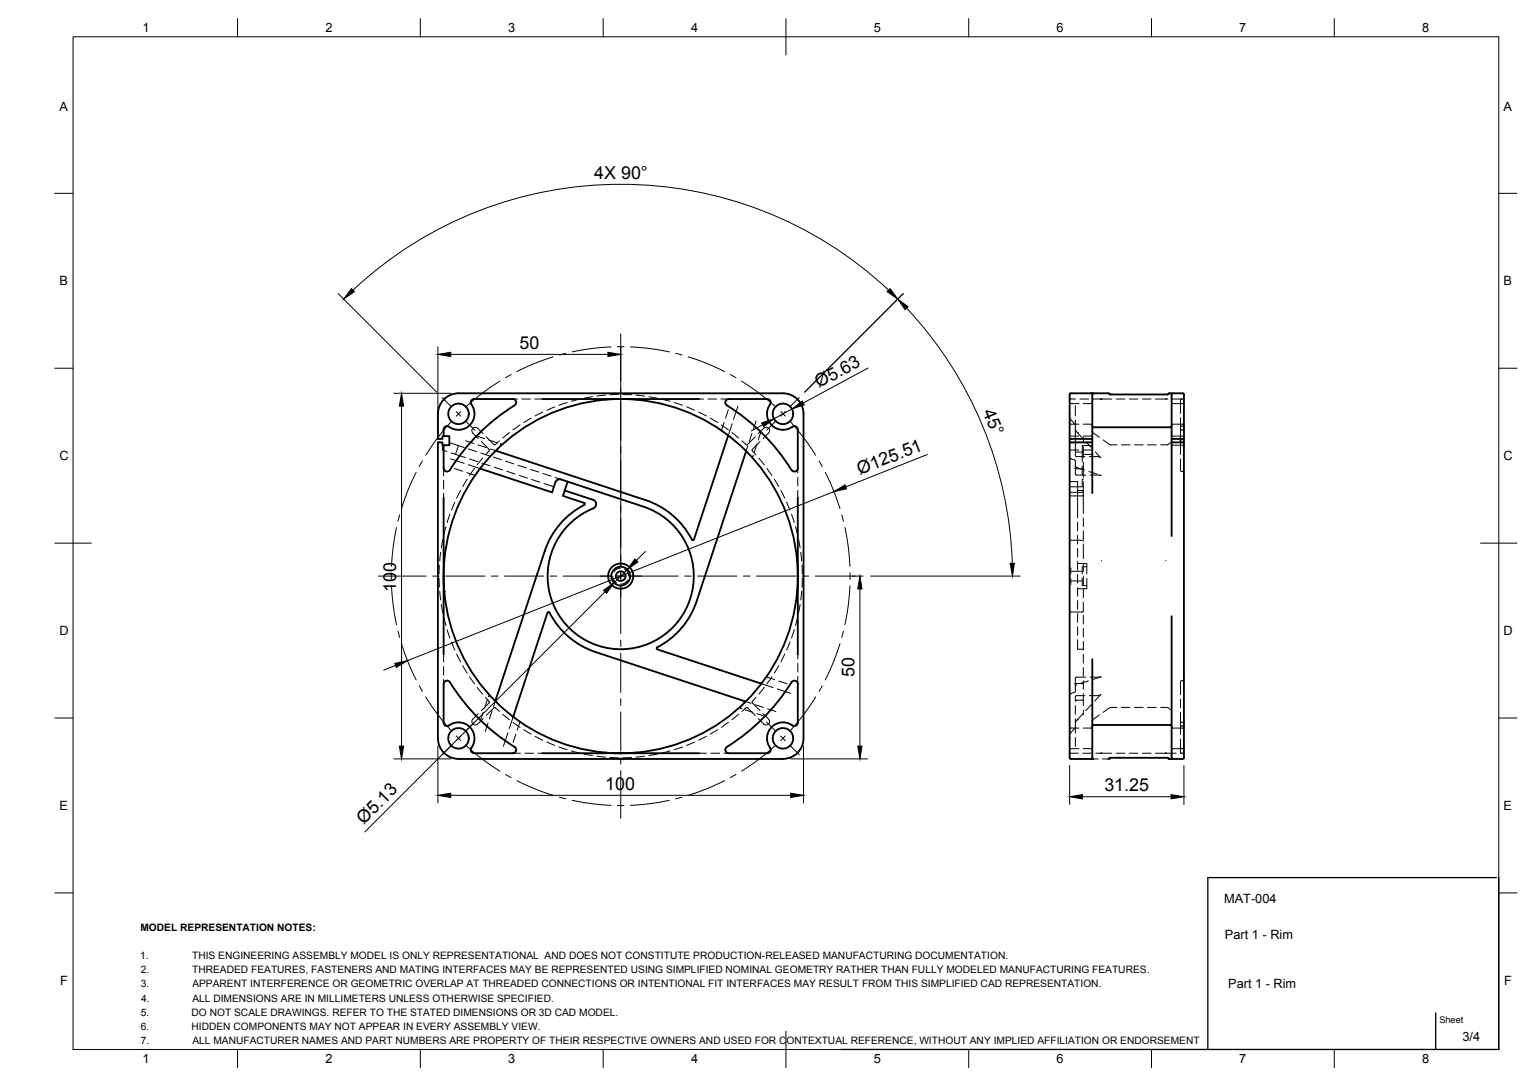
ISO-10303-21;
HEADER;
/* Generated by software containing ST-Developer
 * from STEP Tools, Inc. (www.steptools.com) 
 */

FILE_DESCRIPTION(
/* description */ ('STEP AP214'),
/* implementation_level */ '2;1');

FILE_NAME(
/* name */ 'Part 1 - Rim.step',
/* time_stamp */ '2026-11-14T05:34:33-08:00',
/* author */ (''),
/* organization */ (''),
/* preprocessor_version */ 'ST-DEVELOPER v20.2',
/* originating_system */ 'Autodesk Translation Framework v15.17.0.0',
/* authorisation */ '');

FILE_SCHEMA (('AUTOMOTIVE_DESIGN { 1 0 10303 214 3 1 1 }'));
ENDSEC;

DATA;
#10=MECHANICAL_DESIGN_GEOMETRIC_PRESENTATION_REPRESENTATION('',(#23),#37625);
#19=SHAPE_REPRESENTATION_RELATIONSHIP('SRR','None',#37639,#21);
#21=ADVANCED_BREP_SHAPE_REPRESENTATION('',(#25),#37623);
#23=STYLED_ITEM('',(#37658),#25);
#25=MANIFOLD_SOLID_BREP('Body1',#11497);
#27=SPHERICAL_SURFACE('',#12271,0.3125);
#28=SPHERICAL_SURFACE('',#12276,0.3125);
#29=SPHERICAL_SURFACE('',#12302,0.3125);
#30=SPHERICAL_SURFACE('',#12304,0.3125);
#31=SPHERICAL_SURFACE('',#12340,0.3125);
#32=SPHERICAL_SURFACE('',#12342,0.3125);
#33=SPHERICAL_SURFACE('',#12382,0.3125);
#34=SPHERICAL_SURFACE('',#12385,0.3125);
#35=SPHERICAL_SURFACE('',#12394,0.3125);
#36=SPHERICAL_SURFACE('',#12396,0.3125);
#37=SPHERICAL_SURFACE('',#12445,0.3125);
#38=SPHERICAL_SURFACE('',#12447,0.3125);
#39=SPHERICAL_SURFACE('',#12466,0.3125);
#40=SPHERICAL_SURFACE('',#12481,0.3125);
#41=SPHERICAL_SURFACE('',#12525,0.3125);
#42=SPHERICAL_SURFACE('',#12532,0.3125);
#43=SPHERICAL_SURFACE('',#12539,0.3125);
#44=SPHERICAL_SURFACE('',#12541,0.3125);
#45=SPHERICAL_SURFACE('',#12549,0.3125);
#46=SPHERICAL_SURFACE('',#12552,0.3125);
#47=SPHERICAL_SURFACE('',#12570,0.3125);
#48=SPHERICAL_SURFACE('',#12573,0.3125);
#49=SPHERICAL_SURFACE('',#12575,0.3125);
#50=SPHERICAL_SURFACE('',#12580,0.3125);
#51=SPHERICAL_SURFACE('',#12597,0.3125);
#52=SPHERICAL_SURFACE('',#12605,0.3125);
#53=SPHERICAL_SURFACE('',#12628,0.3125);
#54=SPHERICAL_SURFACE('',#12633,0.3125);
#55=SPHERICAL_SURFACE('',#12637,0.3125);
#56=SPHERICAL_SURFACE('',#12640,0.3125);
#57=SPHERICAL_SURFACE('',#12665,0.3125);
#58=SPHERICAL_SURFACE('',#12668,0.3125);
#59=SPHERICAL_SURFACE('',#12674,0.3125);
#60=SPHERICAL_SURFACE('',#12676,0.3125);
#61=SPHERICAL_SURFACE('',#12702,0.3125);
#62=SPHERICAL_SURFACE('',#12704,0.3125);
#63=SPHERICAL_SURFACE('',#12706,0.3125);
#64=SPHERICAL_SURFACE('',#12711,0.3125);
#65=SPHERICAL_SURFACE('',#12733,0.3125);
#66=SPHERICAL_SURFACE('',#12735,0.3125);
#67=SPHERICAL_SURFACE('',#12759,0.3125);
#68=SPHERICAL_SURFACE('',#12761,0.3125);
#69=SPHERICAL_SURFACE('',#12763,0.3125);
#70=SPHERICAL_SURFACE('',#12765,0.3125);
#71=SPHERICAL_SURFACE('',#12779,0.3125);
#72=SPHERICAL_SURFACE('',#12781,0.3125);
#73=SPHERICAL_SURFACE('',#12788,0.3125);
#74=SPHERICAL_SURFACE('',#12790,0.3125);
#75=(
BOUNDED_SURFACE()
B_SPLINE_SURFACE(3,2,((#23896,#23897,#23898),(#23899,#23900,#23901),(#23902,
#23903,#23904),(#23905,#23906,#23907)),.UNSPECIFIED.,.F.,.F.,.F.)
B_SPLINE_SURFACE_WITH_KNOTS((4,4),(3,3),(0.0326127356995135,0.0421285143028756),
(0.,1.),.UNSPECIFIED.)
GEOMETRIC_REPRESENTATION_ITEM()
RATIONAL_B_SPLINE_SURFACE(((1.,0.77336849210705,1.),(1.,0.770480922349025,
1.),(1.,0.767957745429666,1.),(1.,0.765689104422505,1.)))
REPRESENTATION_ITEM('')
SURFACE()
);
#76=(
BOUNDED_SURFACE()
B_SPLINE_SURFACE(3,2,((#23985,#23986,#23987),(#23988,#23989,#23990),(#23991,
#23992,#23993),(#23994,#23995,#23996),(#23997,#23998,#23999),(#24000,#24001,
#24002),(#24003,#24004,#24005),(#24006,#24007,#24008)),.UNSPECIFIED.,.F.,
 .F.,.F.)
B_SPLINE_SURFACE_WITH_KNOTS((4,2,2,4),(3,3),(0.000802853902805026,0.00108948501086238,
0.00137611611891974,0.00194937833503446),(0.,1.),.UNSPECIFIED.)
GEOMETRIC_REPRESENTATION_ITEM()
RATIONAL_B_SPLINE_SURFACE(((1.,0.923879532511285,1.),(1.,0.93126028758527,
1.),(1.,0.931596165488004,1.),(1.,0.918734528780574,1.),(1.,0.905994810924641,
1.),(1.,0.858462949893107,1.),(1.,0.814112175968656,1.),(1.,0.765689104422502,
1.)))
REPRESENTATION_ITEM('')
SURFACE()
);
#77=(
BOUNDED_SURFACE()
B_SPLINE_SURFACE(3,2,((#24068,#24069,#24070),(#24071,#24072,#24073),(#24074,
#24075,#24076),(#24077,#24078,#24079),(#24080,#24081,#24082),(#24083,#24084,
#24085),(#24086,#24087,#24088),(#24089,#24090,#24091)),.UNSPECIFIED.,.F.,
 .F.,.F.)
B_SPLINE_SURFACE_WITH_KNOTS((4,2,2,4),(3,3),(0.000686358375502128,0.000929437613321109,
0.00117251685114009,0.00165867532677805),(0.,1.),.UNSPECIFIED.)
GEOMETRIC_REPRESENTATION_ITEM()
RATIONAL_B_SPLINE_SURFACE(((1.,0.923879532511287,1.),(1.,0.92889985757716,
1.),(1.,0.929018384212628,1.),(1.,0.920008474882563,1.),(1.,0.910871684991149,
1.),(1.,0.87513924549097,1.),(1.,0.84081307837336,1.),(1.,0.802338883728525,
1.)))
REPRESENTATION_ITEM('')
SURFACE()
);
#78=(
BOUNDED_SURFACE()
B_SPLINE_SURFACE(3,2,((#24101,#24102,#24103),(#24104,#24105,#24106),(#24107,
#24108,#24109),(#24110,#24111,#24112),(#24113,#24114,#24115),(#24116,#24117,
#24118),(#24119,#24120,#24121),(#24122,#24123,#24124),(#24125,#24126,#24127),
(#24128,#24129,#24130)),.UNSPECIFIED.,.F.,.F.,.F.)
B_SPLINE_SURFACE_WITH_KNOTS((4,2,2,2,4),(3,3),(0.0314170682308584,0.0383717968941293,
0.0418491612257648,0.0453265255574003,0.0592359828839421),(0.,1.00015514532272),
 .UNSPECIFIED.)
GEOMETRIC_REPRESENTATION_ITEM()
RATIONAL_B_SPLINE_SURFACE(((1.,0.893712741719904,1.00003297994197),(1.,
0.896924595267972,1.00003198333386),(1.,0.900137133821891,1.0000309865132),
(1.,0.904798383538125,1.00002954017102),(1.,0.906325496636901,1.00002906632211),
(1.,0.909290323001115,1.00002814636422),(1.,0.910726187593686,1.00002770082887),
(1.,0.917498844645671,1.00002559933674),(1.,0.921671404518462,1.00002430463045),
(1.,0.923199103012375,1.0000238305999)))
REPRESENTATION_ITEM('')
SURFACE()
);
#79=(
BOUNDED_SURFACE()
B_SPLINE_SURFACE(3,2,((#24156,#24157,#24158),(#24159,#24160,#24161),(#24162,
#24163,#24164),(#24165,#24166,#24167),(#24168,#24169,#24170),(#24171,#24172,
#24173),(#24174,#24175,#24176),(#24177,#24178,#24179),(#24180,#24181,#24182),
(#24183,#24184,#24185)),.UNSPECIFIED.,.F.,.F.,.F.)
B_SPLINE_SURFACE_WITH_KNOTS((4,2,2,2,4),(3,3),(0.0303364035364412,0.0372910338575461,
0.0407683490180985,0.0442456641786509,0.0581549248208605),(0.,1.),
 .UNSPECIFIED.)
GEOMETRIC_REPRESENTATION_ITEM()
RATIONAL_B_SPLINE_SURFACE(((1.,0.893729285230293,1.),(1.,0.8969398694082,
1.),(1.,0.900150686104865,1.),(1.,0.904808789101856,1.),(1.,0.906334760566901,
1.),(1.,0.909297199463308,1.),(1.,0.91073457572851,1.),(1.,0.917512859277436,
1.),(1.,0.921684639637439,1.),(1.,0.923210992612934,1.)))
REPRESENTATION_ITEM('')
SURFACE()
);
#80=(
BOUNDED_SURFACE()
B_SPLINE_SURFACE(3,2,((#24220,#24221,#24222),(#24223,#24224,#24225),(#24226,
#24227,#24228),(#24229,#24230,#24231),(#24232,#24233,#24234),(#24235,#24236,
#24237)),.UNSPECIFIED.,.F.,.F.,.F.)
B_SPLINE_SURFACE_WITH_KNOTS((4,2,4),(3,3),(0.000158496916905221,0.000711650690198974,
0.00126480446349273),(0.,1.),.UNSPECIFIED.)
GEOMETRIC_REPRESENTATION_ITEM()
RATIONAL_B_SPLINE_SURFACE(((1.,0.707106781186549,1.),(1.,0.750150820630032,
1.),(1.,0.789088418359452,1.),(1.,0.861437064777228,1.),(1.,0.895323131481853,
1.),(1.,0.92387953251129,1.)))
REPRESENTATION_ITEM('')
SURFACE()
);
#81=(
BOUNDED_SURFACE()
B_SPLINE_SURFACE(3,2,((#24242,#24243,#24244),(#24245,#24246,#24247),(#24248,
#24249,#24250),(#24251,#24252,#24253),(#24254,#24255,#24256),(#24257,#24258,
#24259),(#24260,#24261,#24262),(#24263,#24264,#24265)),.UNSPECIFIED.,.F.,
 .F.,.F.)
B_SPLINE_SURFACE_WITH_KNOTS((4,2,2,4),(3,3),(0.000174437971377146,0.00101920216019031,
0.00137118723886246,0.00186396634900332),(0.,1.00024356555363),
 .UNSPECIFIED.)
GEOMETRIC_REPRESENTATION_ITEM()
RATIONAL_B_SPLINE_SURFACE(((1.,0.539098756316927,1.00022451933317),(1.,
0.633858154865208,1.00017835908243),(1.,0.717178341053912,1.00013777122788),
(1.,0.814824555144991,1.00009020471949),(1.,0.841538081526998,1.0000771917298),
(1.,0.898531920368047,1.00004942825798),(1.,0.925786672706503,1.0000361516203),
(1.,0.937456960617578,1.00003046666003)))
REPRESENTATION_ITEM('')
SURFACE()
);
#82=(
BOUNDED_SURFACE()
B_SPLINE_SURFACE(3,2,((#24441,#24442,#24443),(#24444,#24445,#24446),(#24447,
#24448,#24449),(#24450,#24451,#24452),(#24453,#24454,#24455),(#24456,#24457,
#24458)),.UNSPECIFIED.,.F.,.F.,.F.)
B_SPLINE_SURFACE_WITH_KNOTS((4,2,4),(3,3),(0.000796035510927852,0.00146280219164561,
0.00212956887236337),(0.,1.00047905246342),.UNSPECIFIED.)
GEOMETRIC_REPRESENTATION_ITEM()
RATIONAL_B_SPLINE_SURFACE(((1.,0.680382792871542,1.00030622682085),(1.,
0.734649451169007,1.00025423366818),(1.,0.782184849656497,1.00020868976868),
(1.,0.8686687938328,1.00012582907568),(1.,0.90836300942771,1.00008779785215),
(1.,0.940539343963641,1.0000569695475)))
REPRESENTATION_ITEM('')
SURFACE()
);
#83=(
BOUNDED_SURFACE()
B_SPLINE_SURFACE(3,2,((#24462,#24463,#24464),(#24465,#24466,#24467),(#24468,
#24469,#24470),(#24471,#24472,#24473)),.UNSPECIFIED.,.F.,.F.,.F.)
B_SPLINE_SURFACE_WITH_KNOTS((4,4),(3,3),(0.0647248597593566,0.0667277597197425),
(0.,1.),.UNSPECIFIED.)
GEOMETRIC_REPRESENTATION_ITEM()
RATIONAL_B_SPLINE_SURFACE(((1.,0.77254330703138,1.),(1.,0.773053168552101,
1.),(1.,0.773574707201174,1.),(1.,0.774108727913442,1.)))
REPRESENTATION_ITEM('')
SURFACE()
);
#84=(
BOUNDED_SURFACE()
B_SPLINE_SURFACE(3,2,((#24557,#24558,#24559),(#24560,#24561,#24562),(#24563,
#24564,#24565),(#24566,#24567,#24568)),.UNSPECIFIED.,.F.,.F.,.F.)
B_SPLINE_SURFACE_WITH_KNOTS((4,4),(3,3),(0.0554293707990946,0.067219986976584),
(0.,1.00093204202966),.UNSPECIFIED.)
GEOMETRIC_REPRESENTATION_ITEM()
RATIONAL_B_SPLINE_SURFACE(((1.,0.586730971631016,1.00077036820799),(1.,
0.580458668850621,1.00078206030762),(1.,0.573277155045983,1.00079544725303),
(1.,0.564689221730742,1.00081145588262)))
REPRESENTATION_ITEM('')
SURFACE()
);
#85=(
BOUNDED_SURFACE()
B_SPLINE_SURFACE(3,2,((#24588,#24589,#24590),(#24591,#24592,#24593),(#24594,
#24595,#24596),(#24597,#24598,#24599),(#24600,#24601,#24602),(#24603,#24604,
#24605),(#24606,#24607,#24608),(#24609,#24610,#24611),(#24612,#24613,#24614),
(#24615,#24616,#24617)),.UNSPECIFIED.,.F.,.F.,.F.)
B_SPLINE_SURFACE_WITH_KNOTS((4,2,2,2,4),(3,3),(0.000140109886117696,0.000666559814939625,
0.00108521714444999,0.00150387447396035,0.00203032440278269),(-0.000871030384560204,
1.),.UNSPECIFIED.)
GEOMETRIC_REPRESENTATION_ITEM()
RATIONAL_B_SPLINE_SURFACE(((1.00092572483597,0.468603591574399,1.),(1.00081905401985,
0.5298361375373,1.),(1.00071568618447,0.589172664263207,1.),(1.00054995854446,
0.684305763488853,1.),(1.00048250324099,0.723027319401472,1.),(1.00035800741942,
0.794492002940391,1.),(1.00030258788071,0.826304635251683,1.),(1.00018948908564,
0.891227051893231,1.),(1.00013836850255,0.920571942721851,1.),(1.00011502671673,
0.933970893113149,1.)))
REPRESENTATION_ITEM('')
SURFACE()
);
#86=(
BOUNDED_SURFACE()
B_SPLINE_SURFACE(3,2,((#24621,#24622,#24623),(#24624,#24625,#24626),(#24627,
#24628,#24629),(#24630,#24631,#24632)),.UNSPECIFIED.,.F.,.F.,.F.)
B_SPLINE_SURFACE_WITH_KNOTS((4,4),(3,3),(0.0554293708282248,0.0672199869474538),
(0.,1.00093204200053),.UNSPECIFIED.)
GEOMETRIC_REPRESENTATION_ITEM()
RATIONAL_B_SPLINE_SURFACE(((1.,0.586730971596549,1.00077036818398),(1.,
0.580458668842862,1.00078206028319),(1.,0.573277155072649,1.00079544722812),
(1.,0.564689221807079,1.00081145585712)))
REPRESENTATION_ITEM('')
SURFACE()
);
#87=(
BOUNDED_SURFACE()
B_SPLINE_SURFACE(3,2,((#24651,#24652,#24653),(#24654,#24655,#24656),(#24657,
#24658,#24659),(#24660,#24661,#24662),(#24663,#24664,#24665),(#24666,#24667,
#24668)),.UNSPECIFIED.,.F.,.F.,.F.)
B_SPLINE_SURFACE_WITH_KNOTS((4,2,4),(3,3),(0.000315513320331966,0.000961720209151386,
0.00160792712680523),(-0.00216992936483643,1.),.UNSPECIFIED.)
GEOMETRIC_REPRESENTATION_ITEM()
RATIONAL_B_SPLINE_SURFACE(((1.00140856318051,0.675435706956244,1.),(1.00113480498433,
0.73851568564515,1.),(1.00088601384726,0.795842698473231,1.),(1.00048533380217,
0.888168294775817,1.),(1.00032603746989,0.924873713592471,1.),(1.00031273915803,
0.927937940493073,1.)))
REPRESENTATION_ITEM('')
SURFACE()
);
#88=(
BOUNDED_SURFACE()
B_SPLINE_SURFACE(3,2,((#24670,#24671,#24672),(#24673,#24674,#24675),(#24676,
#24677,#24678),(#24679,#24680,#24681),(#24682,#24683,#24684),(#24685,#24686,
#24687)),.UNSPECIFIED.,.F.,.F.,.F.)
B_SPLINE_SURFACE_WITH_KNOTS((4,2,4),(3,3),(0.000402895580047919,0.000905401753400751,
0.00140790792675358),(0.,1.),.UNSPECIFIED.)
GEOMETRIC_REPRESENTATION_ITEM()
RATIONAL_B_SPLINE_SURFACE(((1.,0.813540597401216,1.),(1.,0.813784197152837,
1.),(1.,0.801974141898952,1.),(1.,0.763153562323537,1.),(1.,0.735816595983232,
1.),(1.,0.707106781186551,1.)))
REPRESENTATION_ITEM('')
SURFACE()
);
#89=(
BOUNDED_SURFACE()
B_SPLINE_SURFACE(3,2,((#24694,#24695,#24696),(#24697,#24698,#24699),(#24700,
#24701,#24702),(#24703,#24704,#24705),(#24706,#24707,#24708),(#24709,#24710,
#24711)),.UNSPECIFIED.,.F.,.F.,.F.)
B_SPLINE_SURFACE_WITH_KNOTS((4,2,4),(3,3),(0.000800222346544408,0.00146699934948425,
0.00213377635242409),(0.,1.0004790524742),.UNSPECIFIED.)
GEOMETRIC_REPRESENTATION_ITEM()
RATIONAL_B_SPLINE_SURFACE(((1.,0.680382792868073,1.00030622682775),(1.,
0.73464945116617,1.0002542336739),(1.,0.782184849654142,1.00020868977338),
(1.,0.868668793831392,1.00012582907851),(1.,0.908363009426711,1.00008779785413),
(1.,0.940539343963006,1.00005696954878)))
REPRESENTATION_ITEM('')
SURFACE()
);
#90=(
BOUNDED_SURFACE()
B_SPLINE_SURFACE(3,2,((#24741,#24742,#24743),(#24744,#24745,#24746),(#24747,
#24748,#24749),(#24750,#24751,#24752),(#24753,#24754,#24755),(#24756,#24757,
#24758),(#24759,#24760,#24761),(#24762,#24763,#24764),(#24765,#24766,#24767),
(#24768,#24769,#24770)),.UNSPECIFIED.,.F.,.F.,.F.)
B_SPLINE_SURFACE_WITH_KNOTS((4,2,2,2,4),(3,3),(0.0314170682308576,0.0383717968941285,
0.041849161225764,0.0453265255573995,0.0592359828839414),(0.,1.00015514533033),
 .UNSPECIFIED.)
GEOMETRIC_REPRESENTATION_ITEM()
RATIONAL_B_SPLINE_SURFACE(((1.,0.893712741719095,1.00003297994359),(1.,
0.896924595266501,1.00003198333543),(1.,0.900137133822039,1.00003098651472),
(1.,0.904798383536946,1.00002954017247),(1.,0.906325496636188,1.00002906632354),
(1.,0.909290323000425,1.0000281463656),(1.,0.910726187593075,1.00002770083023),
(1.,0.917498844644786,1.000025599338),(1.,0.921671404518056,1.00002430463164),
(1.,0.923199103011791,1.00002383060107)))
REPRESENTATION_ITEM('')
SURFACE()
);
#91=(
BOUNDED_SURFACE()
B_SPLINE_SURFACE(3,2,((#24796,#24797,#24798),(#24799,#24800,#24801),(#24802,
#24803,#24804),(#24805,#24806,#24807),(#24808,#24809,#24810),(#24811,#24812,
#24813),(#24814,#24815,#24816),(#24817,#24818,#24819),(#24820,#24821,#24822),
(#24823,#24824,#24825)),.UNSPECIFIED.,.F.,.F.,.F.)
B_SPLINE_SURFACE_WITH_KNOTS((4,2,2,2,4),(3,3),(0.0303364035364412,0.0372910338575461,
0.0407683490180985,0.0442456641786509,0.0581549248208606),(0.,1.),
 .UNSPECIFIED.)
GEOMETRIC_REPRESENTATION_ITEM()
RATIONAL_B_SPLINE_SURFACE(((1.,0.893729285230296,1.),(1.,0.89693986940752,
1.),(1.,0.900150686105771,1.),(1.,0.904808789101402,1.),(1.,0.906334760567093,
1.),(1.,0.909297199463109,1.),(1.,0.91073457572825,1.),(1.,0.917512859278478,
1.),(1.,0.921684639636655,1.),(1.,0.923210992612934,1.)))
REPRESENTATION_ITEM('')
SURFACE()
);
#92=(
BOUNDED_SURFACE()
B_SPLINE_SURFACE(3,2,((#24827,#24828,#24829),(#24830,#24831,#24832),(#24833,
#24834,#24835),(#24836,#24837,#24838),(#24839,#24840,#24841),(#24842,#24843,
#24844),(#24845,#24846,#24847),(#24848,#24849,#24850),(#24851,#24852,#24853),
(#24854,#24855,#24856)),.UNSPECIFIED.,.F.,.F.,.F.)
B_SPLINE_SURFACE_WITH_KNOTS((4,2,2,2,4),(3,3),(0.000140109886348097,0.00066655981493961,
0.00108521714444997,0.00150387447396033,0.00203032440255225),(-0.000871030383072034,
1.),.UNSPECIFIED.)
GEOMETRIC_REPRESENTATION_ITEM()
RATIONAL_B_SPLINE_SURFACE(((1.00092572483425,0.468603591655602,1.),(1.00081905401836,
0.529836137589938,1.),(1.00071568618321,0.589172664287011,1.),(1.00054995854352,
0.684305763489321,1.),(1.00048250324016,0.723027319402148,1.),(1.00035800741881,
0.794492002940432,1.),(1.00030258788019,0.826304635252028,1.),(1.00018948908534,
0.891227051877456,1.),(1.00013836850236,0.920571942696442,1.),(1.00011502671656,
0.933970893095549,1.)))
REPRESENTATION_ITEM('')
SURFACE()
);
#93=(
BOUNDED_SURFACE()
B_SPLINE_SURFACE(3,2,((#24858,#24859,#24860),(#24861,#24862,#24863),(#24864,
#24865,#24866),(#24867,#24868,#24869),(#24870,#24871,#24872),(#24873,#24874,
#24875),(#24876,#24877,#24878),(#24879,#24880,#24881)),.UNSPECIFIED.,.F.,
 .F.,.F.)
B_SPLINE_SURFACE_WITH_KNOTS((4,2,2,4),(3,3),(0.000174437971377159,0.00101920216019031,
0.00137118723886246,0.00186396634900331),(0.,1.00024356555507),
 .UNSPECIFIED.)
GEOMETRIC_REPRESENTATION_ITEM()
RATIONAL_B_SPLINE_SURFACE(((1.,0.53909875631573,1.0002245193345),(1.,0.633858154865746,
1.00017835908349),(1.,0.717178341052667,1.0001377712287),(1.,0.814824555145073,
1.00009020472002),(1.,0.841538081527084,1.00007719173026),(1.,0.89853192036746,
1.00004942825828),(1.,0.92578667270721,1.00003615162051),(1.,0.937456960616711,
1.00003046666021)))
REPRESENTATION_ITEM('')
SURFACE()
);
#94=(
BOUNDED_SURFACE()
B_SPLINE_SURFACE(3,2,((#24935,#24936,#24937),(#24938,#24939,#24940),(#24941,
#24942,#24943),(#24944,#24945,#24946),(#24947,#24948,#24949),(#24950,#24951,
#24952),(#24953,#24954,#24955),(#24956,#24957,#24958),(#24959,#24960,#24961),
(#24962,#24963,#24964)),.UNSPECIFIED.,.F.,.F.,.F.)
B_SPLINE_SURFACE_WITH_KNOTS((4,2,2,2,4),(3,3),(0.000329019594184255,0.000643209132708098,
0.000817758876492274,0.00116685836406063,0.00200469706399122),(-0.00396994925378904,
1.),.UNSPECIFIED.)
GEOMETRIC_REPRESENTATION_ITEM()
RATIONAL_B_SPLINE_SURFACE(((1.00073501708023,0.907427396013615,1.),(1.000615151231,
0.922524043548762,1.),(1.00054588724346,0.931247579180259,1.),(1.00054531256499,
0.931319957746567,1.),(1.00056655237271,0.928644884796654,1.),(1.00068340691792,
0.913927499543016,1.),(1.00082907221214,0.895581510097415,1.),(1.00142178903535,
0.820931081928685,1.),(1.00200380422997,0.747628483153123,1.),(1.00265356605592,
0.665793453986162,1.)))
REPRESENTATION_ITEM('')
SURFACE()
);
#95=(
BOUNDED_SURFACE()
B_SPLINE_SURFACE(3,2,((#25082,#25083,#25084),(#25085,#25086,#25087),(#25088,
#25089,#25090),(#25091,#25092,#25093)),.UNSPECIFIED.,.F.,.F.,.F.)
B_SPLINE_SURFACE_WITH_KNOTS((4,4),(3,3),(0.0650014074844314,0.0670796431839287),
(0.,1.),.UNSPECIFIED.)
GEOMETRIC_REPRESENTATION_ITEM()
RATIONAL_B_SPLINE_SURFACE(((1.,0.601781042690493,1.),(1.,0.600836260738882,
1.),(1.,0.599866989417514,1.),(1.,0.598871405423905,1.)))
REPRESENTATION_ITEM('')
SURFACE()
);
#96=(
BOUNDED_SURFACE()
B_SPLINE_SURFACE(3,2,((#25157,#25158,#25159),(#25160,#25161,#25162),(#25163,
#25164,#25165),(#25166,#25167,#25168),(#25169,#25170,#25171),(#25172,#25173,
#25174)),.UNSPECIFIED.,.F.,.F.,.F.)
B_SPLINE_SURFACE_WITH_KNOTS((4,2,4),(3,3),(0.000158380329178595,0.000711237088130122,
0.00126409384708165),(0.,1.),.UNSPECIFIED.)
GEOMETRIC_REPRESENTATION_ITEM()
RATIONAL_B_SPLINE_SURFACE(((1.,0.707106781186546,1.),(1.,0.750152861189045,
1.),(1.,0.789073569306456,1.),(1.,0.861356580931207,1.),(1.,0.895247679276223,
1.),(1.,0.923879532511291,1.)))
REPRESENTATION_ITEM('')
SURFACE()
);
#97=(
BOUNDED_SURFACE()
B_SPLINE_SURFACE(3,2,((#25243,#25244,#25245),(#25246,#25247,#25248),(#25249,
#25250,#25251),(#25252,#25253,#25254)),.UNSPECIFIED.,.F.,.F.,.F.)
B_SPLINE_SURFACE_WITH_KNOTS((4,4),(3,3),(0.0650014074844314,0.0670796431839287),
(0.,1.),.UNSPECIFIED.)
GEOMETRIC_REPRESENTATION_ITEM()
RATIONAL_B_SPLINE_SURFACE(((1.,0.601781042690495,1.),(1.,0.600836260738928,
1.),(1.,0.599866989417502,1.),(1.,0.598871405423905,1.)))
REPRESENTATION_ITEM('')
SURFACE()
);
#98=(
BOUNDED_SURFACE()
B_SPLINE_SURFACE(3,2,((#25256,#25257,#25258),(#25259,#25260,#25261),(#25262,
#25263,#25264),(#25265,#25266,#25267),(#25268,#25269,#25270),(#25271,#25272,
#25273)),.UNSPECIFIED.,.F.,.F.,.F.)
B_SPLINE_SURFACE_WITH_KNOTS((4,2,4),(3,3),(0.000402651921819617,0.000906087614430024,
0.00140952330704043),(0.,1.),.UNSPECIFIED.)
GEOMETRIC_REPRESENTATION_ITEM()
RATIONAL_B_SPLINE_SURFACE(((1.,0.813540597401216,1.),(1.,0.813739345537075,
1.),(1.,0.802648961762859,1.),(1.,0.764608789261971,1.),(1.,0.737258306119054,
1.),(1.,0.707106781186554,1.)))
REPRESENTATION_ITEM('')
SURFACE()
);
#99=(
BOUNDED_SURFACE()
B_SPLINE_SURFACE(3,2,((#25312,#25313,#25314),(#25315,#25316,#25317),(#25318,
#25319,#25320),(#25321,#25322,#25323),(#25324,#25325,#25326),(#25327,#25328,
#25329),(#25330,#25331,#25332),(#25333,#25334,#25335),(#25336,#25337,#25338),
(#25339,#25340,#25341)),.UNSPECIFIED.,.F.,.F.,.F.)
B_SPLINE_SURFACE_WITH_KNOTS((4,2,2,2,4),(3,3),(0.000758206618216268,0.00101809884720581,
0.00127799107619535,0.00153788330518489,0.00179777553417443),(0.,1.),
 .UNSPECIFIED.)
GEOMETRIC_REPRESENTATION_ITEM()
RATIONAL_B_SPLINE_SURFACE(((1.,0.707106781186548,1.),(1.,0.686991483272875,
1.),(1.,0.666460369298716,1.),(1.,0.62447089523074,1.),(1.,0.604201592515098,
1.),(1.,0.566291012805826,1.),(1.,0.549844363605541,1.),(1.,0.525862225699567,
1.),(1.,0.51912808872997,1.),(1.,0.51911513123826,1.)))
REPRESENTATION_ITEM('')
SURFACE()
);
#100=(
BOUNDED_SURFACE()
B_SPLINE_SURFACE(3,2,((#25342,#25343,#25344),(#25345,#25346,#25347),(#25348,
#25349,#25350),(#25351,#25352,#25353),(#25354,#25355,#25356),(#25357,#25358,
#25359),(#25360,#25361,#25362),(#25363,#25364,#25365),(#25366,#25367,#25368),
(#25369,#25370,#25371)),.UNSPECIFIED.,.F.,.F.,.F.)
B_SPLINE_SURFACE_WITH_KNOTS((4,2,2,2,4),(3,3),(0.000329019594184018,0.000643209132708091,
0.000817758876492263,0.00116685836406061,0.00200469706399384),(-0.00396994923486767,
1.),.UNSPECIFIED.)
GEOMETRIC_REPRESENTATION_ITEM()
RATIONAL_B_SPLINE_SURFACE(((1.00073501707671,0.907427396016355,1.),(1.00061515122806,
0.922524043549619,1.),(1.00054588724085,0.931247579181756,1.),(1.00054531256238,
0.93131995774775,1.),(1.00056655237,0.928644884798117,1.),(1.00068340691465,
0.913927499544403,1.),(1.00082907220817,0.895581510099604,1.),(1.00142178902855,
0.820931081931361,1.),(1.00200380422038,0.74762848315811,1.),(1.00265356604323,
0.665793453991339,1.)))
REPRESENTATION_ITEM('')
SURFACE()
);
#101=(
BOUNDED_SURFACE()
B_SPLINE_SURFACE(3,2,((#25375,#25376,#25377),(#25378,#25379,#25380),(#25381,
#25382,#25383),(#25384,#25385,#25386)),.UNSPECIFIED.,.F.,.F.,.F.)
B_SPLINE_SURFACE_WITH_KNOTS((4,4),(3,3),(0.0326127356995135,0.0421285143028756),
(0.,1.),.UNSPECIFIED.)
GEOMETRIC_REPRESENTATION_ITEM()
RATIONAL_B_SPLINE_SURFACE(((1.,0.773368492107047,1.),(1.,0.770480922349026,
1.),(1.,0.767957745429661,1.),(1.,0.765689104422504,1.)))
REPRESENTATION_ITEM('')
SURFACE()
);
#102=(
BOUNDED_SURFACE()
B_SPLINE_SURFACE(3,2,((#25464,#25465,#25466),(#25467,#25468,#25469),(#25470,
#25471,#25472),(#25473,#25474,#25475)),.UNSPECIFIED.,.F.,.F.,.F.)
B_SPLINE_SURFACE_WITH_KNOTS((4,4),(3,3),(0.0313106092150184,0.0408266168605713),
(0.,1.),.UNSPECIFIED.)
GEOMETRIC_REPRESENTATION_ITEM()
RATIONAL_B_SPLINE_SURFACE(((1.,0.773368492015519,1.),(1.,0.77048091928462,
1.),(1.,0.7679577451536,1.),(1.,0.765689104422504,1.)))
REPRESENTATION_ITEM('')
SURFACE()
);
#103=(
BOUNDED_SURFACE()
B_SPLINE_SURFACE(3,2,((#25567,#25568,#25569),(#25570,#25571,#25572),(#25573,
#25574,#25575),(#25576,#25577,#25578),(#25579,#25580,#25581),(#25582,#25583,
#25584)),.UNSPECIFIED.,.F.,.F.,.F.)
B_SPLINE_SURFACE_WITH_KNOTS((4,2,4),(3,3),(0.000315513320334842,0.000961720209151388,
0.00160792712680523),(-0.00216992936498931,1.),.UNSPECIFIED.)
GEOMETRIC_REPRESENTATION_ITEM()
RATIONAL_B_SPLINE_SURFACE(((1.0014085631806,0.675435706956732,1.),(1.0011348049844,
0.73851568564622,1.),(1.00088601384732,0.795842698472947,1.),(1.0004853338022,
0.888168294776257,1.),(1.00032603746992,0.924873713591867,1.),(1.00031273915805,
0.92793794049336,1.)))
REPRESENTATION_ITEM('')
SURFACE()
);
#104=(
BOUNDED_SURFACE()
B_SPLINE_SURFACE(3,2,((#25632,#25633,#25634),(#25635,#25636,#25637),(#25638,
#25639,#25640),(#25641,#25642,#25643),(#25644,#25645,#25646),(#25647,#25648,
#25649),(#25650,#25651,#25652),(#25653,#25654,#25655)),.UNSPECIFIED.,.F.,
 .F.,.F.)
B_SPLINE_SURFACE_WITH_KNOTS((4,2,2,4),(3,3),(0.000802853902805014,0.00108948501086237,
0.00137611611891973,0.00194937833503444),(0.,1.),.UNSPECIFIED.)
GEOMETRIC_REPRESENTATION_ITEM()
RATIONAL_B_SPLINE_SURFACE(((1.,0.923879532511287,1.),(1.,0.931260287585301,
1.),(1.,0.931596165487967,1.),(1.,0.918734528780613,1.),(1.,0.90599481092429,
1.),(1.,0.858462949893807,1.),(1.,0.81411217596811,1.),(1.,0.765689104422511,
1.)))
REPRESENTATION_ITEM('')
SURFACE()
);
#105=(
BOUNDED_SURFACE()
B_SPLINE_SURFACE(3,2,((#25715,#25716,#25717),(#25718,#25719,#25720),(#25721,
#25722,#25723),(#25724,#25725,#25726),(#25727,#25728,#25729),(#25730,#25731,
#25732),(#25733,#25734,#25735),(#25736,#25737,#25738)),.UNSPECIFIED.,.F.,
 .F.,.F.)
B_SPLINE_SURFACE_WITH_KNOTS((4,2,2,4),(3,3),(0.000686358375502152,0.000929437613321132,
0.00117251685114011,0.00165867532677807),(0.,1.),.UNSPECIFIED.)
GEOMETRIC_REPRESENTATION_ITEM()
RATIONAL_B_SPLINE_SURFACE(((1.,0.923879532511286,1.),(1.,0.928899857577065,
1.),(1.,0.929018384212755,1.),(1.,0.920008474882436,1.),(1.,0.910871684991113,
1.),(1.,0.875139245491043,1.),(1.,0.840813078373301,1.),(1.,0.802338883728528,
1.)))
REPRESENTATION_ITEM('')
SURFACE()
);
#106=(
BOUNDED_SURFACE()
B_SPLINE_SURFACE(3,2,((#25739,#25740,#25741),(#25742,#25743,#25744),(#25745,
#25746,#25747),(#25748,#25749,#25750),(#25751,#25752,#25753),(#25754,#25755,
#25756),(#25757,#25758,#25759),(#25760,#25761,#25762)),.UNSPECIFIED.,.F.,
 .F.,.F.)
B_SPLINE_SURFACE_WITH_KNOTS((4,2,2,4),(3,3),(0.000802853902805007,0.00108948501086237,
0.00137611611891972,0.00194937833503444),(0.,1.),.UNSPECIFIED.)
GEOMETRIC_REPRESENTATION_ITEM()
RATIONAL_B_SPLINE_SURFACE(((1.,0.923879532511287,1.),(1.,0.931260287585252,
1.),(1.,0.931596165488031,1.),(1.,0.918734528780548,1.),(1.,0.905994810924283,
1.),(1.,0.858462949893815,1.),(1.,0.814112175968112,1.),(1.,0.765689104422505,
1.)))
REPRESENTATION_ITEM('')
SURFACE()
);
#107=(
BOUNDED_SURFACE()
B_SPLINE_SURFACE(3,2,((#25822,#25823,#25824),(#25825,#25826,#25827),(#25828,
#25829,#25830),(#25831,#25832,#25833),(#25834,#25835,#25836),(#25837,#25838,
#25839),(#25840,#25841,#25842),(#25843,#25844,#25845)),.UNSPECIFIED.,.F.,
 .F.,.F.)
B_SPLINE_SURFACE_WITH_KNOTS((4,2,2,4),(3,3),(0.000686358375502721,0.000929437613321688,
0.00117251685114066,0.00165867532677859),(0.,1.),.UNSPECIFIED.)
GEOMETRIC_REPRESENTATION_ITEM()
RATIONAL_B_SPLINE_SURFACE(((1.,0.923879532511325,1.),(1.,0.928899857576951,
1.),(1.,0.929018384212867,1.),(1.,0.920008474882321,1.),(1.,0.910871684991292,
1.),(1.,0.875139245490692,1.),(1.,0.840813078373569,1.),(1.,0.802338883728525,
1.)))
REPRESENTATION_ITEM('')
SURFACE()
);
#108=(
BOUNDED_SURFACE()
B_SPLINE_SURFACE(3,2,((#25905,#25906,#25907),(#25908,#25909,#25910),(#25911,
#25912,#25913),(#25914,#25915,#25916),(#25917,#25918,#25919),(#25920,#25921,
#25922),(#25923,#25924,#25925),(#25926,#25927,#25928),(#25929,#25930,#25931),
(#25932,#25933,#25934)),.UNSPECIFIED.,.F.,.F.,.F.)
B_SPLINE_SURFACE_WITH_KNOTS((4,2,2,2,4),(3,3),(0.00051215679899462,0.000771582496110788,
0.00103100819322696,0.00129043389034312,0.00154985958745929),(0.,1.),
 .UNSPECIFIED.)
GEOMETRIC_REPRESENTATION_ITEM()
RATIONAL_B_SPLINE_SURFACE(((1.,0.707106781186548,1.),(1.,0.687254414974402,
1.),(1.,0.666880865311976,1.),(1.,0.625068437161317,1.),(1.,0.604779625068006,
1.),(1.,0.566741718306699,1.),(1.,0.550156755482303,1.),(1.,0.52595679230038,
1.),(1.,0.519123228378,1.),(1.,0.51911513123826,1.)))
REPRESENTATION_ITEM('')
SURFACE()
);
#109=(
BOUNDED_SURFACE()
B_SPLINE_SURFACE(3,2,((#25985,#25986,#25987),(#25988,#25989,#25990),(#25991,
#25992,#25993),(#25994,#25995,#25996)),.UNSPECIFIED.,.F.,.F.,.F.)
B_SPLINE_SURFACE_WITH_KNOTS((4,4),(3,3),(0.0647248597593566,0.0667277597197425),
(0.,1.),.UNSPECIFIED.)
GEOMETRIC_REPRESENTATION_ITEM()
RATIONAL_B_SPLINE_SURFACE(((1.,0.772543307031375,1.),(1.,0.773053168552095,
1.),(1.,0.773574707201188,1.),(1.,0.774108727913435,1.)))
REPRESENTATION_ITEM('')
SURFACE()
);
#110=(
BOUNDED_SURFACE()
B_SPLINE_SURFACE(3,2,((#26003,#26004,#26005),(#26006,#26007,#26008),(#26009,
#26010,#26011),(#26012,#26013,#26014),(#26015,#26016,#26017),(#26018,#26019,
#26020),(#26021,#26022,#26023),(#26024,#26025,#26026),(#26027,#26028,#26029),
(#26030,#26031,#26032)),.UNSPECIFIED.,.F.,.F.,.F.)
B_SPLINE_SURFACE_WITH_KNOTS((4,2,2,2,4),(3,3),(0.031417068230858,0.0383717968941289,
0.0418491612257644,0.0453265255573999,0.0592359828839417),(0.,1.00015514531871),
 .UNSPECIFIED.)
GEOMETRIC_REPRESENTATION_ITEM()
RATIONAL_B_SPLINE_SURFACE(((1.,0.893712741720332,1.00003297994112),(1.,
0.896924595268385,1.00003198333304),(1.,0.900137133822292,1.0000309865124),
(1.,0.904798383538507,1.00002954017025),(1.,0.906325496637147,1.00002906632136),
(1.,0.90929032300161,1.0000281463635),(1.,0.910726187594044,1.00002770082816),
(1.,0.917498844646002,1.00002559933608),(1.,0.921671404518776,1.00002430462982),
(1.,0.923199103012683,1.00002383059928)))
REPRESENTATION_ITEM('')
SURFACE()
);
#111=(
BOUNDED_SURFACE()
B_SPLINE_SURFACE(3,2,((#26058,#26059,#26060),(#26061,#26062,#26063),(#26064,
#26065,#26066),(#26067,#26068,#26069),(#26070,#26071,#26072),(#26073,#26074,
#26075),(#26076,#26077,#26078),(#26079,#26080,#26081),(#26082,#26083,#26084),
(#26085,#26086,#26087)),.UNSPECIFIED.,.F.,.F.,.F.)
B_SPLINE_SURFACE_WITH_KNOTS((4,2,2,2,4),(3,3),(0.03033640353644,0.0372910338575448,
0.0407683490180972,0.0442456641786496,0.0581549248208593),(0.,1.),
 .UNSPECIFIED.)
GEOMETRIC_REPRESENTATION_ITEM()
RATIONAL_B_SPLINE_SURFACE(((1.,0.893729285230292,1.),(1.,0.896939869408588,
1.),(1.,0.900150686104346,1.),(1.,0.904808789102115,1.),(1.,0.906334760566706,
1.),(1.,0.909297199463503,1.),(1.,0.91073457572825,1.),(1.,0.917512859278477,
1.),(1.,0.921684639636657,1.),(1.,0.923210992612934,1.)))
REPRESENTATION_ITEM('')
SURFACE()
);
#112=(
BOUNDED_SURFACE()
B_SPLINE_SURFACE(3,2,((#26122,#26123,#26124),(#26125,#26126,#26127),(#26128,
#26129,#26130),(#26131,#26132,#26133),(#26134,#26135,#26136),(#26137,#26138,
#26139)),.UNSPECIFIED.,.F.,.F.,.F.)
B_SPLINE_SURFACE_WITH_KNOTS((4,2,4),(3,3),(0.000158484458110993,0.000711605405373087,
0.00126472635263518),(0.,1.),.UNSPECIFIED.)
GEOMETRIC_REPRESENTATION_ITEM()
RATIONAL_B_SPLINE_SURFACE(((1.,0.707106781186548,1.),(1.,0.750150943531002,
1.),(1.,0.789086629669813,1.),(1.,0.861428008632711,1.),(1.,0.895315681224068,
1.),(1.,0.923879532511287,1.)))
REPRESENTATION_ITEM('')
SURFACE()
);
#113=(
BOUNDED_SURFACE()
B_SPLINE_SURFACE(3,2,((#26146,#26147,#26148),(#26149,#26150,#26151),(#26152,
#26153,#26154),(#26155,#26156,#26157),(#26158,#26159,#26160),(#26161,#26162,
#26163),(#26164,#26165,#26166),(#26167,#26168,#26169),(#26170,#26171,#26172),
(#26173,#26174,#26175)),.UNSPECIFIED.,.F.,.F.,.F.)
B_SPLINE_SURFACE_WITH_KNOTS((4,2,2,2,4),(3,3),(0.000758206618216247,0.00101809884720579,
0.00127799107619532,0.00153788330518486,0.0017977755341744),(0.,1.),
 .UNSPECIFIED.)
GEOMETRIC_REPRESENTATION_ITEM()
RATIONAL_B_SPLINE_SURFACE(((1.,0.707106781186548,1.),(1.,0.686991483272796,
1.),(1.,0.666460369298813,1.),(1.,0.624470895230632,1.),(1.,0.604201592515102,
1.),(1.,0.56629101280583,1.),(1.,0.549844363605635,1.),(1.,0.525862225699477,
1.),(1.,0.519128088730044,1.),(1.,0.51911513123826,1.)))
REPRESENTATION_ITEM('')
SURFACE()
);
#114=(
BOUNDED_SURFACE()
B_SPLINE_SURFACE(3,2,((#26306,#26307,#26308),(#26309,#26310,#26311),(#26312,
#26313,#26314),(#26315,#26316,#26317),(#26318,#26319,#26320),(#26321,#26322,
#26323)),.UNSPECIFIED.,.F.,.F.,.F.)
B_SPLINE_SURFACE_WITH_KNOTS((4,2,4),(3,3),(0.0008282178255691,0.00149505479343247,
0.00216189176129584),(0.,1.00047905254905),.UNSPECIFIED.)
GEOMETRIC_REPRESENTATION_ITEM()
RATIONAL_B_SPLINE_SURFACE(((1.,0.680382792843981,1.00030622687562),(1.,
0.734649451146706,1.00025423371364),(1.,0.782184849637538,1.00020868980601),
(1.,0.868668793821875,1.00012582909818),(1.,0.908363009419454,1.00008779786785),
(1.,0.940539343958763,1.00005696955769)))
REPRESENTATION_ITEM('')
SURFACE()
);
#115=(
BOUNDED_SURFACE()
B_SPLINE_SURFACE(3,2,((#26327,#26328,#26329),(#26330,#26331,#26332),(#26333,
#26334,#26335),(#26336,#26337,#26338)),.UNSPECIFIED.,.F.,.F.,.F.)
B_SPLINE_SURFACE_WITH_KNOTS((4,4),(3,3),(0.0647248597593566,0.0667277597197425),
(0.,1.),.UNSPECIFIED.)
GEOMETRIC_REPRESENTATION_ITEM()
RATIONAL_B_SPLINE_SURFACE(((1.,0.772543307031376,1.),(1.,0.773053168552096,
1.),(1.,0.773574707201185,1.),(1.,0.774108727913434,1.)))
REPRESENTATION_ITEM('')
SURFACE()
);
#116=(
BOUNDED_SURFACE()
B_SPLINE_SURFACE(3,2,((#26514,#26515,#26516),(#26517,#26518,#26519),(#26520,
#26521,#26522),(#26523,#26524,#26525)),.UNSPECIFIED.,.F.,.F.,.F.)
B_SPLINE_SURFACE_WITH_KNOTS((4,4),(3,3),(0.0554293708229056,0.0672199869527731),
(0.,1.00093204200585),.UNSPECIFIED.)
GEOMETRIC_REPRESENTATION_ITEM()
RATIONAL_B_SPLINE_SURFACE(((1.,0.586730971602853,1.00077036818836),(1.,
0.580458668844265,1.00078206028765),(1.,0.573277155067799,1.00079544723266),
(1.,0.564689221793136,1.00081145586177)))
REPRESENTATION_ITEM('')
SURFACE()
);
#117=(
BOUNDED_SURFACE()
B_SPLINE_SURFACE(3,2,((#26544,#26545,#26546),(#26547,#26548,#26549),(#26550,
#26551,#26552),(#26553,#26554,#26555),(#26556,#26557,#26558),(#26559,#26560,
#26561)),.UNSPECIFIED.,.F.,.F.,.F.)
B_SPLINE_SURFACE_WITH_KNOTS((4,2,4),(3,3),(0.000315513320331309,0.000961720209151386,
0.00160792712678291),(-0.00216992935563672,1.),.UNSPECIFIED.)
GEOMETRIC_REPRESENTATION_ITEM()
RATIONAL_B_SPLINE_SURFACE(((1.00140856317452,0.675435706958829,1.),(1.0011348049795,
0.738515685647825,1.),(1.00088601384349,0.795842698474753,1.),(1.00048533380011,
0.888168294775546,1.),(1.00032603746852,0.924873713590241,1.),(1.0003127391567,
0.927937940493613,1.)))
REPRESENTATION_ITEM('')
SURFACE()
);
#118=(
BOUNDED_SURFACE()
B_SPLINE_SURFACE(3,2,((#26563,#26564,#26565),(#26566,#26567,#26568),(#26569,
#26570,#26571),(#26572,#26573,#26574),(#26575,#26576,#26577),(#26578,#26579,
#26580)),.UNSPECIFIED.,.F.,.F.,.F.)
B_SPLINE_SURFACE_WITH_KNOTS((4,2,4),(3,3),(0.000402895580047916,0.000905401753400752,
0.00140790792675359),(0.,1.),.UNSPECIFIED.)
GEOMETRIC_REPRESENTATION_ITEM()
RATIONAL_B_SPLINE_SURFACE(((1.,0.813540597401216,1.),(1.,0.813784197152609,
1.),(1.,0.801974141899261,1.),(1.,0.763153562323214,1.),(1.,0.735816595983473,
1.),(1.,0.707106781186551,1.)))
REPRESENTATION_ITEM('')
SURFACE()
);
#119=(
BOUNDED_SURFACE()
B_SPLINE_SURFACE(3,2,((#26581,#26582,#26583),(#26584,#26585,#26586),(#26587,
#26588,#26589),(#26590,#26591,#26592),(#26593,#26594,#26595),(#26596,#26597,
#26598),(#26599,#26600,#26601),(#26602,#26603,#26604),(#26605,#26606,#26607),
(#26608,#26609,#26610)),.UNSPECIFIED.,.F.,.F.,.F.)
B_SPLINE_SURFACE_WITH_KNOTS((4,2,2,2,4),(3,3),(0.000512156798994636,0.000771582496110804,
0.00103100819322697,0.00129043389034314,0.00154985958745931),(0.,1.),
 .UNSPECIFIED.)
GEOMETRIC_REPRESENTATION_ITEM()
RATIONAL_B_SPLINE_SURFACE(((1.,0.707106781186548,1.),(1.,0.687254414974208,
1.),(1.,0.666880865312242,1.),(1.,0.625068437161066,1.),(1.,0.604779625068108,
1.),(1.,0.566741718306607,1.),(1.,0.550156755482368,1.),(1.,0.525956792300315,
1.),(1.,0.519123228378055,1.),(1.,0.51911513123826,1.)))
REPRESENTATION_ITEM('')
SURFACE()
);
#120=(
BOUNDED_SURFACE()
B_SPLINE_SURFACE(3,2,((#26613,#26614,#26615),(#26616,#26617,#26618),(#26619,
#26620,#26621),(#26622,#26623,#26624),(#26625,#26626,#26627),(#26628,#26629,
#26630)),.UNSPECIFIED.,.F.,.F.,.F.)
B_SPLINE_SURFACE_WITH_KNOTS((4,2,4),(3,3),(0.000402895580047916,0.000905401753400748,
0.00140790792675358),(0.,1.),.UNSPECIFIED.)
GEOMETRIC_REPRESENTATION_ITEM()
RATIONAL_B_SPLINE_SURFACE(((1.,0.813540597401212,1.),(1.,0.813784197152736,
1.),(1.,0.801974141899088,1.),(1.,0.763153562323395,1.),(1.,0.735816595983341,
1.),(1.,0.707106781186551,1.)))
REPRESENTATION_ITEM('')
SURFACE()
);
#121=(
BOUNDED_SURFACE()
B_SPLINE_SURFACE(3,2,((#26632,#26633,#26634),(#26635,#26636,#26637),(#26638,
#26639,#26640),(#26641,#26642,#26643),(#26644,#26645,#26646),(#26647,#26648,
#26649),(#26650,#26651,#26652),(#26653,#26654,#26655),(#26656,#26657,#26658),
(#26659,#26660,#26661)),.UNSPECIFIED.,.F.,.F.,.F.)
B_SPLINE_SURFACE_WITH_KNOTS((4,2,2,2,4),(3,3),(0.000140109886326165,0.000666559814939612,
0.00108521714444997,0.00150387447396033,0.00203032440257419),(-0.000871030383667572,
1.),.UNSPECIFIED.)
GEOMETRIC_REPRESENTATION_ITEM()
RATIONAL_B_SPLINE_SURFACE(((1.0009257248349,0.468603591646683,1.),(1.00081905401893,
0.529836137586218,1.),(1.0007156861837,0.58917266428352,1.),(1.0005499585439,
0.684305763489983,1.),(1.0004825032405,0.723027319401027,1.),(1.00035800741905,
0.794492002941265,1.),(1.0003025878804,0.82630463525224,1.),(1.00018948908547,
0.891227051878505,1.),(1.00013836850245,0.920571942699409,1.),(1.00011502671664,
0.933970893096821,1.)))
REPRESENTATION_ITEM('')
SURFACE()
);
#122=(
BOUNDED_SURFACE()
B_SPLINE_SURFACE(3,2,((#26662,#26663,#26664),(#26665,#26666,#26667),(#26668,
#26669,#26670),(#26671,#26672,#26673),(#26674,#26675,#26676),(#26677,#26678,
#26679),(#26680,#26681,#26682),(#26683,#26684,#26685)),.UNSPECIFIED.,.F.,
 .F.,.F.)
B_SPLINE_SURFACE_WITH_KNOTS((4,2,2,4),(3,3),(0.000174437971377122,0.00101920216019029,
0.00137118723886245,0.00186396634900331),(0.,1.00024356555371),
 .UNSPECIFIED.)
GEOMETRIC_REPRESENTATION_ITEM()
RATIONAL_B_SPLINE_SURFACE(((1.,0.539098756316595,1.00022451933325),(1.,
0.633858154865795,1.00017835908249),(1.,0.71717834105338,1.00013777122792),
(1.,0.814824555145193,1.00009020471952),(1.,0.841538081526984,1.00007719172983),
(1.,0.898531920368038,1.000049428258),(1.,0.925786672706506,1.00003615162031),
(1.,0.937456960617548,1.00003046666004)))
REPRESENTATION_ITEM('')
SURFACE()
);
#123=(
BOUNDED_SURFACE()
B_SPLINE_SURFACE(3,2,((#26739,#26740,#26741),(#26742,#26743,#26744),(#26745,
#26746,#26747),(#26748,#26749,#26750),(#26751,#26752,#26753),(#26754,#26755,
#26756),(#26757,#26758,#26759),(#26760,#26761,#26762),(#26763,#26764,#26765),
(#26766,#26767,#26768)),.UNSPECIFIED.,.F.,.F.,.F.)
B_SPLINE_SURFACE_WITH_KNOTS((4,2,2,2,4),(3,3),(0.000329019594182719,0.000643209132708097,
0.00081775887649227,0.00116685836406061,0.00200469706399139),(-0.00396994925120382,
1.),.UNSPECIFIED.)
GEOMETRIC_REPRESENTATION_ITEM()
RATIONAL_B_SPLINE_SURFACE(((1.00073501707975,0.907427396014608,1.),(1.0006151512306,
0.922524043548314,1.),(1.0005458872431,0.931247579180626,1.),(1.00054531256463,
0.93131995774664,1.),(1.00056655237234,0.928644884796926,1.),(1.00068340691748,
0.913927499543062,1.),(1.0008290722116,0.895581510097823,1.),(1.00142178903442,
0.820931081928786,1.),(1.00200380422865,0.747628483154187,1.),(1.00265356605419,
0.665793453986733,1.)))
REPRESENTATION_ITEM('')
SURFACE()
);
#124=(
BOUNDED_SURFACE()
B_SPLINE_SURFACE(3,2,((#26878,#26879,#26880),(#26881,#26882,#26883),(#26884,
#26885,#26886),(#26887,#26888,#26889)),.UNSPECIFIED.,.F.,.F.,.F.)
B_SPLINE_SURFACE_WITH_KNOTS((4,4),(3,3),(0.0650014074844314,0.0670796431839287),
(0.,1.),.UNSPECIFIED.)
GEOMETRIC_REPRESENTATION_ITEM()
RATIONAL_B_SPLINE_SURFACE(((1.,0.601781042690497,1.),(1.,0.600836260738914,
1.),(1.,0.599866989417508,1.),(1.,0.598871405423911,1.)))
REPRESENTATION_ITEM('')
SURFACE()
);
#125=(
BOUNDED_SURFACE()
B_SPLINE_SURFACE(3,2,((#26893,#26894,#26895),(#26896,#26897,#26898),(#26899,
#26900,#26901),(#26902,#26903,#26904),(#26905,#26906,#26907),(#26908,#26909,
#26910)),.UNSPECIFIED.,.F.,.F.,.F.)
B_SPLINE_SURFACE_WITH_KNOTS((4,2,4),(3,3),(0.000402651921819611,0.000906087614430015,
0.00140952330704042),(0.,1.),.UNSPECIFIED.)
GEOMETRIC_REPRESENTATION_ITEM()
RATIONAL_B_SPLINE_SURFACE(((1.,0.813540597401223,1.),(1.,0.81373934553701,
1.),(1.,0.802648961762943,1.),(1.,0.764608789261887,1.),(1.,0.737258306119129,
1.),(1.,0.707106781186548,1.)))
REPRESENTATION_ITEM('')
SURFACE()
);
#126=(
BOUNDED_SURFACE()
B_SPLINE_SURFACE(3,2,((#26948,#26949,#26950),(#26951,#26952,#26953),(#26954,
#26955,#26956),(#26957,#26958,#26959),(#26960,#26961,#26962),(#26963,#26964,
#26965)),.UNSPECIFIED.,.F.,.F.,.F.)
B_SPLINE_SURFACE_WITH_KNOTS((4,2,4),(3,3),(0.000351891753521461,0.000906087614430015,
0.00146028347533855),(0.,1.0000507601683),.UNSPECIFIED.)
GEOMETRIC_REPRESENTATION_ITEM()
RATIONAL_B_SPLINE_SURFACE(((1.,0.813123248342986,1.00001897179073),(1.,
0.815885817109806,1.00001869133382),(1.,0.804556789508961,1.00001984146051),
(1.,0.762678995446481,1.00002409290826),(1.,0.731644634342391,1.00002724352705),
(0.999999999999999,0.697891377178904,1.00003067016908)))
REPRESENTATION_ITEM('')
SURFACE()
);
#127=(
BOUNDED_SURFACE()
B_SPLINE_SURFACE(3,2,((#26983,#26984,#26985),(#26986,#26987,#26988),(#26989,
#26990,#26991),(#26992,#26993,#26994),(#26995,#26996,#26997),(#26998,#26999,
#27000),(#27001,#27002,#27003),(#27004,#27005,#27006),(#27007,#27008,#27009),
(#27010,#27011,#27012)),.UNSPECIFIED.,.F.,.F.,.F.)
B_SPLINE_SURFACE_WITH_KNOTS((4,2,2,2,4),(3,3),(0.000758206618216247,0.00101809884720579,
0.00127799107619532,0.00153788330518486,0.0017977755341744),(0.,1.),
 .UNSPECIFIED.)
GEOMETRIC_REPRESENTATION_ITEM()
RATIONAL_B_SPLINE_SURFACE(((1.,0.707106781186548,1.),(1.,0.686991483272722,
1.),(1.,0.666460369298913,1.),(1.,0.624470895230527,1.),(1.,0.604201592515,
1.),(1.,0.566291012805924,1.),(1.,0.54984436360562,1.),(1.,0.525862225699491,
1.),(1.,0.519128088730035,1.),(1.,0.51911513123826,1.)))
REPRESENTATION_ITEM('')
SURFACE()
);
#128=(
BOUNDED_SURFACE()
B_SPLINE_SURFACE(3,2,((#27110,#27111,#27112),(#27113,#27114,#27115),(#27116,
#27117,#27118),(#27119,#27120,#27121),(#27122,#27123,#27124),(#27125,#27126,
#27127),(#27128,#27129,#27130),(#27131,#27132,#27133),(#27134,#27135,#27136),
(#27137,#27138,#27139)),.UNSPECIFIED.,.F.,.F.,.F.)
B_SPLINE_SURFACE_WITH_KNOTS((4,2,2,2,4),(3,3),(0.000512156798994631,0.0007715824961108,
0.00103100819322697,0.00129043389034314,0.00154985958745931),(0.,1.),
 .UNSPECIFIED.)
GEOMETRIC_REPRESENTATION_ITEM()
RATIONAL_B_SPLINE_SURFACE(((1.,0.707106781186548,1.),(1.,0.687254414974094,
1.),(1.,0.666880865312397,1.),(1.,0.62506843716091,1.),(1.,0.604779625068046,
1.),(1.,0.56674171830669,1.),(1.,0.550156755482675,1.),(1.,0.525956792299999,
1.),(1.,0.519123228378293,1.),(1.,0.51911513123826,1.)))
REPRESENTATION_ITEM('')
SURFACE()
);
#129=(
BOUNDED_SURFACE()
B_SPLINE_SURFACE(3,2,((#27247,#27248,#27249),(#27250,#27251,#27252),(#27253,
#27254,#27255),(#27256,#27257,#27258),(#27259,#27260,#27261),(#27262,#27263,
#27264),(#27265,#27266,#27267),(#27268,#27269,#27270),(#27271,#27272,#27273),
(#27274,#27275,#27276)),.UNSPECIFIED.,.F.,.F.,.F.)
B_SPLINE_SURFACE_WITH_KNOTS((4,2,2,2,4),(3,3),(0.000758206618216244,0.00101809884720578,
0.00127799107619532,0.00153788330518486,0.0017977755341744),(0.,1.),
 .UNSPECIFIED.)
GEOMETRIC_REPRESENTATION_ITEM()
RATIONAL_B_SPLINE_SURFACE(((1.,0.707106781186548,1.),(1.,0.686991483272723,
1.),(1.,0.666460369298916,1.),(1.,0.62447089523053,1.),(1.,0.604201592515084,
1.),(1.,0.566291012805851,1.),(1.,0.549844363605341,1.),(1.,0.525862225699786,
1.),(1.,0.519128088729817,1.),(1.,0.519115131238269,1.)))
REPRESENTATION_ITEM('')
SURFACE()
);
#130=(
BOUNDED_SURFACE()
B_SPLINE_SURFACE(3,2,((#27282,#27283,#27284),(#27285,#27286,#27287),(#27288,
#27289,#27290),(#27291,#27292,#27293)),.UNSPECIFIED.,.F.,.F.,.F.)
B_SPLINE_SURFACE_WITH_KNOTS((4,4),(3,3),(0.0650014074844314,0.0670796431839287),
(0.,1.),.UNSPECIFIED.)
GEOMETRIC_REPRESENTATION_ITEM()
RATIONAL_B_SPLINE_SURFACE(((1.,0.601781042690495,1.),(1.,0.600836260738911,
1.),(1.,0.599866989417508,1.),(1.,0.598871405423905,1.)))
REPRESENTATION_ITEM('')
SURFACE()
);
#131=(
BOUNDED_SURFACE()
B_SPLINE_SURFACE(3,2,((#27355,#27356,#27357),(#27358,#27359,#27360),(#27361,
#27362,#27363),(#27364,#27365,#27366),(#27367,#27368,#27369),(#27370,#27371,
#27372),(#27373,#27374,#27375),(#27376,#27377,#27378)),.UNSPECIFIED.,.F.,
 .F.,.F.)
B_SPLINE_SURFACE_WITH_KNOTS((4,2,2,4),(3,3),(0.000174437971377159,0.00101920216019031,
0.00137118723886246,0.00186396634900331),(0.,1.00024356555379),
 .UNSPECIFIED.)
GEOMETRIC_REPRESENTATION_ITEM()
RATIONAL_B_SPLINE_SURFACE(((1.,0.53909875631675,1.00022451933332),(1.,0.633858154865377,
1.00017835908255),(1.,0.717178341053683,1.00013777122797),(1.,0.81482455514504,
1.00009020471955),(1.,0.841538081527261,1.00007719172985),(1.,0.898531920367626,
1.00004942825801),(1.,0.925786672707243,1.00003615162032),(1.,0.937456960616858,
1.00003046666005)))
REPRESENTATION_ITEM('')
SURFACE()
);
#132=(
BOUNDED_SURFACE()
B_SPLINE_SURFACE(3,2,((#27432,#27433,#27434),(#27435,#27436,#27437),(#27438,
#27439,#27440),(#27441,#27442,#27443),(#27444,#27445,#27446),(#27447,#27448,
#27449),(#27450,#27451,#27452),(#27453,#27454,#27455),(#27456,#27457,#27458),
(#27459,#27460,#27461)),.UNSPECIFIED.,.F.,.F.,.F.)
B_SPLINE_SURFACE_WITH_KNOTS((4,2,2,2,4),(3,3),(0.000329019594184677,0.000643209132708098,
0.000817758876492274,0.00116685836406063,0.0020046970639932),(-0.00396994925886359,
1.),.UNSPECIFIED.)
GEOMETRIC_REPRESENTATION_ITEM()
RATIONAL_B_SPLINE_SURFACE(((1.00073501708117,0.907427396013494,1.),(1.00061515123179,
0.922524043548232,1.),(1.00054588724416,0.931247579179964,1.),(1.00054531256569,
0.93131995774619,1.),(1.00056655237344,0.928644884796249,1.),(1.0006834069188,
0.913927499542673,1.),(1.0008290722132,0.89558151009713,1.),(1.00142178903718,
0.820931081927077,1.),(1.00200380423254,0.747628483152259,1.),(1.00265356605933,
0.665793453983509,1.)))
REPRESENTATION_ITEM('')
SURFACE()
);
#133=(
BOUNDED_SURFACE()
B_SPLINE_SURFACE(3,2,((#27466,#27467,#27468),(#27469,#27470,#27471),(#27472,
#27473,#27474),(#27475,#27476,#27477)),.UNSPECIFIED.,.F.,.F.,.F.)
B_SPLINE_SURFACE_WITH_KNOTS((4,4),(3,3),(0.0554293708055474,0.0672199869701312),
(0.,1.00093204202321),.UNSPECIFIED.)
GEOMETRIC_REPRESENTATION_ITEM()
RATIONAL_B_SPLINE_SURFACE(((1.,0.586730971623377,1.00077036820267),(1.,
0.580458668848917,1.00078206030221),(1.,0.573277155051876,1.00079544724751),
(1.,0.564689221747664,1.00081145587697)))
REPRESENTATION_ITEM('')
SURFACE()
);
#134=(
BOUNDED_SURFACE()
B_SPLINE_SURFACE(3,2,((#27492,#27493,#27494),(#27495,#27496,#27497),(#27498,
#27499,#27500),(#27501,#27502,#27503),(#27504,#27505,#27506),(#27507,#27508,
#27509),(#27510,#27511,#27512),(#27513,#27514,#27515),(#27516,#27517,#27518),
(#27519,#27520,#27521)),.UNSPECIFIED.,.F.,.F.,.F.)
B_SPLINE_SURFACE_WITH_KNOTS((4,2,2,2,4),(3,3),(0.000512156798994632,0.000771582496110797,
0.00103100819322696,0.00129043389034313,0.00154985958745929),(0.,1.),
 .UNSPECIFIED.)
GEOMETRIC_REPRESENTATION_ITEM()
RATIONAL_B_SPLINE_SURFACE(((1.,0.707106781186553,1.),(1.,0.687254414974218,
1.),(1.,0.66688086531225,1.),(1.,0.625068437161066,1.),(1.,0.604779625067387,
1.),(1.,0.566741718307357,1.),(1.,0.550156755482311,1.),(1.,0.525956792300389,
1.),(1.,0.519123228378017,1.),(1.,0.519115131238272,1.)))
REPRESENTATION_ITEM('')
SURFACE()
);
#135=(
BOUNDED_SURFACE()
B_SPLINE_SURFACE(3,2,((#27525,#27526,#27527),(#27528,#27529,#27530),(#27531,
#27532,#27533),(#27534,#27535,#27536),(#27537,#27538,#27539),(#27540,#27541,
#27542)),.UNSPECIFIED.,.F.,.F.,.F.)
B_SPLINE_SURFACE_WITH_KNOTS((4,2,4),(3,3),(0.00081372363230002,0.00148053147917474,
0.00214733932604946),(0.,1.00047905251364),.UNSPECIFIED.)
GEOMETRIC_REPRESENTATION_ITEM()
RATIONAL_B_SPLINE_SURFACE(((1.,0.680382792855505,1.00030622685297),(1.,
0.734649451155677,1.00025423369484),(1.,0.782184849645572,1.00020868979057),
(1.,0.868668793826199,1.00012582908887),(1.,0.908363009423125,1.00008779786136),
(1.,0.940539343960651,1.00005696955348)))
REPRESENTATION_ITEM('')
SURFACE()
);
#136=(
BOUNDED_SURFACE()
B_SPLINE_SURFACE(3,2,((#27569,#27570,#27571),(#27572,#27573,#27574),(#27575,
#27576,#27577),(#27578,#27579,#27580),(#27581,#27582,#27583),(#27584,#27585,
#27586),(#27587,#27588,#27589),(#27590,#27591,#27592),(#27593,#27594,#27595),
(#27596,#27597,#27598)),.UNSPECIFIED.,.F.,.F.,.F.)
B_SPLINE_SURFACE_WITH_KNOTS((4,2,2,2,4),(3,3),(0.00014010988641719,0.000666559814939611,
0.00108521714444997,0.00150387447396033,0.00203032440248315),(-0.000871030382132827,
1.),.UNSPECIFIED.)
GEOMETRIC_REPRESENTATION_ITEM()
RATIONAL_B_SPLINE_SURFACE(((1.00092572483321,0.468603591680183,1.),(1.00081905401745,
0.529836137605996,1.),(1.00071568618242,0.589172664294323,1.),(1.00054995854293,
0.684305763489641,1.),(1.00048250323964,0.723027319402385,1.),(1.00035800741842,
0.794492002940648,1.),(1.00030258787986,0.826304635252159,1.),(1.00018948908515,
0.89122705187285,1.),(1.00013836850222,0.920571942688749,1.),(1.00011502671645,
0.933970893090378,1.)))
REPRESENTATION_ITEM('')
SURFACE()
);
#137=(
BOUNDED_SURFACE()
B_SPLINE_SURFACE(3,2,((#27638,#27639,#27640),(#27641,#27642,#27643),(#27644,
#27645,#27646),(#27647,#27648,#27649),(#27650,#27651,#27652),(#27653,#27654,
#27655),(#27656,#27657,#27658),(#27659,#27660,#27661),(#27662,#27663,#27664),
(#27665,#27666,#27667)),.UNSPECIFIED.,.F.,.F.,.F.)
B_SPLINE_SURFACE_WITH_KNOTS((4,2,2,2,4),(3,3),(0.0314170682308593,0.0383717968941302,
0.0418491612257657,0.0453265255574011,0.059235982883943),(0.,1.00015514532807),
 .UNSPECIFIED.)
GEOMETRIC_REPRESENTATION_ITEM()
RATIONAL_B_SPLINE_SURFACE(((1.,0.893712741719336,1.00003297994311),(1.,
0.896924595267128,1.00003198333497),(1.,0.900137133821746,1.00003098651427),
(1.,0.904798383537421,1.00002954017204),(1.,0.90632549663627,1.00002906632311),
(1.,0.90929032300076,1.00002814636519),(1.,0.910726187593208,1.00002770082983),
(1.,0.917498844645229,1.00002559933763),(1.,0.921671404518043,1.00002430463129),
(1.,0.923199103011964,1.00002383060072)))
REPRESENTATION_ITEM('')
SURFACE()
);
#138=(
BOUNDED_SURFACE()
B_SPLINE_SURFACE(3,2,((#27693,#27694,#27695),(#27696,#27697,#27698),(#27699,
#27700,#27701),(#27702,#27703,#27704),(#27705,#27706,#27707),(#27708,#27709,
#27710),(#27711,#27712,#27713),(#27714,#27715,#27716),(#27717,#27718,#27719),
(#27720,#27721,#27722)),.UNSPECIFIED.,.F.,.F.,.F.)
B_SPLINE_SURFACE_WITH_KNOTS((4,2,2,2,4),(3,3),(0.030336403536441,0.0372910338575459,
0.0407683490180983,0.0442456641786507,0.0581549248208604),(0.,1.),
 .UNSPECIFIED.)
GEOMETRIC_REPRESENTATION_ITEM()
RATIONAL_B_SPLINE_SURFACE(((1.,0.893729285230291,1.),(1.,0.89693986940859,
1.),(1.,0.900150686104346,1.),(1.,0.904808789102114,1.),(1.,0.906334760566898,
1.),(1.,0.909297199463304,1.),(1.,0.91073457572851,1.),(1.,0.917512859277436,
1.),(1.,0.921684639637439,1.),(1.,0.923210992612934,1.)))
REPRESENTATION_ITEM('')
SURFACE()
);
#139=(
BOUNDED_SURFACE()
B_SPLINE_SURFACE(3,2,((#27724,#27725,#27726),(#27727,#27728,#27729),(#27730,
#27731,#27732),(#27733,#27734,#27735),(#27736,#27737,#27738),(#27739,#27740,
#27741)),.UNSPECIFIED.,.F.,.F.,.F.)
B_SPLINE_SURFACE_WITH_KNOTS((4,2,4),(3,3),(0.000351891754458639,0.000906087614430021,
0.00146028347440139),(0.,1.00005076016736),.UNSPECIFIED.)
GEOMETRIC_REPRESENTATION_ITEM()
RATIONAL_B_SPLINE_SURFACE(((1.,0.813123248357043,1.00001897179038),(1.,
0.815885817072131,1.00001869133348),(1.,0.804556789473276,1.00001984146015),
(1.,0.762678995482577,1.00002409290781),(1.,0.73164463444712,1.00002724352654),
(1.,0.697891377350557,1.00003067016849)))
REPRESENTATION_ITEM('')
SURFACE()
);
#140=(
BOUNDED_SURFACE()
B_SPLINE_SURFACE(3,2,((#27745,#27746,#27747),(#27748,#27749,#27750),(#27751,
#27752,#27753),(#27754,#27755,#27756),(#27757,#27758,#27759),(#27760,#27761,
#27762)),.UNSPECIFIED.,.F.,.F.,.F.)
B_SPLINE_SURFACE_WITH_KNOTS((4,2,4),(3,3),(0.000158430205536936,0.000711411267607371,
0.00126439232967781),(0.,1.),.UNSPECIFIED.)
GEOMETRIC_REPRESENTATION_ITEM()
RATIONAL_B_SPLINE_SURFACE(((1.,0.707106781186549,1.),(1.,0.750151746622362,
1.),(1.,0.789079409670008,1.),(1.,0.861389858264012,1.),(1.,0.895281520101449,
1.),(1.,0.92387953251129,1.)))
REPRESENTATION_ITEM('')
SURFACE()
);
#141=(
BOUNDED_SURFACE()
B_SPLINE_SURFACE(3,2,((#27872,#27873,#27874),(#27875,#27876,#27877),(#27878,
#27879,#27880),(#27881,#27882,#27883),(#27884,#27885,#27886),(#27887,#27888,
#27889)),.UNSPECIFIED.,.F.,.F.,.F.)
B_SPLINE_SURFACE_WITH_KNOTS((4,2,4),(3,3),(0.000402895580047922,0.000905401753400751,
0.00140790792675358),(0.,1.),.UNSPECIFIED.)
GEOMETRIC_REPRESENTATION_ITEM()
RATIONAL_B_SPLINE_SURFACE(((1.,0.813540597401209,1.),(1.,0.813784197152548,
1.),(1.,0.801974141899337,1.),(1.,0.763153562323141,1.),(1.,0.735816595983534,
1.),(1.,0.707106781186548,1.)))
REPRESENTATION_ITEM('')
SURFACE()
);
#142=(
BOUNDED_SURFACE()
B_SPLINE_SURFACE(3,2,((#27891,#27892,#27893),(#27894,#27895,#27896),(#27897,
#27898,#27899),(#27900,#27901,#27902),(#27903,#27904,#27905),(#27906,#27907,
#27908)),.UNSPECIFIED.,.F.,.F.,.F.)
B_SPLINE_SURFACE_WITH_KNOTS((4,2,4),(3,3),(0.000315513320329165,0.000961720209151403,
0.00160792712680524),(-0.00216992936573831,1.),.UNSPECIFIED.)
GEOMETRIC_REPRESENTATION_ITEM()
RATIONAL_B_SPLINE_SURFACE(((1.0014085631811,0.675435706954971,1.),(1.0011348049848,
0.738515685644707,1.),(1.00088601384763,0.795842698472626,1.),(1.00048533380237,
0.88816829477593,1.),(1.00032603747003,0.924873713592137,1.),(1.00031273915816,
0.927937940493142,1.)))
REPRESENTATION_ITEM('')
SURFACE()
);
#143=(
BOUNDED_SURFACE()
B_SPLINE_SURFACE(3,2,((#27955,#27956,#27957),(#27958,#27959,#27960),(#27961,
#27962,#27963),(#27964,#27965,#27966),(#27967,#27968,#27969),(#27970,#27971,
#27972),(#27973,#27974,#27975),(#27976,#27977,#27978)),.UNSPECIFIED.,.F.,
 .F.,.F.)
B_SPLINE_SURFACE_WITH_KNOTS((4,2,2,4),(3,3),(0.000686358375502124,0.000929437613321101,
0.00117251685114008,0.00165867532677803),(0.,1.),.UNSPECIFIED.)
GEOMETRIC_REPRESENTATION_ITEM()
RATIONAL_B_SPLINE_SURFACE(((1.,0.923879532511285,1.),(1.,0.928899857577083,
1.),(1.,0.929018384212736,1.),(1.,0.920008474882453,1.),(1.,0.91087168499111,
1.),(1.,0.875139245491054,1.),(1.,0.840813078373297,1.),(1.,0.802338883728532,
1.)))
REPRESENTATION_ITEM('')
SURFACE()
);
#144=(
BOUNDED_SURFACE()
B_SPLINE_SURFACE(3,2,((#28068,#28069,#28070),(#28071,#28072,#28073),(#28074,
#28075,#28076),(#28077,#28078,#28079)),.UNSPECIFIED.,.F.,.F.,.F.)
B_SPLINE_SURFACE_WITH_KNOTS((4,4),(3,3),(0.0647248597593566,0.0667277597197425),
(0.,1.),.UNSPECIFIED.)
GEOMETRIC_REPRESENTATION_ITEM()
RATIONAL_B_SPLINE_SURFACE(((1.,0.772543307031377,1.),(1.,0.773053168552098,
1.),(1.,0.773574707201177,1.),(1.,0.774108727913437,1.)))
REPRESENTATION_ITEM('')
SURFACE()
);
#145=(
BOUNDED_SURFACE()
B_SPLINE_SURFACE(3,2,((#28081,#28082,#28083),(#28084,#28085,#28086),(#28087,
#28088,#28089),(#28090,#28091,#28092)),.UNSPECIFIED.,.F.,.F.,.F.)
B_SPLINE_SURFACE_WITH_KNOTS((4,4),(3,3),(0.0326127356995135,0.0421285143028756),
(0.,1.),.UNSPECIFIED.)
GEOMETRIC_REPRESENTATION_ITEM()
RATIONAL_B_SPLINE_SURFACE(((1.,0.773368492107045,1.),(1.,0.770480922349017,
1.),(1.,0.767957745429662,1.),(1.,0.765689104422499,1.)))
REPRESENTATION_ITEM('')
SURFACE()
);
#146=(
BOUNDED_SURFACE()
B_SPLINE_SURFACE(3,2,((#28185,#28186,#28187),(#28188,#28189,#28190),(#28191,
#28192,#28193),(#28194,#28195,#28196),(#28197,#28198,#28199),(#28200,#28201,
#28202),(#28203,#28204,#28205),(#28206,#28207,#28208)),.UNSPECIFIED.,.F.,
 .F.,.F.)
B_SPLINE_SURFACE_WITH_KNOTS((4,2,2,4),(3,3),(0.000802853902804998,0.00108948501086235,
0.00137611611891971,0.00194937833503442),(0.,1.),.UNSPECIFIED.)
GEOMETRIC_REPRESENTATION_ITEM()
RATIONAL_B_SPLINE_SURFACE(((1.,0.923879532511286,1.),(1.,0.93126028758523,
1.),(1.,0.931596165488065,1.),(1.,0.918734528780506,1.),(1.,0.905994810924508,
1.),(1.,0.858462949893356,1.),(1.,0.814112175968461,1.),(1.,0.765689104422506,
1.)))
REPRESENTATION_ITEM('')
SURFACE()
);
#147=(
BOUNDED_SURFACE()
B_SPLINE_SURFACE(3,2,((#28242,#28243,#28244),(#28245,#28246,#28247),(#28248,
#28249,#28250),(#28251,#28252,#28253),(#28254,#28255,#28256),(#28257,#28258,
#28259)),.UNSPECIFIED.,.F.,.F.,.F.)
B_SPLINE_SURFACE_WITH_KNOTS((4,2,4),(3,3),(0.00125184933893988,0.00239738856741525,
0.00354292779589063),(0.,1.),.UNSPECIFIED.)
GEOMETRIC_REPRESENTATION_ITEM()
RATIONAL_B_SPLINE_SURFACE(((1.,0.707106781186548,1.),(1.,0.752499298133503,
1.),(1.,0.791707406457373,1.),(1.,0.86205547054867,1.),(1.,0.893085809396533,
1.),(1.,0.9210299078221,1.)))
REPRESENTATION_ITEM('')
SURFACE()
);
#148=(
BOUNDED_SURFACE()
B_SPLINE_SURFACE(3,2,((#28264,#28265,#28266),(#28267,#28268,#28269),(#28270,
#28271,#28272),(#28273,#28274,#28275)),.UNSPECIFIED.,.F.,.F.,.F.)
B_SPLINE_SURFACE_WITH_KNOTS((4,4),(3,3),(0.307250934553085,0.313798890571649),
(0.,1.),.UNSPECIFIED.)
GEOMETRIC_REPRESENTATION_ITEM()
RATIONAL_B_SPLINE_SURFACE(((1.,0.712804186852904,1.),(1.,0.71296450813891,
1.),(1.,0.71313821972869,1.),(1.,0.713329401304079,1.)))
REPRESENTATION_ITEM('')
SURFACE()
);
#149=(
BOUNDED_SURFACE()
B_SPLINE_SURFACE(3,2,((#28299,#28300,#28301),(#28302,#28303,#28304),(#28305,
#28306,#28307),(#28308,#28309,#28310),(#28311,#28312,#28313),(#28314,#28315,
#28316),(#28317,#28318,#28319),(#28320,#28321,#28322)),.UNSPECIFIED.,.F.,
 .F.,.F.)
B_SPLINE_SURFACE_WITH_KNOTS((4,2,2,4),(3,3),(0.0301024650456266,0.0387558943228362,
0.0430826089614409,0.0474093236000457),(0.,1.),.UNSPECIFIED.)
GEOMETRIC_REPRESENTATION_ITEM()
RATIONAL_B_SPLINE_SURFACE(((1.,0.921029907823249,1.),(1.,0.922877070064105,
1.),(1.,0.923876933766823,1.),(1.,0.92388082420723,1.),(1.,0.923630934244524,
1.),(1.,0.92266268253527,1.),(1.,0.921946472339213,1.),(1.,0.921029907823249,
1.)))
REPRESENTATION_ITEM('')
SURFACE()
);
#150=(
BOUNDED_SURFACE()
B_SPLINE_SURFACE(3,2,((#28335,#28336,#28337),(#28338,#28339,#28340),(#28341,
#28342,#28343),(#28344,#28345,#28346),(#28347,#28348,#28349),(#28350,#28351,
#28352)),.UNSPECIFIED.,.F.,.F.,.F.)
B_SPLINE_SURFACE_WITH_KNOTS((4,2,4),(3,3),(0.000625612417698575,0.00177266924615975,
0.00291972607462092),(0.,1.),.UNSPECIFIED.)
GEOMETRIC_REPRESENTATION_ITEM()
RATIONAL_B_SPLINE_SURFACE(((1.,0.921029907823245,1.),(1.,0.89303286027976,
1.),(1.,0.862014836405081,1.),(1.,0.791625319509651,1.),(1.,0.752373092952147,
1.),(1.,0.707106781186546,1.)))
REPRESENTATION_ITEM('')
SURFACE()
);
#151=(
BOUNDED_SURFACE()
B_SPLINE_SURFACE(3,2,((#28383,#28384,#28385),(#28386,#28387,#28388),(#28389,
#28390,#28391),(#28392,#28393,#28394)),.UNSPECIFIED.,.F.,.F.,.F.)
B_SPLINE_SURFACE_WITH_KNOTS((4,4),(3,3),(0.307250934553085,0.313798890571649),
(0.,1.),.UNSPECIFIED.)
GEOMETRIC_REPRESENTATION_ITEM()
RATIONAL_B_SPLINE_SURFACE(((1.,0.712804186852904,1.),(1.,0.712964508138907,
1.),(1.,0.713138219728696,1.),(1.,0.713329401304078,1.)))
REPRESENTATION_ITEM('')
SURFACE()
);
#152=(
BOUNDED_SURFACE()
B_SPLINE_SURFACE(3,2,((#28421,#28422,#28423),(#28424,#28425,#28426),(#28427,
#28428,#28429),(#28430,#28431,#28432),(#28433,#28434,#28435),(#28436,#28437,
#28438)),.UNSPECIFIED.,.F.,.F.,.F.)
B_SPLINE_SURFACE_WITH_KNOTS((4,2,4),(3,3),(0.000678304539097152,0.00122793525694894,
0.00177756597480073),(0.,1.),.UNSPECIFIED.)
GEOMETRIC_REPRESENTATION_ITEM()
RATIONAL_B_SPLINE_SURFACE(((1.,0.70710678118654,1.),(1.,0.746184084332961,
1.),(1.,0.782509959683157,1.),(1.,0.849214842808394,1.),(1.,0.879717238316117,
1.),(1.,0.907850513788111,1.)))
REPRESENTATION_ITEM('')
SURFACE()
);
#153=(
BOUNDED_SURFACE()
B_SPLINE_SURFACE(3,2,((#28448,#28449,#28450),(#28451,#28452,#28453),(#28454,
#28455,#28456),(#28457,#28458,#28459),(#28460,#28461,#28462),(#28463,#28464,
#28465)),.UNSPECIFIED.,.F.,.F.,.F.)
B_SPLINE_SURFACE_WITH_KNOTS((4,2,4),(3,3),(0.000625612417698574,0.00177266924615979,
0.002919726074621),(0.,1.),.UNSPECIFIED.)
GEOMETRIC_REPRESENTATION_ITEM()
RATIONAL_B_SPLINE_SURFACE(((1.,0.921029907823249,1.),(1.,0.893032860280521,
1.),(1.,0.862014836404084,1.),(1.,0.791625319510648,1.),(1.,0.7523730929514,
1.),(1.,0.707106781186553,1.)))
REPRESENTATION_ITEM('')
SURFACE()
);
#154=(
BOUNDED_SURFACE()
B_SPLINE_SURFACE(3,2,((#28474,#28475,#28476),(#28477,#28478,#28479),(#28480,
#28481,#28482),(#28483,#28484,#28485),(#28486,#28487,#28488),(#28489,#28490,
#28491),(#28492,#28493,#28494),(#28495,#28496,#28497),(#28498,#28499,#28500),
(#28501,#28502,#28503),(#28504,#28505,#28506),(#28507,#28508,#28509),(#28510,
#28511,#28512),(#28513,#28514,#28515),(#28516,#28517,#28518),(#28519,#28520,
#28521),(#28522,#28523,#28524),(#28525,#28526,#28527)),.UNSPECIFIED.,.F.,
 .F.,.F.)
B_SPLINE_SURFACE_WITH_KNOTS((4,2,2,2,2,2,2,2,4),(3,3),(0.0489197875214898,
0.0601853600247889,0.0657063758111463,0.068466883704325,0.0712273915975036,
0.0822694231702183,0.085029931063397,0.0877904389565757,0.093311454742933),
(0.,1.00022354093058),.UNSPECIFIED.)
GEOMETRIC_REPRESENTATION_ITEM()
RATIONAL_B_SPLINE_SURFACE(((1.,0.907555692141296,1.00004133017321),(1.,
0.912172103884354,1.00003926625926),(1.,0.91629725938563,1.00003742197706),
(1.,0.92068483810848,1.0000354603702),(1.,0.921842485532916,1.00003494280703),
(1.,0.92303257596533,1.00003441073919),(1.,0.923338391926672,1.00003427401442),
(1.,0.923751986701146,1.0000340891037),(1.,0.923857671595064,1.0000340418539),
(1.,0.923881080298134,1.00003403138829),(1.,0.922241806174626,1.00003476427802),
(1.,0.918599911621013,1.00003639250301),(1.,0.917794373423119,1.00003675264453),
(1.,0.916066405850502,1.00003752518749),(1.,0.91514227300216,1.00003793835052),
(1.,0.912223658689289,1.00003924321004),(1.,0.910083556365811,1.00004020001097),
(1.,0.907829914607839,1.00004120757332)))
REPRESENTATION_ITEM('')
SURFACE()
);
#155=(
BOUNDED_SURFACE()
B_SPLINE_SURFACE(3,2,((#28569,#28570,#28571),(#28572,#28573,#28574),(#28575,
#28576,#28577),(#28578,#28579,#28580),(#28581,#28582,#28583),(#28584,#28585,
#28586),(#28587,#28588,#28589),(#28590,#28591,#28592)),.UNSPECIFIED.,.F.,
 .F.,.F.)
B_SPLINE_SURFACE_WITH_KNOTS((4,2,2,4),(3,3),(0.0301024650456266,0.0387558943228361,
0.0430826089614409,0.0474093236000456),(0.,1.),.UNSPECIFIED.)
GEOMETRIC_REPRESENTATION_ITEM()
RATIONAL_B_SPLINE_SURFACE(((1.,0.921029907823249,1.),(1.,0.922877070064102,
1.),(1.,0.923876933766823,1.),(1.,0.92388082420723,1.),(1.,0.923630934244043,
1.),(1.,0.922662682535757,1.),(1.,0.921946472338846,1.),(1.,0.921029907823249,
1.)))
REPRESENTATION_ITEM('')
SURFACE()
);
#156=(
BOUNDED_SURFACE()
B_SPLINE_SURFACE(3,2,((#28598,#28599,#28600),(#28601,#28602,#28603),(#28604,
#28605,#28606),(#28607,#28608,#28609)),.UNSPECIFIED.,.F.,.F.,.F.)
B_SPLINE_SURFACE_WITH_KNOTS((4,4),(3,3),(0.307250934553084,0.313798890571649),
(0.,1.),.UNSPECIFIED.)
GEOMETRIC_REPRESENTATION_ITEM()
RATIONAL_B_SPLINE_SURFACE(((1.,0.712804186852904,1.),(1.,0.712964508138908,
1.),(1.,0.713138219728696,1.),(1.,0.713329401304078,1.)))
REPRESENTATION_ITEM('')
SURFACE()
);
#157=(
BOUNDED_SURFACE()
B_SPLINE_SURFACE(3,2,((#28616,#28617,#28618),(#28619,#28620,#28621),(#28622,
#28623,#28624),(#28625,#28626,#28627),(#28628,#28629,#28630),(#28631,#28632,
#28633)),.UNSPECIFIED.,.F.,.F.,.F.)
B_SPLINE_SURFACE_WITH_KNOTS((4,2,4),(3,3),(0.00086265399393263,0.00141381336854384,
0.00196497274315506),(0.,1.),.UNSPECIFIED.)
GEOMETRIC_REPRESENTATION_ITEM()
RATIONAL_B_SPLINE_SURFACE(((1.,0.707106781186548,1.),(1.,0.746708654901981,
1.),(1.,0.782505247018089,1.),(1.,0.84894802268141,1.),(1.,0.87977370861613,
1.),(1.,0.90785051378974,1.)))
REPRESENTATION_ITEM('')
SURFACE()
);
#158=(
BOUNDED_SURFACE()
B_SPLINE_SURFACE(3,2,((#28637,#28638,#28639),(#28640,#28641,#28642),(#28643,
#28644,#28645),(#28646,#28647,#28648),(#28649,#28650,#28651),(#28652,#28653,
#28654)),.UNSPECIFIED.,.F.,.F.,.F.)
B_SPLINE_SURFACE_WITH_KNOTS((4,2,4),(3,3),(0.00125184933893988,0.00239738856741524,
0.00354292779589061),(0.,1.),.UNSPECIFIED.)
GEOMETRIC_REPRESENTATION_ITEM()
RATIONAL_B_SPLINE_SURFACE(((1.,0.707106781186555,1.),(1.,0.752499298132554,
1.),(1.,0.791707406458655,1.),(1.,0.862055470547405,1.),(1.,0.893085809397482,
1.),(1.,0.921029907822106,1.)))
REPRESENTATION_ITEM('')
SURFACE()
);
#159=(
BOUNDED_SURFACE()
B_SPLINE_SURFACE(3,2,((#28656,#28657,#28658),(#28659,#28660,#28661),(#28662,
#28663,#28664),(#28665,#28666,#28667),(#28668,#28669,#28670),(#28671,#28672,
#28673)),.UNSPECIFIED.,.F.,.F.,.F.)
B_SPLINE_SURFACE_WITH_KNOTS((4,2,4),(3,3),(0.00125184933893988,0.00239738856741526,
0.00354292779589064),(0.,1.),.UNSPECIFIED.)
GEOMETRIC_REPRESENTATION_ITEM()
RATIONAL_B_SPLINE_SURFACE(((1.,0.707106781186548,1.),(1.,0.752499298132371,
1.),(1.,0.791707406458881,1.),(1.,0.862055470547165,1.),(1.,0.893085809397659,
1.),(1.,0.9210299078221,1.)))
REPRESENTATION_ITEM('')
SURFACE()
);
#160=(
BOUNDED_SURFACE()
B_SPLINE_SURFACE(3,2,((#28721,#28722,#28723),(#28724,#28725,#28726),(#28727,
#28728,#28729),(#28730,#28731,#28732),(#28733,#28734,#28735),(#28736,#28737,
#28738)),.UNSPECIFIED.,.F.,.F.,.F.)
B_SPLINE_SURFACE_WITH_KNOTS((4,2,4),(3,3),(0.0491065561917184,0.0576730069527121,
0.0662394577137058),(0.,1.),.UNSPECIFIED.)
GEOMETRIC_REPRESENTATION_ITEM()
RATIONAL_B_SPLINE_SURFACE(((1.,0.921029907823248,1.),(1.,0.922875643094769,
1.),(1.,0.923881929396489,1.),(1.,0.923877126948933,1.),(1.,0.922867245922119,
1.),(1.,0.921029907823249,1.)))
REPRESENTATION_ITEM('')
SURFACE()
);
#161=(
BOUNDED_SURFACE()
B_SPLINE_SURFACE(3,2,((#28750,#28751,#28752),(#28753,#28754,#28755),(#28756,
#28757,#28758),(#28759,#28760,#28761),(#28762,#28763,#28764),(#28765,#28766,
#28767)),.UNSPECIFIED.,.F.,.F.,.F.)
B_SPLINE_SURFACE_WITH_KNOTS((4,2,4),(3,3),(0.000862653993932642,0.00141381336854385,
0.00196497274315505),(0.,1.),.UNSPECIFIED.)
GEOMETRIC_REPRESENTATION_ITEM()
RATIONAL_B_SPLINE_SURFACE(((1.,0.70710678118654,1.),(1.,0.746708654901505,
1.),(1.,0.782505247018736,1.),(1.,0.84894802268075,1.),(1.,0.879773708616637,
1.),(1.,0.907850513789743,1.)))
REPRESENTATION_ITEM('')
SURFACE()
);
#162=(
BOUNDED_SURFACE()
B_SPLINE_SURFACE(3,2,((#28777,#28778,#28779),(#28780,#28781,#28782),(#28783,
#28784,#28785),(#28786,#28787,#28788),(#28789,#28790,#28791),(#28792,#28793,
#28794)),.UNSPECIFIED.,.F.,.F.,.F.)
B_SPLINE_SURFACE_WITH_KNOTS((4,2,4),(3,3),(0.000625612417698576,0.00177266924615977,
0.00291972607462096),(0.,1.),.UNSPECIFIED.)
GEOMETRIC_REPRESENTATION_ITEM()
RATIONAL_B_SPLINE_SURFACE(((1.,0.92102990782325,1.),(1.,0.893032860280475,
1.),(1.,0.862014836404147,1.),(1.,0.791625319510585,1.),(1.,0.752373092951458,
1.),(1.,0.707106781186553,1.)))
REPRESENTATION_ITEM('')
SURFACE()
);
#163=(
BOUNDED_SURFACE()
B_SPLINE_SURFACE(3,2,((#28818,#28819,#28820),(#28821,#28822,#28823),(#28824,
#28825,#28826),(#28827,#28828,#28829),(#28830,#28831,#28832),(#28833,#28834,
#28835),(#28836,#28837,#28838),(#28839,#28840,#28841),(#28842,#28843,#28844),
(#28845,#28846,#28847),(#28848,#28849,#28850),(#28851,#28852,#28853),(#28854,
#28855,#28856),(#28857,#28858,#28859),(#28860,#28861,#28862),(#28863,#28864,
#28865),(#28866,#28867,#28868),(#28869,#28870,#28871)),.UNSPECIFIED.,.F.,
 .F.,.F.)
B_SPLINE_SURFACE_WITH_KNOTS((4,2,2,2,2,2,2,2,4),(3,3),(0.0489197875016647,
0.060185360024789,0.0657063758111463,0.068466883704325,0.0712273915975037,
0.0822694231702183,0.085029931063397,0.0877904389565757,0.0933114547429331),
(0.,1.00022354095041),.UNSPECIFIED.)
GEOMETRIC_REPRESENTATION_ITEM()
RATIONAL_B_SPLINE_SURFACE(((1.,0.907555692115104,1.00004133017689),(1.,
0.912172103867759,1.00003926626275),(1.,0.916297259379205,1.00003742198038),
(1.,0.920684838106704,1.00003546037334),(1.,0.921842485531367,1.00003494281013),
(1.,0.923032575963804,1.00003441074224),(1.,0.923338391925153,1.00003427401746),
(1.,0.923751986699634,1.00003408910672),(1.,0.923857671593554,1.00003404185692),
(1.,0.923881080296625,1.00003403139131),(1.,0.922241806173293,1.0000347642811),
(1.,0.918599911619347,1.00003639250624),(1.,0.917794373421593,1.00003675264779),
(1.,0.916066405848735,1.00003752519082),(1.,0.915142273000684,1.00003793835389),
(1.,0.912223658687137,1.00003924321352),(1.,0.910083556364339,1.00004020001454),
(1.,0.907829914606016,1.00004120757698)))
REPRESENTATION_ITEM('')
SURFACE()
);
#164=(
BOUNDED_SURFACE()
B_SPLINE_SURFACE(3,2,((#28898,#28899,#28900),(#28901,#28902,#28903),(#28904,
#28905,#28906),(#28907,#28908,#28909)),.UNSPECIFIED.,.F.,.F.,.F.)
B_SPLINE_SURFACE_WITH_KNOTS((4,4),(3,3),(0.306318309032005,0.312866265050619),
(0.,1.),.UNSPECIFIED.)
GEOMETRIC_REPRESENTATION_ITEM()
RATIONAL_B_SPLINE_SURFACE(((1.,0.712804186852904,1.),(1.,0.712964508138909,
1.),(1.,0.713138219728695,1.),(1.,0.713329401304078,1.)))
REPRESENTATION_ITEM('')
SURFACE()
);
#165=(
BOUNDED_SURFACE()
B_SPLINE_SURFACE(3,2,((#28925,#28926,#28927),(#28928,#28929,#28930),(#28931,
#28932,#28933),(#28934,#28935,#28936)),.UNSPECIFIED.,.F.,.F.,.F.)
B_SPLINE_SURFACE_WITH_KNOTS((4,4),(3,3),(0.307250934553084,0.313798890571649),
(0.,1.),.UNSPECIFIED.)
GEOMETRIC_REPRESENTATION_ITEM()
RATIONAL_B_SPLINE_SURFACE(((1.,0.712804186852904,1.),(1.,0.712964508138909,
1.),(1.,0.713138219728695,1.),(1.,0.713329401304078,1.)))
REPRESENTATION_ITEM('')
SURFACE()
);
#166=(
BOUNDED_SURFACE()
B_SPLINE_SURFACE(3,2,((#28962,#28963,#28964),(#28965,#28966,#28967),(#28968,
#28969,#28970),(#28971,#28972,#28973),(#28974,#28975,#28976),(#28977,#28978,
#28979)),.UNSPECIFIED.,.F.,.F.,.F.)
B_SPLINE_SURFACE_WITH_KNOTS((4,2,4),(3,3),(0.00067830453909708,0.00122793525694887,
0.00177756597480066),(0.,1.),.UNSPECIFIED.)
GEOMETRIC_REPRESENTATION_ITEM()
RATIONAL_B_SPLINE_SURFACE(((1.,0.70710678118654,1.),(1.,0.74618408433299,
1.),(1.,0.78250995968311,1.),(1.,0.849214842808429,1.),(1.,0.879717238316075,
1.),(1.,0.907850513788108,1.)))
REPRESENTATION_ITEM('')
SURFACE()
);
#167=(
BOUNDED_SURFACE()
B_SPLINE_SURFACE(3,2,((#28981,#28982,#28983),(#28984,#28985,#28986),(#28987,
#28988,#28989),(#28990,#28991,#28992),(#28993,#28994,#28995),(#28996,#28997,
#28998)),.UNSPECIFIED.,.F.,.F.,.F.)
B_SPLINE_SURFACE_WITH_KNOTS((4,2,4),(3,3),(0.000678304539097056,0.00122793525694883,
0.0017775659748006),(0.,1.),.UNSPECIFIED.)
GEOMETRIC_REPRESENTATION_ITEM()
RATIONAL_B_SPLINE_SURFACE(((1.,0.707106781186548,1.),(1.,0.746184084332992,
1.),(1.,0.782509959683127,1.),(1.,0.849214842808424,1.),(1.,0.8797172383161,
1.),(1.,0.90785051378811,1.)))
REPRESENTATION_ITEM('')
SURFACE()
);
#168=(
BOUNDED_SURFACE()
B_SPLINE_SURFACE(3,2,((#29008,#29009,#29010),(#29011,#29012,#29013),(#29014,
#29015,#29016),(#29017,#29018,#29019),(#29020,#29021,#29022),(#29023,#29024,
#29025)),.UNSPECIFIED.,.F.,.F.,.F.)
B_SPLINE_SURFACE_WITH_KNOTS((4,2,4),(3,3),(0.000625612417698575,0.00177266924615975,
0.00291972607462092),(0.,1.),.UNSPECIFIED.)
GEOMETRIC_REPRESENTATION_ITEM()
RATIONAL_B_SPLINE_SURFACE(((1.,0.921029907823245,1.),(1.,0.89303286027976,
1.),(1.,0.862014836405081,1.),(1.,0.791625319509651,1.),(1.,0.752373092952147,
1.),(1.,0.707106781186546,1.)))
REPRESENTATION_ITEM('')
SURFACE()
);
#169=(
BOUNDED_SURFACE()
B_SPLINE_SURFACE(3,2,((#29047,#29048,#29049),(#29050,#29051,#29052),(#29053,
#29054,#29055),(#29056,#29057,#29058),(#29059,#29060,#29061),(#29062,#29063,
#29064),(#29065,#29066,#29067),(#29068,#29069,#29070),(#29071,#29072,#29073),
(#29074,#29075,#29076),(#29077,#29078,#29079),(#29080,#29081,#29082),(#29083,
#29084,#29085),(#29086,#29087,#29088),(#29089,#29090,#29091),(#29092,#29093,
#29094),(#29095,#29096,#29097),(#29098,#29099,#29100),(#29101,#29102,#29103),
(#29104,#29105,#29106)),.UNSPECIFIED.,.F.,.F.,.F.)
B_SPLINE_SURFACE_WITH_KNOTS((4,2,2,2,2,2,2,2,2,4),(3,3),(0.0165870372170484,
0.0222388347236946,0.0250006537634149,0.0277624728031351,0.0388097489620161,
0.0415715680017363,0.0443333870414566,0.049857025120897,0.0553806632003375,
0.0610324607069837),(-0.000128159427205692,1.),.UNSPECIFIED.)
GEOMETRIC_REPRESENTATION_ITEM()
RATIONAL_B_SPLINE_SURFACE(((1.00002366285482,0.907681957774734,1.),(1.00002307158425,
0.909988735295067,1.),(1.00002250978471,0.912180534803509,1.),(1.0000217503978,
0.915143199855024,1.),(1.00002151350586,0.916067407863037,1.),(1.00002107037521,
0.917796233671169,1.),(1.00002086466642,0.918598784051383,1.),(1.00001993577826,
0.922222739703994,1.),(1.00001951311599,0.923871710355246,1.),(1.00001951373601,
0.923869291421499,1.),(1.00001953985541,0.923767389414861,1.),(1.00001964298269,
0.923365049627104,1.),(1.00001971973799,0.923065597204644,1.),(1.00002002011192,
0.921893721121883,1.),(1.0000203140672,0.920746886721891,1.),(1.0000210516324,
0.917869356720474,1.),(1.00002149497007,0.916139723229799,1.),(1.00002250053566,
0.912216618982122,1.),(1.00002306616987,0.910009858911181,1.),(1.00002366324673,
0.907680428794268,1.)))
REPRESENTATION_ITEM('')
SURFACE()
);
#170=(
BOUNDED_SURFACE()
B_SPLINE_SURFACE(3,2,((#29115,#29116,#29117),(#29118,#29119,#29120),(#29121,
#29122,#29123),(#29124,#29125,#29126),(#29127,#29128,#29129),(#29130,#29131,
#29132),(#29133,#29134,#29135),(#29136,#29137,#29138)),.UNSPECIFIED.,.F.,
 .F.,.F.)
B_SPLINE_SURFACE_WITH_KNOTS((4,2,2,4),(3,3),(0.0301024650456266,0.0387558943228362,
0.0430826089614409,0.0474093236000457),(0.,1.),.UNSPECIFIED.)
GEOMETRIC_REPRESENTATION_ITEM()
RATIONAL_B_SPLINE_SURFACE(((1.,0.921029907823249,1.),(1.,0.922877070064105,
1.),(1.,0.923876933766823,1.),(1.,0.92388082420723,1.),(1.,0.923630934244524,
1.),(1.,0.92266268253527,1.),(1.,0.921946472339213,1.),(1.,0.921029907823249,
1.)))
REPRESENTATION_ITEM('')
SURFACE()
);
#171=(
BOUNDED_SURFACE()
B_SPLINE_SURFACE(3,2,((#29148,#29149,#29150),(#29151,#29152,#29153),(#29154,
#29155,#29156),(#29157,#29158,#29159),(#29160,#29161,#29162),(#29163,#29164,
#29165)),.UNSPECIFIED.,.F.,.F.,.F.)
B_SPLINE_SURFACE_WITH_KNOTS((4,2,4),(3,3),(0.000862653993932655,0.00141381336854386,
0.00196497274315507),(0.,1.),.UNSPECIFIED.)
GEOMETRIC_REPRESENTATION_ITEM()
RATIONAL_B_SPLINE_SURFACE(((1.,0.707106781186548,1.),(1.,0.746708654901537,
1.),(1.,0.782505247018702,1.),(1.,0.848948022680798,1.),(1.,0.879773708616591,
1.),(1.,0.907850513789744,1.)))
REPRESENTATION_ITEM('')
SURFACE()
);
#172=(
BOUNDED_SURFACE()
B_SPLINE_SURFACE(3,2,((#29188,#29189,#29190),(#29191,#29192,#29193),(#29194,
#29195,#29196),(#29197,#29198,#29199),(#29200,#29201,#29202),(#29203,#29204,
#29205)),.UNSPECIFIED.,.F.,.F.,.F.)
B_SPLINE_SURFACE_WITH_KNOTS((4,2,4),(3,3),(0.00125184933893988,0.00239738856741524,
0.00354292779589061),(0.,1.),.UNSPECIFIED.)
GEOMETRIC_REPRESENTATION_ITEM()
RATIONAL_B_SPLINE_SURFACE(((1.,0.707106781186555,1.),(1.,0.752499298132528,
1.),(1.,0.791707406458668,1.),(1.,0.862055470547376,1.),(1.,0.893085809397505,
1.),(1.,0.9210299078221,1.)))
REPRESENTATION_ITEM('')
SURFACE()
);
#173=(
BOUNDED_SURFACE()
B_SPLINE_SURFACE(3,2,((#29229,#29230,#29231),(#29232,#29233,#29234),(#29235,
#29236,#29237),(#29238,#29239,#29240)),.UNSPECIFIED.,.F.,.F.,.F.)
B_SPLINE_SURFACE_WITH_KNOTS((4,4),(3,3),(0.306318309032005,0.312866265050619),
(0.,1.),.UNSPECIFIED.)
GEOMETRIC_REPRESENTATION_ITEM()
RATIONAL_B_SPLINE_SURFACE(((1.,0.71280418685291,1.),(1.,0.712964508138911,
1.),(1.,0.713138219728701,1.),(1.,0.713329401304078,1.)))
REPRESENTATION_ITEM('')
SURFACE()
);
#174=(
BOUNDED_SURFACE()
B_SPLINE_SURFACE(3,2,((#29271,#29272,#29273),(#29274,#29275,#29276),(#29277,
#29278,#29279),(#29280,#29281,#29282),(#29283,#29284,#29285),(#29286,#29287,
#29288)),.UNSPECIFIED.,.F.,.F.,.F.)
B_SPLINE_SURFACE_WITH_KNOTS((4,2,4),(3,3),(0.00086265399393263,0.00141381336854384,
0.00196497274315506),(0.,1.),.UNSPECIFIED.)
GEOMETRIC_REPRESENTATION_ITEM()
RATIONAL_B_SPLINE_SURFACE(((1.,0.707106781186548,1.),(1.,0.746708654901981,
1.),(1.,0.782505247018089,1.),(1.,0.84894802268141,1.),(1.,0.87977370861613,
1.),(1.,0.907850513789739,1.)))
REPRESENTATION_ITEM('')
SURFACE()
);
#175=(
BOUNDED_SURFACE()
B_SPLINE_SURFACE(3,2,((#29300,#29301,#29302),(#29303,#29304,#29305),(#29306,
#29307,#29308),(#29309,#29310,#29311),(#29312,#29313,#29314),(#29315,#29316,
#29317),(#29318,#29319,#29320),(#29321,#29322,#29323),(#29324,#29325,#29326),
(#29327,#29328,#29329),(#29330,#29331,#29332),(#29333,#29334,#29335),(#29336,
#29337,#29338),(#29339,#29340,#29341),(#29342,#29343,#29344),(#29345,#29346,
#29347),(#29348,#29349,#29350),(#29351,#29352,#29353)),.UNSPECIFIED.,.F.,
 .F.,.F.)
B_SPLINE_SURFACE_WITH_KNOTS((4,2,2,2,2,2,2,2,4),(3,3),(0.0489197875179387,
0.0601853600247889,0.0657063758111463,0.068466883704325,0.0712273915975036,
0.0822694231702183,0.085029931063397,0.0877904389565757,0.093311454742933),
(0.,1.00022354093414),.UNSPECIFIED.)
GEOMETRIC_REPRESENTATION_ITEM()
RATIONAL_B_SPLINE_SURFACE(((1.,0.907555692136622,1.00004133017387),(1.,
0.912172103881105,1.00003926625988),(1.,0.916297259384821,1.00003742197765),
(1.,0.920684838107995,1.00003546037076),(1.,0.921842485532638,1.00003494280759),
(1.,0.923032575965056,1.00003441073973),(1.,0.9233383919264,1.00003427401496),
(1.,0.923751986700875,1.00003408910424),(1.,0.923857671594793,1.00003404185444),
(1.,0.923881080297864,1.00003403138883),(1.,0.922241806174143,1.00003476427857),
(1.,0.918599911620776,1.00003639250359),(1.,0.917794373422827,1.00003675264511),
(1.,0.916066405850204,1.00003752518808),(1.,0.915142273001859,1.00003793835112),
(1.,0.912223658688977,1.00003924321066),(1.,0.910083556365492,1.00004020001161),
(1.,0.907829914607512,1.00004120757398)))
REPRESENTATION_ITEM('')
SURFACE()
);
#176=(
BOUNDED_SURFACE()
B_SPLINE_SURFACE(3,2,((#29363,#29364,#29365),(#29366,#29367,#29368),(#29369,
#29370,#29371),(#29372,#29373,#29374)),.UNSPECIFIED.,.F.,.F.,.F.)
B_SPLINE_SURFACE_WITH_KNOTS((4,4),(3,3),(0.307250934553086,0.31379889057165),
(0.,1.),.UNSPECIFIED.)
GEOMETRIC_REPRESENTATION_ITEM()
RATIONAL_B_SPLINE_SURFACE(((1.,0.712804186852904,1.),(1.,0.712964508138908,
1.),(1.,0.713138219728696,1.),(1.,0.713329401304078,1.)))
REPRESENTATION_ITEM('')
SURFACE()
);
#177=(
BOUNDED_SURFACE()
B_SPLINE_SURFACE(3,2,((#29376,#29377,#29378),(#29379,#29380,#29381),(#29382,
#29383,#29384),(#29385,#29386,#29387),(#29388,#29389,#29390),(#29391,#29392,
#29393)),.UNSPECIFIED.,.F.,.F.,.F.)
B_SPLINE_SURFACE_WITH_KNOTS((4,2,4),(3,3),(0.000678304539097038,0.00122793525694883,
0.00177756597480063),(0.,1.),.UNSPECIFIED.)
GEOMETRIC_REPRESENTATION_ITEM()
RATIONAL_B_SPLINE_SURFACE(((1.,0.70710678118654,1.),(1.,0.746184084332961,
1.),(1.,0.782509959683157,1.),(1.,0.849214842808395,1.),(1.,0.879717238316122,
1.),(1.,0.907850513788111,1.)))
REPRESENTATION_ITEM('')
SURFACE()
);
#178=(
BOUNDED_SURFACE()
B_SPLINE_SURFACE(3,2,((#29431,#29432,#29433),(#29434,#29435,#29436),(#29437,
#29438,#29439),(#29440,#29441,#29442)),.UNSPECIFIED.,.F.,.F.,.F.)
B_SPLINE_SURFACE_WITH_KNOTS((4,4),(3,3),(0.307250934553086,0.31379889057165),
(0.,1.),.UNSPECIFIED.)
GEOMETRIC_REPRESENTATION_ITEM()
RATIONAL_B_SPLINE_SURFACE(((1.,0.712804186852903,1.),(1.,0.712964508138911,
1.),(1.,0.713138219728697,1.),(1.,0.713329401304077,1.)))
REPRESENTATION_ITEM('')
SURFACE()
);
#179=(
BOUNDED_SURFACE()
B_SPLINE_SURFACE(3,2,((#31143,#31144,#31145),(#31146,#31147,#31148),(#31149,
#31150,#31151),(#31152,#31153,#31154),(#31155,#31156,#31157),(#31158,#31159,
#31160)),.UNSPECIFIED.,.F.,.F.,.F.)
B_SPLINE_SURFACE_WITH_KNOTS((4,2,4),(3,3),(0.00106076019035493,0.00169847101257237,
0.00233618183478981),(0.,1.),.UNSPECIFIED.)
GEOMETRIC_REPRESENTATION_ITEM()
RATIONAL_B_SPLINE_SURFACE(((1.,0.707106781186634,1.),(1.,0.749398144477624,
1.),(1.,0.787950893928372,1.),(1.,0.859993702049886,1.),(1.,0.893886360722003,
1.),(1.,0.923879532510764,1.)))
REPRESENTATION_ITEM('')
SURFACE()
);
#180=(
BOUNDED_SURFACE()
B_SPLINE_SURFACE(3,2,((#31184,#31185,#31186),(#31187,#31188,#31189),(#31190,
#31191,#31192),(#31193,#31194,#31195),(#31196,#31197,#31198),(#31199,#31200,
#31201)),.UNSPECIFIED.,.F.,.F.,.F.)
B_SPLINE_SURFACE_WITH_KNOTS((4,2,4),(3,3),(0.000793141102904165,0.00155796281789264,
0.00232278453288111),(-0.000567486199232424,1.),.UNSPECIFIED.)
GEOMETRIC_REPRESENTATION_ITEM()
RATIONAL_B_SPLINE_SURFACE(((1.0003619027993,0.681135153781566,1.),(1.0003023133926,
0.733638110485494,1.),(1.00024889602588,0.780703014258753,1.),(1.00015092061996,
0.867027057078915,1.),(1.00010588522079,0.906706787818273,1.),(1.00006613376639,
0.941730947393786,1.)))
REPRESENTATION_ITEM('')
SURFACE()
);
#181=(
BOUNDED_SURFACE()
B_SPLINE_SURFACE(3,2,((#31225,#31226,#31227),(#31228,#31229,#31230),(#31231,
#31232,#31233),(#31234,#31235,#31236),(#31237,#31238,#31239),(#31240,#31241,
#31242),(#31243,#31244,#31245),(#31246,#31247,#31248)),.UNSPECIFIED.,.F.,
 .F.,.F.)
B_SPLINE_SURFACE_WITH_KNOTS((4,2,2,4),(3,3),(0.0113699589602356,0.0215499319036472,
0.0263330282216041,0.031727010144494),(0.,1.00072721389233),
 .UNSPECIFIED.)
GEOMETRIC_REPRESENTATION_ITEM()
RATIONAL_B_SPLINE_SURFACE(((0.999999999999999,0.904674950757355,1.00013864340019),
(1.,0.909119912835753,1.00013217852384),(1.,0.913289332689208,1.00012611440376),
(1.,0.918180475671682,1.00011900058951),(1.,0.91955733112885,1.00011699805268),
(1.,0.92190730676968,1.00011358018281),(1.,0.922815134510754,1.00011225981292),
(1.,0.923326705446227,1.00011151576994)))
REPRESENTATION_ITEM('')
SURFACE()
);
#182=(
BOUNDED_SURFACE()
B_SPLINE_SURFACE(3,2,((#31249,#31250,#31251),(#31252,#31253,#31254),(#31255,
#31256,#31257),(#31258,#31259,#31260),(#31261,#31262,#31263),(#31264,#31265,
#31266),(#31267,#31268,#31269),(#31270,#31271,#31272)),.UNSPECIFIED.,.F.,
 .F.,.F.)
B_SPLINE_SURFACE_WITH_KNOTS((4,2,2,4),(3,3),(0.0119004725603816,0.0216177878121986,
0.0264008481563397,0.0313322083477393),(-0.000264627279374309,1.),
 .UNSPECIFIED.)
GEOMETRIC_REPRESENTATION_ITEM()
RATIONAL_B_SPLINE_SURFACE(((1.00005010827284,0.90532292634548,1.),(1.00004787696662,
0.909538867776431,1.),(1.0000457907739,0.913480624500144,1.),(1.0000432831544,
0.918218646038307,1.),(1.00004255484361,0.919594752826323,1.),(1.00004136830048,
0.921836666698683,1.),(1.00004091524432,0.922692693631796,1.),(1.0000406351647,
0.923221890052849,1.)))
REPRESENTATION_ITEM('')
SURFACE()
);
#183=(
BOUNDED_SURFACE()
B_SPLINE_SURFACE(3,2,((#31405,#31406,#31407),(#31408,#31409,#31410),(#31411,
#31412,#31413),(#31414,#31415,#31416),(#31417,#31418,#31419),(#31420,#31421,
#31422)),.UNSPECIFIED.,.F.,.F.,.F.)
B_SPLINE_SURFACE_WITH_KNOTS((4,2,4),(3,3),(0.000848991610552184,0.00148839833350338,
0.00212780505645457),(0.,1.),.UNSPECIFIED.)
GEOMETRIC_REPRESENTATION_ITEM()
RATIONAL_B_SPLINE_SURFACE(((1.,0.707106781186638,1.),(1.,0.749413725208667,
1.),(1.,0.788293333703998,1.),(1.,0.860148103423894,1.),(1.,0.893310888592562,
1.),(1.,0.923879532511264,1.)))
REPRESENTATION_ITEM('')
SURFACE()
);
#184=(
BOUNDED_SURFACE()
B_SPLINE_SURFACE(3,2,((#31448,#31449,#31450),(#31451,#31452,#31453),(#31454,
#31455,#31456),(#31457,#31458,#31459),(#31460,#31461,#31462),(#31463,#31464,
#31465)),.UNSPECIFIED.,.F.,.F.,.F.)
B_SPLINE_SURFACE_WITH_KNOTS((4,2,4),(3,3),(0.00106076019035492,0.00169895425208248,
0.00233714831381003),(0.,1.),.UNSPECIFIED.)
GEOMETRIC_REPRESENTATION_ITEM()
RATIONAL_B_SPLINE_SURFACE(((1.,0.707106781186618,1.),(1.,0.749428557966193,
1.),(1.,0.787940856472646,1.),(1.,0.859781915358774,1.),(1.,0.893307888347381,
1.),(1.,0.923879532511264,1.)))
REPRESENTATION_ITEM('')
SURFACE()
);
#185=(
BOUNDED_SURFACE()
B_SPLINE_SURFACE(3,2,((#31489,#31490,#31491),(#31492,#31493,#31494),(#31495,
#31496,#31497),(#31498,#31499,#31500),(#31501,#31502,#31503),(#31504,#31505,
#31506)),.UNSPECIFIED.,.F.,.F.,.F.)
B_SPLINE_SURFACE_WITH_KNOTS((4,2,4),(3,3),(0.00106076019035499,0.00169856943267974,
0.00233637867500449),(0.,1.),.UNSPECIFIED.)
GEOMETRIC_REPRESENTATION_ITEM()
RATIONAL_B_SPLINE_SURFACE(((1.,0.707106781186626,1.),(1.,0.749404516349508,
1.),(1.,0.787956723757177,1.),(1.,0.859986866015709,1.),(1.,0.893873946401784,
1.),(1.,0.923879532510069,1.)))
REPRESENTATION_ITEM('')
SURFACE()
);
#186=(
BOUNDED_SURFACE()
B_SPLINE_SURFACE(3,2,((#31530,#31531,#31532),(#31533,#31534,#31535),(#31536,
#31537,#31538),(#31539,#31540,#31541),(#31542,#31543,#31544),(#31545,#31546,
#31547),(#31548,#31549,#31550),(#31551,#31552,#31553)),.UNSPECIFIED.,.F.,
 .F.,.F.)
B_SPLINE_SURFACE_WITH_KNOTS((4,2,2,4),(3,3),(0.0119004725412382,0.0216177878121984,
0.0264008481563395,0.0313322083668821),(-0.000264627298517322,1.),
 .UNSPECIFIED.)
GEOMETRIC_REPRESENTATION_ITEM()
RATIONAL_B_SPLINE_SURFACE(((1.00005010827648,0.905322926318752,1.),(1.00004787697009,
0.90953886775917,1.),(1.00004579077722,0.913480624492233,1.),(1.00004328315754,
0.918218646036742,1.),(1.00004255484669,0.919594752824784,1.),(1.00004136830347,
0.921836666701605,1.),(1.00004091524728,0.922692693636962,1.),(1.00004063516764,
0.923221890057542,1.)))
REPRESENTATION_ITEM('')
SURFACE()
);
#187=(
BOUNDED_SURFACE()
B_SPLINE_SURFACE(3,2,((#31556,#31557,#31558),(#31559,#31560,#31561),(#31562,
#31563,#31564),(#31565,#31566,#31567),(#31568,#31569,#31570),(#31571,#31572,
#31573),(#31574,#31575,#31576),(#31577,#31578,#31579)),.UNSPECIFIED.,.F.,
 .F.,.F.)
B_SPLINE_SURFACE_WITH_KNOTS((4,2,2,4),(3,3),(0.0113699590143702,0.0215499319036474,
0.0263330282216043,0.0317270100903599),(0.,1.0007272138382),
 .UNSPECIFIED.)
GEOMETRIC_REPRESENTATION_ITEM()
RATIONAL_B_SPLINE_SURFACE(((1.,0.904674950833136,1.00013864338976),(1.,
0.9091199128866,1.00013217851393),(1.,0.913289332709887,1.00012611439435),
(1.,0.918180475676915,1.00011900058065),(1.,0.91955733113338,1.00011699804396),
(1.,0.921907306761203,1.00011358017437),(1.,0.922815134496923,1.00011225980459),
(1.,0.923326705434899,1.00011151576166)))
REPRESENTATION_ITEM('')
SURFACE()
);
#188=(
BOUNDED_SURFACE()
B_SPLINE_SURFACE(3,2,((#31580,#31581,#31582),(#31583,#31584,#31585),(#31586,
#31587,#31588),(#31589,#31590,#31591),(#31592,#31593,#31594),(#31595,#31596,
#31597),(#31598,#31599,#31600),(#31601,#31602,#31603)),.UNSPECIFIED.,.F.,
 .F.,.F.)
B_SPLINE_SURFACE_WITH_KNOTS((4,2,2,4),(3,3),(0.0119004725305903,0.0216177878121981,
0.0264008481563393,0.0313322083775296),(-0.000264627309164933,1.),
 .UNSPECIFIED.)
GEOMETRIC_REPRESENTATION_ITEM()
RATIONAL_B_SPLINE_SURFACE(((1.0000501082785,0.905322926303854,1.),(1.00004787697202,
0.909538867750149,1.),(1.00004579077906,0.913480624487108,1.),(1.00004328315928,
0.918218646036229,1.),(1.00004255484841,0.919594752823839,1.),(1.00004136830513,
0.921836666703322,1.),(1.00004091524892,0.922692693639759,1.),(1.00004063516927,
0.92322189006016,1.)))
REPRESENTATION_ITEM('')
SURFACE()
);
#189=(
BOUNDED_SURFACE()
B_SPLINE_SURFACE(3,2,((#31614,#31615,#31616),(#31617,#31618,#31619),(#31620,
#31621,#31622),(#31623,#31624,#31625),(#31626,#31627,#31628),(#31629,#31630,
#31631),(#31632,#31633,#31634),(#31635,#31636,#31637)),.UNSPECIFIED.,.F.,
 .F.,.F.)
B_SPLINE_SURFACE_WITH_KNOTS((4,2,2,4),(3,3),(0.0113699590001087,0.0215499319036469,
0.0263330282216038,0.0317270101046203),(0.,1.00072721385246),
 .UNSPECIFIED.)
GEOMETRIC_REPRESENTATION_ITEM()
RATIONAL_B_SPLINE_SURFACE(((1.,0.904674950813353,1.00013864339251),(1.,
0.909119912872212,1.00013217851654),(1.,0.913289332705507,1.00012611439682),
(1.,0.918180475675032,1.00011900058298),(1.,0.919557331132055,1.00011699804626),
(1.,0.921907306763585,1.00011358017659),(1.,0.922815134500407,1.00011225980678),
(1.,0.923326705437937,1.00011151576384)))
REPRESENTATION_ITEM('')
SURFACE()
);
#190=(
BOUNDED_SURFACE()
B_SPLINE_SURFACE(3,2,((#31840,#31841,#31842),(#31843,#31844,#31845),(#31846,
#31847,#31848),(#31849,#31850,#31851),(#31852,#31853,#31854),(#31855,#31856,
#31857)),.UNSPECIFIED.,.F.,.F.,.F.)
B_SPLINE_SURFACE_WITH_KNOTS((4,2,4),(3,3),(0.000793141102904163,0.00155796281789264,
0.00232278453288111),(-0.000567486199155168,1.),.UNSPECIFIED.)
GEOMETRIC_REPRESENTATION_ITEM()
RATIONAL_B_SPLINE_SURFACE(((1.00036190279925,0.681135153781591,1.),(1.00030231339256,
0.733638110485514,1.),(1.00024889602585,0.78070301425877,1.),(1.00015092061994,
0.867027057078926,1.),(1.00010588522078,0.90670678781828,1.),(1.00006613376638,
0.941730947393792,1.)))
REPRESENTATION_ITEM('')
SURFACE()
);
#191=(
BOUNDED_SURFACE()
B_SPLINE_SURFACE(3,2,((#31881,#31882,#31883),(#31884,#31885,#31886),(#31887,
#31888,#31889),(#31890,#31891,#31892),(#31893,#31894,#31895),(#31896,#31897,
#31898)),.UNSPECIFIED.,.F.,.F.,.F.)
B_SPLINE_SURFACE_WITH_KNOTS((4,2,4),(3,3),(0.000885251653512216,0.00152482279265937,
0.00216439393180653),(0.,1.),.UNSPECIFIED.)
GEOMETRIC_REPRESENTATION_ITEM()
RATIONAL_B_SPLINE_SURFACE(((1.,0.70710678118663,1.),(1.,0.749482754810037,
1.),(1.,0.788287146221274,1.),(1.,0.860112372061843,1.),(1.,0.893279480387377,
1.),(1.,0.923879532511264,1.)))
REPRESENTATION_ITEM('')
SURFACE()
);
#192=(
BOUNDED_SURFACE()
B_SPLINE_SURFACE(3,2,((#31902,#31903,#31904),(#31905,#31906,#31907),(#31908,
#31909,#31910),(#31911,#31912,#31913),(#31914,#31915,#31916),(#31917,#31918,
#31919),(#31920,#31921,#31922),(#31923,#31924,#31925)),.UNSPECIFIED.,.F.,
 .F.,.F.)
B_SPLINE_SURFACE_WITH_KNOTS((4,2,2,4),(3,3),(0.0113699589780933,0.0215499319036469,
0.0263330282216038,0.0317270101266359),(0.,1.00072721387447),
 .UNSPECIFIED.)
GEOMETRIC_REPRESENTATION_ITEM()
RATIONAL_B_SPLINE_SURFACE(((1.,0.904674950782418,1.00013864339675),(1.,
0.909119912852179,1.00013217852057),(1.,0.913289332696403,1.00012611440066),
(1.,0.918180475673232,1.00011900058659),(1.,0.919557331130196,1.0001169980498),
(1.,0.921907306767051,1.00011358018003),(1.,0.922815134506009,1.00011225981017),
(1.,0.923326705442552,1.00011151576721)))
REPRESENTATION_ITEM('')
SURFACE()
);
#193=(
BOUNDED_SURFACE()
B_SPLINE_SURFACE(3,2,((#31979,#31980,#31981),(#31982,#31983,#31984),(#31985,
#31986,#31987),(#31988,#31989,#31990),(#31991,#31992,#31993),(#31994,#31995,
#31996)),.UNSPECIFIED.,.F.,.F.,.F.)
B_SPLINE_SURFACE_WITH_KNOTS((4,2,4),(3,3),(0.00106076019035493,0.00169847101257236,
0.0023361818347898),(0.,1.),.UNSPECIFIED.)
GEOMETRIC_REPRESENTATION_ITEM()
RATIONAL_B_SPLINE_SURFACE(((1.,0.707106781186638,1.),(1.,0.749398144477821,
1.),(1.,0.787950893928113,1.),(1.,0.859993702050145,1.),(1.,0.893886360721809,
1.),(1.,0.923879532510763,1.)))
REPRESENTATION_ITEM('')
SURFACE()
);
#194=(
BOUNDED_SURFACE()
B_SPLINE_SURFACE(3,2,((#32019,#32020,#32021),(#32022,#32023,#32024),(#32025,
#32026,#32027),(#32028,#32029,#32030),(#32031,#32032,#32033),(#32034,#32035,
#32036),(#32037,#32038,#32039),(#32040,#32041,#32042)),.UNSPECIFIED.,.F.,
 .F.,.F.)
B_SPLINE_SURFACE_WITH_KNOTS((4,2,2,4),(3,3),(0.0119004725361997,0.0216177878121993,
0.0264008481563403,0.0313322083719226),(-0.000264627303556973,1.),
 .UNSPECIFIED.)
GEOMETRIC_REPRESENTATION_ITEM()
RATIONAL_B_SPLINE_SURFACE(((1.00005010827744,0.905322926311723,1.),(1.00004787697101,
0.909538867754481,1.),(1.00004579077809,0.913480624490332,1.),(1.00004328315836,
0.918218646036241,1.),(1.0000425548475,0.919594752824379,1.),(1.00004136830425,
0.921836666702374,1.),(1.00004091524806,0.922692693638322,1.),(1.00004063516841,
0.923221890058778,1.)))
REPRESENTATION_ITEM('')
SURFACE()
);
#195=B_SPLINE_SURFACE_WITH_KNOTS('',3,3,((#22254,#22255,#22256,#22257,#22258,
#22259,#22260,#22261,#22262,#22263),(#22264,#22265,#22266,#22267,#22268,
#22269,#22270,#22271,#22272,#22273),(#22274,#22275,#22276,#22277,#22278,
#22279,#22280,#22281,#22282,#22283),(#22284,#22285,#22286,#22287,#22288,
#22289,#22290,#22291,#22292,#22293),(#22294,#22295,#22296,#22297,#22298,
#22299,#22300,#22301,#22302,#22303),(#22304,#22305,#22306,#22307,#22308,
#22309,#22310,#22311,#22312,#22313)),.UNSPECIFIED.,.F.,.F.,.F.,(4,2,4),
(4,2,2,2,4),(0.,0.5,1.),(0.,0.25,0.5,0.75,1.),.UNSPECIFIED.);
#196=B_SPLINE_SURFACE_WITH_KNOTS('',3,3,((#22344,#22345,#22346,#22347,#22348,
#22349,#22350,#22351),(#22352,#22353,#22354,#22355,#22356,#22357,#22358,
#22359),(#22360,#22361,#22362,#22363,#22364,#22365,#22366,#22367),(#22368,
#22369,#22370,#22371,#22372,#22373,#22374,#22375),(#22376,#22377,#22378,
#22379,#22380,#22381,#22382,#22383),(#22384,#22385,#22386,#22387,#22388,
#22389,#22390,#22391),(#22392,#22393,#22394,#22395,#22396,#22397,#22398,
#22399),(#22400,#22401,#22402,#22403,#22404,#22405,#22406,#22407)),
 .UNSPECIFIED.,.F.,.F.,.F.,(4,2,2,4),(4,2,2,4),(0.,0.25,0.5,1.),(0.,0.25,
0.5,1.),.UNSPECIFIED.);
#197=B_SPLINE_SURFACE_WITH_KNOTS('',3,3,((#22425,#22426,#22427,#22428,#22429,
#22430),(#22431,#22432,#22433,#22434,#22435,#22436),(#22437,#22438,#22439,
#22440,#22441,#22442),(#22443,#22444,#22445,#22446,#22447,#22448),(#22449,
#22450,#22451,#22452,#22453,#22454),(#22455,#22456,#22457,#22458,#22459,
#22460),(#22461,#22462,#22463,#22464,#22465,#22466),(#22467,#22468,#22469,
#22470,#22471,#22472)),.UNSPECIFIED.,.F.,.F.,.F.,(4,2,2,4),(4,2,4),(0.,
0.25,0.5,1.),(0.,0.5,1.),.UNSPECIFIED.);
#198=B_SPLINE_SURFACE_WITH_KNOTS('',3,3,((#22495,#22496,#22497,#22498,#22499,
#22500,#22501,#22502),(#22503,#22504,#22505,#22506,#22507,#22508,#22509,
#22510),(#22511,#22512,#22513,#22514,#22515,#22516,#22517,#22518),(#22519,
#22520,#22521,#22522,#22523,#22524,#22525,#22526),(#22527,#22528,#22529,
#22530,#22531,#22532,#22533,#22534),(#22535,#22536,#22537,#22538,#22539,
#22540,#22541,#22542)),.UNSPECIFIED.,.F.,.F.,.F.,(4,2,4),(4,2,2,4),(0.,
0.5,1.),(0.,0.25,0.5,1.),.UNSPECIFIED.);
#199=B_SPLINE_SURFACE_WITH_KNOTS('',3,3,((#22566,#22567,#22568,#22569,#22570,
#22571,#22572,#22573),(#22574,#22575,#22576,#22577,#22578,#22579,#22580,
#22581),(#22582,#22583,#22584,#22585,#22586,#22587,#22588,#22589),(#22590,
#22591,#22592,#22593,#22594,#22595,#22596,#22597),(#22598,#22599,#22600,
#22601,#22602,#22603,#22604,#22605),(#22606,#22607,#22608,#22609,#22610,
#22611,#22612,#22613),(#22614,#22615,#22616,#22617,#22618,#22619,#22620,
#22621),(#22622,#22623,#22624,#22625,#22626,#22627,#22628,#22629)),
 .UNSPECIFIED.,.F.,.F.,.F.,(4,2,2,4),(4,2,2,4),(0.,0.25,0.5,1.),(0.,0.25,
0.5,1.),.UNSPECIFIED.);
#200=B_SPLINE_SURFACE_WITH_KNOTS('',3,3,((#22698,#22699,#22700,#22701,#22702,
#22703),(#22704,#22705,#22706,#22707,#22708,#22709),(#22710,#22711,#22712,
#22713,#22714,#22715),(#22716,#22717,#22718,#22719,#22720,#22721),(#22722,
#22723,#22724,#22725,#22726,#22727),(#22728,#22729,#22730,#22731,#22732,
#22733),(#22734,#22735,#22736,#22737,#22738,#22739),(#22740,#22741,#22742,
#22743,#22744,#22745)),.UNSPECIFIED.,.F.,.F.,.F.,(4,2,2,4),(4,2,4),(0.,
0.25,0.5,1.),(0.,0.5,1.),.UNSPECIFIED.);
#201=B_SPLINE_SURFACE_WITH_KNOTS('',3,3,((#22776,#22777,#22778,#22779,#22780,
#22781,#22782,#22783),(#22784,#22785,#22786,#22787,#22788,#22789,#22790,
#22791),(#22792,#22793,#22794,#22795,#22796,#22797,#22798,#22799),(#22800,
#22801,#22802,#22803,#22804,#22805,#22806,#22807),(#22808,#22809,#22810,
#22811,#22812,#22813,#22814,#22815),(#22816,#22817,#22818,#22819,#22820,
#22821,#22822,#22823)),.UNSPECIFIED.,.F.,.F.,.F.,(4,2,4),(4,2,2,4),(0.,
0.5,1.),(0.,0.25,0.5,1.),.UNSPECIFIED.);
#202=B_SPLINE_SURFACE_WITH_KNOTS('',3,3,((#22847,#22848,#22849,#22850,#22851,
#22852,#22853,#22854),(#22855,#22856,#22857,#22858,#22859,#22860,#22861,
#22862),(#22863,#22864,#22865,#22866,#22867,#22868,#22869,#22870),(#22871,
#22872,#22873,#22874,#22875,#22876,#22877,#22878),(#22879,#22880,#22881,
#22882,#22883,#22884,#22885,#22886),(#22887,#22888,#22889,#22890,#22891,
#22892,#22893,#22894),(#22895,#22896,#22897,#22898,#22899,#22900,#22901,
#22902),(#22903,#22904,#22905,#22906,#22907,#22908,#22909,#22910)),
 .UNSPECIFIED.,.F.,.F.,.F.,(4,2,2,4),(4,2,2,4),(0.,0.25,0.5,1.),(0.,0.25,
0.5,1.),.UNSPECIFIED.);
#203=B_SPLINE_SURFACE_WITH_KNOTS('',3,3,((#22928,#22929,#22930,#22931,#22932,
#22933),(#22934,#22935,#22936,#22937,#22938,#22939),(#22940,#22941,#22942,
#22943,#22944,#22945),(#22946,#22947,#22948,#22949,#22950,#22951),(#22952,
#22953,#22954,#22955,#22956,#22957),(#22958,#22959,#22960,#22961,#22962,
#22963),(#22964,#22965,#22966,#22967,#22968,#22969),(#22970,#22971,#22972,
#22973,#22974,#22975),(#22976,#22977,#22978,#22979,#22980,#22981),(#22982,
#22983,#22984,#22985,#22986,#22987)),.UNSPECIFIED.,.F.,.F.,.F.,(4,2,2,2,
4),(4,2,4),(0.,0.25,0.5,0.75,1.),(0.,0.5,1.),.UNSPECIFIED.);
#204=B_SPLINE_SURFACE_WITH_KNOTS('',3,3,((#23007,#23008,#23009,#23010,#23011,
#23012,#23013,#23014,#23015,#23016),(#23017,#23018,#23019,#23020,#23021,
#23022,#23023,#23024,#23025,#23026),(#23027,#23028,#23029,#23030,#23031,
#23032,#23033,#23034,#23035,#23036),(#23037,#23038,#23039,#23040,#23041,
#23042,#23043,#23044,#23045,#23046),(#23047,#23048,#23049,#23050,#23051,
#23052,#23053,#23054,#23055,#23056),(#23057,#23058,#23059,#23060,#23061,
#23062,#23063,#23064,#23065,#23066)),.UNSPECIFIED.,.F.,.F.,.F.,(4,2,4),
(4,2,2,2,4),(0.,0.5,1.),(0.,0.25,0.5,0.75,1.),.UNSPECIFIED.);
#205=B_SPLINE_SURFACE_WITH_KNOTS('',3,3,((#23075,#23076,#23077,#23078,#23079,
#23080,#23081,#23082,#23083,#23084),(#23085,#23086,#23087,#23088,#23089,
#23090,#23091,#23092,#23093,#23094),(#23095,#23096,#23097,#23098,#23099,
#23100,#23101,#23102,#23103,#23104),(#23105,#23106,#23107,#23108,#23109,
#23110,#23111,#23112,#23113,#23114),(#23115,#23116,#23117,#23118,#23119,
#23120,#23121,#23122,#23123,#23124),(#23125,#23126,#23127,#23128,#23129,
#23130,#23131,#23132,#23133,#23134)),.UNSPECIFIED.,.F.,.F.,.F.,(4,2,4),
(4,2,2,2,4),(0.,0.5,1.),(0.,0.25,0.5,0.75,1.),.UNSPECIFIED.);
#206=B_SPLINE_SURFACE_WITH_KNOTS('',3,3,((#23165,#23166,#23167,#23168,#23169,
#23170,#23171,#23172),(#23173,#23174,#23175,#23176,#23177,#23178,#23179,
#23180),(#23181,#23182,#23183,#23184,#23185,#23186,#23187,#23188),(#23189,
#23190,#23191,#23192,#23193,#23194,#23195,#23196),(#23197,#23198,#23199,
#23200,#23201,#23202,#23203,#23204),(#23205,#23206,#23207,#23208,#23209,
#23210,#23211,#23212),(#23213,#23214,#23215,#23216,#23217,#23218,#23219,
#23220),(#23221,#23222,#23223,#23224,#23225,#23226,#23227,#23228)),
 .UNSPECIFIED.,.F.,.F.,.F.,(4,2,2,4),(4,2,2,4),(0.,0.25,0.5,1.),(0.,0.25,
0.5,1.),.UNSPECIFIED.);
#207=B_SPLINE_SURFACE_WITH_KNOTS('',3,3,((#23246,#23247,#23248,#23249,#23250,
#23251),(#23252,#23253,#23254,#23255,#23256,#23257),(#23258,#23259,#23260,
#23261,#23262,#23263),(#23264,#23265,#23266,#23267,#23268,#23269),(#23270,
#23271,#23272,#23273,#23274,#23275),(#23276,#23277,#23278,#23279,#23280,
#23281),(#23282,#23283,#23284,#23285,#23286,#23287),(#23288,#23289,#23290,
#23291,#23292,#23293)),.UNSPECIFIED.,.F.,.F.,.F.,(4,2,2,4),(4,2,4),(0.,
0.25,0.5,1.),(0.,0.5,1.),.UNSPECIFIED.);
#208=B_SPLINE_SURFACE_WITH_KNOTS('',3,3,((#23316,#23317,#23318,#23319,#23320,
#23321,#23322,#23323),(#23324,#23325,#23326,#23327,#23328,#23329,#23330,
#23331),(#23332,#23333,#23334,#23335,#23336,#23337,#23338,#23339),(#23340,
#23341,#23342,#23343,#23344,#23345,#23346,#23347),(#23348,#23349,#23350,
#23351,#23352,#23353,#23354,#23355),(#23356,#23357,#23358,#23359,#23360,
#23361,#23362,#23363)),.UNSPECIFIED.,.F.,.F.,.F.,(4,2,4),(4,2,2,4),(0.,
0.5,1.),(0.,0.25,0.5,1.),.UNSPECIFIED.);
#209=B_SPLINE_SURFACE_WITH_KNOTS('',3,3,((#23387,#23388,#23389,#23390,#23391,
#23392,#23393,#23394),(#23395,#23396,#23397,#23398,#23399,#23400,#23401,
#23402),(#23403,#23404,#23405,#23406,#23407,#23408,#23409,#23410),(#23411,
#23412,#23413,#23414,#23415,#23416,#23417,#23418),(#23419,#23420,#23421,
#23422,#23423,#23424,#23425,#23426),(#23427,#23428,#23429,#23430,#23431,
#23432,#23433,#23434),(#23435,#23436,#23437,#23438,#23439,#23440,#23441,
#23442),(#23443,#23444,#23445,#23446,#23447,#23448,#23449,#23450)),
 .UNSPECIFIED.,.F.,.F.,.F.,(4,2,2,4),(4,2,2,4),(0.,0.25,0.5,1.),(0.,0.25,
0.5,1.),.UNSPECIFIED.);
#210=B_SPLINE_SURFACE_WITH_KNOTS('',3,3,((#23519,#23520,#23521,#23522,#23523,
#23524),(#23525,#23526,#23527,#23528,#23529,#23530),(#23531,#23532,#23533,
#23534,#23535,#23536),(#23537,#23538,#23539,#23540,#23541,#23542),(#23543,
#23544,#23545,#23546,#23547,#23548),(#23549,#23550,#23551,#23552,#23553,
#23554),(#23555,#23556,#23557,#23558,#23559,#23560),(#23561,#23562,#23563,
#23564,#23565,#23566)),.UNSPECIFIED.,.F.,.F.,.F.,(4,2,2,4),(4,2,4),(0.,
0.25,0.5,1.),(0.,0.5,1.),.UNSPECIFIED.);
#211=B_SPLINE_SURFACE_WITH_KNOTS('',3,3,((#23597,#23598,#23599,#23600,#23601,
#23602,#23603,#23604),(#23605,#23606,#23607,#23608,#23609,#23610,#23611,
#23612),(#23613,#23614,#23615,#23616,#23617,#23618,#23619,#23620),(#23621,
#23622,#23623,#23624,#23625,#23626,#23627,#23628),(#23629,#23630,#23631,
#23632,#23633,#23634,#23635,#23636),(#23637,#23638,#23639,#23640,#23641,
#23642,#23643,#23644)),.UNSPECIFIED.,.F.,.F.,.F.,(4,2,4),(4,2,2,4),(0.,
0.5,1.),(0.,0.25,0.5,1.),.UNSPECIFIED.);
#212=B_SPLINE_SURFACE_WITH_KNOTS('',3,3,((#23668,#23669,#23670,#23671,#23672,
#23673,#23674,#23675),(#23676,#23677,#23678,#23679,#23680,#23681,#23682,
#23683),(#23684,#23685,#23686,#23687,#23688,#23689,#23690,#23691),(#23692,
#23693,#23694,#23695,#23696,#23697,#23698,#23699),(#23700,#23701,#23702,
#23703,#23704,#23705,#23706,#23707),(#23708,#23709,#23710,#23711,#23712,
#23713,#23714,#23715),(#23716,#23717,#23718,#23719,#23720,#23721,#23722,
#23723),(#23724,#23725,#23726,#23727,#23728,#23729,#23730,#23731)),
 .UNSPECIFIED.,.F.,.F.,.F.,(4,2,2,4),(4,2,2,4),(0.,0.25,0.5,1.),(0.,0.25,
0.5,1.),.UNSPECIFIED.);
#213=B_SPLINE_SURFACE_WITH_KNOTS('',3,3,((#23749,#23750,#23751,#23752,#23753,
#23754),(#23755,#23756,#23757,#23758,#23759,#23760),(#23761,#23762,#23763,
#23764,#23765,#23766),(#23767,#23768,#23769,#23770,#23771,#23772),(#23773,
#23774,#23775,#23776,#23777,#23778),(#23779,#23780,#23781,#23782,#23783,
#23784),(#23785,#23786,#23787,#23788,#23789,#23790),(#23791,#23792,#23793,
#23794,#23795,#23796),(#23797,#23798,#23799,#23800,#23801,#23802),(#23803,
#23804,#23805,#23806,#23807,#23808)),.UNSPECIFIED.,.F.,.F.,.F.,(4,2,2,2,
4),(4,2,4),(0.,0.25,0.5,0.75,1.),(0.,0.5,1.),.UNSPECIFIED.);
#214=B_SPLINE_SURFACE_WITH_KNOTS('',3,3,((#23828,#23829,#23830,#23831,#23832,
#23833,#23834,#23835,#23836,#23837),(#23838,#23839,#23840,#23841,#23842,
#23843,#23844,#23845,#23846,#23847),(#23848,#23849,#23850,#23851,#23852,
#23853,#23854,#23855,#23856,#23857),(#23858,#23859,#23860,#23861,#23862,
#23863,#23864,#23865,#23866,#23867),(#23868,#23869,#23870,#23871,#23872,
#23873,#23874,#23875,#23876,#23877),(#23878,#23879,#23880,#23881,#23882,
#23883,#23884,#23885,#23886,#23887)),.UNSPECIFIED.,.F.,.F.,.F.,(4,2,4),
(4,2,2,2,4),(0.,0.5,1.),(0.,0.25,0.5,0.75,1.),.UNSPECIFIED.);
#215=B_SPLINE_SURFACE_WITH_KNOTS('',3,3,((#24322,#24323,#24324,#24325,#24326,
#24327,#24328,#24329),(#24330,#24331,#24332,#24333,#24334,#24335,#24336,
#24337),(#24338,#24339,#24340,#24341,#24342,#24343,#24344,#24345),(#24346,
#24347,#24348,#24349,#24350,#24351,#24352,#24353),(#24354,#24355,#24356,
#24357,#24358,#24359,#24360,#24361),(#24362,#24363,#24364,#24365,#24366,
#24367,#24368,#24369),(#24370,#24371,#24372,#24373,#24374,#24375,#24376,
#24377),(#24378,#24379,#24380,#24381,#24382,#24383,#24384,#24385)),
 .UNSPECIFIED.,.F.,.F.,.F.,(4,2,2,4),(4,2,2,4),(0.,0.25,0.5,1.),(0.,0.25,
0.5,1.),.UNSPECIFIED.);
#216=B_SPLINE_SURFACE_WITH_KNOTS('',3,3,((#25176,#25177,#25178,#25179,#25180,
#25181),(#25182,#25183,#25184,#25185,#25186,#25187),(#25188,#25189,#25190,
#25191,#25192,#25193),(#25194,#25195,#25196,#25197,#25198,#25199),(#25200,
#25201,#25202,#25203,#25204,#25205),(#25206,#25207,#25208,#25209,#25210,
#25211),(#25212,#25213,#25214,#25215,#25216,#25217),(#25218,#25219,#25220,
#25221,#25222,#25223),(#25224,#25225,#25226,#25227,#25228,#25229),(#25230,
#25231,#25232,#25233,#25234,#25235)),.UNSPECIFIED.,.F.,.F.,.F.,(4,2,2,2,
4),(4,2,4),(0.,0.25,0.5,0.75,1.),(0.,0.5,1.),.UNSPECIFIED.);
#217=B_SPLINE_SURFACE_WITH_KNOTS('',3,3,((#26187,#26188,#26189,#26190,#26191,
#26192,#26193,#26194),(#26195,#26196,#26197,#26198,#26199,#26200,#26201,
#26202),(#26203,#26204,#26205,#26206,#26207,#26208,#26209,#26210),(#26211,
#26212,#26213,#26214,#26215,#26216,#26217,#26218),(#26219,#26220,#26221,
#26222,#26223,#26224,#26225,#26226),(#26227,#26228,#26229,#26230,#26231,
#26232,#26233,#26234),(#26235,#26236,#26237,#26238,#26239,#26240,#26241,
#26242),(#26243,#26244,#26245,#26246,#26247,#26248,#26249,#26250)),
 .UNSPECIFIED.,.F.,.F.,.F.,(4,2,2,4),(4,2,2,4),(0.,0.25,0.5,1.),(0.,0.25,
0.5,1.),.UNSPECIFIED.);
#218=B_SPLINE_SURFACE_WITH_KNOTS('',3,3,((#27764,#27765,#27766,#27767,#27768,
#27769),(#27770,#27771,#27772,#27773,#27774,#27775),(#27776,#27777,#27778,
#27779,#27780,#27781),(#27782,#27783,#27784,#27785,#27786,#27787),(#27788,
#27789,#27790,#27791,#27792,#27793),(#27794,#27795,#27796,#27797,#27798,
#27799),(#27800,#27801,#27802,#27803,#27804,#27805),(#27806,#27807,#27808,
#27809,#27810,#27811),(#27812,#27813,#27814,#27815,#27816,#27817),(#27818,
#27819,#27820,#27821,#27822,#27823)),.UNSPECIFIED.,.F.,.F.,.F.,(4,2,2,2,
4),(4,2,4),(0.,0.25,0.5,0.75,1.),(0.,0.5,1.),.UNSPECIFIED.);
#219=B_SPLINE_SURFACE_WITH_KNOTS('',3,3,((#29443,#29444,#29445,#29446,#29447,
#29448,#29449,#29450),(#29451,#29452,#29453,#29454,#29455,#29456,#29457,
#29458),(#29459,#29460,#29461,#29462,#29463,#29464,#29465,#29466),(#29467,
#29468,#29469,#29470,#29471,#29472,#29473,#29474),(#29475,#29476,#29477,
#29478,#29479,#29480,#29481,#29482),(#29483,#29484,#29485,#29486,#29487,
#29488,#29489,#29490)),.UNSPECIFIED.,.F.,.F.,.F.,(4,2,4),(4,2,2,4),(0.,
0.5,1.),(0.,0.25,0.5,1.),.UNSPECIFIED.);
#220=B_SPLINE_SURFACE_WITH_KNOTS('',3,3,((#29521,#29522,#29523,#29524,#29525,
#29526,#29527,#29528),(#29529,#29530,#29531,#29532,#29533,#29534,#29535,
#29536),(#29537,#29538,#29539,#29540,#29541,#29542,#29543,#29544),(#29545,
#29546,#29547,#29548,#29549,#29550,#29551,#29552),(#29553,#29554,#29555,
#29556,#29557,#29558,#29559,#29560),(#29561,#29562,#29563,#29564,#29565,
#29566,#29567,#29568),(#29569,#29570,#29571,#29572,#29573,#29574,#29575,
#29576),(#29577,#29578,#29579,#29580,#29581,#29582,#29583,#29584)),
 .UNSPECIFIED.,.F.,.F.,.F.,(4,2,2,4),(4,2,2,4),(0.,0.25,0.5,1.),(0.,0.25,
0.5,1.),.UNSPECIFIED.);
#221=B_SPLINE_SURFACE_WITH_KNOTS('',3,3,((#29602,#29603,#29604,#29605,#29606,
#29607),(#29608,#29609,#29610,#29611,#29612,#29613),(#29614,#29615,#29616,
#29617,#29618,#29619),(#29620,#29621,#29622,#29623,#29624,#29625),(#29626,
#29627,#29628,#29629,#29630,#29631),(#29632,#29633,#29634,#29635,#29636,
#29637),(#29638,#29639,#29640,#29641,#29642,#29643),(#29644,#29645,#29646,
#29647,#29648,#29649),(#29650,#29651,#29652,#29653,#29654,#29655),(#29656,
#29657,#29658,#29659,#29660,#29661)),.UNSPECIFIED.,.F.,.F.,.F.,(4,2,2,2,
4),(4,2,4),(0.,0.25,0.5,0.75,1.),(0.,0.5,1.),.UNSPECIFIED.);
#222=B_SPLINE_SURFACE_WITH_KNOTS('',3,3,((#29681,#29682,#29683,#29684,#29685,
#29686,#29687,#29688,#29689,#29690),(#29691,#29692,#29693,#29694,#29695,
#29696,#29697,#29698,#29699,#29700),(#29701,#29702,#29703,#29704,#29705,
#29706,#29707,#29708,#29709,#29710),(#29711,#29712,#29713,#29714,#29715,
#29716,#29717,#29718,#29719,#29720),(#29721,#29722,#29723,#29724,#29725,
#29726,#29727,#29728,#29729,#29730),(#29731,#29732,#29733,#29734,#29735,
#29736,#29737,#29738,#29739,#29740)),.UNSPECIFIED.,.F.,.F.,.F.,(4,2,4),
(4,2,2,2,4),(0.,0.5,1.),(0.,0.25,0.5,0.75,1.),.UNSPECIFIED.);
#223=B_SPLINE_SURFACE_WITH_KNOTS('',3,3,((#29764,#29765,#29766,#29767,#29768,
#29769,#29770,#29771),(#29772,#29773,#29774,#29775,#29776,#29777,#29778,
#29779),(#29780,#29781,#29782,#29783,#29784,#29785,#29786,#29787),(#29788,
#29789,#29790,#29791,#29792,#29793,#29794,#29795),(#29796,#29797,#29798,
#29799,#29800,#29801,#29802,#29803),(#29804,#29805,#29806,#29807,#29808,
#29809,#29810,#29811),(#29812,#29813,#29814,#29815,#29816,#29817,#29818,
#29819),(#29820,#29821,#29822,#29823,#29824,#29825,#29826,#29827)),
 .UNSPECIFIED.,.F.,.F.,.F.,(4,2,2,4),(4,2,2,4),(0.,0.25,0.5,1.),(0.,0.25,
0.5,1.),.UNSPECIFIED.);
#224=B_SPLINE_SURFACE_WITH_KNOTS('',3,3,((#29903,#29904,#29905,#29906,#29907,
#29908),(#29909,#29910,#29911,#29912,#29913,#29914),(#29915,#29916,#29917,
#29918,#29919,#29920),(#29921,#29922,#29923,#29924,#29925,#29926),(#29927,
#29928,#29929,#29930,#29931,#29932),(#29933,#29934,#29935,#29936,#29937,
#29938),(#29939,#29940,#29941,#29942,#29943,#29944),(#29945,#29946,#29947,
#29948,#29949,#29950)),.UNSPECIFIED.,.F.,.F.,.F.,(4,2,2,4),(4,2,4),(0.,
0.25,0.5,1.),(0.,0.5,1.),.UNSPECIFIED.);
#225=B_SPLINE_SURFACE_WITH_KNOTS('',3,3,((#29981,#29982,#29983,#29984,#29985,
#29986,#29987,#29988),(#29989,#29990,#29991,#29992,#29993,#29994,#29995,
#29996),(#29997,#29998,#29999,#30000,#30001,#30002,#30003,#30004),(#30005,
#30006,#30007,#30008,#30009,#30010,#30011,#30012),(#30013,#30014,#30015,
#30016,#30017,#30018,#30019,#30020),(#30021,#30022,#30023,#30024,#30025,
#30026,#30027,#30028)),.UNSPECIFIED.,.F.,.F.,.F.,(4,2,4),(4,2,2,4),(0.,
0.5,1.),(0.,0.25,0.5,1.),.UNSPECIFIED.);
#226=B_SPLINE_SURFACE_WITH_KNOTS('',3,3,((#30052,#30053,#30054,#30055,#30056,
#30057,#30058,#30059),(#30060,#30061,#30062,#30063,#30064,#30065,#30066,
#30067),(#30068,#30069,#30070,#30071,#30072,#30073,#30074,#30075),(#30076,
#30077,#30078,#30079,#30080,#30081,#30082,#30083),(#30084,#30085,#30086,
#30087,#30088,#30089,#30090,#30091),(#30092,#30093,#30094,#30095,#30096,
#30097,#30098,#30099),(#30100,#30101,#30102,#30103,#30104,#30105,#30106,
#30107),(#30108,#30109,#30110,#30111,#30112,#30113,#30114,#30115)),
 .UNSPECIFIED.,.F.,.F.,.F.,(4,2,2,4),(4,2,2,4),(0.,0.25,0.5,1.),(0.,0.25,
0.5,1.),.UNSPECIFIED.);
#227=B_SPLINE_SURFACE_WITH_KNOTS('',3,3,((#30133,#30134,#30135,#30136,#30137,
#30138),(#30139,#30140,#30141,#30142,#30143,#30144),(#30145,#30146,#30147,
#30148,#30149,#30150),(#30151,#30152,#30153,#30154,#30155,#30156),(#30157,
#30158,#30159,#30160,#30161,#30162),(#30163,#30164,#30165,#30166,#30167,
#30168),(#30169,#30170,#30171,#30172,#30173,#30174),(#30175,#30176,#30177,
#30178,#30179,#30180),(#30181,#30182,#30183,#30184,#30185,#30186),(#30187,
#30188,#30189,#30190,#30191,#30192)),.UNSPECIFIED.,.F.,.F.,.F.,(4,2,2,2,
4),(4,2,4),(0.,0.25,0.5,0.75,1.),(0.,0.5,1.),.UNSPECIFIED.);
#228=B_SPLINE_SURFACE_WITH_KNOTS('',3,3,((#30212,#30213,#30214,#30215,#30216,
#30217,#30218,#30219,#30220,#30221),(#30222,#30223,#30224,#30225,#30226,
#30227,#30228,#30229,#30230,#30231),(#30232,#30233,#30234,#30235,#30236,
#30237,#30238,#30239,#30240,#30241),(#30242,#30243,#30244,#30245,#30246,
#30247,#30248,#30249,#30250,#30251),(#30252,#30253,#30254,#30255,#30256,
#30257,#30258,#30259,#30260,#30261),(#30262,#30263,#30264,#30265,#30266,
#30267,#30268,#30269,#30270,#30271)),.UNSPECIFIED.,.F.,.F.,.F.,(4,2,4),
(4,2,2,2,4),(0.,0.5,1.),(0.,0.25,0.5,0.75,1.),.UNSPECIFIED.);
#229=B_SPLINE_SURFACE_WITH_KNOTS('',3,3,((#30280,#30281,#30282,#30283,#30284,
#30285,#30286,#30287,#30288,#30289),(#30290,#30291,#30292,#30293,#30294,
#30295,#30296,#30297,#30298,#30299),(#30300,#30301,#30302,#30303,#30304,
#30305,#30306,#30307,#30308,#30309),(#30310,#30311,#30312,#30313,#30314,
#30315,#30316,#30317,#30318,#30319),(#30320,#30321,#30322,#30323,#30324,
#30325,#30326,#30327,#30328,#30329),(#30330,#30331,#30332,#30333,#30334,
#30335,#30336,#30337,#30338,#30339)),.UNSPECIFIED.,.F.,.F.,.F.,(4,2,4),
(4,2,2,2,4),(0.,0.5,1.),(0.,0.25,0.5,0.75,1.),.UNSPECIFIED.);
#230=B_SPLINE_SURFACE_WITH_KNOTS('',3,3,((#30370,#30371,#30372,#30373,#30374,
#30375,#30376,#30377),(#30378,#30379,#30380,#30381,#30382,#30383,#30384,
#30385),(#30386,#30387,#30388,#30389,#30390,#30391,#30392,#30393),(#30394,
#30395,#30396,#30397,#30398,#30399,#30400,#30401),(#30402,#30403,#30404,
#30405,#30406,#30407,#30408,#30409),(#30410,#30411,#30412,#30413,#30414,
#30415,#30416,#30417),(#30418,#30419,#30420,#30421,#30422,#30423,#30424,
#30425),(#30426,#30427,#30428,#30429,#30430,#30431,#30432,#30433)),
 .UNSPECIFIED.,.F.,.F.,.F.,(4,2,2,4),(4,2,2,4),(0.,0.25,0.5,1.),(0.,0.25,
0.5,1.),.UNSPECIFIED.);
#231=B_SPLINE_SURFACE_WITH_KNOTS('',3,3,((#30451,#30452,#30453,#30454,#30455,
#30456),(#30457,#30458,#30459,#30460,#30461,#30462),(#30463,#30464,#30465,
#30466,#30467,#30468),(#30469,#30470,#30471,#30472,#30473,#30474),(#30475,
#30476,#30477,#30478,#30479,#30480),(#30481,#30482,#30483,#30484,#30485,
#30486),(#30487,#30488,#30489,#30490,#30491,#30492),(#30493,#30494,#30495,
#30496,#30497,#30498)),.UNSPECIFIED.,.F.,.F.,.F.,(4,2,2,4),(4,2,4),(0.,
0.25,0.5,1.),(0.,0.5,1.),.UNSPECIFIED.);
#232=B_SPLINE_SURFACE_WITH_KNOTS('',3,3,((#30521,#30522,#30523,#30524,#30525,
#30526,#30527,#30528),(#30529,#30530,#30531,#30532,#30533,#30534,#30535,
#30536),(#30537,#30538,#30539,#30540,#30541,#30542,#30543,#30544),(#30545,
#30546,#30547,#30548,#30549,#30550,#30551,#30552),(#30553,#30554,#30555,
#30556,#30557,#30558,#30559,#30560),(#30561,#30562,#30563,#30564,#30565,
#30566,#30567,#30568)),.UNSPECIFIED.,.F.,.F.,.F.,(4,2,4),(4,2,2,4),(0.,
0.5,1.),(0.,0.25,0.5,1.),.UNSPECIFIED.);
#233=B_SPLINE_SURFACE_WITH_KNOTS('',3,3,((#30592,#30593,#30594,#30595,#30596,
#30597,#30598,#30599),(#30600,#30601,#30602,#30603,#30604,#30605,#30606,
#30607),(#30608,#30609,#30610,#30611,#30612,#30613,#30614,#30615),(#30616,
#30617,#30618,#30619,#30620,#30621,#30622,#30623),(#30624,#30625,#30626,
#30627,#30628,#30629,#30630,#30631),(#30632,#30633,#30634,#30635,#30636,
#30637,#30638,#30639),(#30640,#30641,#30642,#30643,#30644,#30645,#30646,
#30647),(#30648,#30649,#30650,#30651,#30652,#30653,#30654,#30655)),
 .UNSPECIFIED.,.F.,.F.,.F.,(4,2,2,4),(4,2,2,4),(0.,0.25,0.5,1.),(0.,0.25,
0.5,1.),.UNSPECIFIED.);
#234=B_SPLINE_SURFACE_WITH_KNOTS('',3,3,((#30724,#30725,#30726,#30727,#30728,
#30729),(#30730,#30731,#30732,#30733,#30734,#30735),(#30736,#30737,#30738,
#30739,#30740,#30741),(#30742,#30743,#30744,#30745,#30746,#30747),(#30748,
#30749,#30750,#30751,#30752,#30753),(#30754,#30755,#30756,#30757,#30758,
#30759),(#30760,#30761,#30762,#30763,#30764,#30765),(#30766,#30767,#30768,
#30769,#30770,#30771)),.UNSPECIFIED.,.F.,.F.,.F.,(4,2,2,4),(4,2,4),(0.,
0.25,0.5,1.),(0.,0.5,1.),.UNSPECIFIED.);
#235=B_SPLINE_SURFACE_WITH_KNOTS('',3,3,((#30802,#30803,#30804,#30805,#30806,
#30807,#30808,#30809),(#30810,#30811,#30812,#30813,#30814,#30815,#30816,
#30817),(#30818,#30819,#30820,#30821,#30822,#30823,#30824,#30825),(#30826,
#30827,#30828,#30829,#30830,#30831,#30832,#30833),(#30834,#30835,#30836,
#30837,#30838,#30839,#30840,#30841),(#30842,#30843,#30844,#30845,#30846,
#30847,#30848,#30849)),.UNSPECIFIED.,.F.,.F.,.F.,(4,2,4),(4,2,2,4),(0.,
0.5,1.),(0.,0.25,0.5,1.),.UNSPECIFIED.);
#236=B_SPLINE_SURFACE_WITH_KNOTS('',3,3,((#30873,#30874,#30875,#30876,#30877,
#30878,#30879,#30880),(#30881,#30882,#30883,#30884,#30885,#30886,#30887,
#30888),(#30889,#30890,#30891,#30892,#30893,#30894,#30895,#30896),(#30897,
#30898,#30899,#30900,#30901,#30902,#30903,#30904),(#30905,#30906,#30907,
#30908,#30909,#30910,#30911,#30912),(#30913,#30914,#30915,#30916,#30917,
#30918,#30919,#30920),(#30921,#30922,#30923,#30924,#30925,#30926,#30927,
#30928),(#30929,#30930,#30931,#30932,#30933,#30934,#30935,#30936)),
 .UNSPECIFIED.,.F.,.F.,.F.,(4,2,2,4),(4,2,2,4),(0.,0.25,0.5,1.),(0.,0.25,
0.5,1.),.UNSPECIFIED.);
#237=B_SPLINE_SURFACE_WITH_KNOTS('',3,3,((#31005,#31006,#31007,#31008,#31009,
#31010),(#31011,#31012,#31013,#31014,#31015,#31016),(#31017,#31018,#31019,
#31020,#31021,#31022),(#31023,#31024,#31025,#31026,#31027,#31028),(#31029,
#31030,#31031,#31032,#31033,#31034),(#31035,#31036,#31037,#31038,#31039,
#31040),(#31041,#31042,#31043,#31044,#31045,#31046),(#31047,#31048,#31049,
#31050,#31051,#31052),(#31053,#31054,#31055,#31056,#31057,#31058),(#31059,
#31060,#31061,#31062,#31063,#31064)),.UNSPECIFIED.,.F.,.F.,.F.,(4,2,2,2,
4),(4,2,4),(0.,0.25,0.5,0.75,1.),(0.,0.5,1.),.UNSPECIFIED.);
#238=B_SPLINE_SURFACE_WITH_KNOTS('',3,3,((#31072,#31073,#31074,#31075,#31076,
#31077,#31078,#31079,#31080,#31081),(#31082,#31083,#31084,#31085,#31086,
#31087,#31088,#31089,#31090,#31091),(#31092,#31093,#31094,#31095,#31096,
#31097,#31098,#31099,#31100,#31101),(#31102,#31103,#31104,#31105,#31106,
#31107,#31108,#31109,#31110,#31111),(#31112,#31113,#31114,#31115,#31116,
#31117,#31118,#31119,#31120,#31121),(#31122,#31123,#31124,#31125,#31126,
#31127,#31128,#31129,#31130,#31131)),.UNSPECIFIED.,.F.,.F.,.F.,(4,2,4),
(4,2,2,2,4),(0.,0.5,1.),(0.,0.25,0.5,0.75,1.),.UNSPECIFIED.);
#239=B_SPLINE_SURFACE_WITH_KNOTS('',3,3,((#31286,#31287,#31288,#31289,#31290,
#31291,#31292,#31293),(#31294,#31295,#31296,#31297,#31298,#31299,#31300,
#31301),(#31302,#31303,#31304,#31305,#31306,#31307,#31308,#31309),(#31310,
#31311,#31312,#31313,#31314,#31315,#31316,#31317),(#31318,#31319,#31320,
#31321,#31322,#31323,#31324,#31325),(#31326,#31327,#31328,#31329,#31330,
#31331,#31332,#31333),(#31334,#31335,#31336,#31337,#31338,#31339,#31340,
#31341),(#31342,#31343,#31344,#31345,#31346,#31347,#31348,#31349)),
 .UNSPECIFIED.,.F.,.F.,.F.,(4,2,2,4),(4,2,2,4),(0.,0.25,0.5,1.),(0.,0.25,
0.5,1.),.UNSPECIFIED.);
#240=B_SPLINE_SURFACE_WITH_KNOTS('',3,3,((#31663,#31664,#31665,#31666,#31667,
#31668),(#31669,#31670,#31671,#31672,#31673,#31674),(#31675,#31676,#31677,
#31678,#31679,#31680),(#31681,#31682,#31683,#31684,#31685,#31686),(#31687,
#31688,#31689,#31690,#31691,#31692),(#31693,#31694,#31695,#31696,#31697,
#31698),(#31699,#31700,#31701,#31702,#31703,#31704),(#31705,#31706,#31707,
#31708,#31709,#31710),(#31711,#31712,#31713,#31714,#31715,#31716),(#31717,
#31718,#31719,#31720,#31721,#31722)),.UNSPECIFIED.,.F.,.F.,.F.,(4,2,2,2,
4),(4,2,4),(0.,0.25,0.5,0.75,1.),(0.,0.5,1.),.UNSPECIFIED.);
#241=B_SPLINE_SURFACE_WITH_KNOTS('',3,3,((#31724,#31725,#31726,#31727,#31728,
#31729,#31730,#31731),(#31732,#31733,#31734,#31735,#31736,#31737,#31738,
#31739),(#31740,#31741,#31742,#31743,#31744,#31745,#31746,#31747),(#31748,
#31749,#31750,#31751,#31752,#31753,#31754,#31755),(#31756,#31757,#31758,
#31759,#31760,#31761,#31762,#31763),(#31764,#31765,#31766,#31767,#31768,
#31769,#31770,#31771),(#31772,#31773,#31774,#31775,#31776,#31777,#31778,
#31779),(#31780,#31781,#31782,#31783,#31784,#31785,#31786,#31787)),
 .UNSPECIFIED.,.F.,.F.,.F.,(4,2,2,4),(4,2,2,4),(0.,0.25,0.5,1.),(0.,0.25,
0.5,1.),.UNSPECIFIED.);
#242=B_SPLINE_SURFACE_WITH_KNOTS('',3,3,((#31930,#31931,#31932,#31933,#31934,
#31935),(#31936,#31937,#31938,#31939,#31940,#31941),(#31942,#31943,#31944,
#31945,#31946,#31947),(#31948,#31949,#31950,#31951,#31952,#31953),(#31954,
#31955,#31956,#31957,#31958,#31959),(#31960,#31961,#31962,#31963,#31964,
#31965),(#31966,#31967,#31968,#31969,#31970,#31971),(#31972,#31973,#31974,
#31975,#31976,#31977)),.UNSPECIFIED.,.F.,.F.,.F.,(4,2,2,4),(4,2,4),(0.,
0.25,0.5,1.),(0.,0.5,1.),.UNSPECIFIED.);
#264=ELLIPSE('',#11887,72.7371534489403,59.3518142583655);
#265=ELLIPSE('',#11888,72.7371534278831,59.3518142500034);
#266=ELLIPSE('',#11890,72.7371534418997,59.3518142555308);
#267=ELLIPSE('',#11891,72.7371534042391,59.3518142403299);
#268=ELLIPSE('',#11893,72.7371534315122,59.3518142517928);
#269=ELLIPSE('',#11894,72.7371534760386,59.3518142697471);
#270=ELLIPSE('',#11896,72.7371534484564,59.3518142581681);
#271=ELLIPSE('',#11897,72.7371534338909,59.351814252458);
#272=ELLIPSE('',#11900,267.033279968916,3.97556846403247);
#273=ELLIPSE('',#11988,72.7371534233152,59.3518142481207);
#274=ELLIPSE('',#11989,72.7371534254535,59.3518142493252);
#275=ELLIPSE('',#11991,72.7371534314927,59.3518142515694);
#276=ELLIPSE('',#11992,72.7371534149343,59.351814244469);
#277=ELLIPSE('',#12027,267.033273104505,3.97556839267334);
#278=ELLIPSE('',#12068,72.7371534238836,59.3518142483897);
#279=ELLIPSE('',#12069,72.737153424688,59.3518142489889);
#280=ELLIPSE('',#12102,267.033281117203,3.97556847604632);
#281=ELLIPSE('',#12131,72.7371533930096,59.3518142357707);
#282=ELLIPSE('',#12132,72.7371534556984,59.3518142616426);
#283=ELLIPSE('',#12166,267.033271548161,3.97556837688584);
#284=FACE_BOUND('',#1832,.T.);
#285=FACE_BOUND('',#1833,.T.);
#286=FACE_BOUND('',#1834,.T.);
#287=FACE_BOUND('',#1835,.T.);
#288=FACE_BOUND('',#1836,.T.);
#289=FACE_BOUND('',#1837,.T.);
#290=FACE_BOUND('',#1838,.T.);
#291=FACE_BOUND('',#1839,.T.);
#292=FACE_BOUND('',#1843,.T.);
#293=FACE_BOUND('',#1845,.T.);
#294=FACE_BOUND('',#1857,.T.);
#295=FACE_BOUND('',#1873,.T.);
#296=FACE_BOUND('',#1875,.T.);
#297=FACE_BOUND('',#1882,.T.);
#298=FACE_BOUND('',#1883,.T.);
#299=FACE_BOUND('',#1884,.T.);
#300=FACE_BOUND('',#1885,.T.);
#301=FACE_BOUND('',#1886,.T.);
#302=FACE_BOUND('',#1887,.T.);
#303=FACE_BOUND('',#1888,.T.);
#304=FACE_BOUND('',#1889,.T.);
#305=FACE_BOUND('',#1915,.T.);
#306=FACE_BOUND('',#1917,.T.);
#307=FACE_BOUND('',#1969,.T.);
#308=FACE_BOUND('',#1971,.T.);
#309=FACE_BOUND('',#2471,.T.);
#310=FACE_BOUND('',#2473,.T.);
#311=FACE_BOUND('',#2475,.T.);
#315=PLANE('',#11821);
#316=PLANE('',#11848);
#317=PLANE('',#11849);
#318=PLANE('',#11850);
#319=PLANE('',#11855);
#320=PLANE('',#11859);
#321=PLANE('',#11876);
#322=PLANE('',#11883);
#323=PLANE('',#11886);
#324=PLANE('',#11889);
#325=PLANE('',#11892);
#326=PLANE('',#11895);
#327=PLANE('',#11904);
#328=PLANE('',#11918);
#329=PLANE('',#11920);
#330=PLANE('',#11945);
#331=PLANE('',#11949);
#332=PLANE('',#11954);
#333=PLANE('',#11955);
#334=PLANE('',#11959);
#335=PLANE('',#11960);
#336=PLANE('',#11961);
#337=PLANE('',#11987);
#338=PLANE('',#11990);
#339=PLANE('',#11993);
#340=PLANE('',#11994);
#341=PLANE('',#11998);
#342=PLANE('',#12001);
#343=PLANE('',#12002);
#344=PLANE('',#12005);
#345=PLANE('',#12009);
#346=PLANE('',#12010);
#347=PLANE('',#12011);
#348=PLANE('',#12031);
#349=PLANE('',#12033);
#350=PLANE('',#12047);
#351=PLANE('',#12051);
#352=PLANE('',#12056);
#353=PLANE('',#12060);
#354=PLANE('',#12067);
#355=PLANE('',#12070);
#356=PLANE('',#12071);
#357=PLANE('',#12075);
#358=PLANE('',#12078);
#359=PLANE('',#12079);
#360=PLANE('',#12082);
#361=PLANE('',#12086);
#362=PLANE('',#12087);
#363=PLANE('',#12088);
#364=PLANE('',#12106);
#365=PLANE('',#12108);
#366=PLANE('',#12119);
#367=PLANE('',#12123);
#368=PLANE('',#12130);
#369=PLANE('',#12133);
#370=PLANE('',#12134);
#371=PLANE('',#12138);
#372=PLANE('',#12141);
#373=PLANE('',#12142);
#374=PLANE('',#12145);
#375=PLANE('',#12149);
#376=PLANE('',#12150);
#377=PLANE('',#12151);
#378=PLANE('',#12170);
#379=PLANE('',#12172);
#380=PLANE('',#12179);
#381=PLANE('',#12184);
#382=PLANE('',#12197);
#383=PLANE('',#12198);
#384=PLANE('',#12202);
#385=PLANE('',#12205);
#386=PLANE('',#12206);
#387=PLANE('',#12209);
#388=PLANE('',#12213);
#389=PLANE('',#12214);
#390=PLANE('',#12215);
#391=PLANE('',#12926);
#392=PLANE('',#12927);
#393=PLANE('',#12929);
#394=PLANE('',#12930);
#395=PLANE('',#12931);
#396=PLANE('',#12932);
#397=PLANE('',#12933);
#398=PLANE('',#12934);
#399=PLANE('',#12935);
#400=PLANE('',#12936);
#401=PLANE('',#12937);
#402=PLANE('',#12938);
#403=PLANE('',#12939);
#404=PLANE('',#12940);
#405=PLANE('',#12941);
#406=PLANE('',#12942);
#407=PLANE('',#12943);
#408=PLANE('',#12944);
#409=PLANE('',#12945);
#410=PLANE('',#12946);
#411=PLANE('',#12947);
#412=PLANE('',#12948);
#413=PLANE('',#12949);
#419=B_SPLINE_CURVE_WITH_KNOTS('',3,(#16807,#16808,#16809,#16810,#16811,
#16812,#16813,#16814),.UNSPECIFIED.,.F.,.F.,(4,2,2,4),(0.,0.000625000000000717,
0.00312500000008064,0.00654794813346023),.UNSPECIFIED.);
#420=B_SPLINE_CURVE_WITH_KNOTS('',3,(#16818,#16819,#16820,#16821,#16822,
#16823,#16824,#16825,#16826,#16827),.UNSPECIFIED.,.F.,.F.,(4,2,2,2,4),(0.,
0.0110943326857293,0.016641499028594,0.0194150822000263,0.0221886653714586),
 .UNSPECIFIED.);
#421=B_SPLINE_CURVE_WITH_KNOTS('',3,(#16829,#16830,#16831,#16832,#16833,
#16834,#16835,#16836,#16837,#16838),.UNSPECIFIED.,.F.,.F.,(4,2,2,2,4),(0.0221886653714586,
0.0332305757457702,0.0359910533393481,0.038751530932926,0.0442724861200818),
 .UNSPECIFIED.);
#422=B_SPLINE_CURVE_WITH_KNOTS('',3,(#16841,#16842,#16843,#16844,#16845,
#16846,#16847,#16848),.UNSPECIFIED.,.F.,.F.,(4,2,2,4),(1.30968750346023E-17,
0.000625000000000436,0.00312500000006035,0.0065479481334553),
 .UNSPECIFIED.);
#423=B_SPLINE_CURVE_WITH_KNOTS('',3,(#16876,#16877,#16878,#16879,#16880,
#16881,#16882,#16883),.UNSPECIFIED.,.F.,.F.,(4,2,2,4),(0.,0.000625000000000718,
0.00312500000008064,0.00654794813346023),.UNSPECIFIED.);
#424=B_SPLINE_CURVE_WITH_KNOTS('',3,(#16887,#16888,#16889,#16890,#16891,
#16892,#16893,#16894,#16895,#16896),.UNSPECIFIED.,.F.,.F.,(4,2,2,2,4),(0.,
0.0110943326857293,0.016641499028594,0.0194150822000263,0.0221886653714587),
 .UNSPECIFIED.);
#425=B_SPLINE_CURVE_WITH_KNOTS('',3,(#16898,#16899,#16900,#16901,#16902,
#16903,#16904,#16905,#16906,#16907),.UNSPECIFIED.,.F.,.F.,(4,2,2,2,4),(0.0221886653714587,
0.0332305757457703,0.0359910533393482,0.0387515309329261,0.0442724861200819),
 .UNSPECIFIED.);
#426=B_SPLINE_CURVE_WITH_KNOTS('',3,(#16910,#16911,#16912,#16913,#16914,
#16915,#16916,#16917),.UNSPECIFIED.,.F.,.F.,(4,2,2,4),(1.7347234759768E-18,
0.000625000000000437,0.00312500000006035,0.00654794813345528),
 .UNSPECIFIED.);
#427=B_SPLINE_CURVE_WITH_KNOTS('',3,(#16951,#16952,#16953,#16954,#16955,
#16956,#16957,#16958,#16959,#16960,#16961,#16962,#16963,#16964,#16965,#16966,
#16967,#16968,#16969,#16970,#16971,#16972,#16973,#16974,#16975,#16976,#16977,
#16978,#16979,#16980,#16981,#16982,#16983,#16984,#16985,#16986,#16987,#16988,
#16989,#16990,#16991,#16992,#16993,#16994,#16995,#16996),.UNSPECIFIED.,
 .F.,.F.,(4,3,3,3,3,3,3,3,3,3,3,3,3,3,3,4),(0.,6.08280066317253E-5,0.000143504025129764,
0.000222132236425273,0.000243312026526901,0.000273726029842764,0.000390756960305233,
0.000486624053053802,0.000487092885051584,0.000652104140181452,0.000729936079580703,
0.000730491914653075,0.000807330947238038,0.000884197975618414,0.000957724799089441,
0.000973248106107605),.UNSPECIFIED.);
#428=B_SPLINE_CURVE_WITH_KNOTS('',3,(#17004,#17005,#17006,#17007,#17008,
#17009,#17010,#17011,#17012,#17013,#17014,#17015,#17016,#17017,#17018,#17019,
#17020,#17021,#17022,#17023,#17024,#17025,#17026,#17027,#17028,#17029,#17030,
#17031,#17032,#17033,#17034),.UNSPECIFIED.,.F.,.F.,(4,3,3,3,3,3,3,3,3,3,
4),(0.,0.000110044300705118,0.000227537679381867,0.000345953766308564,0.000459500393964181,
0.000506968361890626,0.000507607986069998,0.000621724537891899,0.000763599672892467,
0.000889140904463126,0.00101393672378125),.UNSPECIFIED.);
#429=B_SPLINE_CURVE_WITH_KNOTS('',3,(#17038,#17039,#17040,#17041,#17042,
#17043,#17044,#17045,#17046,#17047,#17048,#17049,#17050,#17051,#17052,#17053,
#17054,#17055,#17056,#17057,#17058,#17059,#17060,#17061,#17062,#17063,#17064,
#17065,#17066,#17067,#17068,#17069,#17070,#17071),.UNSPECIFIED.,.F.,.F.,
(4,3,3,3,3,3,3,3,3,3,3,4),(0.,9.75727287245357E-5,0.000197558568026697,
0.000263369830764718,0.000264501976385977,0.000410751214877331,0.000527720220099539,
0.000529003952771953,0.000711275183632117,0.000792685220207556,0.000986383339260414,
0.0010580079055439),.UNSPECIFIED.);
#430=B_SPLINE_CURVE_WITH_KNOTS('',3,(#17076,#17077,#17078,#17079,#17080,
#17081,#17082,#17083,#17084,#17085,#17086,#17087,#17088,#17089,#17090,#17091,
#17092,#17093,#17094,#17095,#17096,#17097,#17098,#17099,#17100,#17101,#17102,
#17103,#17104,#17105,#17106,#17107,#17108,#17109,#17110,#17111,#17112,#17113,
#17114,#17115,#17116,#17117,#17118),.UNSPECIFIED.,.F.,.F.,(4,3,3,3,3,3,
3,3,3,3,3,3,3,3,4),(0.,0.000122774773559688,0.000252172289553419,0.000391124229753653,
0.000417443869709968,0.000418563871648259,0.000739329890793104,0.000834887739419937,
0.000836592389993165,0.00109817436603959,0.0012523316091299,0.00125385075554294,
0.0014203606660688,0.0015569180076674,0.00166977547883987),
 .UNSPECIFIED.);
#431=B_SPLINE_CURVE_WITH_KNOTS('',3,(#17128,#17129,#17130,#17131,#17132,
#17133,#17134,#17135,#17136,#17137,#17138,#17139,#17140,#17141,#17142,#17143,
#17144,#17145,#17146,#17147,#17148,#17149,#17150,#17151,#17152,#17153,#17154,
#17155,#17156,#17157,#17158,#17159,#17160,#17161,#17162,#17163,#17164,#17165,
#17166,#17167,#17168,#17169,#17170,#17171,#17172,#17173),.UNSPECIFIED.,
 .F.,.F.,(4,3,3,3,3,3,3,3,3,3,3,3,3,3,3,4),(0.,6.0828006631726E-5,0.000143504025135297,
0.000222132236434781,0.000243312026526904,0.000273726029842767,0.000390756960268089,
0.000486624053053808,0.000487092885051566,0.000652104140206423,0.000729936079580712,
0.000730491914653054,0.000807330947229213,0.000884197975603245,0.000957724799069373,
0.000973248106107616),.UNSPECIFIED.);
#432=B_SPLINE_CURVE_WITH_KNOTS('',3,(#17178,#17179,#17180,#17181,#17182,
#17183,#17184,#17185,#17186,#17187,#17188,#17189,#17190,#17191,#17192,#17193,
#17194,#17195,#17196,#17197,#17198,#17199,#17200,#17201,#17202,#17203,#17204,
#17205,#17206,#17207,#17208),.UNSPECIFIED.,.F.,.F.,(4,3,3,3,3,3,3,3,3,3,
4),(0.,0.000110044300698099,0.000227537679367299,0.00034595376628619,0.000459500393933875,
0.000506968361890626,0.000507607986070002,0.000621724537891888,0.00076359967287861,
0.000889140904441178,0.00101393672378125),.UNSPECIFIED.);
#433=B_SPLINE_CURVE_WITH_KNOTS('',3,(#17212,#17213,#17214,#17215,#17216,
#17217,#17218,#17219,#17220,#17221,#17222,#17223,#17224,#17225,#17226,#17227,
#17228,#17229,#17230,#17231,#17232,#17233,#17234,#17235,#17236,#17237,#17238,
#17239,#17240,#17241,#17242,#17243,#17244,#17245),.UNSPECIFIED.,.F.,.F.,
(4,3,3,3,3,3,3,3,3,3,3,4),(0.,9.7572728723403E-5,0.000197558568027757,0.000263369830764721,
0.000264501976385979,0.000410751214966632,0.000527720220099549,0.000529003952771959,
0.000711275183702182,0.000792685220207923,0.000986383339293457,0.00105800790554391),
 .UNSPECIFIED.);
#434=B_SPLINE_CURVE_WITH_KNOTS('',3,(#17253,#17254,#17255,#17256,#17257,
#17258,#17259,#17260,#17261,#17262,#17263,#17264,#17265,#17266,#17267,#17268,
#17269,#17270,#17271,#17272,#17273,#17274,#17275,#17276,#17277,#17278,#17279,
#17280,#17281,#17282,#17283,#17284,#17285,#17286,#17287,#17288,#17289,#17290,
#17291,#17292,#17293,#17294,#17295),.UNSPECIFIED.,.F.,.F.,(4,3,3,3,3,3,
3,3,3,3,3,3,3,3,4),(0.,0.000122774773565863,0.000252172289565749,0.000391124229768784,
0.000417443869709969,0.000418563871648259,0.000739329889542507,0.000834887739419938,
0.000836592389993165,0.00109817436553555,0.00125233160912991,0.00125385075554295,
0.00142036066599669,0.00155691800753188,0.00166977547883988),
 .UNSPECIFIED.);
#435=B_SPLINE_CURVE_WITH_KNOTS('',3,(#17305,#17306,#17307,#17308,#17309,
#17310,#17311,#17312,#17313,#17314,#17315,#17316,#17317,#17318,#17319,#17320,
#17321,#17322,#17323,#17324,#17325,#17326,#17327,#17328,#17329,#17330,#17331,
#17332,#17333,#17334,#17335,#17336,#17337,#17338,#17339,#17340,#17341,#17342,
#17343,#17344,#17345,#17346,#17347,#17348,#17349,#17350),.UNSPECIFIED.,
 .F.,.F.,(4,3,3,3,3,3,3,3,3,3,3,3,3,3,3,4),(0.,6.08280066317263E-5,0.000143504025126593,
0.000222132236418946,0.000243312026526905,0.000273726029842769,0.000390756960322061,
0.000486624053053811,0.000487092885051591,0.000652104140237346,0.000729936079580716,
0.000730491914653081,0.000807330947238143,0.000884197975617686,0.000957724799086867,
0.000973248106107622),.UNSPECIFIED.);
#436=B_SPLINE_CURVE_WITH_KNOTS('',3,(#17358,#17359,#17360,#17361,#17362,
#17363,#17364,#17365,#17366,#17367,#17368,#17369,#17370,#17371,#17372,#17373,
#17374,#17375,#17376,#17377,#17378,#17379,#17380,#17381,#17382,#17383,#17384,
#17385,#17386,#17387,#17388),.UNSPECIFIED.,.F.,.F.,(4,3,3,3,3,3,3,3,3,3,
4),(0.,0.000110044300710652,0.00022753767939358,0.000345953766326745,0.000459500393988843,
0.000506968361890628,0.000507607986070015,0.000621724537891887,0.000763599672912397,
0.000889140904505298,0.00101393672378126),.UNSPECIFIED.);
#437=B_SPLINE_CURVE_WITH_KNOTS('',3,(#17391,#17392,#17393,#17394,#17395,
#17396,#17397,#17398,#17399,#17400,#17401,#17402,#17403,#17404,#17405,#17406,
#17407,#17408,#17409,#17410,#17411,#17412,#17413,#17414,#17415,#17416,#17417,
#17418,#17419,#17420,#17421,#17422,#17423,#17424),.UNSPECIFIED.,.F.,.F.,
(4,3,3,3,3,3,3,3,3,3,3,4),(0.,9.75727287165792E-5,0.000197558568020339,
0.000263369830764727,0.000264501976385978,0.000410751214991148,0.000527720220099542,
0.000529003952771956,0.000711275183778258,0.000792685220207718,0.000986383339389978,
0.0010580079055439),.UNSPECIFIED.);
#438=B_SPLINE_CURVE_WITH_KNOTS('',3,(#17430,#17431,#17432,#17433,#17434,
#17435,#17436,#17437,#17438,#17439,#17440,#17441,#17442,#17443,#17444,#17445,
#17446,#17447,#17448,#17449,#17450,#17451,#17452,#17453,#17454,#17455,#17456,
#17457,#17458,#17459,#17460,#17461,#17462,#17463,#17464,#17465,#17466,#17467,
#17468,#17469,#17470,#17471,#17472),.UNSPECIFIED.,.F.,.F.,(4,3,3,3,3,3,
3,3,3,3,3,3,3,3,4),(0.,0.000122774773560884,0.000252172289555377,0.000391124229755383,
0.000417443869709971,0.000418563871648265,0.000739329890771365,0.000834887739419941,
0.000836592389993166,0.00109817436572929,0.00125233160912991,0.00125385075554294,
0.00142036066608084,0.00155691800768044,0.00166977547883988),
 .UNSPECIFIED.);
#439=B_SPLINE_CURVE_WITH_KNOTS('',3,(#17481,#17482,#17483,#17484,#17485,
#17486,#17487,#17488,#17489,#17490,#17491,#17492,#17493,#17494,#17495,#17496,
#17497,#17498,#17499,#17500,#17501,#17502,#17503,#17504,#17505,#17506,#17507,
#17508,#17509,#17510,#17511,#17512,#17513,#17514,#17515,#17516,#17517,#17518,
#17519,#17520,#17521,#17522,#17523,#17524,#17525,#17526),.UNSPECIFIED.,
 .F.,.F.,(4,3,3,3,3,3,3,3,3,3,3,3,3,3,3,4),(0.,6.08280066317253E-5,0.000143504025133277,
0.000222132236430928,0.000243312026526901,0.000273726029842764,0.000390756960290358,
0.000486624053053802,0.000487092885051583,0.000652104140099763,0.000729936079580704,
0.000730491914653072,0.000807330947240576,0.000884197975626852,0.000957724799105996,
0.000973248106107605),.UNSPECIFIED.);
#440=B_SPLINE_CURVE_WITH_KNOTS('',3,(#17532,#17533,#17534,#17535,#17536,
#17537,#17538,#17539,#17540,#17541,#17542,#17543,#17544,#17545,#17546,#17547,
#17548,#17549,#17550,#17551,#17552,#17553,#17554,#17555,#17556,#17557,#17558,
#17559,#17560,#17561,#17562),.UNSPECIFIED.,.F.,.F.,(4,3,3,3,3,3,3,3,3,3,
4),(0.,0.000110044300698132,0.000227537679367395,0.000345953766286372,0.000459500393934088,
0.000506968361890626,0.000507607986070008,0.0006217245378919,0.000763599672881826,
0.000889140904448288,0.00101393672378125),.UNSPECIFIED.);
#441=B_SPLINE_CURVE_WITH_KNOTS('',3,(#17566,#17567,#17568,#17569,#17570,
#17571,#17572,#17573,#17574,#17575,#17576,#17577,#17578,#17579,#17580,#17581,
#17582,#17583,#17584,#17585,#17586,#17587,#17588,#17589,#17590,#17591,#17592,
#17593,#17594,#17595,#17596,#17597,#17598,#17599),.UNSPECIFIED.,.F.,.F.,
(4,3,3,3,3,3,3,3,3,3,3,4),(0.,9.75727287258748E-5,0.000197558568032606,
0.000263369830764718,0.000264501976385979,0.000410751215061321,0.000527720220099554,
0.000529003952771959,0.000711275183839031,0.000792685220207918,0.000986383339454815,
0.00105800790554391),.UNSPECIFIED.);
#442=B_SPLINE_CURVE_WITH_KNOTS('',3,(#17607,#17608,#17609,#17610,#17611,
#17612,#17613,#17614,#17615,#17616,#17617,#17618,#17619,#17620,#17621,#17622,
#17623,#17624,#17625,#17626,#17627,#17628,#17629,#17630,#17631,#17632,#17633,
#17634,#17635,#17636,#17637,#17638,#17639,#17640,#17641,#17642,#17643,#17644,
#17645,#17646,#17647,#17648,#17649),.UNSPECIFIED.,.F.,.F.,(4,3,3,3,3,3,
3,3,3,3,3,3,3,3,4),(0.,0.000122774773571519,0.000252172289575277,0.000391124229778881,
0.000417443869709969,0.000418563871648264,0.000739329890508021,0.000834887739419938,
0.000836592389993168,0.0010981743657467,0.00125233160912991,0.00125385075554294,
0.00142036066604611,0.00155691800761702,0.00166977547883988),
 .UNSPECIFIED.);
#443=B_SPLINE_CURVE_WITH_KNOTS('',3,(#17673,#17674,#17675,#17676,#17677,
#17678,#17679,#17680),.UNSPECIFIED.,.F.,.F.,(4,2,2,4),(0.,0.00062500000000072,
0.00312500000008065,0.00654794813346023),.UNSPECIFIED.);
#444=B_SPLINE_CURVE_WITH_KNOTS('',3,(#17684,#17685,#17686,#17687,#17688,
#17689,#17690,#17691,#17692,#17693),.UNSPECIFIED.,.F.,.F.,(4,2,2,2,4),(0.,
0.0110943326857293,0.016641499028594,0.0194150822000263,0.0221886653714587),
 .UNSPECIFIED.);
#445=B_SPLINE_CURVE_WITH_KNOTS('',3,(#17695,#17696,#17697,#17698,#17699,
#17700,#17701,#17702,#17703,#17704),.UNSPECIFIED.,.F.,.F.,(4,2,2,2,4),(0.0221886653714587,
0.0332305757457702,0.0359910533393481,0.038751530932926,0.0442724861200819),
 .UNSPECIFIED.);
#446=B_SPLINE_CURVE_WITH_KNOTS('',3,(#17707,#17708,#17709,#17710,#17711,
#17712,#17713,#17714),.UNSPECIFIED.,.F.,.F.,(4,2,2,4),(1.30968750346023E-17,
0.000625000000000436,0.00312500000006035,0.0065479481334553),
 .UNSPECIFIED.);
#447=B_SPLINE_CURVE_WITH_KNOTS('',3,(#17807,#17808,#17809,#17810,#17811,
#17812,#17813,#17814),.UNSPECIFIED.,.F.,.F.,(4,2,2,4),(0.,0.000324140863782348,
0.000648281727564695,0.00129656345512939),.UNSPECIFIED.);
#448=B_SPLINE_CURVE_WITH_KNOTS('',3,(#17818,#17819,#17820,#17821,#17822,
#17823,#17824,#17825),.UNSPECIFIED.,.F.,.F.,(4,2,2,4),(0.,0.000642153724747558,
0.000963230587121339,0.00128430744949512),.UNSPECIFIED.);
#449=B_SPLINE_CURVE_WITH_KNOTS('',3,(#17829,#17830,#17831,#17832,#17833,
#17834,#17835,#17836,#17837,#17838,#17839,#17840,#17841,#17842,#17843,#17844,
#17845,#17846,#17847),.UNSPECIFIED.,.F.,.F.,(4,3,3,3,3,3,4),(0.,0.000195874855531394,
0.000407633432445313,0.000642628402010786,0.000643366204945988,0.00124146542702823,
0.00128673240989198),.UNSPECIFIED.);
#450=B_SPLINE_CURVE_WITH_KNOTS('',3,(#17851,#17852,#17853,#17854,#17855,
#17856,#17857,#17858,#17859,#17860,#17861,#17862,#17863,#17864,#17865,#17866,
#17867,#17868,#17869),.UNSPECIFIED.,.F.,.F.,(4,3,3,3,3,3,4),(0.,0.000446723853990593,
0.000644054549895828,0.000644233932867389,0.000966350899301084,0.00120471562689313,
0.00128846786573478),.UNSPECIFIED.);
#451=B_SPLINE_CURVE_WITH_KNOTS('',3,(#17873,#17874,#17875,#17876,#17877,
#17878,#17879,#17880,#17881,#17882,#17883,#17884,#17885,#17886,#17887,#17888,
#17889,#17890,#17891),.UNSPECIFIED.,.F.,.F.,(4,3,3,3,3,3,4),(0.,0.000198161496041495,
0.000412566761351645,0.000642956139405752,0.000643725422538401,0.00123968599593009,
0.0012874508450768),.UNSPECIFIED.);
#452=B_SPLINE_CURVE_WITH_KNOTS('',3,(#17895,#17896,#17897,#17898,#17899,
#17900,#17901,#17902),.UNSPECIFIED.,.F.,.F.,(4,2,2,4),(0.,0.000642153724747562,
0.000963230587121341,0.00128430744949512),.UNSPECIFIED.);
#453=B_SPLINE_CURVE_WITH_KNOTS('',3,(#17906,#17907,#17908,#17909,#17910,
#17911,#17912,#17913,#17914,#17915,#17916,#17917,#17918,#17919,#17920,#17921,
#17922,#17923,#17924),.UNSPECIFIED.,.F.,.F.,(4,3,3,3,3,3,4),(0.,0.000195874855548819,
0.000407633432483008,0.000642628402010788,0.000643366204945996,0.00124146543005707,
0.00128673240989199),.UNSPECIFIED.);
#454=B_SPLINE_CURVE_WITH_KNOTS('',3,(#17928,#17929,#17930,#17931,#17932,
#17933,#17934,#17935,#17936,#17937,#17938,#17939,#17940,#17941,#17942,#17943,
#17944,#17945,#17946),.UNSPECIFIED.,.F.,.F.,(4,3,3,3,3,3,4),(0.,0.000501649919473043,
0.000643648102817533,0.000643900482232717,0.000965850723349075,0.00120614192088348,
0.00128780096446543),.UNSPECIFIED.);
#455=B_SPLINE_CURVE_WITH_KNOTS('',3,(#18100,#18101,#18102,#18103,#18104,
#18105,#18106,#18107,#18108,#18109,#18110,#18111,#18112,#18113,#18114,#18115,
#18116,#18117,#18118,#18119,#18120,#18121,#18122,#18123,#18124,#18125,#18126,
#18127,#18128,#18129,#18130),.UNSPECIFIED.,.F.,.F.,(4,3,3,3,3,3,3,3,3,3,
4),(0.00423087891556426,0.013713375686686,0.0177375823121115,0.0182590193856104,
0.020118220117775,0.0211142581612483,0.0218072955502234,0.0244909340103851,
0.0253408764930824,0.0282925811008705,0.0312442857086587),.UNSPECIFIED.);
#456=B_SPLINE_CURVE_WITH_KNOTS('',3,(#18133,#18134,#18135,#18136,#18137,
#18138,#18139,#18140,#18141,#18142,#18143,#18144,#18145,#18146,#18147,#18148,
#18149,#18150,#18151,#18152,#18153,#18154,#18155,#18156,#18157,#18158,#18159,
#18160,#18161,#18162,#18163,#18164,#18165,#18166,#18167,#18168,#18169),
 .UNSPECIFIED.,.F.,.F.,(4,3,3,3,3,3,3,3,3,3,3,3,4),(0.,0.00293383627619356,
0.00586767255238711,0.00671399432426571,0.00908462661832189,0.00938017817101472,
0.0100709914863986,0.0117876962259593,0.0129061418604891,0.0134279886485314,
0.0185395617742769,0.0234677093302294,0.0268559772970629),.UNSPECIFIED.);
#457=B_SPLINE_CURVE_WITH_KNOTS('',3,(#18177,#18178,#18179,#18180,#18181,
#18182,#18183,#18184,#18185,#18186,#18187,#18188,#18189,#18190,#18191,#18192,
#18193,#18194,#18195,#18196,#18197,#18198,#18199,#18200,#18201,#18202,#18203,
#18204,#18205,#18206,#18207),.UNSPECIFIED.,.F.,.F.,(4,3,3,3,3,3,3,3,3,3,
4),(0.00423087891556413,0.0137133751566899,0.0177375823121114,0.0182590193856102,
0.0201182201175346,0.0211142581612482,0.0218072955502231,0.024490934010385,
0.0253408764930823,0.0282925811008705,0.0312442857086587),.UNSPECIFIED.);
#458=B_SPLINE_CURVE_WITH_KNOTS('',3,(#18210,#18211,#18212,#18213,#18214,
#18215,#18216,#18217,#18218,#18219,#18220,#18221,#18222,#18223,#18224,#18225,
#18226,#18227,#18228,#18229,#18230,#18231,#18232,#18233,#18234,#18235,#18236,
#18237,#18238,#18239,#18240,#18241,#18242,#18243,#18244,#18245,#18246),
 .UNSPECIFIED.,.F.,.F.,(4,3,3,3,3,3,3,3,3,3,3,3,4),(0.,0.00293383627619322,
0.00586767255238644,0.00671399432426573,0.00908462661700898,0.00938017817101484,
0.0100709914863986,0.0117876962256719,0.0129061418604892,0.0134279886485315,
0.018539561770304,0.02346770932428,0.0268559772970629),.UNSPECIFIED.);
#459=B_SPLINE_CURVE_WITH_KNOTS('',3,(#18254,#18255,#18256,#18257,#18258,
#18259,#18260,#18261,#18262,#18263,#18264,#18265,#18266,#18267,#18268,#18269,
#18270,#18271,#18272,#18273,#18274,#18275,#18276,#18277,#18278,#18279,#18280,
#18281,#18282,#18283,#18284,#18285,#18286,#18287),.UNSPECIFIED.,.F.,.F.,
(4,3,3,3,3,3,3,3,3,3,3,4),(0.0041940778674379,0.00785137044488797,0.00864322402522931,
0.00888216076442238,0.0105632172613147,0.0122879239676185,0.0130923701830207,
0.0136962196480358,0.0161859644978567,0.0187205500997639,0.0213309666493633,
0.0219906624986036),.UNSPECIFIED.);
#460=B_SPLINE_CURVE_WITH_KNOTS('',3,(#18290,#18291,#18292,#18293,#18294,
#18295,#18296,#18297,#18298,#18299,#18300,#18301,#18302,#18303,#18304,#18305,
#18306,#18307,#18308,#18309,#18310,#18311,#18312,#18313,#18314,#18315,#18316,
#18317,#18318,#18319,#18320,#18321,#18322,#18323),.UNSPECIFIED.,.F.,.F.,
(4,3,3,3,3,3,3,3,3,3,3,4),(0.,0.00259497273974606,0.00513490948945618,0.00760920564936369,
0.0083165426104236,0.00892204401521707,0.0106541774038738,0.012350736986894,
0.0131434725515692,0.0133830660228256,0.0170412668483451,0.0178440880304342),
 .UNSPECIFIED.);
#461=B_SPLINE_CURVE_WITH_KNOTS('',3,(#18331,#18332,#18333,#18334,#18335,
#18336,#18337,#18338,#18339,#18340,#18341,#18342,#18343,#18344,#18345,#18346,
#18347,#18348,#18349,#18350,#18351,#18352,#18353,#18354,#18355,#18356,#18357,
#18358,#18359,#18360,#18361),.UNSPECIFIED.,.F.,.F.,(4,3,3,3,3,3,3,3,3,3,
4),(0.00423087891556429,0.0137133753564976,0.0177375823121115,0.0182590193856104,
0.0201182201184656,0.0211142581612483,0.0218072955502225,0.0244909340103851,
0.0253408764930806,0.0282925811008696,0.0312442857086587),.UNSPECIFIED.);
#462=B_SPLINE_CURVE_WITH_KNOTS('',3,(#18364,#18365,#18366,#18367,#18368,
#18369,#18370,#18371,#18372,#18373,#18374,#18375,#18376,#18377,#18378,#18379,
#18380,#18381,#18382,#18383,#18384,#18385,#18386,#18387,#18388,#18389,#18390,
#18391,#18392,#18393,#18394,#18395,#18396,#18397,#18398,#18399,#18400),
 .UNSPECIFIED.,.F.,.F.,(4,3,3,3,3,3,3,3,3,3,3,3,4),(0.,0.00293383627619317,
0.00586767255238635,0.00671399432426571,0.0090846266183258,0.00938017817101421,
0.0100709914863986,0.0117876962251359,0.012906141860489,0.0134279886485314,
0.0185395617767228,0.0234677093338155,0.0268559772970629),.UNSPECIFIED.);
#463=B_SPLINE_CURVE_WITH_KNOTS('',3,(#18406,#18407,#18408,#18409,#18410,
#18411,#18412,#18413,#18414,#18415,#18416,#18417,#18418,#18419,#18420,#18421,
#18422,#18423,#18424,#18425,#18426,#18427,#18428,#18429,#18430,#18431,#18432,
#18433,#18434,#18435,#18436,#18437,#18438,#18439,#18440,#18441,#18442,#18443,
#18444,#18445,#18446,#18447,#18448,#18449,#18450,#18451,#18452,#18453,#18454),
 .UNSPECIFIED.,.F.,.F.,(4,3,3,3,3,3,3,3,3,3,3,3,3,3,3,3,4),(0.,0.000121245606235739,
0.000242857142540301,0.000287360877759073,0.000288270017838695,0.00044340391293331,
0.000574721755518147,0.000575971165655795,0.000665917057789352,0.000718402194397684,
0.000790242413837452,0.000826162523557336,0.00086208263327722,0.000975072145641068,
0.00100576307215676,0.00111728780497372,0.00114944351103629),
 .UNSPECIFIED.);
#464=B_SPLINE_CURVE_WITH_KNOTS('',3,(#18460,#18461,#18462,#18463,#18464,
#18465,#18466,#18467),.UNSPECIFIED.,.F.,.F.,(4,2,2,4),(0.,0.0138082473482012,
0.0207123710223017,0.0276164946964023),.UNSPECIFIED.);
#465=B_SPLINE_CURVE_WITH_KNOTS('',3,(#18525,#18526,#18527,#18528,#18529,
#18530,#18531,#18532,#18533,#18534,#18535,#18536,#18537,#18538,#18539,#18540,
#18541,#18542,#18543,#18544,#18545,#18546,#18547,#18548,#18549,#18550,#18551,
#18552,#18553,#18554,#18555,#18556,#18557,#18558),.UNSPECIFIED.,.F.,.F.,
(4,3,3,3,3,3,3,3,3,3,3,4),(0.,0.000110567770978162,0.000229163742149365,
0.000349602945021368,0.000466129197479698,0.000503962612308792,0.000504370554078785,
0.000654658246769462,0.00073377218761534,0.000861351750975835,0.000986409541182947,
0.00100874110815757),.UNSPECIFIED.);
#466=B_SPLINE_CURVE_WITH_KNOTS('',3,(#18578,#18579,#18580,#18581,#18582,
#18583,#18584,#18585,#18586,#18587,#18588,#18589,#18590,#18591,#18592,#18593,
#18594,#18595,#18596,#18597,#18598,#18599,#18600,#18601,#18602,#18603,#18604,
#18605),.UNSPECIFIED.,.F.,.F.,(4,3,3,3,3,3,3,3,3,4),(0.,9.61627041774626E-5,
0.00019464312403552,0.000263598431963766,0.00026390914929366,0.000510523427512722,
0.000527611135930377,0.00052781829858732,0.000791654292983114,0.00105563659717466),
 .UNSPECIFIED.);
#467=B_SPLINE_CURVE_WITH_KNOTS('',3,(#18611,#18612,#18613,#18614,#18615,
#18616,#18617,#18618,#18619,#18620,#18621,#18622,#18623,#18624,#18625,#18626),
 .UNSPECIFIED.,.F.,.F.,(4,3,3,3,3,4),(4.52743470429961E-15,0.00201520691454984,
0.00402253547201281,0.00602595242279557,0.00802370171969772,0.00993491157965328),
 .UNSPECIFIED.);
#468=B_SPLINE_CURVE_WITH_KNOTS('',3,(#18628,#18629,#18630,#18631,#18632,
#18633,#18634,#18635,#18636,#18637,#18638,#18639,#18640,#18641,#18642,#18643,
#18644,#18645,#18646,#18647,#18648,#18649,#18650,#18651,#18652,#18653,#18654,
#18655,#18656,#18657,#18658,#18659,#18660,#18661,#18662,#18663,#18664,#18665,
#18666,#18667,#18668,#18669,#18670),.UNSPECIFIED.,.F.,.F.,(4,3,3,3,3,3,
3,3,3,3,3,3,3,3,4),(0.,0.000142261508725732,0.000306612281624613,0.000354680426257006,
0.000354839578464806,0.000671890824680844,0.000709360852514012,0.000709794319645988,
0.000798030959078264,0.000931036118924641,0.00106404127877102,0.00117707199637736,
0.00124138149189952,0.00135612593307565,0.00141872170502802),
 .UNSPECIFIED.);
#469=B_SPLINE_CURVE_WITH_KNOTS('',3,(#18677,#18678,#18679,#18680,#18681,
#18682,#18683,#18684,#18685,#18686,#18687,#18688,#18689,#18690,#18691,#18692,
#18693,#18694,#18695,#18696,#18697,#18698,#18699,#18700,#18701,#18702,#18703,
#18704,#18705,#18706,#18707,#18708,#18709,#18710,#18711,#18712,#18713,#18714,
#18715,#18716,#18717,#18718,#18719,#18720,#18721,#18722,#18723,#18724,#18725,
#18726,#18727,#18728,#18729,#18730,#18731),.UNSPECIFIED.,.F.,.F.,(4,3,3,
3,3,3,3,3,3,3,3,3,3,3,3,3,3,3,4),(0.,0.00292798214671484,0.00577262065274856,
0.0068275614526255,0.00693335737727641,0.00947217443703029,0.0103475581420102,
0.0104000360659146,0.0118697041217895,0.0132773954669506,0.0138667147545528,
0.0138781145226839,0.0166264516367541,0.017333393443191,0.0189487413424379,
0.0205003989925137,0.0210540430942383,0.0243937363013933,0.0277334295085482),
 .UNSPECIFIED.);
#470=B_SPLINE_CURVE_WITH_KNOTS('',3,(#18735,#18736,#18737,#18738,#18739,
#18740,#18741,#18742),.UNSPECIFIED.,.F.,.F.,(4,2,2,4),(1.11076499342709E-17,
0.000625000000000437,0.00312500000006035,0.00654794813345529),
 .UNSPECIFIED.);
#471=B_SPLINE_CURVE_WITH_KNOTS('',3,(#18746,#18747,#18748,#18749,#18750,
#18751,#18752,#18753),.UNSPECIFIED.,.F.,.F.,(4,2,2,4),(0.,0.000625000000000718,
0.00312500000008064,0.00654794813346023),.UNSPECIFIED.);
#472=B_SPLINE_CURVE_WITH_KNOTS('',3,(#18757,#18758,#18759,#18760,#18761,
#18762,#18763,#18764,#18765,#18766,#18767,#18768,#18769,#18770,#18771,#18772,
#18773,#18774,#18775,#18776),.UNSPECIFIED.,.F.,.F.,(4,2,2,2,2,2,2,2,2,4),
(0.,0.00559909194960567,0.0111981838992113,0.016797275848817,0.0195968218236199,
0.0223963677984227,0.033594551697634,0.0363940976724369,0.0391936436472397,
0.0447927355968454),.UNSPECIFIED.);
#473=B_SPLINE_CURVE_WITH_KNOTS('',3,(#18801,#18802,#18803,#18804,#18805,
#18806,#18807,#18808,#18809,#18810,#18811,#18812,#18813,#18814,#18815,#18816,
#18817,#18818,#18819,#18820,#18821,#18822,#18823,#18824,#18825,#18826,#18827,
#18828),.UNSPECIFIED.,.F.,.F.,(4,3,3,3,3,3,3,3,3,4),(0.,0.00303616132428222,
0.00606003537843287,0.00872529453770153,0.00872704110520405,0.0106174542445287,
0.012537763933558,0.0144774647805997,0.0164504962233993,0.0174540822104081),
 .UNSPECIFIED.);
#474=B_SPLINE_CURVE_WITH_KNOTS('',3,(#18841,#18842,#18843,#18844,#18845,
#18846,#18847,#18848,#18849,#18850,#18851,#18852,#18853,#18854,#18855,#18856,
#18857,#18858,#18859,#18860,#18861,#18862,#18863,#18864,#18865,#18866,#18867,
#18868,#18869,#18870,#18871,#18872,#18873,#18874,#18875,#18876,#18877,#18878,
#18879,#18880),.UNSPECIFIED.,.F.,.F.,(4,3,3,3,3,3,3,3,3,3,3,3,3,4),(0.,
0.0026172239816427,0.00435913346757955,0.00436870952384852,0.00564078314582411,
0.00692512632488316,0.00818670413876967,0.00873741904769704,0.00874916468941873,
0.0122136783028643,0.0131061285715456,0.0147515701824665,0.016420240909831,
0.0174748380953941),.UNSPECIFIED.);
#475=B_SPLINE_CURVE_WITH_KNOTS('',3,(#18916,#18917,#18918,#18919,#18920,
#18921,#18922,#18923,#18924,#18925,#18926,#18927,#18928,#18929,#18930,#18931,
#18932,#18933,#18934),.UNSPECIFIED.,.F.,.F.,(4,3,3,3,3,3,4),(0.,0.000209520759761111,
0.000422285836657762,0.000553215152468023,0.00055421709622049,0.000897330597716815,
0.00110843419244098),.UNSPECIFIED.);
#476=B_SPLINE_CURVE_WITH_KNOTS('',3,(#18946,#18947,#18948,#18949,#18950,
#18951,#18952,#18953,#18954,#18955,#18956,#18957,#18958),.UNSPECIFIED.,
 .F.,.F.,(4,3,3,3,4),(0.,0.000355508868027555,0.000556947538855294,0.000557267210332349,
0.0011145344206647),.UNSPECIFIED.);
#477=B_SPLINE_CURVE_WITH_KNOTS('',3,(#18959,#18960,#18961,#18962,#18963,
#18964,#18965,#18966,#18967,#18968,#18969,#18970,#18971,#18972,#18973,#18974,
#18975,#18976,#18977,#18978,#18979,#18980,#18981,#18982,#18983,#18984,#18985,
#18986,#18987,#18988,#18989,#18990,#18991,#18992,#18993,#18994,#18995,#18996,
#18997,#18998,#18999,#19000,#19001,#19002,#19003,#19004,#19005,#19006,#19007,
#19008,#19009,#19010,#19011,#19012,#19013,#19014,#19015,#19016,#19017,#19018,
#19019,#19020,#19021,#19022,#19023,#19024,#19025),.UNSPECIFIED.,.F.,.F.,
(4,3,3,3,3,3,3,3,3,3,3,3,3,3,3,3,3,3,3,3,3,3,4),(0.,0.00277040425654158,
0.00554080851308316,0.00557505688803485,0.00791560355491117,0.0083263576942907,
0.00836258533205228,0.0100018252555059,0.011122873465018,0.0111501137760697,
0.0223002275521394,0.0223209744612517,0.0250877559961568,0.025120499376563,
0.0278752844401742,0.0279173397075124,0.0311894101771566,0.0334503413282091,
0.0334957141052527,0.0369394202827424,0.0404389072898065,0.0440271687430516,
0.0446004551042788),.UNSPECIFIED.);
#478=B_SPLINE_CURVE_WITH_KNOTS('',3,(#19033,#19034,#19035,#19036,#19037,
#19038,#19039,#19040,#19041,#19042,#19043,#19044,#19045),.UNSPECIFIED.,
 .F.,.F.,(4,3,3,3,4),(0.,0.000355508867930007,0.000556947538855285,0.000557267210332339,
0.00111453442066468),.UNSPECIFIED.);
#479=B_SPLINE_CURVE_WITH_KNOTS('',3,(#19047,#19048,#19049,#19050,#19051,
#19052,#19053,#19054,#19055,#19056,#19057,#19058,#19059,#19060,#19061,#19062,
#19063,#19064,#19065,#19066,#19067,#19068,#19069,#19070,#19071,#19072,#19073,
#19074,#19075,#19076,#19077,#19078,#19079,#19080,#19081,#19082,#19083,#19084,
#19085,#19086,#19087,#19088,#19089,#19090,#19091,#19092,#19093,#19094,#19095,
#19096,#19097,#19098,#19099,#19100,#19101,#19102,#19103,#19104,#19105,#19106,
#19107,#19108,#19109,#19110,#19111,#19112,#19113,#19114,#19115,#19116,#19117,
#19118,#19119,#19120,#19121,#19122,#19123,#19124,#19125,#19126,#19127,#19128),
 .UNSPECIFIED.,.F.,.F.,(4,3,3,3,3,3,3,3,3,3,3,3,3,3,3,3,3,3,3,3,3,3,3,3,
3,3,3,4),(0.,0.00276800820692877,0.00539608564417642,0.00553601641385754,
0.00558313544569878,0.00832024774722178,0.00837470316854816,0.0100465608585699,
0.0111128364927737,0.0111662708913976,0.016725314895809,0.0220049729595792,
0.0222843589002204,0.0223325417827951,0.0244828693201949,0.0250773155042266,
0.0251241095056445,0.0278715865387033,0.0279156772284939,0.0323589146455993,
0.0334651286339482,0.0334988126741926,0.0357819208078993,0.0381532193852836,
0.0390680317130243,0.0415764658205088,0.0441988527874511,0.0446650835655902),
 .UNSPECIFIED.);
#480=B_SPLINE_CURVE_WITH_KNOTS('',3,(#19130,#19131,#19132,#19133,#19134,
#19135,#19136,#19137,#19138,#19139,#19140,#19141,#19142,#19143,#19144,#19145,
#19146,#19147,#19148),.UNSPECIFIED.,.F.,.F.,(4,3,3,3,3,3,4),(0.,0.000209520759735746,
0.000422285836606947,0.000553215152468011,0.000554217096220475,0.00089733059735611,
0.00110843419244095),.UNSPECIFIED.);
#481=B_SPLINE_CURVE_WITH_KNOTS('',3,(#19164,#19165,#19166,#19167,#19168,
#19169,#19170,#19171,#19172,#19173,#19174,#19175,#19176),.UNSPECIFIED.,
 .F.,.F.,(4,3,3,3,4),(0.,0.000732343305453042,0.00114589002873166,0.00114609016424996,
0.00229218032849993),.UNSPECIFIED.);
#482=B_SPLINE_CURVE_WITH_KNOTS('',3,(#19178,#19179,#19180,#19181,#19182,
#19183,#19184,#19185,#19186,#19187,#19188,#19189,#19190,#19191,#19192,#19193,
#19194,#19195,#19196,#19197,#19198,#19199,#19200,#19201,#19202,#19203,#19204,
#19205,#19206,#19207,#19208,#19209,#19210,#19211),.UNSPECIFIED.,.F.,.F.,
(4,3,3,3,3,3,3,3,3,3,3,4),(0.,0.00365414724118507,0.0072761561111727,0.0086843723171071,
0.00868483454405469,0.0100721107296485,0.0114668861298135,0.012827029272143,
0.0130265584756607,0.0130435595235905,0.0155867439515361,0.0173687446342142),
 .UNSPECIFIED.);
#483=B_SPLINE_CURVE_WITH_KNOTS('',3,(#19213,#19214,#19215,#19216,#19217,
#19218,#19219,#19220,#19221,#19222,#19223,#19224,#19225),.UNSPECIFIED.,
 .F.,.F.,(4,3,3,3,4),(0.,0.000722789662616506,0.00114552600039172,0.00114627200830295,
0.00229254401660589),.UNSPECIFIED.);
#484=B_SPLINE_CURVE_WITH_KNOTS('',3,(#19234,#19235,#19236,#19237,#19238,
#19239,#19240,#19241,#19242,#19243,#19244,#19245,#19246),.UNSPECIFIED.,
 .F.,.F.,(4,3,3,3,4),(0.,0.000722789662305103,0.00114552600039174,0.00114627200830296,
0.00229254401660593),.UNSPECIFIED.);
#485=B_SPLINE_CURVE_WITH_KNOTS('',3,(#19258,#19259,#19260,#19261,#19262,
#19263,#19264,#19265,#19266,#19267,#19268,#19269,#19270),.UNSPECIFIED.,
 .F.,.F.,(4,3,3,3,4),(0.,0.000732343305065348,0.00114589002873164,0.00114609016424995,
0.00229218032849991),.UNSPECIFIED.);
#486=B_SPLINE_CURVE_WITH_KNOTS('',3,(#19271,#19272,#19273,#19274,#19275,
#19276,#19277,#19278,#19279,#19280,#19281,#19282,#19283,#19284,#19285,#19286,
#19287,#19288,#19289),.UNSPECIFIED.,.F.,.F.,(4,3,3,3,3,3,4),(0.,0.00521863817648657,
0.00869843096504882,0.00870860595373375,0.0117141048141897,0.0147339377832446,
0.0173968619300976),.UNSPECIFIED.);
#487=B_SPLINE_CURVE_WITH_KNOTS('',3,(#19305,#19306,#19307,#19308,#19309,
#19310,#19311,#19312,#19313,#19314,#19315,#19316,#19317,#19318,#19319,#19320,
#19321,#19322,#19323,#19324,#19325,#19326,#19327,#19328,#19329,#19330,#19331,
#19332,#19333,#19334,#19335,#19336,#19337,#19338,#19339,#19340,#19341,#19342,
#19343,#19344,#19345,#19346,#19347,#19348,#19349,#19350,#19351,#19352,#19353,
#19354,#19355,#19356,#19357,#19358,#19359),.UNSPECIFIED.,.F.,.F.,(4,3,3,
3,3,3,3,3,3,3,3,3,3,3,3,3,3,3,4),(0.,1.698189733476E-5,8.14940608034467E-5,
0.00014434612734546,0.000176187184848135,0.000188127581411639,0.000198575428404704,
0.000271710357356161,0.000368390804286231,0.000407565536034241,0.000522428725604158,
0.000543393651925955,0.000543420714712321,0.000611348304051362,0.000713239688059922,
0.000815131072068482,0.000915281326817688,0.00101655523193233,0.00108684142942464),
 .UNSPECIFIED.);
#488=B_SPLINE_CURVE_WITH_KNOTS('',3,(#19363,#19364,#19365,#19366,#19367,
#19368,#19369,#19370,#19371,#19372,#19373,#19374,#19375,#19376,#19377,#19378,
#19379,#19380,#19381),.UNSPECIFIED.,.F.,.F.,(4,3,3,3,3,3,4),(0.,0.000386464906251142,
0.000552252634628128,0.000553922129943384,0.000781486939925102,0.000957814850417398,
0.00110784425988677),.UNSPECIFIED.);
#489=B_SPLINE_CURVE_WITH_KNOTS('',3,(#19385,#19386,#19387,#19388,#19389,
#19390,#19391,#19392),.UNSPECIFIED.,.F.,.F.,(4,2,2,4),(0.,0.000279899994294907,
0.000559799988589814,0.00111959997717964),.UNSPECIFIED.);
#490=B_SPLINE_CURVE_WITH_KNOTS('',3,(#19396,#19397,#19398,#19399,#19400,
#19401,#19402,#19403,#19404,#19405,#19406,#19407,#19408,#19409,#19410,#19411,
#19412,#19413,#19414,#19415,#19416,#19417,#19418,#19419,#19420,#19421,#19422,
#19423,#19424,#19425,#19426,#19427,#19428,#19429,#19430,#19431,#19432,#19433,
#19434,#19435,#19436,#19437,#19438,#19439,#19440,#19441,#19442,#19443,#19444,
#19445,#19446,#19447,#19448,#19449,#19450),.UNSPECIFIED.,.F.,.F.,(4,3,3,
3,3,3,3,3,3,3,3,3,3,3,3,3,3,3,4),(0.,6.41135074222687E-5,0.000127328256831397,
0.000175449478231306,0.000175455278330882,0.000350898956462612,0.000350910556668815,
0.000701797912925202,0.000701821113336483,0.000745660282483025,0.000850761974087649,
0.000899178575935408,0.0009759377226616,0.0010143172960247,0.00105269686938779,
0.00115231295106207,0.00122814634761909,0.00133756611931813,0.00140359582585038),
 .UNSPECIFIED.);
#491=B_SPLINE_CURVE_WITH_KNOTS('',3,(#19484,#19485,#19486,#19487,#19488,
#19489,#19490,#19491,#19492,#19493,#19494,#19495,#19496,#19497,#19498,#19499,
#19500,#19501,#19502,#19503,#19504,#19505,#19506,#19507,#19508,#19509,#19510,
#19511,#19512,#19513,#19514,#19515,#19516,#19517,#19518,#19519,#19520,#19521,
#19522,#19523,#19524,#19525,#19526,#19527,#19528,#19529,#19530,#19531,#19532,
#19533,#19534,#19535,#19536,#19537,#19538),.UNSPECIFIED.,.F.,.F.,(4,3,3,
3,3,3,3,3,3,3,3,3,3,3,3,3,3,3,4),(0.,6.41135074144232E-5,0.000127328256817319,
0.000175449478231299,0.000175455278330868,0.000350898956462599,0.000350910556668804,
0.000701797912925195,0.000701821113336461,0.00074566028248302,0.000850761974086255,
0.000899178575935406,0.000975937722661599,0.0010143172960247,0.00105269686938779,
0.00115231295106248,0.00122814634761909,0.00133756611931546,0.00140359582585039),
 .UNSPECIFIED.);
#492=B_SPLINE_CURVE_WITH_KNOTS('',3,(#19548,#19549,#19550,#19551,#19552,
#19553,#19554,#19555,#19556,#19557,#19558,#19559,#19560,#19561,#19562,#19563,
#19564,#19565,#19566,#19567,#19568,#19569,#19570,#19571,#19572,#19573,#19574,
#19575,#19576,#19577,#19578,#19579,#19580,#19581,#19582,#19583,#19584,#19585,
#19586,#19587,#19588,#19589,#19590,#19591,#19592,#19593,#19594,#19595,#19596,
#19597,#19598,#19599,#19600,#19601,#19602),.UNSPECIFIED.,.F.,.F.,(4,3,3,
3,3,3,3,3,3,3,3,3,3,3,3,3,3,3,4),(0.,1.69818973347599E-5,8.14940608033093E-5,
0.000144346127345459,0.000176187184848134,0.000188127581411637,0.000198575428404702,
0.000271710357356158,0.000368390804288842,0.000407565536034237,0.00052242872560825,
0.000543393651925955,0.000543420714712316,0.000611348304051356,0.000713239688059915,
0.000815131072068475,0.000915281326823676,0.00101655523194574,0.00108684142942463),
 .UNSPECIFIED.);
#493=B_SPLINE_CURVE_WITH_KNOTS('',3,(#19606,#19607,#19608,#19609,#19610,
#19611,#19612,#19613,#19614,#19615,#19616,#19617,#19618,#19619,#19620,#19621,
#19622,#19623,#19624,#19625,#19626,#19627),.UNSPECIFIED.,.F.,.F.,(4,3,3,
3,3,3,3,4),(0.,0.000386658565627056,0.000552413504322274,0.000554054021566752,
0.00077021335329488,0.000939160698214192,0.00109876969131035,0.0011081080431335),
 .UNSPECIFIED.);
#494=B_SPLINE_CURVE_WITH_KNOTS('',3,(#19630,#19631,#19632,#19633,#19634,
#19635,#19636,#19637),.UNSPECIFIED.,.F.,.F.,(4,2,2,4),(0.,0.000279899994294914,
0.000559799988589829,0.00111959997717965),.UNSPECIFIED.);
#495=B_SPLINE_CURVE_WITH_KNOTS('',3,(#19642,#19643,#19644,#19645,#19646,
#19647,#19648,#19649,#19650,#19651,#19652,#19653,#19654,#19655,#19656,#19657,
#19658,#19659,#19660,#19661,#19662,#19663,#19664,#19665,#19666,#19667,#19668,
#19669,#19670,#19671,#19672,#19673,#19674,#19675,#19676,#19677,#19678,#19679,
#19680,#19681,#19682,#19683,#19684,#19685,#19686,#19687,#19688,#19689,#19690,
#19691,#19692,#19693,#19694,#19695,#19696),.UNSPECIFIED.,.F.,.F.,(4,3,3,
3,3,3,3,3,3,3,3,3,3,3,3,3,3,3,4),(0.,6.41135074167853E-5,0.000127328256820419,
0.000175449478231291,0.000175455278330845,0.000350898956462582,0.000350910556668788,
0.000701797912925185,0.000701821113336456,0.00074566028248301,0.000850761974083129,
0.000899178575935398,0.000975937722661593,0.00101431729602469,0.00105269686938779,
0.0011523129510611,0.00122814634761909,0.00133756611931672,0.00140359582585039),
 .UNSPECIFIED.);
#496=B_SPLINE_CURVE_WITH_KNOTS('',3,(#19703,#19704,#19705,#19706,#19707,
#19708,#19709,#19710,#19711,#19712,#19713,#19714,#19715,#19716,#19717,#19718,
#19719,#19720,#19721,#19722,#19723,#19724,#19725,#19726,#19727,#19728,#19729,
#19730,#19731,#19732,#19733,#19734,#19735,#19736,#19737,#19738,#19739,#19740,
#19741,#19742,#19743,#19744,#19745,#19746,#19747,#19748,#19749,#19750,#19751,
#19752,#19753,#19754,#19755,#19756,#19757),.UNSPECIFIED.,.F.,.F.,(4,3,3,
3,3,3,3,3,3,3,3,3,3,3,3,3,3,3,4),(0.,1.69818973347599E-5,8.1494060804179E-5,
0.000144346127345459,0.000176187184848134,0.000188127581411637,0.000198575428404702,
0.000271710357356159,0.000368390804303863,0.000407565536034238,0.000522428725615084,
0.000543393651925945,0.000543420714712318,0.000611348304051357,0.000713239688059917,
0.000815131072068476,0.000915281326813642,0.00101655523192292,0.00108684142942464),
 .UNSPECIFIED.);
#497=B_SPLINE_CURVE_WITH_KNOTS('',3,(#19761,#19762,#19763,#19764,#19765,
#19766,#19767,#19768,#19769,#19770,#19771,#19772,#19773,#19774,#19775,#19776,
#19777,#19778,#19779,#19780,#19781,#19782),.UNSPECIFIED.,.F.,.F.,(4,3,3,
3,3,3,3,4),(0.,0.000387102023918642,0.00055263573178344,0.000554236032887,
0.000759142685557146,0.000933807375665573,0.00108627346338914,0.001108472065774),
 .UNSPECIFIED.);
#498=B_SPLINE_CURVE_WITH_KNOTS('',3,(#19785,#19786,#19787,#19788,#19789,
#19790,#19791,#19792),.UNSPECIFIED.,.F.,.F.,(4,2,2,4),(0.,0.000279899994294914,
0.000559799988589829,0.00111959997717965),.UNSPECIFIED.);
#499=B_SPLINE_CURVE_WITH_KNOTS('',3,(#19801,#19802,#19803,#19804,#19805,
#19806,#19807,#19808,#19809,#19810,#19811,#19812,#19813,#19814,#19815,#19816,
#19817,#19818,#19819,#19820,#19821,#19822,#19823,#19824,#19825,#19826,#19827,
#19828,#19829,#19830,#19831,#19832,#19833,#19834,#19835,#19836,#19837,#19838,
#19839,#19840,#19841,#19842,#19843,#19844,#19845,#19846,#19847,#19848,#19849,
#19850,#19851,#19852,#19853,#19854,#19855),.UNSPECIFIED.,.F.,.F.,(4,3,3,
3,3,3,3,3,3,3,3,3,3,3,3,3,3,3,4),(0.,1.69818973347602E-5,8.14940608001835E-5,
0.000144346127345461,0.000176187184848137,0.00018812758141164,0.000198575428404705,
0.000271710357356162,0.000368390804273793,0.000407565536034244,0.00052242872563187,
0.000543393651925935,0.000543420714712325,0.000611348304051366,0.000713239688059926,
0.000815131072068487,0.000915281326815586,0.00101655523192821,0.00108684142942465),
 .UNSPECIFIED.);
#500=B_SPLINE_CURVE_WITH_KNOTS('',3,(#19859,#19860,#19861,#19862,#19863,
#19864,#19865,#19866,#19867,#19868,#19869,#19870,#19871,#19872,#19873,#19874,
#19875,#19876,#19877,#19878,#19879,#19880),.UNSPECIFIED.,.F.,.F.,(4,3,3,
3,3,3,3,4),(0.,0.000387003724944105,0.00055259360350697,0.000554201545442304,
0.000760942537037389,0.000934672813960999,0.0010883087198129,0.00110840309088461),
 .UNSPECIFIED.);
#501=B_SPLINE_CURVE_WITH_KNOTS('',3,(#19884,#19885,#19886,#19887,#19888,
#19889,#19890,#19891),.UNSPECIFIED.,.F.,.F.,(4,2,2,4),(0.,0.000279899994294911,
0.000559799988589822,0.00111959997717963),.UNSPECIFIED.);
#502=B_SPLINE_CURVE_WITH_KNOTS('',3,(#19895,#19896,#19897,#19898,#19899,
#19900,#19901,#19902,#19903,#19904,#19905,#19906,#19907,#19908,#19909,#19910,
#19911,#19912,#19913,#19914,#19915,#19916,#19917,#19918,#19919,#19920,#19921,
#19922,#19923,#19924,#19925,#19926,#19927,#19928,#19929,#19930,#19931,#19932,
#19933,#19934,#19935,#19936,#19937,#19938,#19939,#19940,#19941,#19942,#19943,
#19944,#19945,#19946,#19947,#19948,#19949),.UNSPECIFIED.,.F.,.F.,(4,3,3,
3,3,3,3,3,3,3,3,3,3,3,3,3,3,3,4),(0.,6.41135074214198E-5,0.000127328256829034,
0.00017544947823129,0.000175455278330849,0.000350898956462581,0.000350910556668772,
0.000701797912925182,0.00070182111333644,0.000745660282483008,0.000850761974083878,
0.000899178575935396,0.00097593772266159,0.00101431729602469,0.00105269686938778,
0.00115231295106392,0.00122814634761908,0.0013375661193188,0.00140359582585039),
 .UNSPECIFIED.);
#503=B_SPLINE_CURVE_WITH_KNOTS('',3,(#19957,#19958,#19959,#19960,#19961,
#19962,#19963,#19964),.UNSPECIFIED.,.F.,.F.,(4,2,2,4),(0.,0.00951523528670846,
0.0142728529300627,0.0190304705734169),.UNSPECIFIED.);
#504=B_SPLINE_CURVE_WITH_KNOTS('',3,(#19968,#19969,#19970,#19971,#19972,
#19973,#19974,#19975),.UNSPECIFIED.,.F.,.F.,(4,2,2,4),(0.,0.00476132581272555,
0.00952265162545109,0.0190453032509022),.UNSPECIFIED.);
#505=B_SPLINE_CURVE_WITH_KNOTS('',3,(#19982,#19983,#19984,#19985,#19986,
#19987,#19988,#19989,#19990,#19991,#19992,#19993,#19994,#19995,#19996,#19997,
#19998,#19999,#20000,#20001,#20002,#20003,#20004,#20005,#20006,#20007,#20008,
#20009,#20010,#20011,#20012,#20013,#20014,#20015),.UNSPECIFIED.,.F.,.F.,
(4,3,3,3,3,3,3,3,3,3,3,4),(0.00419407786743781,0.00785137040128593,0.00864322402522921,
0.0088821607644223,0.0105632172612041,0.0122879239673615,0.0130923701830206,
0.0136962196480357,0.0161859644983365,0.018720550100699,0.0213309666507153,
0.0219906624986034),.UNSPECIFIED.);
#506=B_SPLINE_CURVE_WITH_KNOTS('',3,(#20019,#20020,#20021,#20022,#20023,
#20024,#20025,#20026,#20027,#20028,#20029,#20030,#20031,#20032,#20033,#20034,
#20035,#20036,#20037,#20038,#20039,#20040,#20041,#20042,#20043,#20044,#20045,
#20046,#20047,#20048,#20049,#20050,#20051,#20052),.UNSPECIFIED.,.F.,.F.,
(4,3,3,3,3,3,3,3,3,3,3,4),(0.,0.00259497273884202,0.00513490948758917,0.00760920564643932,
0.00831654261042366,0.00892204401521709,0.0106541774041306,0.0123507369871751,
0.0131434725515692,0.0133830660228256,0.0170412668384166,0.0178440880304342),
 .UNSPECIFIED.);
#507=B_SPLINE_CURVE_WITH_KNOTS('',3,(#20059,#20060,#20061,#20062,#20063,
#20064,#20065,#20066,#20067,#20068,#20069,#20070,#20071,#20072,#20073,#20074,
#20075,#20076,#20077,#20078,#20079,#20080,#20081,#20082,#20083,#20084,#20085,
#20086,#20087,#20088,#20089),.UNSPECIFIED.,.F.,.F.,(4,3,3,3,3,3,3,3,3,3,
4),(0.00423087891556468,0.0137133753542596,0.0177375823121119,0.0182590193856109,
0.0201182201176651,0.0211142581612487,0.0218072955502239,0.0244909340103855,
0.025340876493083,0.0282925811008711,0.0312442857086592),.UNSPECIFIED.);
#508=B_SPLINE_CURVE_WITH_KNOTS('',3,(#20093,#20094,#20095,#20096,#20097,
#20098,#20099,#20100,#20101,#20102,#20103,#20104,#20105,#20106,#20107,#20108,
#20109,#20110,#20111,#20112,#20113,#20114,#20115,#20116,#20117,#20118,#20119,
#20120,#20121,#20122,#20123,#20124,#20125,#20126,#20127,#20128,#20129),
 .UNSPECIFIED.,.F.,.F.,(4,3,3,3,3,3,3,3,3,3,3,3,4),(0.,0.00293383627619294,
0.00586767255238587,0.0067139943242657,0.00908462661547173,0.00938017817101409,
0.0100709914863986,0.0117876962255473,0.0129061418604892,0.0134279886485314,
0.0185395617459084,0.0234677092734861,0.0268559772970628),.UNSPECIFIED.);
#509=B_SPLINE_CURVE_WITH_KNOTS('',3,(#20133,#20134,#20135,#20136,#20137,
#20138),.UNSPECIFIED.,.F.,.F.,(4,2,4),(0.,0.00327855488628776,0.00654795604494931),
 .UNSPECIFIED.);
#510=B_SPLINE_CURVE_WITH_KNOTS('',3,(#20147,#20148,#20149,#20150,#20151,
#20152),.UNSPECIFIED.,.F.,.F.,(4,2,4),(0.,0.00326940115867362,0.00654795604497327),
 .UNSPECIFIED.);
#511=B_SPLINE_CURVE_WITH_KNOTS('',3,(#20181,#20182,#20183,#20184,#20185,
#20186,#20187),.UNSPECIFIED.,.F.,.F.,(4,3,4),(0.,0.00700450430818859,0.00878441731503683),
 .UNSPECIFIED.);
#512=B_SPLINE_CURVE_WITH_KNOTS('',3,(#20203,#20204,#20205,#20206),
 .UNSPECIFIED.,.F.,.F.,(4,4),(0.,0.00906386388585899),.UNSPECIFIED.);
#513=B_SPLINE_CURVE_WITH_KNOTS('',3,(#20254,#20255,#20256,#20257,#20258,
#20259,#20260,#20261,#20262,#20263,#20264,#20265,#20266,#20267,#20268,#20269,
#20270,#20271,#20272,#20273,#20274,#20275,#20276,#20277,#20278,#20279,#20280,
#20281,#20282,#20283,#20284,#20285,#20286,#20287,#20288,#20289,#20290,#20291,
#20292,#20293,#20294,#20295,#20296,#20297,#20298,#20299,#20300,#20301,#20302),
 .UNSPECIFIED.,.F.,.F.,(4,3,3,3,3,3,3,3,3,3,3,3,3,3,3,3,4),(0.,0.000121245606188157,
0.000242857142460205,0.000287360877759076,0.00028827001783867,0.000443403913026412,
0.000574721755518153,0.000575971165655785,0.000665917057794762,0.000718402194397691,
0.00079024241383746,0.000826162523557345,0.000862082633277229,0.000975072145658159,
0.00100576307215677,0.00111728780498847,0.00114944351103631),
 .UNSPECIFIED.);
#514=B_SPLINE_CURVE_WITH_KNOTS('',3,(#20308,#20309,#20310,#20311,#20312,
#20313,#20314,#20315),.UNSPECIFIED.,.F.,.F.,(4,2,2,4),(0.,0.0138082473482012,
0.0207123710223018,0.0276164946964023),.UNSPECIFIED.);
#515=B_SPLINE_CURVE_WITH_KNOTS('',3,(#20327,#20328,#20329,#20330,#20331,
#20332,#20333,#20334,#20335,#20336,#20337,#20338,#20339,#20340,#20341,#20342,
#20343,#20344,#20345,#20346,#20347,#20348,#20349,#20350,#20351,#20352,#20353,
#20354,#20355,#20356,#20357,#20358,#20359,#20360),.UNSPECIFIED.,.F.,.F.,
(4,3,3,3,3,3,3,3,3,3,3,4),(0.,0.000110567770976802,0.000229163742145944,
0.000349602945016014,0.000466129197473093,0.0005039626123088,0.000504370554078788,
0.000654658246680043,0.000733772187615292,0.000861351751012203,0.000986409541283704,
0.00100874110815758),.UNSPECIFIED.);
#516=B_SPLINE_CURVE_WITH_KNOTS('',3,(#20377,#20378,#20379,#20380,#20381,
#20382,#20383,#20384,#20385,#20386,#20387,#20388,#20389,#20390,#20391,#20392,
#20393,#20394,#20395,#20396,#20397,#20398,#20399,#20400,#20401,#20402,#20403,
#20404),.UNSPECIFIED.,.F.,.F.,(4,3,3,3,3,3,3,3,3,4),(0.,9.61627041892685E-5,
0.000194643124037823,0.000263598431963766,0.000263909149293665,0.000510523428020468,
0.000527611135930389,0.00052781829858733,0.000791654292983009,0.00105563659717465),
 .UNSPECIFIED.);
#517=B_SPLINE_CURVE_WITH_KNOTS('',3,(#20410,#20411,#20412,#20413,#20414,
#20415,#20416,#20417,#20418,#20419,#20420,#20421,#20422,#20423,#20424,#20425),
 .UNSPECIFIED.,.F.,.F.,(4,3,3,3,3,4),(4.53161437099327E-15,0.00201520691464592,
0.00402253547213016,0.00602595242291411,0.00802370171983992,0.00993491157965329),
 .UNSPECIFIED.);
#518=B_SPLINE_CURVE_WITH_KNOTS('',3,(#20427,#20428,#20429,#20430,#20431,
#20432,#20433,#20434,#20435,#20436,#20437,#20438,#20439,#20440,#20441,#20442,
#20443,#20444,#20445,#20446,#20447,#20448,#20449,#20450,#20451,#20452,#20453,
#20454,#20455,#20456,#20457,#20458,#20459,#20460,#20461,#20462,#20463,#20464,
#20465,#20466,#20467,#20468,#20469),.UNSPECIFIED.,.F.,.F.,(4,3,3,3,3,3,
3,3,3,3,3,3,3,3,4),(0.,0.000142261508827042,0.000306612281831946,0.000354680426257009,
0.000354839578464811,0.000671890822089835,0.000709360852514019,0.000709794319646003,
0.000798030959078271,0.00093103611892465,0.00106404127877103,0.00117707199637858,
0.00124138149189953,0.00135612593310508,0.00141872170502804),
 .UNSPECIFIED.);
#519=B_SPLINE_CURVE_WITH_KNOTS('',3,(#20476,#20477,#20478,#20479,#20480,
#20481,#20482,#20483,#20484,#20485,#20486,#20487,#20488,#20489,#20490,#20491,
#20492,#20493,#20494,#20495,#20496,#20497,#20498,#20499,#20500,#20501,#20502,
#20503,#20504,#20505,#20506,#20507,#20508,#20509,#20510,#20511,#20512,#20513,
#20514,#20515,#20516,#20517,#20518,#20519,#20520,#20521,#20522,#20523,#20524,
#20525,#20526,#20527,#20528,#20529,#20530),.UNSPECIFIED.,.F.,.F.,(4,3,3,
3,3,3,3,3,3,3,3,3,3,3,3,3,3,3,4),(0.,0.00292798214607904,0.00577262065187083,
0.00682756145262549,0.00693335737727645,0.00947217443522634,0.0103475581420103,
0.0104000360659147,0.0118697041221879,0.0132773954676776,0.0138667147545529,
0.013878114522684,0.0166264516377915,0.0173333934431911,0.0189487413423515,
0.0205003989924771,0.0210540430948269,0.0243937363016876,0.0277334295085483),
 .UNSPECIFIED.);
#520=B_SPLINE_CURVE_WITH_KNOTS('',3,(#20551,#20552,#20553,#20554,#20555,
#20556,#20557,#20558,#20559,#20560,#20561,#20562,#20563,#20564,#20565,#20566,
#20567,#20568,#20569,#20570,#20571,#20572,#20573,#20574,#20575,#20576,#20577,
#20578,#20579,#20580,#20581,#20582,#20583,#20584,#20585,#20586,#20587,#20588,
#20589,#20590),.UNSPECIFIED.,.F.,.F.,(4,3,3,3,3,3,3,3,3,3,3,3,3,4),(0.,
0.00261722397919538,0.00435913346757957,0.0043687095238485,0.00564078314595562,
0.00692512632512478,0.008186704139069,0.008737419047697,0.0087491646894187,
0.0122136782966271,0.0131061285715455,0.0147515701823087,0.016420240909498,
0.017474838095394),.UNSPECIFIED.);
#521=B_SPLINE_CURVE_WITH_KNOTS('',3,(#20636,#20637,#20638,#20639,#20640,
#20641,#20642,#20643,#20644,#20645,#20646,#20647,#20648),.UNSPECIFIED.,
 .F.,.F.,(4,3,3,3,4),(0.,0.000355508868042915,0.000556947538855278,0.000557267210332337,
0.00111453442066467),.UNSPECIFIED.);
#522=B_SPLINE_CURVE_WITH_KNOTS('',3,(#20650,#20651,#20652,#20653,#20654,
#20655,#20656,#20657,#20658,#20659,#20660,#20661,#20662,#20663,#20664,#20665,
#20666,#20667,#20668,#20669,#20670,#20671,#20672,#20673,#20674,#20675,#20676,
#20677,#20678,#20679,#20680,#20681,#20682,#20683,#20684,#20685,#20686,#20687,
#20688,#20689,#20690,#20691,#20692,#20693,#20694,#20695,#20696,#20697,#20698,
#20699,#20700,#20701,#20702,#20703,#20704,#20705,#20706,#20707,#20708,#20709,
#20710,#20711,#20712,#20713,#20714,#20715,#20716),.UNSPECIFIED.,.F.,.F.,
(4,3,3,3,3,3,3,3,3,3,3,3,3,3,3,3,3,3,3,3,3,3,4),(0.,0.00277040425654159,
0.00554080851308318,0.00557505688803485,0.00791560355762107,0.0083263576942907,
0.00836258533205228,0.0100018252550587,0.011122873465018,0.0111501137760697,
0.0223002275521394,0.0223209744612517,0.0250877559961568,0.025120499376563,
0.0278752844401743,0.0279173397075125,0.0311894101768246,0.0334503413282091,
0.0334957141052527,0.0369394202828642,0.040438907290041,0.044027168743403,
0.0446004551042788),.UNSPECIFIED.);
#523=B_SPLINE_CURVE_WITH_KNOTS('',3,(#20717,#20718,#20719,#20720,#20721,
#20722,#20723,#20724,#20725,#20726,#20727,#20728,#20729,#20730,#20731,#20732,
#20733,#20734,#20735),.UNSPECIFIED.,.F.,.F.,(4,3,3,3,3,3,4),(0.,0.000209520759737123,
0.000422285836605981,0.000553215152468032,0.000554217096220492,0.000897330597223569,
0.00110843419244098),.UNSPECIFIED.);
#524=B_SPLINE_CURVE_WITH_KNOTS('',3,(#20748,#20749,#20750,#20751,#20752,
#20753,#20754,#20755,#20756,#20757,#20758,#20759,#20760),.UNSPECIFIED.,
 .F.,.F.,(4,3,3,3,4),(0.,0.000732343305081284,0.00114589002873166,0.00114609016424997,
0.00229218032849994),.UNSPECIFIED.);
#525=B_SPLINE_CURVE_WITH_KNOTS('',3,(#20762,#20763,#20764,#20765,#20766,
#20767,#20768,#20769,#20770,#20771,#20772,#20773,#20774,#20775,#20776,#20777,
#20778,#20779,#20780,#20781,#20782,#20783,#20784,#20785,#20786,#20787,#20788,
#20789,#20790,#20791,#20792,#20793,#20794,#20795),.UNSPECIFIED.,.F.,.F.,
(4,3,3,3,3,3,3,3,3,3,3,4),(0.,0.0036541472315085,0.00727615609223089,0.00868437231710706,
0.00868483454405465,0.0100721107297951,0.0114668861300835,0.0128270292725488,
0.0130265584756606,0.0130435595235904,0.0155867439443868,0.0173687446342141),
 .UNSPECIFIED.);
#526=B_SPLINE_CURVE_WITH_KNOTS('',3,(#20797,#20798,#20799,#20800,#20801,
#20802,#20803,#20804,#20805,#20806,#20807,#20808,#20809),.UNSPECIFIED.,
 .F.,.F.,(4,3,3,3,4),(0.,0.000722789662749714,0.00114552600039176,0.00114627200830298,
0.00229254401660596),.UNSPECIFIED.);
#527=B_SPLINE_CURVE_WITH_KNOTS('',3,(#20819,#20820,#20821,#20822,#20823,
#20824,#20825,#20826),.UNSPECIFIED.,.F.,.F.,(4,2,2,4),(0.,0.00951523528670842,
0.0142728529300626,0.0190304705734168),.UNSPECIFIED.);
#528=B_SPLINE_CURVE_WITH_KNOTS('',3,(#20830,#20831,#20832,#20833,#20834,
#20835,#20836,#20837),.UNSPECIFIED.,.F.,.F.,(4,2,2,4),(0.,0.00476132581272552,
0.00952265162545105,0.0190453032509021),.UNSPECIFIED.);
#529=B_SPLINE_CURVE_WITH_KNOTS('',3,(#20844,#20845,#20846,#20847,#20848,
#20849,#20850,#20851,#20852,#20853,#20854,#20855,#20856,#20857,#20858,#20859,
#20860,#20861,#20862,#20863,#20864,#20865,#20866,#20867,#20868,#20869,#20870,
#20871,#20872,#20873,#20874,#20875,#20876,#20877),.UNSPECIFIED.,.F.,.F.,
(4,3,3,3,3,3,3,3,3,3,3,4),(0.00419407786743798,0.00785137041686624,0.00864322402522942,
0.00888216076442249,0.0105632172612883,0.0122879239673143,0.0130923701830209,
0.0136962196480359,0.0161859644983103,0.0187205501006744,0.0213309666507051,
0.0219906624986038),.UNSPECIFIED.);
#530=B_SPLINE_CURVE_WITH_KNOTS('',3,(#20881,#20882,#20883,#20884,#20885,
#20886,#20887,#20888,#20889,#20890,#20891,#20892,#20893,#20894,#20895,#20896,
#20897,#20898,#20899,#20900,#20901,#20902,#20903,#20904,#20905,#20906,#20907,
#20908,#20909,#20910,#20911,#20912,#20913,#20914),.UNSPECIFIED.,.F.,.F.,
(4,3,3,3,3,3,3,3,3,3,3,4),(0.,0.00259497273991662,0.00513490948980078,0.0076092056498656,
0.00831654261042356,0.00892204401521706,0.0106541774039888,0.0123507369870092,
0.0131434725515691,0.0133830660228256,0.017041266814901,0.0178440880304341),
 .UNSPECIFIED.);
#531=B_SPLINE_CURVE_WITH_KNOTS('',3,(#20919,#20920,#20921,#20922,#20923,
#20924),.UNSPECIFIED.,.F.,.F.,(4,2,4),(0.,0.00327855488628776,0.00654795604494929),
 .UNSPECIFIED.);
#532=B_SPLINE_CURVE_WITH_KNOTS('',3,(#20934,#20935,#20936,#20937,#20938,
#20939),.UNSPECIFIED.,.F.,.F.,(4,2,4),(0.,0.00326940115867351,0.00654795604497326),
 .UNSPECIFIED.);
#533=B_SPLINE_CURVE_WITH_KNOTS('',3,(#20962,#20963,#20964,#20965,#20966,
#20967,#20968),.UNSPECIFIED.,.F.,.F.,(4,3,4),(0.,0.00700450431179497,0.00878441731503681),
 .UNSPECIFIED.);
#534=B_SPLINE_CURVE_WITH_KNOTS('',3,(#20984,#20985,#20986,#20987),
 .UNSPECIFIED.,.F.,.F.,(4,4),(0.,0.00906386388585898),.UNSPECIFIED.);
#535=B_SPLINE_CURVE_WITH_KNOTS('',3,(#21029,#21030,#21031,#21032,#21033,
#21034,#21035,#21036,#21037,#21038,#21039,#21040,#21041,#21042,#21043,#21044,
#21045,#21046,#21047,#21048,#21049,#21050,#21051,#21052,#21053,#21054,#21055,
#21056,#21057,#21058,#21059,#21060,#21061,#21062,#21063,#21064,#21065,#21066,
#21067,#21068,#21069,#21070,#21071,#21072,#21073,#21074,#21075,#21076,#21077),
 .UNSPECIFIED.,.F.,.F.,(4,3,3,3,3,3,3,3,3,3,3,3,3,3,3,3,4),(0.,0.000121245606219857,
0.00024285714250704,0.000287360877759074,0.000288270017838685,0.000443403913075757,
0.000574721755518148,0.000575971165655791,0.000665917057795795,0.000718402194397685,
0.000790242413837453,0.000826162523557337,0.000862082633277221,0.000975072145653548,
0.00100576307215676,0.00111728780499056,0.0011494435110363),
 .UNSPECIFIED.);
#536=B_SPLINE_CURVE_WITH_KNOTS('',3,(#21083,#21084,#21085,#21086,#21087,
#21088,#21089,#21090),.UNSPECIFIED.,.F.,.F.,(4,2,2,4),(0.,0.0138082473482012,
0.0207123710223018,0.0276164946964024),.UNSPECIFIED.);
#537=B_SPLINE_CURVE_WITH_KNOTS('',3,(#21105,#21106,#21107,#21108,#21109,
#21110,#21111,#21112,#21113,#21114,#21115,#21116,#21117,#21118,#21119,#21120,
#21121,#21122,#21123,#21124,#21125,#21126,#21127,#21128,#21129,#21130,#21131,
#21132,#21133,#21134,#21135,#21136,#21137,#21138),.UNSPECIFIED.,.F.,.F.,
(4,3,3,3,3,3,3,3,3,3,3,4),(0.,0.000110567770962462,0.000229163742115291,
0.000349602944967853,0.000466129197406935,0.000503962612308805,0.000504370554078785,
0.000654658246624721,0.000733772187615348,0.000861351750904368,0.000986409541163883,
0.00100874110815757),.UNSPECIFIED.);
#538=B_SPLINE_CURVE_WITH_KNOTS('',3,(#21156,#21157,#21158,#21159,#21160,
#21161,#21162,#21163,#21164,#21165,#21166,#21167,#21168,#21169,#21170,#21171,
#21172,#21173,#21174,#21175,#21176,#21177,#21178,#21179,#21180,#21181,#21182,
#21183),.UNSPECIFIED.,.F.,.F.,(4,3,3,3,3,3,3,3,3,4),(0.,9.61627041725452E-5,
0.000194643124037966,0.000263598431963772,0.00026390914929366,0.000510523427664749,
0.000527611135930377,0.00052781829858732,0.000791654292983059,0.00105563659717466),
 .UNSPECIFIED.);
#539=B_SPLINE_CURVE_WITH_KNOTS('',3,(#21189,#21190,#21191,#21192,#21193,
#21194,#21195,#21196,#21197,#21198,#21199,#21200,#21201,#21202,#21203,#21204),
 .UNSPECIFIED.,.F.,.F.,(4,3,3,3,3,4),(4.52453455287509E-15,0.00201520691454269,
0.00402253547200752,0.00602595242278867,0.008023701719707,0.00993491157965328),
 .UNSPECIFIED.);
#540=B_SPLINE_CURVE_WITH_KNOTS('',3,(#21206,#21207,#21208,#21209,#21210,
#21211,#21212,#21213,#21214,#21215,#21216,#21217,#21218,#21219,#21220,#21221,
#21222,#21223,#21224,#21225,#21226,#21227,#21228,#21229,#21230,#21231,#21232,
#21233,#21234,#21235,#21236,#21237,#21238,#21239,#21240,#21241,#21242,#21243,
#21244,#21245,#21246,#21247,#21248),.UNSPECIFIED.,.F.,.F.,(4,3,3,3,3,3,
3,3,3,3,3,3,3,3,4),(0.,0.000142261508819856,0.000306612281818102,0.000354680426257006,
0.000354839578464825,0.000671890823263132,0.000709360852514012,0.000709794319645991,
0.000798030959078264,0.000931036118924641,0.00106404127877102,0.00117707199638153,
0.00124138149189952,0.00135612593304764,0.00141872170502802),
 .UNSPECIFIED.);
#541=B_SPLINE_CURVE_WITH_KNOTS('',3,(#21255,#21256,#21257,#21258,#21259,
#21260,#21261,#21262,#21263,#21264,#21265,#21266,#21267,#21268,#21269,#21270,
#21271,#21272,#21273,#21274,#21275,#21276,#21277,#21278,#21279,#21280,#21281,
#21282,#21283,#21284,#21285,#21286,#21287,#21288,#21289,#21290,#21291,#21292,
#21293,#21294,#21295,#21296,#21297,#21298,#21299,#21300,#21301,#21302,#21303,
#21304,#21305,#21306,#21307,#21308,#21309),.UNSPECIFIED.,.F.,.F.,(4,3,3,
3,3,3,3,3,3,3,3,3,3,3,3,3,3,3,4),(0.,0.00292798214153551,0.0057726206412551,
0.00682756145262537,0.00693335737727641,0.00947217442119118,0.0103475581420101,
0.0104000360659146,0.0118697041223215,0.013277395467897,0.0138667147545528,
0.0138781145226838,0.016626451636874,0.017333393443191,0.0189487413424095,
0.0205003989924608,0.0210540430948119,0.02439373630168,0.0277334295085482),
 .UNSPECIFIED.);
#542=B_SPLINE_CURVE_WITH_KNOTS('',3,(#21321,#21322,#21323,#21324,#21325,
#21326,#21327,#21328,#21329,#21330,#21331,#21332,#21333,#21334,#21335,#21336,
#21337,#21338,#21339,#21340,#21341,#21342,#21343,#21344,#21345,#21346,#21347,
#21348,#21349,#21350,#21351,#21352,#21353,#21354,#21355,#21356,#21357,#21358,
#21359,#21360),.UNSPECIFIED.,.F.,.F.,(4,3,3,3,3,3,3,3,3,3,3,3,3,4),(0.,
0.00261722398002284,0.00435913346757954,0.00436870952384852,0.00564078314584605,
0.00692512632493898,0.00818670413883311,0.00873741904769704,0.00874916468941873,
0.0122136783028313,0.0131061285715456,0.0147515701824667,0.0164202409098317,
0.0174748380953941),.UNSPECIFIED.);
#543=B_SPLINE_CURVE_WITH_KNOTS('',3,(#21365,#21366,#21367,#21368,#21369,
#21370,#21371,#21372,#21373,#21374,#21375,#21376,#21377,#21378,#21379,#21380,
#21381,#21382,#21383),.UNSPECIFIED.,.F.,.F.,(4,3,3,3,3,3,4),(0.,0.000209520759759855,
0.000422285836655203,0.000553215152468034,0.000554217096220497,0.000897330597719915,
0.00110843419244099),.UNSPECIFIED.);
#544=B_SPLINE_CURVE_WITH_KNOTS('',3,(#21395,#21396,#21397,#21398,#21399,
#21400,#21401,#21402,#21403,#21404,#21405,#21406,#21407),.UNSPECIFIED.,
 .F.,.F.,(4,3,3,3,4),(0.,0.0003555088680465,0.000556947538855288,0.000557267210332349,
0.0011145344206647),.UNSPECIFIED.);
#545=B_SPLINE_CURVE_WITH_KNOTS('',3,(#21408,#21409,#21410,#21411,#21412,
#21413,#21414,#21415,#21416,#21417,#21418,#21419,#21420,#21421,#21422,#21423,
#21424,#21425,#21426,#21427,#21428,#21429,#21430,#21431,#21432,#21433,#21434,
#21435,#21436,#21437,#21438,#21439,#21440,#21441,#21442,#21443,#21444,#21445,
#21446,#21447,#21448,#21449,#21450,#21451,#21452,#21453,#21454,#21455,#21456,
#21457,#21458,#21459,#21460,#21461,#21462,#21463,#21464,#21465,#21466,#21467,
#21468,#21469,#21470,#21471,#21472,#21473,#21474),.UNSPECIFIED.,.F.,.F.,
(4,3,3,3,3,3,3,3,3,3,3,3,3,3,3,3,3,3,3,3,3,3,4),(0.,0.00277040425654159,
0.00554080851308317,0.00557505688803486,0.00791560355474336,0.0083263576942907,
0.00836258533205228,0.0100018252550135,0.0111228734650181,0.0111501137760697,
0.0223002275521394,0.0223209744612517,0.0250877559961568,0.0251204993765631,
0.0278752844401743,0.0279173397075124,0.0311894101769749,0.0334503413282091,
0.0334957141052527,0.0369394202827702,0.0404389072898642,0.0440271687431145,
0.0446004551042788),.UNSPECIFIED.);
#546=B_SPLINE_CURVE_WITH_KNOTS('',3,(#21485,#21486,#21487,#21488,#21489,
#21490,#21491,#21492,#21493,#21494,#21495,#21496,#21497),.UNSPECIFIED.,
 .F.,.F.,(4,3,3,3,4),(0.,0.000732343305562431,0.00114589002873164,0.00114609016424995,
0.00229218032849991),.UNSPECIFIED.);
#547=B_SPLINE_CURVE_WITH_KNOTS('',3,(#21499,#21500,#21501,#21502,#21503,
#21504,#21505,#21506,#21507,#21508,#21509,#21510,#21511,#21512,#21513,#21514,
#21515,#21516,#21517,#21518,#21519,#21520,#21521,#21522,#21523,#21524,#21525,
#21526,#21527,#21528,#21529,#21530,#21531,#21532),.UNSPECIFIED.,.F.,.F.,
(4,3,3,3,3,3,3,3,3,3,3,4),(0.,0.00365414724118463,0.00727615611117417,0.0086843723171071,
0.0086848345440547,0.0100721107296907,0.0114668861299102,0.0128270292722496,
0.0130265584756607,0.0130435595235905,0.0155867439504688,0.0173687446342142),
 .UNSPECIFIED.);
#548=B_SPLINE_CURVE_WITH_KNOTS('',3,(#21534,#21535,#21536,#21537,#21538,
#21539,#21540,#21541,#21542,#21543,#21544,#21545,#21546),.UNSPECIFIED.,
 .F.,.F.,(4,3,3,3,4),(0.,0.000722789662613087,0.00114552600039172,0.00114627200830295,
0.00229254401660589),.UNSPECIFIED.);
#549=B_SPLINE_CURVE_WITH_KNOTS('',3,(#21558,#21559,#21560,#21561,#21562,
#21563,#21564,#21565),.UNSPECIFIED.,.F.,.F.,(4,2,2,4),(0.,0.00951523528670849,
0.0142728529300627,0.019030470573417),.UNSPECIFIED.);
#550=B_SPLINE_CURVE_WITH_KNOTS('',3,(#21569,#21570,#21571,#21572,#21573,
#21574,#21575,#21576),.UNSPECIFIED.,.F.,.F.,(4,2,2,4),(0.,0.00476132581272557,
0.00952265162545114,0.0190453032509023),.UNSPECIFIED.);
#551=B_SPLINE_CURVE_WITH_KNOTS('',3,(#21583,#21584,#21585,#21586,#21587,
#21588,#21589,#21590,#21591,#21592,#21593,#21594,#21595,#21596,#21597,#21598,
#21599,#21600,#21601,#21602,#21603,#21604,#21605,#21606,#21607,#21608,#21609,
#21610,#21611,#21612,#21613,#21614,#21615,#21616),.UNSPECIFIED.,.F.,.F.,
(4,3,3,3,3,3,3,3,3,3,3,4),(0.00419407786743743,0.00785137040303032,0.00864322402522884,
0.00888216076442196,0.0105632172608223,0.0122879239665899,0.0130923701830202,
0.0136962196480357,0.0161859644983781,0.0187205501007953,0.021330966650845,
0.0219906624986031),.UNSPECIFIED.);
#552=B_SPLINE_CURVE_WITH_KNOTS('',3,(#21620,#21621,#21622,#21623,#21624,
#21625,#21626,#21627,#21628,#21629,#21630,#21631,#21632,#21633,#21634,#21635,
#21636,#21637,#21638,#21639,#21640,#21641,#21642,#21643,#21644,#21645,#21646,
#21647,#21648,#21649,#21650,#21651,#21652,#21653),.UNSPECIFIED.,.F.,.F.,
(4,3,3,3,3,3,3,3,3,3,3,4),(0.,0.00259497273971206,0.00513490948937697,0.00760920564921991,
0.00831654261042337,0.00892204401521714,0.010654177403752,0.0123507369864928,
0.0131434725515693,0.0133830660228257,0.0170412668230596,0.0178440880304343),
 .UNSPECIFIED.);
#553=B_SPLINE_CURVE_WITH_KNOTS('',3,(#21658,#21659,#21660,#21661,#21662,
#21663),.UNSPECIFIED.,.F.,.F.,(4,2,4),(0.,0.00327855488628777,0.00654795604494931),
 .UNSPECIFIED.);
#554=B_SPLINE_CURVE_WITH_KNOTS('',3,(#21674,#21675,#21676,#21677,#21678,
#21679),.UNSPECIFIED.,.F.,.F.,(4,2,4),(0.,0.00326940115867351,0.00654795604497327),
 .UNSPECIFIED.);
#555=B_SPLINE_CURVE_WITH_KNOTS('',3,(#21705,#21706,#21707,#21708,#21709,
#21710,#21711),.UNSPECIFIED.,.F.,.F.,(4,3,4),(0.,0.00700450431517081,0.00878441731503683),
 .UNSPECIFIED.);
#556=B_SPLINE_CURVE_WITH_KNOTS('',3,(#21724,#21725,#21726,#21727),
 .UNSPECIFIED.,.F.,.F.,(4,4),(0.,0.00906386388585899),.UNSPECIFIED.);
#557=B_SPLINE_CURVE_WITH_KNOTS('',3,(#21782,#21783,#21784,#21785,#21786,
#21787,#21788,#21789,#21790,#21791,#21792,#21793,#21794,#21795,#21796,#21797,
#21798,#21799,#21800,#21801,#21802,#21803,#21804,#21805,#21806,#21807,#21808,
#21809,#21810,#21811,#21812,#21813,#21814,#21815,#21816,#21817,#21818,#21819,
#21820,#21821,#21822,#21823,#21824,#21825,#21826,#21827,#21828,#21829,#21830),
 .UNSPECIFIED.,.F.,.F.,(4,3,3,3,3,3,3,3,3,3,3,3,3,3,3,3,4),(0.,0.000121245606178752,
0.000242857142425659,0.000287360877759076,0.000288270017838685,0.000443403913041565,
0.000574721755518153,0.000575971165655798,0.000665917057788043,0.000718402194397691,
0.00079024241383746,0.000826162523557345,0.000862082633277229,0.000975072145641835,
0.00100576307215677,0.00111728780497355,0.00114944351103631),
 .UNSPECIFIED.);
#558=B_SPLINE_CURVE_WITH_KNOTS('',3,(#21836,#21837,#21838,#21839,#21840,
#21841,#21842,#21843),.UNSPECIFIED.,.F.,.F.,(4,2,2,4),(0.,0.0138082473482012,
0.0207123710223018,0.0276164946964023),.UNSPECIFIED.);
#559=B_SPLINE_CURVE_WITH_KNOTS('',3,(#21853,#21854,#21855,#21856,#21857,
#21858,#21859,#21860,#21861,#21862,#21863,#21864,#21865,#21866,#21867,#21868,
#21869,#21870,#21871,#21872,#21873,#21874,#21875,#21876,#21877,#21878,#21879,
#21880,#21881,#21882,#21883,#21884,#21885,#21886),.UNSPECIFIED.,.F.,.F.,
(4,3,3,3,3,3,3,3,3,3,3,4),(0.,0.000110567770974224,0.000229163742141399,
0.000349602945008942,0.000466129197462143,0.00050396261230882,0.00050437055407879,
0.000654658246767277,0.000733772187615245,0.000861351750994649,0.000986409541178866,
0.00100874110815758),.UNSPECIFIED.);
#560=B_SPLINE_CURVE_WITH_KNOTS('',3,(#21903,#21904,#21905,#21906,#21907,
#21908,#21909,#21910,#21911,#21912,#21913,#21914,#21915,#21916,#21917,#21918,
#21919,#21920,#21921,#21922,#21923,#21924,#21925,#21926,#21927,#21928,#21929,
#21930),.UNSPECIFIED.,.F.,.F.,(4,3,3,3,3,3,3,3,3,4),(0.,9.61627041694446E-5,
0.000194643124010955,0.000263598431963752,0.000263909149293657,0.000510523427602487,
0.000527611135930373,0.000527818298587313,0.000791654292982851,0.00105563659717465),
 .UNSPECIFIED.);
#561=B_SPLINE_CURVE_WITH_KNOTS('',3,(#21936,#21937,#21938,#21939,#21940,
#21941,#21942,#21943,#21944,#21945,#21946,#21947,#21948,#21949,#21950,#21951),
 .UNSPECIFIED.,.F.,.F.,(4,3,3,3,3,4),(4.53150918211895E-15,0.0020152069145278,
0.00402253547199676,0.0060259524227816,0.00802370171969666,0.00993491157965328),
 .UNSPECIFIED.);
#562=B_SPLINE_CURVE_WITH_KNOTS('',3,(#21953,#21954,#21955,#21956,#21957,
#21958,#21959,#21960,#21961,#21962,#21963,#21964,#21965,#21966,#21967,#21968,
#21969,#21970,#21971,#21972,#21973,#21974,#21975,#21976,#21977,#21978,#21979,
#21980,#21981,#21982,#21983,#21984,#21985,#21986,#21987,#21988,#21989,#21990,
#21991,#21992,#21993,#21994,#21995),.UNSPECIFIED.,.F.,.F.,(4,3,3,3,3,3,
3,3,3,3,3,3,3,3,4),(0.,0.000142261508866842,0.000306612281910534,0.000354680426257011,
0.000354839578464814,0.000671890822871748,0.000709360852514021,0.00070979431964599,
0.000798030959078274,0.000931036118924653,0.00106404127877103,0.0011770719963786,
0.00124138149189954,0.00135612593306929,0.00141872170502804),
 .UNSPECIFIED.);
#563=B_SPLINE_CURVE_WITH_KNOTS('',3,(#22002,#22003,#22004,#22005,#22006,
#22007,#22008,#22009,#22010,#22011,#22012,#22013,#22014,#22015,#22016,#22017,
#22018,#22019,#22020,#22021,#22022,#22023,#22024,#22025,#22026,#22027,#22028,
#22029,#22030,#22031,#22032,#22033,#22034,#22035,#22036,#22037,#22038,#22039,
#22040,#22041,#22042,#22043,#22044,#22045,#22046,#22047,#22048,#22049,#22050,
#22051,#22052,#22053,#22054,#22055,#22056),.UNSPECIFIED.,.F.,.F.,(4,3,3,
3,3,3,3,3,3,3,3,3,3,3,3,3,3,3,4),(0.,0.00292798214826902,0.00577262065532403,
0.00682756145262549,0.00693335737727643,0.00947217443781762,0.0103475581420102,
0.0104000360659147,0.0118697041220001,0.0132773954673753,0.0138667147545529,
0.013878114522684,0.0166264516375164,0.0173333934431911,0.0189487413423672,
0.0205003989924343,0.021054043092682,0.0243937363006151,0.0277334295085482),
 .UNSPECIFIED.);
#564=B_SPLINE_CURVE_WITH_KNOTS('',3,(#22097,#22098,#22099,#22100,#22101,
#22102,#22103,#22104),.UNSPECIFIED.,.F.,.F.,(4,2,2,4),(0.,0.00951523528670844,
0.0142728529300627,0.0190304705734169),.UNSPECIFIED.);
#565=B_SPLINE_CURVE_WITH_KNOTS('',3,(#22108,#22109,#22110,#22111,#22112,
#22113,#22114,#22115),.UNSPECIFIED.,.F.,.F.,(4,2,2,4),(0.,0.00476132581272554,
0.00952265162545108,0.0190453032509022),.UNSPECIFIED.);
#566=B_SPLINE_CURVE_WITH_KNOTS('',3,(#22120,#22121,#22122,#22123,#22124,
#22125),.UNSPECIFIED.,.F.,.F.,(4,2,4),(0.,0.0032785548862878,0.00654795604494929),
 .UNSPECIFIED.);
#567=B_SPLINE_CURVE_WITH_KNOTS('',3,(#22136,#22137,#22138,#22139,#22140,
#22141),.UNSPECIFIED.,.F.,.F.,(4,2,4),(0.,0.00326940115867351,0.00654795604497326),
 .UNSPECIFIED.);
#568=B_SPLINE_CURVE_WITH_KNOTS('',3,(#22162,#22163,#22164,#22165,#22166,
#22167,#22168),.UNSPECIFIED.,.F.,.F.,(4,3,4),(1.73472347597681E-18,0.00700450431037659,
0.00878441731503682),.UNSPECIFIED.);
#569=B_SPLINE_CURVE_WITH_KNOTS('',3,(#22183,#22184,#22185,#22186),
 .UNSPECIFIED.,.F.,.F.,(4,4),(0.,0.009063863885859),.UNSPECIFIED.);
#570=B_SPLINE_CURVE_WITH_KNOTS('',3,(#22315,#22316,#22317,#22318,#22319,
#22320),.UNSPECIFIED.,.F.,.F.,(4,2,4),(0.,0.5,1.),.UNSPECIFIED.);
#571=B_SPLINE_CURVE_WITH_KNOTS('',3,(#22322,#22323,#22324,#22325,#22326,
#22327,#22328,#22329,#22330,#22331,#22332,#22333,#22334,#22335,#22336,#22337),
 .UNSPECIFIED.,.F.,.F.,(4,3,3,3,3,4),(0.,0.269515461283795,0.518490249146468,
0.759245124573234,0.982227995954739,1.),.UNSPECIFIED.);
#572=B_SPLINE_CURVE_WITH_KNOTS('',3,(#22338,#22339,#22340,#22341,#22342,
#22343),.UNSPECIFIED.,.F.,.F.,(4,2,4),(0.,0.5,1.),.UNSPECIFIED.);
#573=B_SPLINE_CURVE_WITH_KNOTS('',3,(#22408,#22409,#22410,#22411),
 .UNSPECIFIED.,.F.,.F.,(4,4),(0.,0.99999526872431),.UNSPECIFIED.);
#574=B_SPLINE_CURVE_WITH_KNOTS('',3,(#22413,#22414,#22415,#22416,#22417,
#22418),.UNSPECIFIED.,.F.,.F.,(4,2,4),(7.44333906889603E-6,0.5,1.),
 .UNSPECIFIED.);
#575=B_SPLINE_CURVE_WITH_KNOTS('',3,(#22419,#22420,#22421,#22422,#22423,
#22424),.UNSPECIFIED.,.F.,.F.,(4,2,4),(0.,0.5,1.),.UNSPECIFIED.);
#576=B_SPLINE_CURVE_WITH_KNOTS('',3,(#22473,#22474,#22475,#22476,#22477,
#22478,#22479,#22480,#22481,#22482,#22483,#22484,#22485,#22486,#22487,#22488),
 .UNSPECIFIED.,.F.,.F.,(4,3,3,3,3,4),(0.,0.2058948841142,0.424353797242841,
0.652795164048127,0.901134029685474,1.),.UNSPECIFIED.);
#577=B_SPLINE_CURVE_WITH_KNOTS('',3,(#22489,#22490,#22491,#22492,#22493,
#22494),.UNSPECIFIED.,.F.,.F.,(4,2,4),(0.,0.5,1.),.UNSPECIFIED.);
#578=B_SPLINE_CURVE_WITH_KNOTS('',3,(#22544,#22545,#22546,#22547,#22548,
#22549,#22550,#22551,#22552,#22553,#22554,#22555,#22556,#22557,#22558,#22559),
 .UNSPECIFIED.,.F.,.F.,(4,3,3,3,3,4),(0.,0.249999999999982,0.478354309316489,
0.695627207633627,0.902571772792554,0.999999999999926),.UNSPECIFIED.);
#579=B_SPLINE_CURVE_WITH_KNOTS('',3,(#22560,#22561,#22562,#22563,#22564,
#22565),.UNSPECIFIED.,.F.,.F.,(4,2,4),(0.,0.5,1.),.UNSPECIFIED.);
#580=B_SPLINE_CURVE_WITH_KNOTS('',3,(#22630,#22631,#22632,#22633,#22634,
#22635),.UNSPECIFIED.,.F.,.F.,(4,2,4),(0.,0.5,1.),.UNSPECIFIED.);
#581=B_SPLINE_CURVE_WITH_KNOTS('',3,(#22637,#22638,#22639,#22640,#22641,
#22642,#22643,#22644,#22645,#22646,#22647,#22648,#22649,#22650,#22651,#22652,
#22653,#22654,#22655,#22656,#22657,#22658,#22659,#22660,#22661,#22662,#22663,
#22664,#22665,#22666,#22667,#22668,#22669,#22670,#22671,#22672,#22673,#22674,
#22675,#22676,#22677,#22678,#22679,#22680,#22681,#22682,#22683,#22684,#22685,
#22686,#22687,#22688,#22689,#22690,#22691),.UNSPECIFIED.,.F.,.F.,(4,3,3,
3,3,3,3,3,3,3,3,3,3,3,3,3,3,3,4),(0.,0.134829595806097,0.3019357508242,
0.331938859566891,0.520486711309055,0.653948260259039,0.766867847735502,
0.847465247187294,0.903670142103914,0.941441061010362,0.964211312778628,
0.978961681102042,0.986981564546894,0.993490782273447,0.996745391136724,
0.998372695568362,0.999186347492603,0.999785290684486,0.999999999416845),
 .UNSPECIFIED.);
#582=B_SPLINE_CURVE_WITH_KNOTS('',3,(#22692,#22693,#22694,#22695,#22696,
#22697),.UNSPECIFIED.,.F.,.F.,(4,2,4),(0.,0.5,1.),.UNSPECIFIED.);
#583=B_SPLINE_CURVE_WITH_KNOTS('',3,(#22748,#22749,#22750,#22751,#22752,
#22753),.UNSPECIFIED.,.F.,.F.,(4,2,4),(0.,0.5,1.),.UNSPECIFIED.);
#584=B_SPLINE_CURVE_WITH_KNOTS('',3,(#22754,#22755,#22756,#22757,#22758,
#22759,#22760,#22761,#22762,#22763,#22764,#22765,#22766,#22767,#22768,#22769),
 .UNSPECIFIED.,.F.,.F.,(4,3,3,3,3,4),(0.,0.205894884114374,0.424353797243356,
0.652795164048942,0.901134029686469,1.),.UNSPECIFIED.);
#585=B_SPLINE_CURVE_WITH_KNOTS('',3,(#22770,#22771,#22772,#22773,#22774,
#22775),.UNSPECIFIED.,.F.,.F.,(4,2,4),(0.,0.5,1.),.UNSPECIFIED.);
#586=B_SPLINE_CURVE_WITH_KNOTS('',3,(#22825,#22826,#22827,#22828,#22829,
#22830,#22831,#22832,#22833,#22834,#22835,#22836,#22837,#22838,#22839,#22840),
 .UNSPECIFIED.,.F.,.F.,(4,3,3,3,3,4),(0.,0.25,0.478354309317608,0.695627207636338,
0.90257177279645,1.),.UNSPECIFIED.);
#587=B_SPLINE_CURVE_WITH_KNOTS('',3,(#22841,#22842,#22843,#22844,#22845,
#22846),.UNSPECIFIED.,.F.,.F.,(4,2,4),(0.,0.5,1.),.UNSPECIFIED.);
#588=B_SPLINE_CURVE_WITH_KNOTS('',3,(#22911,#22912,#22913,#22914,#22915,
#22916),.UNSPECIFIED.,.F.,.F.,(4,2,4),(0.,0.5,1.),.UNSPECIFIED.);
#589=B_SPLINE_CURVE_WITH_KNOTS('',3,(#22918,#22919,#22920,#22921),
 .UNSPECIFIED.,.F.,.F.,(4,4),(0.,1.),.UNSPECIFIED.);
#590=B_SPLINE_CURVE_WITH_KNOTS('',3,(#22922,#22923,#22924,#22925,#22926,
#22927),.UNSPECIFIED.,.F.,.F.,(4,2,4),(0.,0.5,1.),.UNSPECIFIED.);
#591=B_SPLINE_CURVE_WITH_KNOTS('',3,(#22988,#22989,#22990,#22991,#22992,
#22993,#22994,#22995,#22996,#22997,#22998,#22999,#23000),.UNSPECIFIED.,
 .F.,.F.,(4,3,3,3,4),(0.,0.223169250633758,0.461855220689223,0.714975201891676,
1.),.UNSPECIFIED.);
#592=B_SPLINE_CURVE_WITH_KNOTS('',3,(#23001,#23002,#23003,#23004,#23005,
#23006),.UNSPECIFIED.,.F.,.F.,(4,2,4),(0.,0.5,1.),.UNSPECIFIED.);
#593=B_SPLINE_CURVE_WITH_KNOTS('',3,(#23069,#23070,#23071,#23072,#23073,
#23074),.UNSPECIFIED.,.F.,.F.,(4,2,4),(0.,0.5,1.),.UNSPECIFIED.);
#594=B_SPLINE_CURVE_WITH_KNOTS('',3,(#23136,#23137,#23138,#23139,#23140,
#23141),.UNSPECIFIED.,.F.,.F.,(4,2,4),(0.,0.5,1.),.UNSPECIFIED.);
#595=B_SPLINE_CURVE_WITH_KNOTS('',3,(#23143,#23144,#23145,#23146,#23147,
#23148,#23149,#23150,#23151,#23152,#23153,#23154,#23155,#23156,#23157,#23158),
 .UNSPECIFIED.,.F.,.F.,(4,3,3,3,3,4),(0.,0.269515461284035,0.518490249146748,
0.759245124573374,0.982227995955184,1.),.UNSPECIFIED.);
#596=B_SPLINE_CURVE_WITH_KNOTS('',3,(#23159,#23160,#23161,#23162,#23163,
#23164),.UNSPECIFIED.,.F.,.F.,(4,2,4),(0.,0.5,1.),.UNSPECIFIED.);
#597=B_SPLINE_CURVE_WITH_KNOTS('',3,(#23229,#23230,#23231,#23232),
 .UNSPECIFIED.,.F.,.F.,(4,4),(0.,0.999995268720932),.UNSPECIFIED.);
#598=B_SPLINE_CURVE_WITH_KNOTS('',3,(#23234,#23235,#23236,#23237,#23238,
#23239),.UNSPECIFIED.,.F.,.F.,(4,2,4),(7.44334456133663E-6,0.5,1.),
 .UNSPECIFIED.);
#599=B_SPLINE_CURVE_WITH_KNOTS('',3,(#23240,#23241,#23242,#23243,#23244,
#23245),.UNSPECIFIED.,.F.,.F.,(4,2,4),(0.,0.5,1.),.UNSPECIFIED.);
#600=B_SPLINE_CURVE_WITH_KNOTS('',3,(#23294,#23295,#23296,#23297,#23298,
#23299,#23300,#23301,#23302,#23303,#23304,#23305,#23306,#23307,#23308,#23309),
 .UNSPECIFIED.,.F.,.F.,(4,3,3,3,3,4),(0.,0.205894884114519,0.424353797243679,
0.652795164049289,0.901134029687007,1.),.UNSPECIFIED.);
#601=B_SPLINE_CURVE_WITH_KNOTS('',3,(#23310,#23311,#23312,#23313,#23314,
#23315),.UNSPECIFIED.,.F.,.F.,(4,2,4),(0.,0.5,1.),.UNSPECIFIED.);
#602=B_SPLINE_CURVE_WITH_KNOTS('',3,(#23365,#23366,#23367,#23368,#23369,
#23370,#23371,#23372,#23373,#23374,#23375,#23376,#23377,#23378,#23379,#23380),
 .UNSPECIFIED.,.F.,.F.,(4,3,3,3,3,4),(0.,0.25,0.478354309316686,0.695627207634347,
0.902571772793475,1.),.UNSPECIFIED.);
#603=B_SPLINE_CURVE_WITH_KNOTS('',3,(#23381,#23382,#23383,#23384,#23385,
#23386),.UNSPECIFIED.,.F.,.F.,(4,2,4),(0.,0.5,1.),.UNSPECIFIED.);
#604=B_SPLINE_CURVE_WITH_KNOTS('',3,(#23451,#23452,#23453,#23454,#23455,
#23456),.UNSPECIFIED.,.F.,.F.,(4,2,4),(0.,0.5,1.),.UNSPECIFIED.);
#605=B_SPLINE_CURVE_WITH_KNOTS('',3,(#23458,#23459,#23460,#23461,#23462,
#23463,#23464,#23465,#23466,#23467,#23468,#23469,#23470,#23471,#23472,#23473,
#23474,#23475,#23476,#23477,#23478,#23479,#23480,#23481,#23482,#23483,#23484,
#23485,#23486,#23487,#23488,#23489,#23490,#23491,#23492,#23493,#23494,#23495,
#23496,#23497,#23498,#23499,#23500,#23501,#23502,#23503,#23504,#23505,#23506,
#23507,#23508,#23509,#23510,#23511,#23512),.UNSPECIFIED.,.F.,.F.,(4,3,3,
3,3,3,3,3,3,3,3,3,3,3,3,3,3,3,4),(0.,0.134829323934977,0.301935713922455,
0.331938859566998,0.520486828090896,0.653948260259002,0.765695413226449,
0.845739444745421,0.901726372988166,0.939310870056937,0.962010943846672,
0.977750863055006,0.9886476997431,0.993490782263339,0.99674539113167,0.998372695565835,
0.999186347491368,0.999785290683289,0.999999999416902),.UNSPECIFIED.);
#606=B_SPLINE_CURVE_WITH_KNOTS('',3,(#23513,#23514,#23515,#23516,#23517,
#23518),.UNSPECIFIED.,.F.,.F.,(4,2,4),(0.,0.5,1.),.UNSPECIFIED.);
#607=B_SPLINE_CURVE_WITH_KNOTS('',3,(#23569,#23570,#23571,#23572,#23573,
#23574),.UNSPECIFIED.,.F.,.F.,(4,2,4),(0.,0.5,1.),.UNSPECIFIED.);
#608=B_SPLINE_CURVE_WITH_KNOTS('',3,(#23575,#23576,#23577,#23578,#23579,
#23580,#23581,#23582,#23583,#23584,#23585,#23586,#23587,#23588,#23589,#23590),
 .UNSPECIFIED.,.F.,.F.,(4,3,3,3,3,4),(0.,0.205894884112877,0.424353797240785,
0.652795164045189,0.901134029682195,1.),.UNSPECIFIED.);
#609=B_SPLINE_CURVE_WITH_KNOTS('',3,(#23591,#23592,#23593,#23594,#23595,
#23596),.UNSPECIFIED.,.F.,.F.,(4,2,4),(0.,0.5,1.),.UNSPECIFIED.);
#610=B_SPLINE_CURVE_WITH_KNOTS('',3,(#23646,#23647,#23648,#23649,#23650,
#23651,#23652,#23653,#23654,#23655,#23656,#23657,#23658,#23659,#23660,#23661),
 .UNSPECIFIED.,.F.,.F.,(4,3,3,3,3,4),(0.,0.25,0.478354309316566,0.695627207633873,
0.902571772792968,1.),.UNSPECIFIED.);
#611=B_SPLINE_CURVE_WITH_KNOTS('',3,(#23662,#23663,#23664,#23665,#23666,
#23667),.UNSPECIFIED.,.F.,.F.,(4,2,4),(0.,0.5,1.),.UNSPECIFIED.);
#612=B_SPLINE_CURVE_WITH_KNOTS('',3,(#23732,#23733,#23734,#23735,#23736,
#23737),.UNSPECIFIED.,.F.,.F.,(4,2,4),(0.,0.5,1.),.UNSPECIFIED.);
#613=B_SPLINE_CURVE_WITH_KNOTS('',3,(#23739,#23740,#23741,#23742),
 .UNSPECIFIED.,.F.,.F.,(4,4),(0.,1.),.UNSPECIFIED.);
#614=B_SPLINE_CURVE_WITH_KNOTS('',3,(#23743,#23744,#23745,#23746,#23747,
#23748),.UNSPECIFIED.,.F.,.F.,(4,2,4),(0.,0.5,1.),.UNSPECIFIED.);
#615=B_SPLINE_CURVE_WITH_KNOTS('',3,(#23809,#23810,#23811,#23812,#23813,
#23814,#23815,#23816,#23817,#23818,#23819,#23820,#23821),.UNSPECIFIED.,
 .F.,.F.,(4,3,3,3,4),(0.,0.223169250633671,0.461855220688962,0.714975201891147,
1.),.UNSPECIFIED.);
#616=B_SPLINE_CURVE_WITH_KNOTS('',3,(#23822,#23823,#23824,#23825,#23826,
#23827),.UNSPECIFIED.,.F.,.F.,(4,2,4),(0.,0.5,1.),.UNSPECIFIED.);
#617=B_SPLINE_CURVE_WITH_KNOTS('',3,(#23890,#23891,#23892,#23893,#23894,
#23895),.UNSPECIFIED.,.F.,.F.,(4,2,4),(0.,0.5,1.),.UNSPECIFIED.);
#618=B_SPLINE_CURVE_WITH_KNOTS('',3,(#23908,#23909,#23910,#23911,#23912,
#23913,#23914,#23915,#23916,#23917,#23918,#23919,#23920,#23921,#23922,#23923,
#23924,#23925,#23926,#23927,#23928,#23929,#23930,#23931,#23932,#23933,#23934,
#23935,#23936,#23937,#23938,#23939,#23940,#23941,#23942,#23943,#23944,#23945,
#23946,#23947,#23948,#23949,#23950,#23951,#23952,#23953,#23954,#23955,#23956,
#23957,#23958,#23959,#23960,#23961,#23962,#23963,#23964,#23965,#23966,#23967,
#23968,#23969,#23970,#23971,#23972,#23973,#23974,#23975,#23976,#23977,#23978,
#23979,#23980,#23981,#23982,#23983),.UNSPECIFIED.,.F.,.F.,(4,3,3,3,3,3,
3,3,3,3,3,3,3,3,3,3,3,3,3,3,3,3,3,3,3,4),(0.,1.95383290192994E-5,4.88458225482484E-5,
6.3499569312723E-5,6.71630060038416E-5,7.26581610405195E-5,7.81533160771975E-5,
0.000107954788053304,0.000117229974115796,0.000122114556370621,0.000124319385320046,
0.000126388565843593,0.000156306632154395,0.000183190273141628,0.000195383290192993,
0.000210037036957468,0.000222859065376383,0.000260630252152872,0.000268336943281978,
0.000312613264308788,0.000345493122408439,0.000400681528988149,0.000461636530308903,
0.000526902227788225,0.000600651716916799,0.00062522616402666),
 .UNSPECIFIED.);
#619=B_SPLINE_CURVE_WITH_KNOTS('',3,(#24010,#24011,#24012,#24013,#24014,
#24015,#24016,#24017,#24018,#24019,#24020,#24021,#24022,#24023,#24024,#24025,
#24026,#24027,#24028,#24029,#24030,#24031,#24032,#24033,#24034,#24035,#24036,
#24037,#24038,#24039,#24040,#24041,#24042,#24043,#24044,#24045,#24046,#24047,
#24048,#24049,#24050,#24051,#24052,#24053,#24054,#24055,#24056,#24057,#24058,
#24059,#24060,#24061,#24062,#24063,#24064,#24065,#24066,#24067),
 .UNSPECIFIED.,.F.,.F.,(4,3,3,3,3,3,3,3,3,3,3,3,3,3,3,3,3,3,3,4),(0.,8.33528450034202E-5,
0.000157226441487617,0.000225533822547471,0.00028951662415279,0.000348414967230199,
0.000378847230940207,0.000425063895935628,0.000434497171244448,0.000472969202699083,
0.000509314375642632,0.000542883032634857,0.000568270846410307,0.000610359908966051,
0.000640506736109503,0.000662982654145361,0.000689264740462159,0.000715678191795904,
0.000742518573435838,0.000757694461880414),.UNSPECIFIED.);
#620=B_SPLINE_CURVE_WITH_KNOTS('',3,(#24131,#24132,#24133,#24134,#24135,
#24136,#24137,#24138,#24139,#24140,#24141,#24142,#24143,#24144,#24145,#24146,
#24147,#24148,#24149,#24150,#24151,#24152,#24153,#24154,#24155),
 .UNSPECIFIED.,.F.,.F.,(4,3,3,3,3,3,3,3,4),(0.,8.77855222411457E-5,0.000180911661749747,
0.000284642473054724,0.000399672366761005,0.000487602524799653,0.000496563116819161,
0.000792478626183723,0.000993116632308356),.UNSPECIFIED.);
#621=B_SPLINE_CURVE_WITH_KNOTS('',3,(#24186,#24187,#24188,#24189,#24190,
#24191,#24192,#24193,#24194,#24195,#24196,#24197,#24198,#24199,#24200,#24201,
#24202,#24203,#24204,#24205,#24206,#24207,#24208,#24209,#24210),
 .UNSPECIFIED.,.F.,.F.,(4,3,3,3,3,3,3,3,4),(9.46798387615072E-9,0.000265027614959612,
0.000494820327889037,0.000505114957780789,0.000628257448099428,0.000739957890430424,
0.00084406403792606,0.000940011289227427,0.000989640655778074),
 .UNSPECIFIED.);
#622=B_SPLINE_CURVE_WITH_KNOTS('',3,(#24211,#24212,#24213,#24214,#24215,
#24216),.UNSPECIFIED.,.F.,.F.,(4,2,4),(7.44333395304289E-6,0.5,1.),
 .UNSPECIFIED.);
#623=B_SPLINE_CURVE_WITH_KNOTS('',3,(#24268,#24269,#24270,#24271,#24272,
#24273,#24274,#24275,#24276,#24277,#24278,#24279,#24280,#24281,#24282,#24283,
#24284,#24285,#24286,#24287,#24288,#24289,#24290,#24291,#24292,#24293,#24294,
#24295,#24296,#24297,#24298,#24299,#24300,#24301,#24302,#24303,#24304,#24305,
#24306,#24307,#24308,#24309,#24310,#24311,#24312,#24313,#24314,#24315,#24316,
#24317,#24318,#24319),.UNSPECIFIED.,.F.,.F.,(4,3,3,3,3,3,3,3,3,3,3,3,3,
3,3,3,3,4),(0.,4.1276445995066E-5,8.42546564931361E-5,0.000129571564840061,
0.000139714696155289,0.00019740107551137,0.000258094770764446,0.000279429392310577,
0.000359695196555143,0.000442730223930049,0.000529248927812506,0.000558858784621132,
0.000667945714892336,0.000780388678479812,0.000891339019476349,0.0010045282943593,
0.00110832362887639,0.00111771756924224),.UNSPECIFIED.);
#624=B_SPLINE_CURVE_WITH_KNOTS('',3,(#24386,#24387,#24388,#24389,#24390,
#24391,#24392,#24393,#24394,#24395,#24396,#24397,#24398,#24399,#24400,#24401,
#24402,#24403,#24404,#24405,#24406,#24407,#24408,#24409,#24410,#24411,#24412,
#24413,#24414,#24415,#24416,#24417,#24418,#24419,#24420,#24421,#24422,#24423,
#24424,#24425,#24426,#24427,#24428,#24429,#24430,#24431,#24432,#24433,#24434,
#24435,#24436,#24437,#24438,#24439,#24440),.UNSPECIFIED.,.F.,.F.,(4,3,3,
3,3,3,3,3,3,3,3,3,3,3,3,3,3,3,4),(1.00003361382536E-7,0.000627368768300138,
0.00125605092262165,0.00251210184524329,0.00502420369048659,0.013553717306397,
0.023404944736136,0.0239781242527868,0.0394341509419622,0.0631200523923673,
0.106735413774525,0.174618556157698,0.276325871435081,0.346051748925113,
0.519710818552453,0.668061140433113,0.834030570216557,0.968862390059979,
1.),.UNSPECIFIED.);
#625=B_SPLINE_CURVE_WITH_KNOTS('',3,(#24474,#24475,#24476,#24477,#24478,
#24479,#24480,#24481,#24482,#24483,#24484,#24485,#24486,#24487,#24488,#24489,
#24490,#24491,#24492,#24493,#24494,#24495,#24496,#24497,#24498,#24499,#24500,
#24501,#24502,#24503,#24504,#24505,#24506,#24507,#24508,#24509,#24510,#24511,
#24512,#24513,#24514,#24515,#24516,#24517,#24518,#24519),.UNSPECIFIED.,
 .F.,.F.,(4,3,3,3,3,3,3,3,3,3,3,3,3,3,3,4),(0.,9.72968081736543E-5,0.000188076340042391,
0.000274624933132362,0.000355070980215829,0.000389187232694617,0.000449617363167268,
0.000507814172801453,0.000562918686627687,0.000583780849041926,0.00062425089166696,
0.000662781785097529,0.000699618916511921,0.000735289518531963,0.000769568105219451,
0.000778374465389236),.UNSPECIFIED.);
#626=B_SPLINE_CURVE_WITH_KNOTS('',3,(#24523,#24524,#24525,#24526,#24527,
#24528,#24529,#24530,#24531,#24532,#24533,#24534,#24535,#24536,#24537,#24538,
#24539,#24540,#24541,#24542,#24543,#24544,#24545,#24546,#24547,#24548,#24549,
#24550,#24551,#24552,#24553,#24554,#24555,#24556),.UNSPECIFIED.,.F.,.F.,
(4,3,3,3,3,3,3,3,3,3,3,4),(0.,6.4784657425023E-5,0.000128085038055946,0.00019334280002843,
0.000254275817474415,0.000258600562000915,0.000269706482902608,0.000323662397377516,
0.000382521450096718,0.000443803383543172,0.00050542857129966,0.000539412965805216),
 .UNSPECIFIED.);
#627=B_SPLINE_CURVE_WITH_KNOTS('',3,(#24569,#24570,#24571,#24572,#24573,
#24574,#24575,#24576,#24577,#24578,#24579,#24580),.UNSPECIFIED.,.F.,.F.,
(4,2,2,2,2,4),(9.94226249721363E-9,0.000325172939224849,0.000650345878449699,
0.000975518817674548,0.00113810528728698,0.0013006917568994),
 .UNSPECIFIED.);
#628=B_SPLINE_CURVE_WITH_KNOTS('',3,(#24634,#24635,#24636,#24637,#24638,
#24639,#24640,#24641,#24642,#24643,#24644,#24645),.UNSPECIFIED.,.F.,.F.,
(4,2,2,2,2,4),(9.94226628845883E-9,0.000325172939224847,0.000650345878449693,
0.00097551881767454,0.00113810528728697,0.00130069175689939),
 .UNSPECIFIED.);
#629=B_SPLINE_CURVE_WITH_KNOTS('',3,(#24714,#24715,#24716,#24717,#24718,
#24719,#24720,#24721,#24722,#24723,#24724,#24725,#24726,#24727,#24728,#24729,
#24730,#24731,#24732,#24733,#24734,#24735,#24736,#24737,#24738),
 .UNSPECIFIED.,.F.,.F.,(4,3,3,3,3,3,3,3,4),(0.,9.58519120578613E-5,0.000201048393011152,
0.000313533962690052,0.000443358794827932,0.000487856029895832,0.000498221418747222,
0.000765061137597118,0.000996433304434568),.UNSPECIFIED.);
#630=B_SPLINE_CURVE_WITH_KNOTS('',3,(#24771,#24772,#24773,#24774,#24775,
#24776,#24777,#24778,#24779,#24780,#24781,#24782,#24783,#24784,#24785,#24786,
#24787,#24788,#24789,#24790,#24791,#24792,#24793,#24794,#24795),
 .UNSPECIFIED.,.F.,.F.,(4,3,3,3,3,3,3,3,4),(0.,8.88404632360193E-5,0.000183111749600284,
0.000288167720068051,0.000405111512909157,0.000488005422625335,0.000496805101503793,
0.000790206339202793,0.000993600597453218),.UNSPECIFIED.);
#631=B_SPLINE_CURVE_WITH_KNOTS('',3,(#24882,#24883,#24884,#24885,#24886,
#24887,#24888,#24889,#24890,#24891,#24892,#24893,#24894,#24895,#24896,#24897,
#24898,#24899,#24900,#24901,#24902,#24903,#24904,#24905,#24906,#24907,#24908,
#24909,#24910,#24911,#24912,#24913,#24914,#24915,#24916,#24917,#24918,#24919,
#24920,#24921,#24922,#24923,#24924,#24925,#24926,#24927,#24928,#24929,#24930,
#24931,#24932,#24933),.UNSPECIFIED.,.F.,.F.,(4,3,3,3,3,3,3,3,3,3,3,3,3,
3,3,3,3,4),(0.,4.12764459950958E-5,8.42546564931839E-5,0.000129571564840137,
0.000139714696155272,0.000197401075511458,0.000258094770764663,0.000279429392310544,
0.000359695196555155,0.0004427302239301,0.000529248927812585,0.000558858784621111,
0.000667945714892309,0.000780388678479793,0.000891339019476335,0.00100452829435929,
0.0011083236288764,0.00111771756924224),.UNSPECIFIED.);
#632=B_SPLINE_CURVE_WITH_KNOTS('',3,(#24965,#24966,#24967,#24968,#24969,
#24970,#24971,#24972,#24973,#24974,#24975,#24976,#24977,#24978,#24979,#24980,
#24981,#24982,#24983,#24984,#24985,#24986,#24987,#24988,#24989,#24990,#24991,
#24992,#24993,#24994,#24995,#24996,#24997,#24998,#24999,#25000,#25001,#25002,
#25003,#25004,#25005,#25006,#25007,#25008,#25009,#25010,#25011,#25012,#25013,
#25014,#25015,#25016,#25017,#25018,#25019,#25020,#25021,#25022,#25023,#25024,
#25025,#25026,#25027,#25028),.UNSPECIFIED.,.F.,.F.,(4,3,3,3,3,3,3,3,3,3,
3,3,3,3,3,3,3,3,3,3,3,4),(0.,9.68515416477823E-5,0.000192020529402715,0.000279284320016411,
0.00036189847675362,0.000438321326769842,0.000477527492667515,0.000529607759318425,
0.000578407666764912,0.000625243185949314,0.000670767212475296,0.000713433961486794,
0.000716291239001278,0.0007544629939221,0.000791422812842767,0.000826961927143274,
0.00083567311216816,0.000863826223827008,0.000892456091105036,0.000921613281236568,
0.000951948647270463,0.000955054985335042),.UNSPECIFIED.);
#633=B_SPLINE_CURVE_WITH_KNOTS('',3,(#25034,#25035,#25036,#25037,#25038,
#25039,#25040,#25041,#25042,#25043,#25044,#25045,#25046,#25047,#25048,#25049,
#25050,#25051,#25052,#25053,#25054,#25055,#25056,#25057,#25058,#25059,#25060,
#25061,#25062,#25063,#25064,#25065,#25066,#25067,#25068,#25069,#25070,#25071,
#25072,#25073,#25074,#25075,#25076,#25077,#25078,#25079),.UNSPECIFIED.,
 .F.,.F.,(4,3,3,3,3,3,3,3,3,3,3,3,3,3,3,4),(0.,7.40646428061214E-5,0.000146779369918774,
0.000164860955696857,0.000232495741978612,0.000300130528260368,0.000322950277848782,
0.000361000159968374,0.000375163160325465,0.000412679476358013,0.000450195792390562,
0.000468403009741517,0.000509319401675059,0.000549287864653555,0.000588177998696803,
0.000600261056520756),.UNSPECIFIED.);
#634=B_SPLINE_CURVE_WITH_KNOTS('',3,(#25094,#25095,#25096,#25097,#25098,
#25099,#25100,#25101,#25102,#25103,#25104,#25105,#25106,#25107,#25108,#25109,
#25110,#25111,#25112,#25113,#25114,#25115,#25116,#25117,#25118,#25119,#25120,
#25121,#25122,#25123,#25124,#25125,#25126,#25127,#25128,#25129,#25130,#25131,
#25132,#25133,#25134,#25135,#25136,#25137,#25138,#25139,#25140,#25141,#25142,
#25143,#25144,#25145,#25146,#25147,#25148,#25149,#25150,#25151,#25152,#25153,
#25154),.UNSPECIFIED.,.F.,.F.,(4,3,3,3,3,3,3,3,3,3,3,3,3,3,3,3,3,3,3,3,
4),(0.,3.01683521755624E-5,5.95123638943077E-5,8.83024180022877E-5,0.00011676839189743,
0.00012067340870225,0.000156899735255077,0.000194095346003556,0.000232946053825429,
0.000241346817404499,0.00028483712090787,0.000330243027192198,0.000378792539153568,
0.000430743086981298,0.000482693634809027,0.000560072810733523,0.000642027313860096,
0.00073189117824408,0.000825743849904349,0.000923569286423716,0.000965387269618084),
 .UNSPECIFIED.);
#635=B_SPLINE_CURVE_WITH_KNOTS('',3,(#25274,#25275,#25276,#25277,#25278,
#25279,#25280,#25281,#25282,#25283,#25284,#25285,#25286,#25287,#25288,#25289,
#25290,#25291,#25292,#25293,#25294,#25295,#25296,#25297,#25298,#25299,#25300,
#25301,#25302,#25303,#25304,#25305,#25306,#25307,#25308,#25309,#25310),
 .UNSPECIFIED.,.F.,.F.,(4,3,3,3,3,3,3,3,3,3,3,3,4),(0.,6.99403169130158E-5,
0.00013663881220017,0.00019323995121994,0.000204958218300255,0.000257951721023207,
0.00027327762440034,0.000285453692681066,0.000346137712528328,0.000408654588979332,
0.000472636894880584,0.000539340363922078,0.000546555248800679),
 .UNSPECIFIED.);
#636=B_SPLINE_CURVE_WITH_KNOTS('',3,(#25387,#25388,#25389,#25390,#25391,
#25392,#25393,#25394,#25395,#25396,#25397,#25398,#25399,#25400,#25401,#25402,
#25403,#25404,#25405,#25406,#25407,#25408,#25409,#25410,#25411,#25412,#25413,
#25414,#25415,#25416,#25417,#25418,#25419,#25420,#25421,#25422,#25423,#25424,
#25425,#25426,#25427,#25428,#25429,#25430,#25431,#25432,#25433,#25434,#25435,
#25436,#25437,#25438,#25439,#25440,#25441,#25442,#25443,#25444,#25445,#25446,
#25447,#25448,#25449,#25450,#25451,#25452,#25453,#25454,#25455,#25456,#25457,
#25458,#25459,#25460,#25461,#25462),.UNSPECIFIED.,.F.,.F.,(4,3,3,3,3,3,
3,3,3,3,3,3,3,3,3,3,3,3,3,3,3,3,3,3,3,4),(1.90409143160226E-17,1.95383290192995E-5,
4.88458225482488E-5,6.34995693127234E-5,6.71630060038421E-5,7.26581610405201E-5,
7.8153316077198E-5,0.000107954788056933,0.000117229974115797,0.000122114556370622,
0.00012431938532005,0.000126388565843594,0.000156306632154396,0.000183190273141605,
0.000195383290192993,0.000210037036957467,0.000222859065376382,0.000260630252152406,
0.000268336943281981,0.000312613264308786,0.000345493122480558,0.000400681529065493,
0.000461636530392023,0.000526902227878309,0.000600651717012678,0.000625226164026665),
 .UNSPECIFIED.);
#637=B_SPLINE_CURVE_WITH_KNOTS('',3,(#25476,#25477,#25478,#25479,#25480,
#25481,#25482,#25483,#25484,#25485,#25486,#25487,#25488,#25489,#25490,#25491,
#25492,#25493,#25494,#25495,#25496,#25497,#25498,#25499,#25500,#25501,#25502,
#25503,#25504,#25505,#25506,#25507,#25508,#25509,#25510,#25511,#25512,#25513,
#25514,#25515,#25516,#25517,#25518,#25519,#25520,#25521,#25522,#25523,#25524,
#25525,#25526,#25527,#25528,#25529,#25530,#25531,#25532,#25533,#25534,#25535,
#25536,#25537,#25538,#25539,#25540,#25541,#25542,#25543,#25544,#25545,#25546,
#25547,#25548,#25549,#25550,#25551),.UNSPECIFIED.,.F.,.F.,(4,3,3,3,3,3,
3,3,3,3,3,3,3,3,3,3,3,3,3,3,3,3,3,3,3,4),(0.,1.95383290192989E-5,4.88458225482473E-5,
6.34995693127215E-5,6.71630060038401E-5,7.26581610405179E-5,7.81533160771957E-5,
0.000107954788054619,0.000117229974115794,0.000122114556370618,0.000124319385320053,
0.00012638856584359,0.000156306632154391,0.000183190273142427,0.000195383290192988,
0.000210037036957462,0.000222859065376376,0.000260630252155243,0.000268336943281989,
0.000312613264308778,0.000345493122395937,0.000400681528975873,0.00046163653029605,
0.00052690222777407,0.000600651716897933,0.000625226163983449),
 .UNSPECIFIED.);
#638=B_SPLINE_CURVE_WITH_KNOTS('',3,(#25586,#25587,#25588,#25589,#25590,
#25591,#25592,#25593,#25594,#25595,#25596,#25597,#25598,#25599,#25600,#25601,
#25602,#25603,#25604,#25605,#25606,#25607,#25608,#25609,#25610,#25611,#25612,
#25613,#25614,#25615,#25616,#25617,#25618,#25619,#25620,#25621,#25622,#25623,
#25624,#25625,#25626,#25627,#25628,#25629,#25630,#25631),.UNSPECIFIED.,
 .F.,.F.,(4,3,3,3,3,3,3,3,3,3,3,3,3,3,3,4),(0.,3.50262368530255E-5,7.11751710414925E-5,
0.000109339082869859,0.000148762751082846,0.000189988996389714,0.000198220556017289,
0.000254911247280624,0.000313675244695655,0.00037559496150714,0.000396441112034577,
0.000477792055759519,0.000566506458105226,0.00065905994774777,0.000755430891867985,
0.000792882224069153),.UNSPECIFIED.);
#639=B_SPLINE_CURVE_WITH_KNOTS('',3,(#25657,#25658,#25659,#25660,#25661,
#25662,#25663,#25664,#25665,#25666,#25667,#25668,#25669,#25670,#25671,#25672,
#25673,#25674,#25675,#25676,#25677,#25678,#25679,#25680,#25681,#25682,#25683,
#25684,#25685,#25686,#25687,#25688,#25689,#25690,#25691,#25692,#25693,#25694,
#25695,#25696,#25697,#25698,#25699,#25700,#25701,#25702,#25703,#25704,#25705,
#25706,#25707,#25708,#25709,#25710,#25711,#25712,#25713,#25714),
 .UNSPECIFIED.,.F.,.F.,(4,3,3,3,3,3,3,3,3,3,3,3,3,3,3,3,3,3,3,4),(0.,8.33528450008425E-5,
0.000157226441485683,0.000225533822544734,0.000289516624149074,0.000348414967225308,
0.000378847230940205,0.000425063895934943,0.000434497171244511,0.000472969202698466,
0.000509314375641268,0.000542883032632685,0.000568270846410303,0.000610359908966047,
0.000640506736108079,0.000662982654145355,0.000689264740462126,0.000715678191795885,
0.000742518573435992,0.000757694461880407),.UNSPECIFIED.);
#640=B_SPLINE_CURVE_WITH_KNOTS('',3,(#25764,#25765,#25766,#25767,#25768,
#25769,#25770,#25771,#25772,#25773,#25774,#25775,#25776,#25777,#25778,#25779,
#25780,#25781,#25782,#25783,#25784,#25785,#25786,#25787,#25788,#25789,#25790,
#25791,#25792,#25793,#25794,#25795,#25796,#25797,#25798,#25799,#25800,#25801,
#25802,#25803,#25804,#25805,#25806,#25807,#25808,#25809,#25810,#25811,#25812,
#25813,#25814,#25815,#25816,#25817,#25818,#25819,#25820,#25821),
 .UNSPECIFIED.,.F.,.F.,(4,3,3,3,3,3,3,3,3,3,3,3,3,3,3,3,3,3,3,4),(0.,8.3352844998188E-5,
0.000157226441483691,0.000225533822540938,0.000289516624143318,0.00034841496721732,
0.0003788472309402,0.000425063895934259,0.000434497171244525,0.000472969202698661,
0.000509314375641677,0.000542883032633348,0.000568270846410307,0.000610359908966059,
0.000640506736109255,0.000662982654145359,0.00068926474046212,0.000715678191795907,
0.000742518573436032,0.000757694461880412),.UNSPECIFIED.);
#641=B_SPLINE_CURVE_WITH_KNOTS('',3,(#25855,#25856,#25857,#25858,#25859,
#25860,#25861,#25862,#25863,#25864,#25865,#25866,#25867,#25868,#25869,#25870,
#25871,#25872,#25873,#25874,#25875,#25876,#25877,#25878,#25879,#25880,#25881,
#25882,#25883,#25884,#25885,#25886,#25887,#25888,#25889,#25890,#25891,#25892,
#25893,#25894,#25895,#25896,#25897,#25898,#25899,#25900),.UNSPECIFIED.,
 .F.,.F.,(4,3,3,3,3,3,3,3,3,3,3,3,3,3,3,4),(0.,7.40646428067027E-5,0.00014677936992103,
0.000164860955696577,0.000232495741978471,0.000300130528260365,0.000322950277848778,
0.000361000159970521,0.000375163160325462,0.00041267947635801,0.000450195792390558,
0.000468403009741581,0.000509319401678437,0.000549287864660548,0.000588177998707373,
0.000600261056520751),.UNSPECIFIED.);
#642=B_SPLINE_CURVE_WITH_KNOTS('',3,(#25935,#25936,#25937,#25938,#25939,
#25940,#25941,#25942,#25943,#25944,#25945,#25946,#25947,#25948,#25949,#25950,
#25951,#25952,#25953,#25954,#25955,#25956,#25957,#25958,#25959,#25960,#25961,
#25962,#25963,#25964,#25965,#25966,#25967,#25968,#25969,#25970,#25971,#25972,
#25973,#25974,#25975,#25976,#25977,#25978,#25979,#25980),.UNSPECIFIED.,
 .F.,.F.,(4,3,3,3,3,3,3,3,3,3,3,3,3,3,3,4),(0.,4.01784152582232E-5,8.11318192707994E-5,
0.000123430231631933,0.00013379748131031,0.000151845918076035,0.000189807397595043,
0.000231866097105714,0.000275906952597149,0.000281134062468639,0.000303691836152069,
0.000372309715976617,0.000440927595801166,0.000514103167127634,0.000588539200903764,
0.000607383672304138),.UNSPECIFIED.);
#643=B_SPLINE_CURVE_WITH_KNOTS('',3,(#26033,#26034,#26035,#26036,#26037,
#26038,#26039,#26040,#26041,#26042,#26043,#26044,#26045,#26046,#26047,#26048,
#26049,#26050,#26051,#26052,#26053,#26054,#26055,#26056,#26057),
 .UNSPECIFIED.,.F.,.F.,(4,3,3,3,3,3,3,3,4),(0.,8.78783823229168E-5,0.000181106371765768,
0.000284958381202673,0.000400167490967761,0.000487646104112346,0.000496588354691666,
0.000792223039523606,0.000993167107609097),.UNSPECIFIED.);
#644=B_SPLINE_CURVE_WITH_KNOTS('',3,(#26088,#26089,#26090,#26091,#26092,
#26093,#26094,#26095,#26096,#26097,#26098,#26099,#26100,#26101,#26102,#26103,
#26104,#26105,#26106,#26107,#26108,#26109,#26110,#26111,#26112),
 .UNSPECIFIED.,.F.,.F.,(4,3,3,3,3,3,3,3,4),(9.46798652745075E-9,0.000265027615065046,
0.000494820327888722,0.00050511495778071,0.000628257448094622,0.000739957890426431,
0.000844064037925376,0.000940011289231895,0.000989640655777444),
 .UNSPECIFIED.);
#645=B_SPLINE_CURVE_WITH_KNOTS('',3,(#26113,#26114,#26115,#26116,#26117,
#26118),.UNSPECIFIED.,.F.,.F.,(4,2,4),(7.44334043044855E-6,0.5,1.),
 .UNSPECIFIED.);
#646=B_SPLINE_CURVE_WITH_KNOTS('',3,(#26251,#26252,#26253,#26254,#26255,
#26256,#26257,#26258,#26259,#26260,#26261,#26262,#26263,#26264,#26265,#26266,
#26267,#26268,#26269,#26270,#26271,#26272,#26273,#26274,#26275,#26276,#26277,
#26278,#26279,#26280,#26281,#26282,#26283,#26284,#26285,#26286,#26287,#26288,
#26289,#26290,#26291,#26292,#26293,#26294,#26295,#26296,#26297,#26298,#26299,
#26300,#26301,#26302,#26303,#26304,#26305),.UNSPECIFIED.,.F.,.F.,(4,3,3,
3,3,3,3,3,3,3,3,3,3,3,3,3,3,3,4),(1.00003366271743E-7,0.000627368764008543,
0.00125605094111647,0.00251210188223294,0.00502420376446587,0.0136336598992699,
0.0252314310431504,0.0410681024056911,0.0681502020062923,0.113858415357405,
0.184994129390117,0.291968963770629,0.346051748925135,0.51971092269832,
0.668061140433059,0.82760635706631,0.964639961031585,0.987151573699562,
1.),.UNSPECIFIED.);
#647=B_SPLINE_CURVE_WITH_KNOTS('',3,(#26339,#26340,#26341,#26342,#26343,
#26344,#26345,#26346,#26347,#26348,#26349,#26350,#26351,#26352,#26353,#26354,
#26355,#26356,#26357,#26358,#26359,#26360,#26361,#26362,#26363,#26364,#26365,
#26366,#26367,#26368,#26369,#26370,#26371,#26372,#26373,#26374,#26375,#26376,
#26377,#26378,#26379,#26380,#26381,#26382,#26383,#26384),.UNSPECIFIED.,
 .F.,.F.,(4,3,3,3,3,3,3,3,3,3,3,3,3,3,3,4),(0.,9.7296808173656E-5,0.000188076340040901,
0.000274624933129628,0.000355070980212206,0.000389187232694624,0.000449617363166583,
0.000507814172800233,0.000562918686626053,0.000583780849041926,0.000624250891657903,
0.000662781785090734,0.000699618916497541,0.000735289518509887,0.000769568105189037,
0.000778374465389229),.UNSPECIFIED.);
#648=B_SPLINE_CURVE_WITH_KNOTS('',3,(#26388,#26389,#26390,#26391,#26392,
#26393,#26394,#26395,#26396,#26397,#26398,#26399,#26400,#26401,#26402,#26403,
#26404,#26405,#26406,#26407,#26408,#26409,#26410,#26411,#26412,#26413,#26414,
#26415,#26416,#26417,#26418,#26419,#26420,#26421),.UNSPECIFIED.,.F.,.F.,
(4,3,3,3,3,3,3,3,3,3,3,4),(0.,6.47846574208782E-5,0.000128085038048596,
0.000193342800024759,0.000254275817470981,0.000258600562000923,0.000269706482902613,
0.000323662397375826,0.000382521450093377,0.000443803383538095,0.00050542857129258,
0.000539412965805225),.UNSPECIFIED.);
#649=B_SPLINE_CURVE_WITH_KNOTS('',3,(#26425,#26426,#26427,#26428,#26429,
#26430,#26431,#26432,#26433,#26434,#26435,#26436,#26437,#26438,#26439,#26440,
#26441,#26442,#26443,#26444,#26445,#26446,#26447,#26448,#26449,#26450,#26451,
#26452,#26453,#26454,#26455,#26456,#26457,#26458,#26459,#26460,#26461,#26462,
#26463,#26464,#26465,#26466,#26467,#26468,#26469,#26470),.UNSPECIFIED.,
 .F.,.F.,(4,3,3,3,3,3,3,3,3,3,3,3,3,3,3,4),(0.,7.33096139802609E-5,0.00014538886142587,
0.000163772356053824,0.000231283930773087,0.00029879550549235,0.00032102040376583,
0.000359079183382255,0.000373494381865439,0.000410843820051984,0.000448193258238528,
0.000465950705574258,0.000507344602018312,0.000547782593938721,0.00058711828767304,
0.000597591010984707),.UNSPECIFIED.);
#650=B_SPLINE_CURVE_WITH_KNOTS('',3,(#26478,#26479,#26480,#26481,#26482,
#26483,#26484,#26485,#26486,#26487,#26488,#26489,#26490,#26491,#26492,#26493,
#26494,#26495,#26496,#26497,#26498,#26499,#26500,#26501,#26502,#26503,#26504,
#26505,#26506,#26507,#26508,#26509,#26510,#26511),.UNSPECIFIED.,.F.,.F.,
(4,3,3,3,3,3,3,3,3,3,3,4),(0.,6.47846574211507E-5,0.000128085038050523,
0.000193342800025718,0.000254275817473748,0.000258600562000914,0.000269706482902609,
0.000323662397372321,0.000382521450086426,0.000443803383527674,0.00050542857127833,
0.000539412965805219),.UNSPECIFIED.);
#651=B_SPLINE_CURVE_WITH_KNOTS('',3,(#26527,#26528,#26529,#26530,#26531,
#26532,#26533,#26534,#26535,#26536,#26537,#26538),.UNSPECIFIED.,.F.,.F.,
(4,2,2,2,2,4),(9.94226663611176E-9,0.00032517293922485,0.0006503458784497,
0.00097551881767455,0.00113810528728698,0.0013006917568994),
 .UNSPECIFIED.);
#652=B_SPLINE_CURVE_WITH_KNOTS('',3,(#26686,#26687,#26688,#26689,#26690,
#26691,#26692,#26693,#26694,#26695,#26696,#26697,#26698,#26699,#26700,#26701,
#26702,#26703,#26704,#26705,#26706,#26707,#26708,#26709,#26710,#26711,#26712,
#26713,#26714,#26715,#26716,#26717,#26718,#26719,#26720,#26721,#26722,#26723,
#26724,#26725,#26726,#26727,#26728,#26729,#26730,#26731,#26732,#26733,#26734,
#26735,#26736,#26737),.UNSPECIFIED.,.F.,.F.,(4,3,3,3,3,3,3,3,3,3,3,3,3,
3,3,3,3,4),(0.,4.12764459949069E-5,8.42546564927975E-5,0.000129571564839558,
0.000139714696155275,0.000197401075511389,0.000258094770764511,0.000279429392310549,
0.000359695196555218,0.00044273022393022,0.000529248927812781,0.000558858784621119,
0.000667945714892313,0.000780388678479799,0.000891339019476329,0.00100452829435929,
0.00110832362887638,0.00111771756924225),.UNSPECIFIED.);
#653=B_SPLINE_CURVE_WITH_KNOTS('',3,(#26769,#26770,#26771,#26772,#26773,
#26774,#26775,#26776,#26777,#26778,#26779,#26780,#26781,#26782,#26783,#26784,
#26785,#26786,#26787,#26788,#26789,#26790,#26791,#26792,#26793,#26794,#26795,
#26796,#26797,#26798,#26799,#26800,#26801,#26802,#26803,#26804,#26805,#26806,
#26807,#26808,#26809,#26810,#26811,#26812,#26813,#26814,#26815,#26816,#26817,
#26818,#26819,#26820,#26821,#26822,#26823,#26824,#26825,#26826,#26827,#26828,
#26829,#26830,#26831,#26832),.UNSPECIFIED.,.F.,.F.,(4,3,3,3,3,3,3,3,3,3,
3,3,3,3,3,3,3,3,3,3,3,4),(0.,9.68515416480563E-5,0.000192020529402926,0.000279284320016308,
0.000361898476753293,0.000438321326769534,0.000477527492667534,0.00052960775931866,
0.000578407666765381,0.000625243185950011,0.00067076721247565,0.000713433961487206,
0.000716291239001288,0.000754462993922578,0.000791422812843817,0.000826961927144892,
0.000835673112168161,0.000863826223827739,0.000892456091106298,0.000921613281238493,
0.000951948647272746,0.000955054985335033),.UNSPECIFIED.);
#654=B_SPLINE_CURVE_WITH_KNOTS('',3,(#26841,#26842,#26843,#26844,#26845,
#26846,#26847,#26848,#26849,#26850,#26851,#26852,#26853,#26854,#26855,#26856,
#26857,#26858,#26859,#26860,#26861,#26862,#26863,#26864,#26865,#26866,#26867,
#26868,#26869,#26870,#26871),.UNSPECIFIED.,.F.,.F.,(4,3,3,3,3,3,3,3,3,3,
4),(0.,4.98163029433582E-5,0.000100000315597884,0.000150867282275571,0.000202142388486024,
0.000254132046646703,0.000271251473618865,0.000333586404663745,0.000403372432315032,
0.000481003240191196,0.00054250294723773),.UNSPECIFIED.);
#655=B_SPLINE_CURVE_WITH_KNOTS('',3,(#26911,#26912,#26913,#26914,#26915,
#26916,#26917,#26918,#26919,#26920,#26921,#26922,#26923,#26924,#26925,#26926,
#26927,#26928,#26929,#26930,#26931,#26932,#26933,#26934,#26935,#26936,#26937,
#26938,#26939,#26940,#26941,#26942,#26943,#26944,#26945,#26946,#26947),
 .UNSPECIFIED.,.F.,.F.,(4,3,3,3,3,3,3,3,3,3,3,3,4),(0.,6.99403168951901E-5,
0.000136638812200168,0.00019323995121385,0.000204958218300252,0.000257951721019661,
0.000273277624400336,0.00028545369268105,0.000346137712527676,0.00040865458897473,
0.00047263689487051,0.000539340363905251,0.000546555248800672),
 .UNSPECIFIED.);
#656=B_SPLINE_CURVE_WITH_KNOTS('',3,(#27013,#27014,#27015,#27016,#27017,
#27018,#27019,#27020,#27021,#27022,#27023,#27024,#27025,#27026,#27027,#27028,
#27029,#27030,#27031,#27032,#27033,#27034,#27035,#27036,#27037,#27038,#27039,
#27040,#27041,#27042,#27043,#27044,#27045,#27046,#27047,#27048,#27049,#27050,
#27051,#27052,#27053,#27054,#27055,#27056,#27057,#27058),.UNSPECIFIED.,
 .F.,.F.,(4,3,3,3,3,3,3,3,3,3,3,3,3,3,3,4),(0.,3.97160926935229E-5,8.01799642593007E-5,
0.000121988391402582,0.000134049545972337,0.000152559369824133,0.000190699212280166,
0.000233020073010242,0.000277317564290133,0.000281953897382099,0.000305118739648266,
0.000373877625544705,0.000442636511441145,0.000516471370795696,0.000591684329573585,
0.000610237479296514),.UNSPECIFIED.);
#657=B_SPLINE_CURVE_WITH_KNOTS('',3,(#27060,#27061,#27062,#27063,#27064,
#27065,#27066,#27067,#27068,#27069,#27070,#27071,#27072,#27073,#27074,#27075,
#27076,#27077,#27078,#27079,#27080,#27081,#27082,#27083,#27084,#27085,#27086,
#27087,#27088,#27089,#27090,#27091,#27092,#27093,#27094,#27095,#27096,#27097,
#27098,#27099,#27100,#27101,#27102,#27103,#27104,#27105),.UNSPECIFIED.,
 .F.,.F.,(4,3,3,3,3,3,3,3,3,3,3,3,3,3,3,4),(0.,7.40646428074384E-5,0.000146779369922617,
0.000164860955696866,0.000232495741978627,0.000300130528260388,0.000322950277848808,
0.000361000159970105,0.000375163160325479,0.000412679476358025,0.000450195792390571,
0.000468403009741553,0.000509319401678602,0.000549287864660367,0.000588177998706901,
0.000600261056520754),.UNSPECIFIED.);
#658=B_SPLINE_CURVE_WITH_KNOTS('',3,(#27140,#27141,#27142,#27143,#27144,
#27145,#27146,#27147,#27148,#27149,#27150,#27151,#27152,#27153,#27154,#27155,
#27156,#27157,#27158,#27159,#27160,#27161,#27162,#27163,#27164,#27165,#27166,
#27167,#27168,#27169,#27170,#27171,#27172,#27173,#27174,#27175,#27176,#27177,
#27178,#27179,#27180,#27181,#27182,#27183,#27184,#27185),.UNSPECIFIED.,
 .F.,.F.,(4,3,3,3,3,3,3,3,3,3,3,3,3,3,3,4),(0.,4.01784152590413E-5,8.11318192717161E-5,
0.00012343023163194,0.000133797481310322,0.000151845918076025,0.000189807397595031,
0.000231866097106636,0.000275906952598724,0.000281134062468662,0.000303691836152049,
0.000372309715976737,0.000440927595801426,0.000514103167120356,0.000588539200891124,
0.000607383672304106),.UNSPECIFIED.);
#659=B_SPLINE_CURVE_WITH_KNOTS('',3,(#27193,#27194,#27195,#27196,#27197,
#27198,#27199,#27200,#27201,#27202,#27203,#27204,#27205,#27206,#27207,#27208,
#27209,#27210,#27211,#27212,#27213,#27214,#27215,#27216,#27217,#27218,#27219,
#27220,#27221,#27222,#27223,#27224,#27225,#27226,#27227,#27228,#27229,#27230,
#27231,#27232,#27233,#27234,#27235,#27236,#27237,#27238,#27239,#27240,#27241,
#27242,#27243,#27244),.UNSPECIFIED.,.F.,.F.,(4,3,3,3,3,3,3,3,3,3,3,3,3,
3,3,3,3,4),(0.,0.000104093954358116,0.000217335668171905,0.000328639449066821,
0.000442850129340045,0.000551144481414275,0.00055706080961327,0.0006429177227539,
0.000726322659738398,0.00080560830646621,0.000835591214419904,0.000896354287923508,
0.000954074031547537,0.000974856416823221,0.00101967443613433,0.00106279159941887,
0.00110343944760186,0.00111412161922654),.UNSPECIFIED.);
#660=B_SPLINE_CURVE_WITH_KNOTS('',3,(#27294,#27295,#27296,#27297,#27298,
#27299,#27300,#27301,#27302,#27303,#27304,#27305,#27306,#27307,#27308,#27309,
#27310,#27311,#27312,#27313,#27314,#27315,#27316,#27317,#27318,#27319,#27320,
#27321,#27322,#27323,#27324,#27325,#27326,#27327,#27328,#27329,#27330,#27331,
#27332,#27333,#27334,#27335,#27336,#27337,#27338,#27339,#27340,#27341,#27342,
#27343,#27344,#27345,#27346,#27347,#27348,#27349,#27350,#27351,#27352,#27353,
#27354),.UNSPECIFIED.,.F.,.F.,(4,3,3,3,3,3,3,3,3,3,3,3,3,3,3,3,3,3,3,3,
4),(0.,3.01683521755654E-5,5.95123638939948E-5,8.83024180015813E-5,0.000116768391896489,
0.000120673408702262,0.000156899735254867,0.000194095346003115,0.000232946053824629,
0.000241346817404523,0.000284837120908685,0.000330243027193698,0.000378792539155905,
0.000430743086982471,0.000482693634809037,0.00056007281073296,0.000642027313858774,
0.000731891178241761,0.00082574384990152,0.000923569286420814,0.000965387269618077),
 .UNSPECIFIED.);
#661=B_SPLINE_CURVE_WITH_KNOTS('',3,(#27385,#27386,#27387,#27388,#27389,
#27390,#27391,#27392,#27393,#27394,#27395,#27396,#27397,#27398,#27399,#27400,
#27401,#27402,#27403,#27404,#27405,#27406,#27407,#27408,#27409,#27410,#27411,
#27412,#27413,#27414,#27415,#27416,#27417,#27418,#27419,#27420,#27421,#27422,
#27423,#27424,#27425,#27426,#27427,#27428,#27429,#27430),.UNSPECIFIED.,
 .F.,.F.,(4,3,3,3,3,3,3,3,3,3,3,3,3,3,3,4),(0.,7.33096139968579E-5,0.000145388861463487,
0.000163772356054208,0.000231283930773278,0.000298795505492349,0.000321020403765824,
0.000359079183383553,0.000373494381865434,0.000410843820051977,0.00044819325823852,
0.000465950705574249,0.000507344602017609,0.000547782593937178,0.000587118287670288,
0.000597591010984692),.UNSPECIFIED.);
#662=B_SPLINE_CURVE_WITH_KNOTS('',3,(#27478,#27479,#27480,#27481,#27482,
#27483,#27484,#27485,#27486,#27487,#27488,#27489),.UNSPECIFIED.,.F.,.F.,
(4,2,2,2,2,4),(9.9422622804038E-9,0.000325172939224853,0.000650345878449707,
0.00097551881767456,0.00113810528728698,0.00130069175689939),
 .UNSPECIFIED.);
#663=B_SPLINE_CURVE_WITH_KNOTS('',3,(#27544,#27545,#27546,#27547,#27548,
#27549,#27550,#27551,#27552,#27553,#27554,#27555,#27556,#27557,#27558,#27559,
#27560,#27561,#27562,#27563,#27564,#27565,#27566,#27567,#27568),
 .UNSPECIFIED.,.F.,.F.,(4,3,3,3,3,3,3,3,4),(0.,9.58519120559013E-5,0.000201048393009301,
0.000313533962690425,0.000443358794838372,0.000487856029895822,0.000498221418747226,
0.000765061137597183,0.000996433304431859),.UNSPECIFIED.);
#664=B_SPLINE_CURVE_WITH_KNOTS('',3,(#27603,#27604,#27605,#27606,#27607,
#27608,#27609,#27610,#27611,#27612,#27613,#27614,#27615,#27616,#27617,#27618,
#27619,#27620,#27621,#27622,#27623,#27624,#27625,#27626,#27627,#27628,#27629,
#27630,#27631,#27632,#27633),.UNSPECIFIED.,.F.,.F.,(4,3,3,3,3,3,3,3,3,3,
4),(0.,4.98163029433653E-5,0.000100000315597862,0.000150867282275564,0.000202142388486088,
0.000254132046646779,0.000271251473618865,0.000333586404663683,0.000403372432314982,
0.000481003240191066,0.00054250294723773),.UNSPECIFIED.);
#665=B_SPLINE_CURVE_WITH_KNOTS('',3,(#27668,#27669,#27670,#27671,#27672,
#27673,#27674,#27675,#27676,#27677,#27678,#27679,#27680,#27681,#27682,#27683,
#27684,#27685,#27686,#27687,#27688,#27689,#27690,#27691,#27692),
 .UNSPECIFIED.,.F.,.F.,(4,3,3,3,3,3,3,3,4),(0.,8.83378490479586E-5,0.000182066239385022,
0.000286502548781802,0.000402561956922467,0.000487834363092893,0.000496699977573566,
0.000791146466104245,0.000993390351418002),.UNSPECIFIED.);
#666=B_SPLINE_CURVE_WITH_KNOTS('',3,(#27837,#27838,#27839,#27840,#27841,
#27842,#27843,#27844,#27845,#27846,#27847,#27848,#27849,#27850,#27851,#27852,
#27853,#27854,#27855,#27856,#27857,#27858,#27859,#27860,#27861,#27862,#27863,
#27864,#27865,#27866,#27867,#27868,#27869,#27870),.UNSPECIFIED.,.F.,.F.,
(4,3,3,3,3,3,3,3,3,3,3,4),(0.,6.47846574223387E-5,0.000128085038052483,
0.000193342800026691,0.000254275817474483,0.000258600562000898,0.000269706482902605,
0.000323662397373896,0.000382521450089233,0.000443803383531375,0.000505428571282867,
0.00053941296580521),.UNSPECIFIED.);
#667=B_SPLINE_CURVE_WITH_KNOTS('',3,(#27909,#27910,#27911,#27912,#27913,
#27914,#27915,#27916,#27917,#27918,#27919,#27920,#27921,#27922,#27923,#27924,
#27925,#27926,#27927,#27928,#27929,#27930,#27931,#27932,#27933,#27934,#27935,
#27936,#27937,#27938,#27939,#27940,#27941,#27942,#27943,#27944,#27945,#27946,
#27947,#27948,#27949,#27950,#27951,#27952,#27953,#27954),.UNSPECIFIED.,
 .F.,.F.,(4,3,3,3,3,3,3,3,3,3,3,3,3,3,3,4),(0.,3.50262368532445E-5,7.11751710419857E-5,
0.000109339082870391,0.000148762751083315,0.000189988996390031,0.000198220556017292,
0.000254911247279634,0.000313675244693709,0.000375594961504314,0.000396441112034585,
0.000477792055753319,0.000566506458090588,0.000659059947720601,0.000755430891818796,
0.000792882224069168),.UNSPECIFIED.);
#668=B_SPLINE_CURVE_WITH_KNOTS('',3,(#27979,#27980,#27981,#27982,#27983,
#27984,#27985,#27986,#27987,#27988,#27989,#27990,#27991,#27992,#27993,#27994,
#27995,#27996,#27997,#27998,#27999,#28000,#28001,#28002,#28003,#28004,#28005,
#28006,#28007,#28008,#28009,#28010,#28011,#28012,#28013,#28014,#28015,#28016,
#28017,#28018,#28019,#28020,#28021,#28022,#28023,#28024,#28025,#28026,#28027,
#28028,#28029,#28030,#28031,#28032,#28033,#28034,#28035,#28036,#28037,#28038,
#28039,#28040,#28041,#28042,#28043,#28044,#28045,#28046,#28047,#28048,#28049,
#28050,#28051,#28052,#28053,#28054,#28055,#28056,#28057,#28058,#28059,#28060,
#28061,#28062,#28063),.UNSPECIFIED.,.F.,.F.,(4,3,3,3,3,3,3,3,3,3,3,3,3,
3,3,3,3,3,3,3,3,3,3,3,3,3,3,3,4),(3.63939196670295E-10,7.80137041101504E-5,
0.000136523982192763,0.000158465336473743,0.000196862706465458,0.00025445876145303,
0.000283256788946816,0.000297655802693709,0.000312054816440602,0.000356230898886013,
0.000390068520550753,0.000399820233564522,0.000408352982451569,0.000438217603556236,
0.000464692044654508,0.000468082224660904,0.000487585650688441,0.000494899435448768,
0.00049809921628141,0.00050001235016164,0.000504098805342616,0.000534061837383381,
0.000546095928771053,0.000550971785277938,0.000555542900753142,0.000586967153584001,
0.000589826266817172,0.00061930792844511,0.000624109632881203),
 .UNSPECIFIED.);
#669=B_SPLINE_CURVE_WITH_KNOTS('',3,(#28095,#28096,#28097,#28098,#28099,
#28100,#28101,#28102,#28103,#28104,#28105,#28106,#28107,#28108,#28109,#28110,
#28111,#28112,#28113,#28114,#28115,#28116,#28117,#28118,#28119,#28120,#28121,
#28122,#28123,#28124,#28125,#28126,#28127,#28128,#28129,#28130,#28131,#28132,
#28133,#28134,#28135,#28136,#28137,#28138,#28139,#28140,#28141,#28142,#28143,
#28144,#28145,#28146,#28147,#28148,#28149,#28150,#28151,#28152,#28153,#28154,
#28155,#28156,#28157,#28158,#28159,#28160,#28161,#28162,#28163,#28164,#28165,
#28166,#28167,#28168,#28169,#28170,#28171,#28172,#28173,#28174,#28175,#28176,
#28177,#28178,#28179,#28180,#28181,#28182),.UNSPECIFIED.,.F.,.F.,(4,3,3,
3,3,3,3,3,3,3,3,3,3,3,3,3,3,3,3,3,3,3,3,3,3,3,3,3,3,4),(0.,2.50679729420699E-5,
3.13295796930182E-5,4.72260971999786E-5,7.10708734604193E-5,8.29932615906396E-5,
8.89544556557498E-5,9.04447541720273E-5,9.49156497208599E-5,0.000121982835340966,
0.00014237347458129,0.000145339588635067,0.000147646510203545,0.0001803434454297,
0.00018983129944172,0.000220219538030718,0.000237289124302146,0.000255085808624806,
0.000262871858015969,0.000270171279320185,0.000314583791963415,0.000324174511012843,
0.000376787272343466,0.000379662598883424,0.000415768922432964,0.000477328763328744,
0.000543052315574684,0.000616743070253868,0.000699630235102015,0.000759325197766855),
 .UNSPECIFIED.);
#670=B_SPLINE_CURVE_WITH_KNOTS('',3,(#28222,#28223,#28224,#28225,#28226,
#28227,#28228,#28229,#28230,#28231,#28232,#28233,#28234),.UNSPECIFIED.,
 .F.,.F.,(4,3,3,3,4),(0.,0.00112869544108361,0.00112886842160677,0.0017855132108252,
0.00225773684321331),.UNSPECIFIED.);
#671=B_SPLINE_CURVE_WITH_KNOTS('',3,(#28282,#28283,#28284,#28285,#28286,
#28287,#28288,#28289,#28290,#28291,#28292,#28293,#28294,#28295,#28296,#28297),
 .UNSPECIFIED.,.F.,.F.,(4,3,3,3,3,4),(1.73472347597681E-18,0.000789165583599754,
0.00112882209307301,0.00112972782036785,0.00186613475216116,0.00225764418614602),
 .UNSPECIFIED.);
#672=B_SPLINE_CURVE_WITH_KNOTS('',3,(#28361,#28362,#28363,#28364,#28365,
#28366,#28367,#28368,#28369,#28370,#28371,#28372,#28373,#28374,#28375,#28376,
#28377,#28378,#28379,#28380,#28381,#28382),.UNSPECIFIED.,.F.,.F.,(4,3,3,
3,3,3,3,4),(0.,0.000187383859258548,0.000390718319973205,0.000506671891006544,
0.000510839709360771,0.000711636939114786,0.00091215180264492,0.00102167941872154),
 .UNSPECIFIED.);
#673=B_SPLINE_CURVE_WITH_KNOTS('',3,(#28403,#28404,#28405,#28406,#28407,
#28408,#28409,#28410,#28411,#28412,#28413,#28414,#28415,#28416,#28417,#28418),
 .UNSPECIFIED.,.F.,.F.,(4,3,3,3,3,4),(3.46944695195361E-18,0.000789165584742738,
0.00112882209307305,0.00112972782036789,0.0018661347548332,0.0022576441861461),
 .UNSPECIFIED.);
#674=B_SPLINE_CURVE_WITH_KNOTS('',3,(#28530,#28531,#28532,#28533,#28534,
#28535,#28536,#28537,#28538,#28539,#28540,#28541,#28542,#28543,#28544,#28545,
#28546,#28547,#28548),.UNSPECIFIED.,.F.,.F.,(4,3,3,3,3,3,4),(0.,0.000411399963284772,
0.000510753962571242,0.000514787301367235,0.000703786539778562,0.000866757158960636,
0.00102150792514248),.UNSPECIFIED.);
#675=B_SPLINE_CURVE_WITH_KNOTS('',3,(#28553,#28554,#28555,#28556,#28557,
#28558,#28559,#28560,#28561,#28562,#28563,#28564,#28565),.UNSPECIFIED.,
 .F.,.F.,(4,3,3,3,4),(0.,0.00112869544108359,0.00112886842160676,0.00178551321104577,
0.00225773684321329),.UNSPECIFIED.);
#676=B_SPLINE_CURVE_WITH_KNOTS('',3,(#28675,#28676,#28677,#28678,#28679,
#28680,#28681,#28682,#28683,#28684,#28685,#28686,#28687),.UNSPECIFIED.,
 .F.,.F.,(4,3,3,3,4),(2.36524922520259E-16,0.000656666445676668,0.00112890565164586,
0.00112907863787392,0.00225781130329172),.UNSPECIFIED.);
#677=B_SPLINE_CURVE_WITH_KNOTS('',3,(#28694,#28695,#28696,#28697,#28698,
#28699,#28700,#28701,#28702,#28703,#28704,#28705,#28706,#28707,#28708,#28709,
#28710,#28711,#28712),.UNSPECIFIED.,.F.,.F.,(4,3,3,3,3,3,4),(0.,0.000411399964056932,
0.00051075396257123,0.000514787301367217,0.000703786539700468,0.000866757158900925,
0.00102150792514246),.UNSPECIFIED.);
#678=B_SPLINE_CURVE_WITH_KNOTS('',3,(#28795,#28796,#28797,#28798,#28799,
#28800,#28801,#28802,#28803,#28804,#28805,#28806,#28807,#28808,#28809,#28810),
 .UNSPECIFIED.,.F.,.F.,(4,3,3,3,3,4),(0.,0.000736491667076813,0.00112804614732749,
0.00112895197883811,0.00191820836757618,0.00225790395767623),
 .UNSPECIFIED.);
#679=B_SPLINE_CURVE_WITH_KNOTS('',3,(#28876,#28877,#28878,#28879,#28880,
#28881,#28882,#28883,#28884,#28885,#28886,#28887,#28888,#28889,#28890,#28891,
#28892,#28893,#28894,#28895,#28896,#28897),.UNSPECIFIED.,.F.,.F.,(4,3,3,
3,3,3,3,4),(0.,0.000187383859222642,0.000390718319947459,0.000506671891006534,
0.000510839709360756,0.000711636939101215,0.000912151802618219,0.00102167941872151),
 .UNSPECIFIED.);
#680=B_SPLINE_CURVE_WITH_KNOTS('',3,(#28939,#28940,#28941,#28942,#28943,
#28944,#28945,#28946,#28947,#28948,#28949,#28950,#28951,#28952,#28953,#28954,
#28955,#28956,#28957,#28958,#28959,#28960),.UNSPECIFIED.,.F.,.F.,(4,3,3,
3,3,3,3,4),(0.,0.000187383859212357,0.000390718320022676,0.000506671891006541,
0.000510839709360768,0.000711636939116541,0.000912151802649271,0.00102167941872154),
 .UNSPECIFIED.);
#681=B_SPLINE_CURVE_WITH_KNOTS('',3,(#29027,#29028,#29029,#29030,#29031,
#29032,#29033,#29034,#29035,#29036,#29037,#29038,#29039,#29040,#29041,#29042),
 .UNSPECIFIED.,.F.,.F.,(4,3,3,3,3,4),(0.,0.000736491665055099,0.00112804614732747,
0.00112895197883809,0.00191820836627224,0.00225790395767619),
 .UNSPECIFIED.);
#682=B_SPLINE_CURVE_WITH_KNOTS('',3,(#29167,#29168,#29169,#29170,#29171,
#29172,#29173,#29174,#29175,#29176,#29177,#29178,#29179,#29180,#29181,#29182,
#29183,#29184,#29185),.UNSPECIFIED.,.F.,.F.,(4,3,3,3,3,3,4),(0.,0.000160829789774429,
0.000333619132037895,0.000508566612075994,0.00051261464436556,0.000925513337291967,
0.00102522928873112),.UNSPECIFIED.);
#683=B_SPLINE_CURVE_WITH_KNOTS('',3,(#29206,#29207,#29208,#29209,#29210,
#29211,#29212,#29213,#29214,#29215,#29216,#29217,#29218),.UNSPECIFIED.,
 .F.,.F.,(4,3,3,3,4),(2.37963132368939E-16,0.000656666445458113,0.00112890565164585,
0.00112907863787391,0.00225781130329169),.UNSPECIFIED.);
#684=B_SPLINE_CURVE_WITH_KNOTS('',3,(#29251,#29252,#29253,#29254,#29255,
#29256,#29257,#29258,#29259,#29260,#29261,#29262,#29263,#29264,#29265,#29266,
#29267,#29268,#29269),.UNSPECIFIED.,.F.,.F.,(4,3,3,3,3,3,4),(0.,0.000411399963336404,
0.000510753962571242,0.000514787301367239,0.000703786539777697,0.000866757158959836,
0.00102150792514248),.UNSPECIFIED.);
#685=B_SPLINE_CURVE_WITH_KNOTS('',3,(#29394,#29395,#29396,#29397,#29398,
#29399,#29400,#29401,#29402,#29403,#29404,#29405,#29406,#29407,#29408,#29409,
#29410,#29411,#29412,#29413,#29414,#29415),.UNSPECIFIED.,.F.,.F.,(4,3,3,
3,3,3,3,4),(0.,0.000197996176151733,0.000401763276582256,0.000511744806759771,
0.000515920009585647,0.000722551962790744,0.000911736942394862,0.00102348961351954),
 .UNSPECIFIED.);
#686=B_SPLINE_CURVE_WITH_KNOTS('',3,(#29492,#29493,#29494,#29495,#29496,
#29497),.UNSPECIFIED.,.F.,.F.,(4,2,4),(0.,0.5,1.),.UNSPECIFIED.);
#687=B_SPLINE_CURVE_WITH_KNOTS('',3,(#29499,#29500,#29501,#29502,#29503,
#29504,#29505,#29506,#29507,#29508,#29509,#29510,#29511,#29512,#29513,#29514),
 .UNSPECIFIED.,.F.,.F.,(4,3,3,3,3,4),(0.,0.25,0.478355226420189,0.695629167073083,
0.902574508587078,1.),.UNSPECIFIED.);
#688=B_SPLINE_CURVE_WITH_KNOTS('',3,(#29515,#29516,#29517,#29518,#29519,
#29520),.UNSPECIFIED.,.F.,.F.,(4,2,4),(0.,0.5,1.),.UNSPECIFIED.);
#689=B_SPLINE_CURVE_WITH_KNOTS('',3,(#29585,#29586,#29587,#29588,#29589,
#29590),.UNSPECIFIED.,.F.,.F.,(4,2,4),(0.,0.5,1.),.UNSPECIFIED.);
#690=B_SPLINE_CURVE_WITH_KNOTS('',3,(#29592,#29593,#29594,#29595),
 .UNSPECIFIED.,.F.,.F.,(4,4),(0.,1.),.UNSPECIFIED.);
#691=B_SPLINE_CURVE_WITH_KNOTS('',3,(#29596,#29597,#29598,#29599,#29600,
#29601),.UNSPECIFIED.,.F.,.F.,(4,2,4),(0.,0.5,1.),.UNSPECIFIED.);
#692=B_SPLINE_CURVE_WITH_KNOTS('',3,(#29662,#29663,#29664,#29665,#29666,
#29667,#29668,#29669,#29670,#29671,#29672,#29673,#29674),.UNSPECIFIED.,
 .F.,.F.,(4,3,3,3,4),(0.,0.223169250634155,0.461855220689887,0.714975201892481,
1.),.UNSPECIFIED.);
#693=B_SPLINE_CURVE_WITH_KNOTS('',3,(#29675,#29676,#29677,#29678,#29679,
#29680),.UNSPECIFIED.,.F.,.F.,(4,2,4),(0.,0.5,1.),.UNSPECIFIED.);
#694=B_SPLINE_CURVE_WITH_KNOTS('',3,(#29742,#29743,#29744,#29745,#29746,
#29747,#29748,#29749,#29750,#29751,#29752,#29753,#29754,#29755,#29756,#29757),
 .UNSPECIFIED.,.F.,.F.,(4,3,3,3,3,4),(0.,0.26951546128406,0.518490249146965,
0.759245124573483,0.982227995955573,1.),.UNSPECIFIED.);
#695=B_SPLINE_CURVE_WITH_KNOTS('',3,(#29758,#29759,#29760,#29761,#29762,
#29763),.UNSPECIFIED.,.F.,.F.,(4,2,4),(0.,0.5,1.),.UNSPECIFIED.);
#696=B_SPLINE_CURVE_WITH_KNOTS('',3,(#29828,#29829,#29830,#29831),
 .UNSPECIFIED.,.F.,.F.,(4,4),(0.,1.),.UNSPECIFIED.);
#697=B_SPLINE_CURVE_WITH_KNOTS('',3,(#29833,#29834,#29835,#29836,#29837,
#29838,#29839,#29840,#29841,#29842,#29843,#29844,#29845,#29846,#29847,#29848,
#29849,#29850,#29851,#29852,#29853,#29854,#29855,#29856,#29857,#29858,#29859,
#29860,#29861,#29862,#29863,#29864,#29865,#29866,#29867,#29868,#29869,#29870,
#29871,#29872,#29873,#29874,#29875,#29876,#29877,#29878,#29879,#29880,#29881,
#29882,#29883,#29884,#29885,#29886,#29887,#29888,#29889,#29890,#29891,#29892,
#29893,#29894,#29895,#29896),.UNSPECIFIED.,.F.,.F.,(4,3,3,3,3,3,3,3,3,3,
3,3,3,3,3,3,3,3,3,3,3,4),(0.,0.184274983493926,0.325645671627907,0.482911947486233,
0.55677277721243,0.609022292004883,0.640178223344559,0.724682266712519,
0.782814976637048,0.841808654689151,0.899384096462184,0.938008402815887,
0.960709962461591,0.975964848021033,0.985714019774265,0.992447416236639,
0.995463191527497,0.997731595763749,0.998865797881874,0.999432898547245,
0.999931188332118,0.999999999212616),.UNSPECIFIED.);
#698=B_SPLINE_CURVE_WITH_KNOTS('',3,(#29897,#29898,#29899,#29900,#29901,
#29902),.UNSPECIFIED.,.F.,.F.,(4,2,4),(0.,0.5,1.),.UNSPECIFIED.);
#699=B_SPLINE_CURVE_WITH_KNOTS('',3,(#29953,#29954,#29955,#29956,#29957,
#29958),.UNSPECIFIED.,.F.,.F.,(4,2,4),(0.,0.5,1.),.UNSPECIFIED.);
#700=B_SPLINE_CURVE_WITH_KNOTS('',3,(#29959,#29960,#29961,#29962,#29963,
#29964,#29965,#29966,#29967,#29968,#29969,#29970,#29971,#29972,#29973,#29974),
 .UNSPECIFIED.,.F.,.F.,(4,3,3,3,3,4),(0.,0.205895634064056,0.424355643769067,
0.652797994841561,0.901136507518082,1.),.UNSPECIFIED.);
#701=B_SPLINE_CURVE_WITH_KNOTS('',3,(#29975,#29976,#29977,#29978,#29979,
#29980),.UNSPECIFIED.,.F.,.F.,(4,2,4),(0.,0.5,1.),.UNSPECIFIED.);
#702=B_SPLINE_CURVE_WITH_KNOTS('',3,(#30030,#30031,#30032,#30033,#30034,
#30035,#30036,#30037,#30038,#30039,#30040,#30041,#30042,#30043,#30044,#30045),
 .UNSPECIFIED.,.F.,.F.,(4,3,3,3,3,4),(0.,0.25,0.478355226419942,0.695629167072226,
0.902574508585992,1.),.UNSPECIFIED.);
#703=B_SPLINE_CURVE_WITH_KNOTS('',3,(#30046,#30047,#30048,#30049,#30050,
#30051),.UNSPECIFIED.,.F.,.F.,(4,2,4),(0.,0.5,1.),.UNSPECIFIED.);
#704=B_SPLINE_CURVE_WITH_KNOTS('',3,(#30116,#30117,#30118,#30119,#30120,
#30121),.UNSPECIFIED.,.F.,.F.,(4,2,4),(0.,0.5,1.),.UNSPECIFIED.);
#705=B_SPLINE_CURVE_WITH_KNOTS('',3,(#30123,#30124,#30125,#30126),
 .UNSPECIFIED.,.F.,.F.,(4,4),(0.,1.),.UNSPECIFIED.);
#706=B_SPLINE_CURVE_WITH_KNOTS('',3,(#30127,#30128,#30129,#30130,#30131,
#30132),.UNSPECIFIED.,.F.,.F.,(4,2,4),(0.,0.5,1.),.UNSPECIFIED.);
#707=B_SPLINE_CURVE_WITH_KNOTS('',3,(#30193,#30194,#30195,#30196,#30197,
#30198,#30199,#30200,#30201,#30202,#30203,#30204,#30205),.UNSPECIFIED.,
 .F.,.F.,(4,3,3,3,4),(0.,0.223169250633592,0.461855220688884,0.714975201891238,
1.),.UNSPECIFIED.);
#708=B_SPLINE_CURVE_WITH_KNOTS('',3,(#30206,#30207,#30208,#30209,#30210,
#30211),.UNSPECIFIED.,.F.,.F.,(4,2,4),(0.,0.5,1.),.UNSPECIFIED.);
#709=B_SPLINE_CURVE_WITH_KNOTS('',3,(#30274,#30275,#30276,#30277,#30278,
#30279),.UNSPECIFIED.,.F.,.F.,(4,2,4),(0.,0.5,1.),.UNSPECIFIED.);
#710=B_SPLINE_CURVE_WITH_KNOTS('',3,(#30341,#30342,#30343,#30344,#30345,
#30346),.UNSPECIFIED.,.F.,.F.,(4,2,4),(0.,0.5,1.),.UNSPECIFIED.);
#711=B_SPLINE_CURVE_WITH_KNOTS('',3,(#30348,#30349,#30350,#30351,#30352,
#30353,#30354,#30355,#30356,#30357,#30358,#30359,#30360,#30361,#30362,#30363),
 .UNSPECIFIED.,.F.,.F.,(4,3,3,3,3,4),(0.,0.269515461284092,0.518490249146695,
0.759245124573347,0.982227995954943,1.),.UNSPECIFIED.);
#712=B_SPLINE_CURVE_WITH_KNOTS('',3,(#30364,#30365,#30366,#30367,#30368,
#30369),.UNSPECIFIED.,.F.,.F.,(4,2,4),(0.,0.5,1.),.UNSPECIFIED.);
#713=B_SPLINE_CURVE_WITH_KNOTS('',3,(#30434,#30435,#30436,#30437),
 .UNSPECIFIED.,.F.,.F.,(4,4),(0.,1.),.UNSPECIFIED.);
#714=B_SPLINE_CURVE_WITH_KNOTS('',3,(#30439,#30440,#30441,#30442,#30443,
#30444),.UNSPECIFIED.,.F.,.F.,(4,2,4),(0.,0.5,1.),.UNSPECIFIED.);
#715=B_SPLINE_CURVE_WITH_KNOTS('',3,(#30445,#30446,#30447,#30448,#30449,
#30450),.UNSPECIFIED.,.F.,.F.,(4,2,4),(0.,0.5,1.),.UNSPECIFIED.);
#716=B_SPLINE_CURVE_WITH_KNOTS('',3,(#30499,#30500,#30501,#30502,#30503,
#30504,#30505,#30506,#30507,#30508,#30509,#30510,#30511,#30512,#30513,#30514),
 .UNSPECIFIED.,.F.,.F.,(4,3,3,3,3,4),(0.,0.205895634064936,0.424355643770462,
0.652797994843313,0.901136507520509,1.),.UNSPECIFIED.);
#717=B_SPLINE_CURVE_WITH_KNOTS('',3,(#30515,#30516,#30517,#30518,#30519,
#30520),.UNSPECIFIED.,.F.,.F.,(4,2,4),(0.,0.5,1.),.UNSPECIFIED.);
#718=B_SPLINE_CURVE_WITH_KNOTS('',3,(#30570,#30571,#30572,#30573,#30574,
#30575,#30576,#30577,#30578,#30579,#30580,#30581,#30582,#30583,#30584,#30585),
 .UNSPECIFIED.,.F.,.F.,(4,3,3,3,3,4),(0.,0.25,0.478355226421249,0.695629167075021,
0.902574508590587,1.),.UNSPECIFIED.);
#719=B_SPLINE_CURVE_WITH_KNOTS('',3,(#30586,#30587,#30588,#30589,#30590,
#30591),.UNSPECIFIED.,.F.,.F.,(4,2,4),(0.,0.5,1.),.UNSPECIFIED.);
#720=B_SPLINE_CURVE_WITH_KNOTS('',3,(#30656,#30657,#30658,#30659,#30660,
#30661),.UNSPECIFIED.,.F.,.F.,(4,2,4),(0.,0.5,1.),.UNSPECIFIED.);
#721=B_SPLINE_CURVE_WITH_KNOTS('',3,(#30663,#30664,#30665,#30666,#30667,
#30668,#30669,#30670,#30671,#30672,#30673,#30674,#30675,#30676,#30677,#30678,
#30679,#30680,#30681,#30682,#30683,#30684,#30685,#30686,#30687,#30688,#30689,
#30690,#30691,#30692,#30693,#30694,#30695,#30696,#30697,#30698,#30699,#30700,
#30701,#30702,#30703,#30704,#30705,#30706,#30707,#30708,#30709,#30710,#30711,
#30712,#30713,#30714,#30715,#30716,#30717),.UNSPECIFIED.,.F.,.F.,(4,3,3,
3,3,3,3,3,3,3,3,3,3,3,3,3,3,3,4),(0.,0.134829460600233,0.301935450994647,
0.331938859566448,0.520486721225732,0.653948260231371,0.766867850117276,
0.847465272943437,0.903670198362982,0.941441109775431,0.964211265170187,
0.978961680044948,0.986981420564942,0.993490710282471,0.996745355141236,
0.998372677570618,0.999186338355832,0.999785281511195,0.999999999141046),
 .UNSPECIFIED.);
#722=B_SPLINE_CURVE_WITH_KNOTS('',3,(#30718,#30719,#30720,#30721,#30722,
#30723),.UNSPECIFIED.,.F.,.F.,(4,2,4),(0.,0.5,1.),.UNSPECIFIED.);
#723=B_SPLINE_CURVE_WITH_KNOTS('',3,(#30774,#30775,#30776,#30777,#30778,
#30779),.UNSPECIFIED.,.F.,.F.,(4,2,4),(0.,0.5,1.),.UNSPECIFIED.);
#724=B_SPLINE_CURVE_WITH_KNOTS('',3,(#30780,#30781,#30782,#30783,#30784,
#30785,#30786,#30787,#30788,#30789,#30790,#30791,#30792,#30793,#30794,#30795),
 .UNSPECIFIED.,.F.,.F.,(4,3,3,3,3,4),(0.,0.205895634064023,0.424355643768918,
0.65279799484117,0.901136507517712,1.),.UNSPECIFIED.);
#725=B_SPLINE_CURVE_WITH_KNOTS('',3,(#30796,#30797,#30798,#30799,#30800,
#30801),.UNSPECIFIED.,.F.,.F.,(4,2,4),(0.,0.5,1.),.UNSPECIFIED.);
#726=B_SPLINE_CURVE_WITH_KNOTS('',3,(#30851,#30852,#30853,#30854,#30855,
#30856,#30857,#30858,#30859,#30860,#30861,#30862,#30863,#30864,#30865,#30866),
 .UNSPECIFIED.,.F.,.F.,(4,3,3,3,3,4),(0.,0.25,0.478355226420375,0.695629167073178,
0.902574508587577,1.),.UNSPECIFIED.);
#727=B_SPLINE_CURVE_WITH_KNOTS('',3,(#30867,#30868,#30869,#30870,#30871,
#30872),.UNSPECIFIED.,.F.,.F.,(4,2,4),(0.,0.5,1.),.UNSPECIFIED.);
#728=B_SPLINE_CURVE_WITH_KNOTS('',3,(#30937,#30938,#30939,#30940,#30941,
#30942),.UNSPECIFIED.,.F.,.F.,(4,2,4),(0.,0.5,1.),.UNSPECIFIED.);
#729=B_SPLINE_CURVE_WITH_KNOTS('',3,(#30944,#30945,#30946,#30947,#30948,
#30949,#30950,#30951,#30952,#30953,#30954,#30955,#30956,#30957,#30958,#30959,
#30960,#30961,#30962,#30963,#30964,#30965,#30966,#30967,#30968,#30969,#30970,
#30971,#30972,#30973,#30974,#30975,#30976,#30977,#30978,#30979,#30980,#30981,
#30982,#30983,#30984,#30985,#30986,#30987,#30988,#30989,#30990,#30991,#30992,
#30993,#30994,#30995,#30996,#30997,#30998),.UNSPECIFIED.,.F.,.F.,(4,3,3,
3,3,3,3,3,3,3,3,3,3,3,3,3,3,3,4),(0.,0.134829524450431,0.301935899082962,
0.331938859566374,0.520486852331808,0.653948260231437,0.765695406250714,
0.845739463039844,0.901726408213813,0.939310939832059,0.962010705761424,
0.977750708016431,0.988647584692032,0.993490710271438,0.996745355135719,
0.998372677567859,0.999186338354459,0.999785281509885,0.999999999141059),
 .UNSPECIFIED.);
#730=B_SPLINE_CURVE_WITH_KNOTS('',3,(#30999,#31000,#31001,#31002,#31003,
#31004),.UNSPECIFIED.,.F.,.F.,(4,2,4),(0.,0.5,1.),.UNSPECIFIED.);
#731=B_SPLINE_CURVE_WITH_KNOTS('',3,(#31066,#31067,#31068,#31069,#31070,
#31071),.UNSPECIFIED.,.F.,.F.,(4,2,4),(0.,0.5,1.),.UNSPECIFIED.);
#732=B_SPLINE_CURVE_WITH_KNOTS('',3,(#31134,#31135,#31136,#31137,#31138,
#31139),.UNSPECIFIED.,.F.,.F.,(4,2,4),(0.,0.5,1.),.UNSPECIFIED.);
#733=B_SPLINE_CURVE_WITH_KNOTS('',3,(#31161,#31162,#31163,#31164,#31165,
#31166,#31167,#31168,#31169,#31170,#31171,#31172,#31173,#31174,#31175,#31176,
#31177,#31178,#31179,#31180,#31181,#31182),.UNSPECIFIED.,.F.,.F.,(4,3,3,
3,3,3,3,4),(0.,0.000123360913687075,0.00025951037912914,0.000406482329163153,
0.000585460068616017,0.000594183385201075,0.000955339327009254,0.00118832361361941),
 .UNSPECIFIED.);
#734=B_SPLINE_CURVE_WITH_KNOTS('',3,(#31203,#31204,#31205,#31206,#31207,
#31208,#31209,#31210,#31211,#31212,#31213,#31214,#31215,#31216,#31217,#31218,
#31219,#31220,#31221,#31222,#31223,#31224),.UNSPECIFIED.,.F.,.F.,(4,3,3,
3,3,3,3,4),(4.30167323683359E-8,0.00029867815700615,0.000593798351081719,
0.000602268552183542,0.0007833357220942,0.000949532856772951,0.00110145074954496,
0.00118759670216344),.UNSPECIFIED.);
#735=B_SPLINE_CURVE_WITH_KNOTS('',3,(#31273,#31274,#31275,#31276,#31277,
#31278),.UNSPECIFIED.,.F.,.F.,(4,2,4),(0.,0.5,1.),.UNSPECIFIED.);
#736=B_SPLINE_CURVE_WITH_KNOTS('',3,(#31350,#31351,#31352,#31353,#31354,
#31355,#31356,#31357,#31358,#31359,#31360,#31361,#31362,#31363,#31364,#31365,
#31366,#31367,#31368,#31369,#31370,#31371,#31372,#31373,#31374,#31375,#31376,
#31377,#31378,#31379,#31380,#31381,#31382,#31383,#31384,#31385,#31386,#31387,
#31388,#31389,#31390,#31391,#31392,#31393,#31394,#31395,#31396,#31397,#31398,
#31399,#31400,#31401,#31402,#31403,#31404),.UNSPECIFIED.,.F.,.F.,(4,3,3,
3,3,3,3,3,3,3,3,3,3,3,3,3,3,3,4),(8.57224357468246E-10,0.000627254895781897,
0.00125605220505132,0.00251210441010265,0.00502420882020529,0.0136336628022367,
0.0252314236373915,0.0410680722324126,0.0681502624529836,0.113858512147431,
0.184994280858008,0.291969184096878,0.346051748925883,0.519710693631118,
0.668061140433536,0.827606356909723,0.964640047971178,0.98715157338591,
1.),.UNSPECIFIED.);
#737=B_SPLINE_CURVE_WITH_KNOTS('',3,(#31423,#31424,#31425,#31426,#31427,
#31428,#31429,#31430,#31431,#31432,#31433,#31434,#31435,#31436,#31437,#31438,
#31439,#31440,#31441,#31442,#31443,#31444,#31445,#31446,#31447),
 .UNSPECIFIED.,.F.,.F.,(4,3,3,3,3,3,3,3,4),(4.30147703006247E-8,0.000270288099787492,
0.000513938606912812,0.00059425364289645,0.000603710958331439,0.000790752044623706,
0.000965824226330528,0.00112861151875137,0.0011885072857929),
 .UNSPECIFIED.);
#738=B_SPLINE_CURVE_WITH_KNOTS('',3,(#31466,#31467,#31468,#31469,#31470,
#31471,#31472,#31473,#31474,#31475,#31476,#31477,#31478,#31479,#31480,#31481,
#31482,#31483,#31484,#31485,#31486,#31487),.UNSPECIFIED.,.F.,.F.,(4,3,3,
3,3,3,3,4),(0.,0.000158882102081258,0.00032688426378663,0.000515357261128183,
0.000587493639452289,0.000595665178359072,0.000945792692676976,0.00119128711121805),
 .UNSPECIFIED.);
#739=B_SPLINE_CURVE_WITH_KNOTS('',3,(#31508,#31509,#31510,#31511,#31512,
#31513,#31514,#31515,#31516,#31517,#31518,#31519,#31520,#31521,#31522,#31523,
#31524,#31525,#31526,#31527,#31528,#31529),.UNSPECIFIED.,.F.,.F.,(4,3,3,
3,3,3,3,4),(1.90660672321663E-16,0.000123777251417005,0.000260370684246027,
0.000407829318327282,0.00058555605220498,0.000594289208708569,0.000954348914487693,
0.00118853525410901),.UNSPECIFIED.);
#740=B_SPLINE_CURVE_WITH_KNOTS('',3,(#31604,#31605,#31606,#31607,#31608,
#31609),.UNSPECIFIED.,.F.,.F.,(4,2,4),(0.,0.5,1.),.UNSPECIFIED.);
#741=B_SPLINE_CURVE_WITH_KNOTS('',3,(#31638,#31639,#31640,#31641,#31642,
#31643,#31644,#31645,#31646,#31647,#31648,#31649,#31650,#31651,#31652,#31653,
#31654,#31655,#31656,#31657,#31658,#31659,#31660,#31661,#31662),
 .UNSPECIFIED.,.F.,.F.,(4,3,3,3,3,3,3,3,4),(0.,0.000164956261028691,0.000338143702530957,
0.000527870844727718,0.000582731284092286,0.000592094961956777,0.000848990011105951,
0.00112806173363088,0.00118414707026094),.UNSPECIFIED.);
#742=B_SPLINE_CURVE_WITH_KNOTS('',3,(#31788,#31789,#31790,#31791,#31792,
#31793,#31794,#31795,#31796,#31797,#31798,#31799,#31800,#31801,#31802,#31803,
#31804,#31805,#31806,#31807,#31808,#31809,#31810,#31811,#31812,#31813,#31814,
#31815,#31816,#31817,#31818,#31819,#31820,#31821,#31822,#31823,#31824,#31825,
#31826,#31827,#31828,#31829,#31830,#31831,#31832,#31833,#31834,#31835,#31836,
#31837,#31838,#31839),.UNSPECIFIED.,.F.,.F.,(4,3,3,3,3,3,3,3,3,3,3,3,3,
3,3,3,3,4),(8.57205116275548E-10,0.00062725489807238,0.00125605219573295,
0.0025121043914659,0.00502420878293179,0.0136336627391616,0.0252314235092207,
0.0410680718371953,0.0681502630269255,0.113858513076608,0.184994282344012,
0.291969186221209,0.34605174892585,0.519710992297142,0.668061140433496,
0.834030570216748,0.968862259433357,1.),.UNSPECIFIED.);
#743=B_SPLINE_CURVE_WITH_KNOTS('',3,(#31858,#31859,#31860,#31861,#31862,
#31863,#31864,#31865,#31866,#31867,#31868,#31869,#31870,#31871,#31872,#31873,
#31874,#31875,#31876,#31877,#31878,#31879),.UNSPECIFIED.,.F.,.F.,(4,3,3,
3,3,3,3,4),(4.30167364622209E-8,0.000298678157011449,0.000593798351081719,
0.000602268552183536,0.000783335722089147,0.000949532856766907,0.00110145074954175,
0.00118759670216344),.UNSPECIFIED.);
#744=B_SPLINE_CURVE_WITH_KNOTS('',3,(#31997,#31998,#31999,#32000,#32001,
#32002,#32003,#32004,#32005,#32006,#32007,#32008,#32009,#32010,#32011,#32012,
#32013,#32014,#32015,#32016,#32017,#32018),.UNSPECIFIED.,.F.,.F.,(4,3,3,
3,3,3,3,4),(0.,0.000123360913700324,0.000259510379141672,0.00040648232915685,
0.000585460068616011,0.000594183385201068,0.000955339326765691,0.00118832361362475),
 .UNSPECIFIED.);
#817=CONICAL_SURFACE('',#11750,54.5,0.785398163397448);
#818=CONICAL_SURFACE('',#11761,54.5,0.785398163397448);
#819=CONICAL_SURFACE('',#11812,54.5,0.785398163397448);
#820=CONICAL_SURFACE('',#11898,48.4375,0.785398163397453);
#821=CONICAL_SURFACE('',#11922,48.4375,0.785398163397453);
#822=CONICAL_SURFACE('',#11927,54.5,0.785398163397448);
#823=CONICAL_SURFACE('',#11937,49.6875,0.785398163397442);
#824=CONICAL_SURFACE('',#11941,49.6875,0.785398163397442);
#825=CONICAL_SURFACE('',#11984,53.4375,0.785398163397454);
#826=CONICAL_SURFACE('',#12025,48.4375,0.785398163397453);
#827=CONICAL_SURFACE('',#12035,48.4375,0.785398163397453);
#828=CONICAL_SURFACE('',#12043,49.6875,0.785398163397442);
#829=CONICAL_SURFACE('',#12064,53.4375,0.785398163397454);
#830=CONICAL_SURFACE('',#12100,48.4375,0.785398163397453);
#831=CONICAL_SURFACE('',#12110,48.4375,0.785398163397453);
#832=CONICAL_SURFACE('',#12116,49.6875,0.785398163397442);
#833=CONICAL_SURFACE('',#12127,53.4375,0.785398163397454);
#834=CONICAL_SURFACE('',#12164,48.4375,0.785398163397453);
#835=CONICAL_SURFACE('',#12174,48.4375,0.785398163397453);
#836=CONICAL_SURFACE('',#12194,53.4375,0.785398163397454);
#837=TOROIDAL_SURFACE('',#11536,3.125,0.3125);
#838=TOROIDAL_SURFACE('',#11541,3.125,0.3125);
#839=TOROIDAL_SURFACE('',#11546,3.125,0.3125);
#840=TOROIDAL_SURFACE('',#11550,3.125,0.3125);
#841=TOROIDAL_SURFACE('',#11555,0.625,0.3125);
#842=TOROIDAL_SURFACE('',#11560,4.6875,0.3125);
#843=TOROIDAL_SURFACE('',#11565,1.25,0.3125);
#844=TOROIDAL_SURFACE('',#11570,4.0625,0.3125);
#845=TOROIDAL_SURFACE('',#11575,3.125,0.3125);
#846=TOROIDAL_SURFACE('',#11580,3.125,0.3125);
#847=TOROIDAL_SURFACE('',#11585,3.125,0.3125);
#848=TOROIDAL_SURFACE('',#11590,3.125,0.3125);
#849=TOROIDAL_SURFACE('',#11595,0.625,0.3125);
#850=TOROIDAL_SURFACE('',#11600,4.6875,0.3125);
#851=TOROIDAL_SURFACE('',#11605,1.25,0.3125);
#852=TOROIDAL_SURFACE('',#11610,4.0625,0.3125);
#853=TOROIDAL_SURFACE('',#11615,3.125,0.3125);
#854=TOROIDAL_SURFACE('',#11619,3.125,0.3125);
#855=TOROIDAL_SURFACE('',#11623,3.125,0.3125);
#856=TOROIDAL_SURFACE('',#11628,3.125,0.3125);
#857=TOROIDAL_SURFACE('',#11632,0.625,0.3125);
#858=TOROIDAL_SURFACE('',#11637,1.25,0.3125);
#859=TOROIDAL_SURFACE('',#11642,3.125,0.3125);
#860=TOROIDAL_SURFACE('',#11647,3.125,0.3125);
#861=TOROIDAL_SURFACE('',#11652,3.125,0.3125);
#862=TOROIDAL_SURFACE('',#11657,3.125,0.3125);
#863=TOROIDAL_SURFACE('',#11662,50.,0.3125);
#864=TOROIDAL_SURFACE('',#11667,50.,0.3125);
#865=TOROIDAL_SURFACE('',#11672,1.25,0.3125);
#866=TOROIDAL_SURFACE('',#11677,1.25,0.3125);
#867=TOROIDAL_SURFACE('',#11682,1.25,0.3125);
#868=TOROIDAL_SURFACE('',#11687,1.25,0.3125);
#869=TOROIDAL_SURFACE('',#11701,0.625,0.3125);
#870=TOROIDAL_SURFACE('',#11717,0.625,0.3125);
#871=TOROIDAL_SURFACE('',#11722,0.625,0.3125);
#872=TOROIDAL_SURFACE('',#11727,1.25,0.3125);
#873=TOROIDAL_SURFACE('',#12228,4.0625,0.3125);
#874=TOROIDAL_SURFACE('',#12230,1.25,0.3125);
#875=TOROIDAL_SURFACE('',#12236,1.25,0.3125);
#876=TOROIDAL_SURFACE('',#12238,1.25,0.3125);
#877=TOROIDAL_SURFACE('',#12240,54.6875,0.3125);
#878=TOROIDAL_SURFACE('',#12241,4.6875,0.3125);
#879=TOROIDAL_SURFACE('',#12243,0.625,0.3125);
#880=TOROIDAL_SURFACE('',#12249,0.625,0.3125);
#881=TOROIDAL_SURFACE('',#12251,0.625,0.3125);
#882=TOROIDAL_SURFACE('',#12253,55.3125,0.3125);
#883=TOROIDAL_SURFACE('',#12260,55.4955582617584,0.3125);
#884=TOROIDAL_SURFACE('',#12266,48.75,0.3125);
#885=TOROIDAL_SURFACE('',#12279,57.3169417382416,0.3125);
#886=TOROIDAL_SURFACE('',#12283,48.75,0.3125);
#887=TOROIDAL_SURFACE('',#12289,55.4955582617584,0.3125);
#888=TOROIDAL_SURFACE('',#12292,48.75,0.3125);
#889=TOROIDAL_SURFACE('',#12295,57.3169417382416,0.3125);
#890=TOROIDAL_SURFACE('',#12311,48.75,0.3125);
#891=TOROIDAL_SURFACE('',#12314,21.5625,0.3125);
#892=TOROIDAL_SURFACE('',#12318,48.75,0.3125);
#893=TOROIDAL_SURFACE('',#12321,57.3169417382416,0.3125);
#894=TOROIDAL_SURFACE('',#12329,55.4955582617584,0.3125);
#895=TOROIDAL_SURFACE('',#12334,57.3169417382416,0.3125);
#896=TOROIDAL_SURFACE('',#12338,48.75,0.3125);
#897=TOROIDAL_SURFACE('',#12348,48.125,0.3125);
#898=TOROIDAL_SURFACE('',#12357,55.4955582617584,0.3125);
#899=TOROIDAL_SURFACE('',#12363,48.75,0.3125);
#900=TOROIDAL_SURFACE('',#12366,0.625,0.3125);
#901=TOROIDAL_SURFACE('',#12368,21.5625,0.3125);
#902=TOROIDAL_SURFACE('',#12373,55.4955582617584,0.3125);
#903=TOROIDAL_SURFACE('',#12377,48.75,0.3125);
#904=TOROIDAL_SURFACE('',#12388,21.5625,0.3125);
#905=TOROIDAL_SURFACE('',#12392,0.625,0.3125);
#906=TOROIDAL_SURFACE('',#12399,57.3169417382416,0.3125);
#907=TOROIDAL_SURFACE('',#12403,48.75,0.3125);
#908=TOROIDAL_SURFACE('',#12407,21.5625,0.3125);
#909=TOROIDAL_SURFACE('',#12413,48.75,0.3125);
#910=TOROIDAL_SURFACE('',#12414,48.75,0.3125);
#911=TOROIDAL_SURFACE('',#12417,57.3169417382416,0.3125);
#912=TOROIDAL_SURFACE('',#12424,0.625,0.3125);
#913=TOROIDAL_SURFACE('',#12427,21.5625,0.3125);
#914=TOROIDAL_SURFACE('',#12431,48.125,0.3125);
#915=TOROIDAL_SURFACE('',#12439,55.4955582617584,0.3125);
#916=TOROIDAL_SURFACE('',#12442,0.625,0.3125);
#917=TOROIDAL_SURFACE('',#12453,48.125,0.3125);
#918=TOROIDAL_SURFACE('',#12461,48.75,0.3125);
#919=TOROIDAL_SURFACE('',#12464,0.625,0.3125);
#920=TOROIDAL_SURFACE('',#12469,55.4955582617584,0.3125);
#921=TOROIDAL_SURFACE('',#12473,48.75,0.3125);
#922=TOROIDAL_SURFACE('',#12476,21.5625,0.3125);
#923=TOROIDAL_SURFACE('',#12486,21.5625,0.3125);
#924=TOROIDAL_SURFACE('',#12489,57.3169417382416,0.3125);
#925=TOROIDAL_SURFACE('',#12498,48.125,0.3125);
#926=TOROIDAL_SURFACE('',#12501,21.5625,0.3125);
#927=TOROIDAL_SURFACE('',#12505,48.75,0.3125);
#928=TOROIDAL_SURFACE('',#12507,0.625,0.3125);
#929=TOROIDAL_SURFACE('',#12515,57.3169417382416,0.3125);
#930=TOROIDAL_SURFACE('',#12517,48.75,0.3125);
#931=TOROIDAL_SURFACE('',#12522,48.75,0.3125);
#932=TOROIDAL_SURFACE('',#12535,55.4955582617584,0.3125);
#933=TOROIDAL_SURFACE('',#12544,50.,0.3125);
#934=TOROIDAL_SURFACE('',#12546,50.8794417382416,0.3125);
#935=TOROIDAL_SURFACE('',#12556,1.25,0.3125);
#936=TOROIDAL_SURFACE('',#12559,50.,0.3125);
#937=TOROIDAL_SURFACE('',#12563,50.8794417382416,0.3125);
#938=TOROIDAL_SURFACE('',#12578,5.3125,0.3125);
#939=TOROIDAL_SURFACE('',#12584,54.6294417382416,0.3125);
#940=TOROIDAL_SURFACE('',#12592,50.8794417382416,0.3125);
#941=TOROIDAL_SURFACE('',#12600,1.25,0.3125);
#942=TOROIDAL_SURFACE('',#12602,5.3125,0.3125);
#943=TOROIDAL_SURFACE('',#12613,54.6294417382416,0.3125);
#944=TOROIDAL_SURFACE('',#12617,50.8794417382416,0.3125);
#945=TOROIDAL_SURFACE('',#12622,50.,0.3125);
#946=TOROIDAL_SURFACE('',#12630,5.3125,0.3125);
#947=TOROIDAL_SURFACE('',#12642,54.6294417382416,0.3125);
#948=TOROIDAL_SURFACE('',#12654,50.8794417382416,0.3125);
#949=TOROIDAL_SURFACE('',#12660,50.,0.3125);
#950=TOROIDAL_SURFACE('',#12663,5.3125,0.3125);
#951=TOROIDAL_SURFACE('',#12672,5.3125,0.3125);
#952=TOROIDAL_SURFACE('',#12681,54.6294417382416,0.3125);
#953=TOROIDAL_SURFACE('',#12685,50.,0.3125);
#954=TOROIDAL_SURFACE('',#12690,50.8794417382416,0.3125);
#955=TOROIDAL_SURFACE('',#12698,54.6294417382416,0.3125);
#956=TOROIDAL_SURFACE('',#12708,5.3125,0.3125);
#957=TOROIDAL_SURFACE('',#12716,50.,0.3125);
#958=TOROIDAL_SURFACE('',#12724,50.8794417382416,0.3125);
#959=TOROIDAL_SURFACE('',#12730,5.3125,0.3125);
#960=TOROIDAL_SURFACE('',#12737,1.25,0.3125);
#961=TOROIDAL_SURFACE('',#12743,54.6294417382416,0.3125);
#962=TOROIDAL_SURFACE('',#12748,50.8794417382416,0.3125);
#963=TOROIDAL_SURFACE('',#12754,54.6294417382416,0.3125);
#964=TOROIDAL_SURFACE('',#12757,5.3125,0.3125);
#965=TOROIDAL_SURFACE('',#12777,1.25,0.3125);
#966=TOROIDAL_SURFACE('',#12782,54.6294417382416,0.3125);
#967=TOROIDAL_SURFACE('',#12800,53.5669417382416,0.3125);
#968=TOROIDAL_SURFACE('',#12805,53.5669417382416,0.3125);
#969=TOROIDAL_SURFACE('',#12809,48.75,0.3125);
#970=TOROIDAL_SURFACE('',#12810,48.75,0.3125);
#971=TOROIDAL_SURFACE('',#12811,53.5669417382416,0.3125);
#972=TOROIDAL_SURFACE('',#12818,48.75,0.3125);
#973=TOROIDAL_SURFACE('',#12819,48.75,0.3125);
#974=TOROIDAL_SURFACE('',#12822,53.5669417382416,0.3125);
#975=TOROIDAL_SURFACE('',#12825,5.3125,0.3125);
#976=TOROIDAL_SURFACE('',#12832,5.3125,0.3125);
#977=TOROIDAL_SURFACE('',#12834,5.3125,0.3125);
#978=TOROIDAL_SURFACE('',#12840,5.3125,0.3125);
#979=TOROIDAL_SURFACE('',#12841,5.3125,0.3125);
#980=TOROIDAL_SURFACE('',#12848,5.3125,0.3125);
#981=TOROIDAL_SURFACE('',#12850,5.3125,0.3125);
#982=TOROIDAL_SURFACE('',#12856,5.3125,0.3125);
#983=TOROIDAL_SURFACE('',#12857,4.0625,0.3125);
#984=TOROIDAL_SURFACE('',#12859,1.25,0.3125);
#985=TOROIDAL_SURFACE('',#12866,1.25,0.3125);
#986=TOROIDAL_SURFACE('',#12868,1.25,0.3125);
#987=TOROIDAL_SURFACE('',#12870,54.6875,0.3125);
#988=TOROIDAL_SURFACE('',#12871,4.6875,0.3125);
#989=TOROIDAL_SURFACE('',#12873,0.625,0.3125);
#990=TOROIDAL_SURFACE('',#12880,0.625,0.3125);
#991=TOROIDAL_SURFACE('',#12882,0.625,0.3125);
#992=TOROIDAL_SURFACE('',#12884,55.3125,0.3125);
#993=TOROIDAL_SURFACE('',#12885,1.25,0.3125);
#994=TOROIDAL_SURFACE('',#12887,1.25,0.3125);
#995=TOROIDAL_SURFACE('',#12892,1.25,0.3125);
#996=TOROIDAL_SURFACE('',#12894,54.6875,0.3125);
#997=TOROIDAL_SURFACE('',#12895,0.625,0.3125);
#998=TOROIDAL_SURFACE('',#12897,0.625,0.3125);
#999=TOROIDAL_SURFACE('',#12902,0.625,0.3125);
#1000=TOROIDAL_SURFACE('',#12904,55.3125,0.3125);
#1001=TOROIDAL_SURFACE('',#12905,1.25,0.3125);
#1002=TOROIDAL_SURFACE('',#12907,1.25,0.3125);
#1003=TOROIDAL_SURFACE('',#12912,1.25,0.3125);
#1004=TOROIDAL_SURFACE('',#12914,54.6875,0.3125);
#1005=TOROIDAL_SURFACE('',#12915,0.625,0.3125);
#1006=TOROIDAL_SURFACE('',#12917,0.625,0.3125);
#1007=TOROIDAL_SURFACE('',#12922,0.625,0.3125);
#1008=TOROIDAL_SURFACE('',#12924,55.3125,0.3125);
#1012=FACE_OUTER_BOUND('',#1759,.T.);
#1013=FACE_OUTER_BOUND('',#1760,.T.);
#1014=FACE_OUTER_BOUND('',#1761,.T.);
#1015=FACE_OUTER_BOUND('',#1762,.T.);
#1016=FACE_OUTER_BOUND('',#1763,.T.);
#1017=FACE_OUTER_BOUND('',#1764,.T.);
#1018=FACE_OUTER_BOUND('',#1765,.T.);
#1019=FACE_OUTER_BOUND('',#1766,.T.);
#1020=FACE_OUTER_BOUND('',#1767,.T.);
#1021=FACE_OUTER_BOUND('',#1768,.T.);
#1022=FACE_OUTER_BOUND('',#1769,.T.);
#1023=FACE_OUTER_BOUND('',#1770,.T.);
#1024=FACE_OUTER_BOUND('',#1771,.T.);
#1025=FACE_OUTER_BOUND('',#1772,.T.);
#1026=FACE_OUTER_BOUND('',#1773,.T.);
#1027=FACE_OUTER_BOUND('',#1774,.T.);
#1028=FACE_OUTER_BOUND('',#1775,.T.);
#1029=FACE_OUTER_BOUND('',#1776,.T.);
#1030=FACE_OUTER_BOUND('',#1777,.T.);
#1031=FACE_OUTER_BOUND('',#1778,.T.);
#1032=FACE_OUTER_BOUND('',#1779,.T.);
#1033=FACE_OUTER_BOUND('',#1780,.T.);
#1034=FACE_OUTER_BOUND('',#1781,.T.);
#1035=FACE_OUTER_BOUND('',#1782,.T.);
#1036=FACE_OUTER_BOUND('',#1783,.T.);
#1037=FACE_OUTER_BOUND('',#1784,.T.);
#1038=FACE_OUTER_BOUND('',#1785,.T.);
#1039=FACE_OUTER_BOUND('',#1786,.T.);
#1040=FACE_OUTER_BOUND('',#1787,.T.);
#1041=FACE_OUTER_BOUND('',#1788,.T.);
#1042=FACE_OUTER_BOUND('',#1789,.T.);
#1043=FACE_OUTER_BOUND('',#1790,.T.);
#1044=FACE_OUTER_BOUND('',#1791,.T.);
#1045=FACE_OUTER_BOUND('',#1792,.T.);
#1046=FACE_OUTER_BOUND('',#1793,.T.);
#1047=FACE_OUTER_BOUND('',#1794,.T.);
#1048=FACE_OUTER_BOUND('',#1795,.T.);
#1049=FACE_OUTER_BOUND('',#1796,.T.);
#1050=FACE_OUTER_BOUND('',#1797,.T.);
#1051=FACE_OUTER_BOUND('',#1798,.T.);
#1052=FACE_OUTER_BOUND('',#1799,.T.);
#1053=FACE_OUTER_BOUND('',#1800,.T.);
#1054=FACE_OUTER_BOUND('',#1801,.T.);
#1055=FACE_OUTER_BOUND('',#1802,.T.);
#1056=FACE_OUTER_BOUND('',#1803,.T.);
#1057=FACE_OUTER_BOUND('',#1804,.T.);
#1058=FACE_OUTER_BOUND('',#1805,.T.);
#1059=FACE_OUTER_BOUND('',#1806,.T.);
#1060=FACE_OUTER_BOUND('',#1807,.T.);
#1061=FACE_OUTER_BOUND('',#1808,.T.);
#1062=FACE_OUTER_BOUND('',#1809,.T.);
#1063=FACE_OUTER_BOUND('',#1810,.T.);
#1064=FACE_OUTER_BOUND('',#1811,.T.);
#1065=FACE_OUTER_BOUND('',#1812,.T.);
#1066=FACE_OUTER_BOUND('',#1813,.T.);
#1067=FACE_OUTER_BOUND('',#1814,.T.);
#1068=FACE_OUTER_BOUND('',#1815,.T.);
#1069=FACE_OUTER_BOUND('',#1816,.T.);
#1070=FACE_OUTER_BOUND('',#1817,.T.);
#1071=FACE_OUTER_BOUND('',#1818,.T.);
#1072=FACE_OUTER_BOUND('',#1819,.T.);
#1073=FACE_OUTER_BOUND('',#1820,.T.);
#1074=FACE_OUTER_BOUND('',#1821,.T.);
#1075=FACE_OUTER_BOUND('',#1822,.T.);
#1076=FACE_OUTER_BOUND('',#1823,.T.);
#1077=FACE_OUTER_BOUND('',#1824,.T.);
#1078=FACE_OUTER_BOUND('',#1825,.T.);
#1079=FACE_OUTER_BOUND('',#1826,.T.);
#1080=FACE_OUTER_BOUND('',#1827,.T.);
#1081=FACE_OUTER_BOUND('',#1828,.T.);
#1082=FACE_OUTER_BOUND('',#1829,.T.);
#1083=FACE_OUTER_BOUND('',#1830,.T.);
#1084=FACE_OUTER_BOUND('',#1831,.T.);
#1085=FACE_OUTER_BOUND('',#1840,.T.);
#1086=FACE_OUTER_BOUND('',#1841,.T.);
#1087=FACE_OUTER_BOUND('',#1842,.T.);
#1088=FACE_OUTER_BOUND('',#1844,.T.);
#1089=FACE_OUTER_BOUND('',#1846,.T.);
#1090=FACE_OUTER_BOUND('',#1847,.T.);
#1091=FACE_OUTER_BOUND('',#1848,.T.);
#1092=FACE_OUTER_BOUND('',#1849,.T.);
#1093=FACE_OUTER_BOUND('',#1850,.T.);
#1094=FACE_OUTER_BOUND('',#1851,.T.);
#1095=FACE_OUTER_BOUND('',#1852,.T.);
#1096=FACE_OUTER_BOUND('',#1853,.T.);
#1097=FACE_OUTER_BOUND('',#1854,.T.);
#1098=FACE_OUTER_BOUND('',#1855,.T.);
#1099=FACE_OUTER_BOUND('',#1856,.T.);
#1100=FACE_OUTER_BOUND('',#1858,.T.);
#1101=FACE_OUTER_BOUND('',#1859,.T.);
#1102=FACE_OUTER_BOUND('',#1860,.T.);
#1103=FACE_OUTER_BOUND('',#1861,.T.);
#1104=FACE_OUTER_BOUND('',#1862,.T.);
#1105=FACE_OUTER_BOUND('',#1863,.T.);
#1106=FACE_OUTER_BOUND('',#1864,.T.);
#1107=FACE_OUTER_BOUND('',#1865,.T.);
#1108=FACE_OUTER_BOUND('',#1866,.T.);
#1109=FACE_OUTER_BOUND('',#1867,.T.);
#1110=FACE_OUTER_BOUND('',#1868,.T.);
#1111=FACE_OUTER_BOUND('',#1869,.T.);
#1112=FACE_OUTER_BOUND('',#1870,.T.);
#1113=FACE_OUTER_BOUND('',#1871,.T.);
#1114=FACE_OUTER_BOUND('',#1872,.T.);
#1115=FACE_OUTER_BOUND('',#1874,.T.);
#1116=FACE_OUTER_BOUND('',#1876,.T.);
#1117=FACE_OUTER_BOUND('',#1877,.T.);
#1118=FACE_OUTER_BOUND('',#1878,.T.);
#1119=FACE_OUTER_BOUND('',#1879,.T.);
#1120=FACE_OUTER_BOUND('',#1880,.T.);
#1121=FACE_OUTER_BOUND('',#1881,.T.);
#1122=FACE_OUTER_BOUND('',#1890,.T.);
#1123=FACE_OUTER_BOUND('',#1891,.T.);
#1124=FACE_OUTER_BOUND('',#1892,.T.);
#1125=FACE_OUTER_BOUND('',#1893,.T.);
#1126=FACE_OUTER_BOUND('',#1894,.T.);
#1127=FACE_OUTER_BOUND('',#1895,.T.);
#1128=FACE_OUTER_BOUND('',#1896,.T.);
#1129=FACE_OUTER_BOUND('',#1897,.T.);
#1130=FACE_OUTER_BOUND('',#1898,.T.);
#1131=FACE_OUTER_BOUND('',#1899,.T.);
#1132=FACE_OUTER_BOUND('',#1900,.T.);
#1133=FACE_OUTER_BOUND('',#1901,.T.);
#1134=FACE_OUTER_BOUND('',#1902,.T.);
#1135=FACE_OUTER_BOUND('',#1903,.T.);
#1136=FACE_OUTER_BOUND('',#1904,.T.);
#1137=FACE_OUTER_BOUND('',#1905,.T.);
#1138=FACE_OUTER_BOUND('',#1906,.T.);
#1139=FACE_OUTER_BOUND('',#1907,.T.);
#1140=FACE_OUTER_BOUND('',#1908,.T.);
#1141=FACE_OUTER_BOUND('',#1909,.T.);
#1142=FACE_OUTER_BOUND('',#1910,.T.);
#1143=FACE_OUTER_BOUND('',#1911,.T.);
#1144=FACE_OUTER_BOUND('',#1912,.T.);
#1145=FACE_OUTER_BOUND('',#1913,.T.);
#1146=FACE_OUTER_BOUND('',#1914,.T.);
#1147=FACE_OUTER_BOUND('',#1916,.T.);
#1148=FACE_OUTER_BOUND('',#1918,.T.);
#1149=FACE_OUTER_BOUND('',#1919,.T.);
#1150=FACE_OUTER_BOUND('',#1920,.T.);
#1151=FACE_OUTER_BOUND('',#1921,.T.);
#1152=FACE_OUTER_BOUND('',#1922,.T.);
#1153=FACE_OUTER_BOUND('',#1923,.T.);
#1154=FACE_OUTER_BOUND('',#1924,.T.);
#1155=FACE_OUTER_BOUND('',#1925,.T.);
#1156=FACE_OUTER_BOUND('',#1926,.T.);
#1157=FACE_OUTER_BOUND('',#1927,.T.);
#1158=FACE_OUTER_BOUND('',#1928,.T.);
#1159=FACE_OUTER_BOUND('',#1929,.T.);
#1160=FACE_OUTER_BOUND('',#1930,.T.);
#1161=FACE_OUTER_BOUND('',#1931,.T.);
#1162=FACE_OUTER_BOUND('',#1932,.T.);
#1163=FACE_OUTER_BOUND('',#1933,.T.);
#1164=FACE_OUTER_BOUND('',#1934,.T.);
#1165=FACE_OUTER_BOUND('',#1935,.T.);
#1166=FACE_OUTER_BOUND('',#1936,.T.);
#1167=FACE_OUTER_BOUND('',#1937,.T.);
#1168=FACE_OUTER_BOUND('',#1938,.T.);
#1169=FACE_OUTER_BOUND('',#1939,.T.);
#1170=FACE_OUTER_BOUND('',#1940,.T.);
#1171=FACE_OUTER_BOUND('',#1941,.T.);
#1172=FACE_OUTER_BOUND('',#1942,.T.);
#1173=FACE_OUTER_BOUND('',#1943,.T.);
#1174=FACE_OUTER_BOUND('',#1944,.T.);
#1175=FACE_OUTER_BOUND('',#1945,.T.);
#1176=FACE_OUTER_BOUND('',#1946,.T.);
#1177=FACE_OUTER_BOUND('',#1947,.T.);
#1178=FACE_OUTER_BOUND('',#1948,.T.);
#1179=FACE_OUTER_BOUND('',#1949,.T.);
#1180=FACE_OUTER_BOUND('',#1950,.T.);
#1181=FACE_OUTER_BOUND('',#1951,.T.);
#1182=FACE_OUTER_BOUND('',#1952,.T.);
#1183=FACE_OUTER_BOUND('',#1953,.T.);
#1184=FACE_OUTER_BOUND('',#1954,.T.);
#1185=FACE_OUTER_BOUND('',#1955,.T.);
#1186=FACE_OUTER_BOUND('',#1956,.T.);
#1187=FACE_OUTER_BOUND('',#1957,.T.);
#1188=FACE_OUTER_BOUND('',#1958,.T.);
#1189=FACE_OUTER_BOUND('',#1959,.T.);
#1190=FACE_OUTER_BOUND('',#1960,.T.);
#1191=FACE_OUTER_BOUND('',#1961,.T.);
#1192=FACE_OUTER_BOUND('',#1962,.T.);
#1193=FACE_OUTER_BOUND('',#1963,.T.);
#1194=FACE_OUTER_BOUND('',#1964,.T.);
#1195=FACE_OUTER_BOUND('',#1965,.T.);
#1196=FACE_OUTER_BOUND('',#1966,.T.);
#1197=FACE_OUTER_BOUND('',#1967,.T.);
#1198=FACE_OUTER_BOUND('',#1968,.T.);
#1199=FACE_OUTER_BOUND('',#1970,.T.);
#1200=FACE_OUTER_BOUND('',#1972,.T.);
#1201=FACE_OUTER_BOUND('',#1973,.T.);
#1202=FACE_OUTER_BOUND('',#1974,.T.);
#1203=FACE_OUTER_BOUND('',#1975,.T.);
#1204=FACE_OUTER_BOUND('',#1976,.T.);
#1205=FACE_OUTER_BOUND('',#1977,.T.);
#1206=FACE_OUTER_BOUND('',#1978,.T.);
#1207=FACE_OUTER_BOUND('',#1979,.T.);
#1208=FACE_OUTER_BOUND('',#1980,.T.);
#1209=FACE_OUTER_BOUND('',#1981,.T.);
#1210=FACE_OUTER_BOUND('',#1982,.T.);
#1211=FACE_OUTER_BOUND('',#1983,.T.);
#1212=FACE_OUTER_BOUND('',#1984,.T.);
#1213=FACE_OUTER_BOUND('',#1985,.T.);
#1214=FACE_OUTER_BOUND('',#1986,.T.);
#1215=FACE_OUTER_BOUND('',#1987,.T.);
#1216=FACE_OUTER_BOUND('',#1988,.T.);
#1217=FACE_OUTER_BOUND('',#1989,.T.);
#1218=FACE_OUTER_BOUND('',#1990,.T.);
#1219=FACE_OUTER_BOUND('',#1991,.T.);
#1220=FACE_OUTER_BOUND('',#1992,.T.);
#1221=FACE_OUTER_BOUND('',#1993,.T.);
#1222=FACE_OUTER_BOUND('',#1994,.T.);
#1223=FACE_OUTER_BOUND('',#1995,.T.);
#1224=FACE_OUTER_BOUND('',#1996,.T.);
#1225=FACE_OUTER_BOUND('',#1997,.T.);
#1226=FACE_OUTER_BOUND('',#1998,.T.);
#1227=FACE_OUTER_BOUND('',#1999,.T.);
#1228=FACE_OUTER_BOUND('',#2000,.T.);
#1229=FACE_OUTER_BOUND('',#2001,.T.);
#1230=FACE_OUTER_BOUND('',#2002,.T.);
#1231=FACE_OUTER_BOUND('',#2003,.T.);
#1232=FACE_OUTER_BOUND('',#2004,.T.);
#1233=FACE_OUTER_BOUND('',#2005,.T.);
#1234=FACE_OUTER_BOUND('',#2006,.T.);
#1235=FACE_OUTER_BOUND('',#2007,.T.);
#1236=FACE_OUTER_BOUND('',#2008,.T.);
#1237=FACE_OUTER_BOUND('',#2009,.T.);
#1238=FACE_OUTER_BOUND('',#2010,.T.);
#1239=FACE_OUTER_BOUND('',#2011,.T.);
#1240=FACE_OUTER_BOUND('',#2012,.T.);
#1241=FACE_OUTER_BOUND('',#2013,.T.);
#1242=FACE_OUTER_BOUND('',#2014,.T.);
#1243=FACE_OUTER_BOUND('',#2015,.T.);
#1244=FACE_OUTER_BOUND('',#2016,.T.);
#1245=FACE_OUTER_BOUND('',#2017,.T.);
#1246=FACE_OUTER_BOUND('',#2018,.T.);
#1247=FACE_OUTER_BOUND('',#2019,.T.);
#1248=FACE_OUTER_BOUND('',#2020,.T.);
#1249=FACE_OUTER_BOUND('',#2021,.T.);
#1250=FACE_OUTER_BOUND('',#2022,.T.);
#1251=FACE_OUTER_BOUND('',#2023,.T.);
#1252=FACE_OUTER_BOUND('',#2024,.T.);
#1253=FACE_OUTER_BOUND('',#2025,.T.);
#1254=FACE_OUTER_BOUND('',#2026,.T.);
#1255=FACE_OUTER_BOUND('',#2027,.T.);
#1256=FACE_OUTER_BOUND('',#2028,.T.);
#1257=FACE_OUTER_BOUND('',#2029,.T.);
#1258=FACE_OUTER_BOUND('',#2030,.T.);
#1259=FACE_OUTER_BOUND('',#2031,.T.);
#1260=FACE_OUTER_BOUND('',#2032,.T.);
#1261=FACE_OUTER_BOUND('',#2033,.T.);
#1262=FACE_OUTER_BOUND('',#2034,.T.);
#1263=FACE_OUTER_BOUND('',#2035,.T.);
#1264=FACE_OUTER_BOUND('',#2036,.T.);
#1265=FACE_OUTER_BOUND('',#2037,.T.);
#1266=FACE_OUTER_BOUND('',#2038,.T.);
#1267=FACE_OUTER_BOUND('',#2039,.T.);
#1268=FACE_OUTER_BOUND('',#2040,.T.);
#1269=FACE_OUTER_BOUND('',#2041,.T.);
#1270=FACE_OUTER_BOUND('',#2042,.T.);
#1271=FACE_OUTER_BOUND('',#2043,.T.);
#1272=FACE_OUTER_BOUND('',#2044,.T.);
#1273=FACE_OUTER_BOUND('',#2045,.T.);
#1274=FACE_OUTER_BOUND('',#2046,.T.);
#1275=FACE_OUTER_BOUND('',#2047,.T.);
#1276=FACE_OUTER_BOUND('',#2048,.T.);
#1277=FACE_OUTER_BOUND('',#2049,.T.);
#1278=FACE_OUTER_BOUND('',#2050,.T.);
#1279=FACE_OUTER_BOUND('',#2051,.T.);
#1280=FACE_OUTER_BOUND('',#2052,.T.);
#1281=FACE_OUTER_BOUND('',#2053,.T.);
#1282=FACE_OUTER_BOUND('',#2054,.T.);
#1283=FACE_OUTER_BOUND('',#2055,.T.);
#1284=FACE_OUTER_BOUND('',#2056,.T.);
#1285=FACE_OUTER_BOUND('',#2057,.T.);
#1286=FACE_OUTER_BOUND('',#2058,.T.);
#1287=FACE_OUTER_BOUND('',#2059,.T.);
#1288=FACE_OUTER_BOUND('',#2060,.T.);
#1289=FACE_OUTER_BOUND('',#2061,.T.);
#1290=FACE_OUTER_BOUND('',#2062,.T.);
#1291=FACE_OUTER_BOUND('',#2063,.T.);
#1292=FACE_OUTER_BOUND('',#2064,.T.);
#1293=FACE_OUTER_BOUND('',#2065,.T.);
#1294=FACE_OUTER_BOUND('',#2066,.T.);
#1295=FACE_OUTER_BOUND('',#2067,.T.);
#1296=FACE_OUTER_BOUND('',#2068,.T.);
#1297=FACE_OUTER_BOUND('',#2069,.T.);
#1298=FACE_OUTER_BOUND('',#2070,.T.);
#1299=FACE_OUTER_BOUND('',#2071,.T.);
#1300=FACE_OUTER_BOUND('',#2072,.T.);
#1301=FACE_OUTER_BOUND('',#2073,.T.);
#1302=FACE_OUTER_BOUND('',#2074,.T.);
#1303=FACE_OUTER_BOUND('',#2075,.T.);
#1304=FACE_OUTER_BOUND('',#2076,.T.);
#1305=FACE_OUTER_BOUND('',#2077,.T.);
#1306=FACE_OUTER_BOUND('',#2078,.T.);
#1307=FACE_OUTER_BOUND('',#2079,.T.);
#1308=FACE_OUTER_BOUND('',#2080,.T.);
#1309=FACE_OUTER_BOUND('',#2081,.T.);
#1310=FACE_OUTER_BOUND('',#2082,.T.);
#1311=FACE_OUTER_BOUND('',#2083,.T.);
#1312=FACE_OUTER_BOUND('',#2084,.T.);
#1313=FACE_OUTER_BOUND('',#2085,.T.);
#1314=FACE_OUTER_BOUND('',#2086,.T.);
#1315=FACE_OUTER_BOUND('',#2087,.T.);
#1316=FACE_OUTER_BOUND('',#2088,.T.);
#1317=FACE_OUTER_BOUND('',#2089,.T.);
#1318=FACE_OUTER_BOUND('',#2090,.T.);
#1319=FACE_OUTER_BOUND('',#2091,.T.);
#1320=FACE_OUTER_BOUND('',#2092,.T.);
#1321=FACE_OUTER_BOUND('',#2093,.T.);
#1322=FACE_OUTER_BOUND('',#2094,.T.);
#1323=FACE_OUTER_BOUND('',#2095,.T.);
#1324=FACE_OUTER_BOUND('',#2096,.T.);
#1325=FACE_OUTER_BOUND('',#2097,.T.);
#1326=FACE_OUTER_BOUND('',#2098,.T.);
#1327=FACE_OUTER_BOUND('',#2099,.T.);
#1328=FACE_OUTER_BOUND('',#2100,.T.);
#1329=FACE_OUTER_BOUND('',#2101,.T.);
#1330=FACE_OUTER_BOUND('',#2102,.T.);
#1331=FACE_OUTER_BOUND('',#2103,.T.);
#1332=FACE_OUTER_BOUND('',#2104,.T.);
#1333=FACE_OUTER_BOUND('',#2105,.T.);
#1334=FACE_OUTER_BOUND('',#2106,.T.);
#1335=FACE_OUTER_BOUND('',#2107,.T.);
#1336=FACE_OUTER_BOUND('',#2108,.T.);
#1337=FACE_OUTER_BOUND('',#2109,.T.);
#1338=FACE_OUTER_BOUND('',#2110,.T.);
#1339=FACE_OUTER_BOUND('',#2111,.T.);
#1340=FACE_OUTER_BOUND('',#2112,.T.);
#1341=FACE_OUTER_BOUND('',#2113,.T.);
#1342=FACE_OUTER_BOUND('',#2114,.T.);
#1343=FACE_OUTER_BOUND('',#2115,.T.);
#1344=FACE_OUTER_BOUND('',#2116,.T.);
#1345=FACE_OUTER_BOUND('',#2117,.T.);
#1346=FACE_OUTER_BOUND('',#2118,.T.);
#1347=FACE_OUTER_BOUND('',#2119,.T.);
#1348=FACE_OUTER_BOUND('',#2120,.T.);
#1349=FACE_OUTER_BOUND('',#2121,.T.);
#1350=FACE_OUTER_BOUND('',#2122,.T.);
#1351=FACE_OUTER_BOUND('',#2123,.T.);
#1352=FACE_OUTER_BOUND('',#2124,.T.);
#1353=FACE_OUTER_BOUND('',#2125,.T.);
#1354=FACE_OUTER_BOUND('',#2126,.T.);
#1355=FACE_OUTER_BOUND('',#2127,.T.);
#1356=FACE_OUTER_BOUND('',#2128,.T.);
#1357=FACE_OUTER_BOUND('',#2129,.T.);
#1358=FACE_OUTER_BOUND('',#2130,.T.);
#1359=FACE_OUTER_BOUND('',#2131,.T.);
#1360=FACE_OUTER_BOUND('',#2132,.T.);
#1361=FACE_OUTER_BOUND('',#2133,.T.);
#1362=FACE_OUTER_BOUND('',#2134,.T.);
#1363=FACE_OUTER_BOUND('',#2135,.T.);
#1364=FACE_OUTER_BOUND('',#2136,.T.);
#1365=FACE_OUTER_BOUND('',#2137,.T.);
#1366=FACE_OUTER_BOUND('',#2138,.T.);
#1367=FACE_OUTER_BOUND('',#2139,.T.);
#1368=FACE_OUTER_BOUND('',#2140,.T.);
#1369=FACE_OUTER_BOUND('',#2141,.T.);
#1370=FACE_OUTER_BOUND('',#2142,.T.);
#1371=FACE_OUTER_BOUND('',#2143,.T.);
#1372=FACE_OUTER_BOUND('',#2144,.T.);
#1373=FACE_OUTER_BOUND('',#2145,.T.);
#1374=FACE_OUTER_BOUND('',#2146,.T.);
#1375=FACE_OUTER_BOUND('',#2147,.T.);
#1376=FACE_OUTER_BOUND('',#2148,.T.);
#1377=FACE_OUTER_BOUND('',#2149,.T.);
#1378=FACE_OUTER_BOUND('',#2150,.T.);
#1379=FACE_OUTER_BOUND('',#2151,.T.);
#1380=FACE_OUTER_BOUND('',#2152,.T.);
#1381=FACE_OUTER_BOUND('',#2153,.T.);
#1382=FACE_OUTER_BOUND('',#2154,.T.);
#1383=FACE_OUTER_BOUND('',#2155,.T.);
#1384=FACE_OUTER_BOUND('',#2156,.T.);
#1385=FACE_OUTER_BOUND('',#2157,.T.);
#1386=FACE_OUTER_BOUND('',#2158,.T.);
#1387=FACE_OUTER_BOUND('',#2159,.T.);
#1388=FACE_OUTER_BOUND('',#2160,.T.);
#1389=FACE_OUTER_BOUND('',#2161,.T.);
#1390=FACE_OUTER_BOUND('',#2162,.T.);
#1391=FACE_OUTER_BOUND('',#2163,.T.);
#1392=FACE_OUTER_BOUND('',#2164,.T.);
#1393=FACE_OUTER_BOUND('',#2165,.T.);
#1394=FACE_OUTER_BOUND('',#2166,.T.);
#1395=FACE_OUTER_BOUND('',#2167,.T.);
#1396=FACE_OUTER_BOUND('',#2168,.T.);
#1397=FACE_OUTER_BOUND('',#2169,.T.);
#1398=FACE_OUTER_BOUND('',#2170,.T.);
#1399=FACE_OUTER_BOUND('',#2171,.T.);
#1400=FACE_OUTER_BOUND('',#2172,.T.);
#1401=FACE_OUTER_BOUND('',#2173,.T.);
#1402=FACE_OUTER_BOUND('',#2174,.T.);
#1403=FACE_OUTER_BOUND('',#2175,.T.);
#1404=FACE_OUTER_BOUND('',#2176,.T.);
#1405=FACE_OUTER_BOUND('',#2177,.T.);
#1406=FACE_OUTER_BOUND('',#2178,.T.);
#1407=FACE_OUTER_BOUND('',#2179,.T.);
#1408=FACE_OUTER_BOUND('',#2180,.T.);
#1409=FACE_OUTER_BOUND('',#2181,.T.);
#1410=FACE_OUTER_BOUND('',#2182,.T.);
#1411=FACE_OUTER_BOUND('',#2183,.T.);
#1412=FACE_OUTER_BOUND('',#2184,.T.);
#1413=FACE_OUTER_BOUND('',#2185,.T.);
#1414=FACE_OUTER_BOUND('',#2186,.T.);
#1415=FACE_OUTER_BOUND('',#2187,.T.);
#1416=FACE_OUTER_BOUND('',#2188,.T.);
#1417=FACE_OUTER_BOUND('',#2189,.T.);
#1418=FACE_OUTER_BOUND('',#2190,.T.);
#1419=FACE_OUTER_BOUND('',#2191,.T.);
#1420=FACE_OUTER_BOUND('',#2192,.T.);
#1421=FACE_OUTER_BOUND('',#2193,.T.);
#1422=FACE_OUTER_BOUND('',#2194,.T.);
#1423=FACE_OUTER_BOUND('',#2195,.T.);
#1424=FACE_OUTER_BOUND('',#2196,.T.);
#1425=FACE_OUTER_BOUND('',#2197,.T.);
#1426=FACE_OUTER_BOUND('',#2198,.T.);
#1427=FACE_OUTER_BOUND('',#2199,.T.);
#1428=FACE_OUTER_BOUND('',#2200,.T.);
#1429=FACE_OUTER_BOUND('',#2201,.T.);
#1430=FACE_OUTER_BOUND('',#2202,.T.);
#1431=FACE_OUTER_BOUND('',#2203,.T.);
#1432=FACE_OUTER_BOUND('',#2204,.T.);
#1433=FACE_OUTER_BOUND('',#2205,.T.);
#1434=FACE_OUTER_BOUND('',#2206,.T.);
#1435=FACE_OUTER_BOUND('',#2207,.T.);
#1436=FACE_OUTER_BOUND('',#2208,.T.);
#1437=FACE_OUTER_BOUND('',#2209,.T.);
#1438=FACE_OUTER_BOUND('',#2210,.T.);
#1439=FACE_OUTER_BOUND('',#2211,.T.);
#1440=FACE_OUTER_BOUND('',#2212,.T.);
#1441=FACE_OUTER_BOUND('',#2213,.T.);
#1442=FACE_OUTER_BOUND('',#2214,.T.);
#1443=FACE_OUTER_BOUND('',#2215,.T.);
#1444=FACE_OUTER_BOUND('',#2216,.T.);
#1445=FACE_OUTER_BOUND('',#2217,.T.);
#1446=FACE_OUTER_BOUND('',#2218,.T.);
#1447=FACE_OUTER_BOUND('',#2219,.T.);
#1448=FACE_OUTER_BOUND('',#2220,.T.);
#1449=FACE_OUTER_BOUND('',#2221,.T.);
#1450=FACE_OUTER_BOUND('',#2222,.T.);
#1451=FACE_OUTER_BOUND('',#2223,.T.);
#1452=FACE_OUTER_BOUND('',#2224,.T.);
#1453=FACE_OUTER_BOUND('',#2225,.T.);
#1454=FACE_OUTER_BOUND('',#2226,.T.);
#1455=FACE_OUTER_BOUND('',#2227,.T.);
#1456=FACE_OUTER_BOUND('',#2228,.T.);
#1457=FACE_OUTER_BOUND('',#2229,.T.);
#1458=FACE_OUTER_BOUND('',#2230,.T.);
#1459=FACE_OUTER_BOUND('',#2231,.T.);
#1460=FACE_OUTER_BOUND('',#2232,.T.);
#1461=FACE_OUTER_BOUND('',#2233,.T.);
#1462=FACE_OUTER_BOUND('',#2234,.T.);
#1463=FACE_OUTER_BOUND('',#2235,.T.);
#1464=FACE_OUTER_BOUND('',#2236,.T.);
#1465=FACE_OUTER_BOUND('',#2237,.T.);
#1466=FACE_OUTER_BOUND('',#2238,.T.);
#1467=FACE_OUTER_BOUND('',#2239,.T.);
#1468=FACE_OUTER_BOUND('',#2240,.T.);
#1469=FACE_OUTER_BOUND('',#2241,.T.);
#1470=FACE_OUTER_BOUND('',#2242,.T.);
#1471=FACE_OUTER_BOUND('',#2243,.T.);
#1472=FACE_OUTER_BOUND('',#2244,.T.);
#1473=FACE_OUTER_BOUND('',#2245,.T.);
#1474=FACE_OUTER_BOUND('',#2246,.T.);
#1475=FACE_OUTER_BOUND('',#2247,.T.);
#1476=FACE_OUTER_BOUND('',#2248,.T.);
#1477=FACE_OUTER_BOUND('',#2249,.T.);
#1478=FACE_OUTER_BOUND('',#2250,.T.);
#1479=FACE_OUTER_BOUND('',#2251,.T.);
#1480=FACE_OUTER_BOUND('',#2252,.T.);
#1481=FACE_OUTER_BOUND('',#2253,.T.);
#1482=FACE_OUTER_BOUND('',#2254,.T.);
#1483=FACE_OUTER_BOUND('',#2255,.T.);
#1484=FACE_OUTER_BOUND('',#2256,.T.);
#1485=FACE_OUTER_BOUND('',#2257,.T.);
#1486=FACE_OUTER_BOUND('',#2258,.T.);
#1487=FACE_OUTER_BOUND('',#2259,.T.);
#1488=FACE_OUTER_BOUND('',#2260,.T.);
#1489=FACE_OUTER_BOUND('',#2261,.T.);
#1490=FACE_OUTER_BOUND('',#2262,.T.);
#1491=FACE_OUTER_BOUND('',#2263,.T.);
#1492=FACE_OUTER_BOUND('',#2264,.T.);
#1493=FACE_OUTER_BOUND('',#2265,.T.);
#1494=FACE_OUTER_BOUND('',#2266,.T.);
#1495=FACE_OUTER_BOUND('',#2267,.T.);
#1496=FACE_OUTER_BOUND('',#2268,.T.);
#1497=FACE_OUTER_BOUND('',#2269,.T.);
#1498=FACE_OUTER_BOUND('',#2270,.T.);
#1499=FACE_OUTER_BOUND('',#2271,.T.);
#1500=FACE_OUTER_BOUND('',#2272,.T.);
#1501=FACE_OUTER_BOUND('',#2273,.T.);
#1502=FACE_OUTER_BOUND('',#2274,.T.);
#1503=FACE_OUTER_BOUND('',#2275,.T.);
#1504=FACE_OUTER_BOUND('',#2276,.T.);
#1505=FACE_OUTER_BOUND('',#2277,.T.);
#1506=FACE_OUTER_BOUND('',#2278,.T.);
#1507=FACE_OUTER_BOUND('',#2279,.T.);
#1508=FACE_OUTER_BOUND('',#2280,.T.);
#1509=FACE_OUTER_BOUND('',#2281,.T.);
#1510=FACE_OUTER_BOUND('',#2282,.T.);
#1511=FACE_OUTER_BOUND('',#2283,.T.);
#1512=FACE_OUTER_BOUND('',#2284,.T.);
#1513=FACE_OUTER_BOUND('',#2285,.T.);
#1514=FACE_OUTER_BOUND('',#2286,.T.);
#1515=FACE_OUTER_BOUND('',#2287,.T.);
#1516=FACE_OUTER_BOUND('',#2288,.T.);
#1517=FACE_OUTER_BOUND('',#2289,.T.);
#1518=FACE_OUTER_BOUND('',#2290,.T.);
#1519=FACE_OUTER_BOUND('',#2291,.T.);
#1520=FACE_OUTER_BOUND('',#2292,.T.);
#1521=FACE_OUTER_BOUND('',#2293,.T.);
#1522=FACE_OUTER_BOUND('',#2294,.T.);
#1523=FACE_OUTER_BOUND('',#2295,.T.);
#1524=FACE_OUTER_BOUND('',#2296,.T.);
#1525=FACE_OUTER_BOUND('',#2297,.T.);
#1526=FACE_OUTER_BOUND('',#2298,.T.);
#1527=FACE_OUTER_BOUND('',#2299,.T.);
#1528=FACE_OUTER_BOUND('',#2300,.T.);
#1529=FACE_OUTER_BOUND('',#2301,.T.);
#1530=FACE_OUTER_BOUND('',#2302,.T.);
#1531=FACE_OUTER_BOUND('',#2303,.T.);
#1532=FACE_OUTER_BOUND('',#2304,.T.);
#1533=FACE_OUTER_BOUND('',#2305,.T.);
#1534=FACE_OUTER_BOUND('',#2306,.T.);
#1535=FACE_OUTER_BOUND('',#2307,.T.);
#1536=FACE_OUTER_BOUND('',#2308,.T.);
#1537=FACE_OUTER_BOUND('',#2309,.T.);
#1538=FACE_OUTER_BOUND('',#2310,.T.);
#1539=FACE_OUTER_BOUND('',#2311,.T.);
#1540=FACE_OUTER_BOUND('',#2312,.T.);
#1541=FACE_OUTER_BOUND('',#2313,.T.);
#1542=FACE_OUTER_BOUND('',#2314,.T.);
#1543=FACE_OUTER_BOUND('',#2315,.T.);
#1544=FACE_OUTER_BOUND('',#2316,.T.);
#1545=FACE_OUTER_BOUND('',#2317,.T.);
#1546=FACE_OUTER_BOUND('',#2318,.T.);
#1547=FACE_OUTER_BOUND('',#2319,.T.);
#1548=FACE_OUTER_BOUND('',#2320,.T.);
#1549=FACE_OUTER_BOUND('',#2321,.T.);
#1550=FACE_OUTER_BOUND('',#2322,.T.);
#1551=FACE_OUTER_BOUND('',#2323,.T.);
#1552=FACE_OUTER_BOUND('',#2324,.T.);
#1553=FACE_OUTER_BOUND('',#2325,.T.);
#1554=FACE_OUTER_BOUND('',#2326,.T.);
#1555=FACE_OUTER_BOUND('',#2327,.T.);
#1556=FACE_OUTER_BOUND('',#2328,.T.);
#1557=FACE_OUTER_BOUND('',#2329,.T.);
#1558=FACE_OUTER_BOUND('',#2330,.T.);
#1559=FACE_OUTER_BOUND('',#2331,.T.);
#1560=FACE_OUTER_BOUND('',#2332,.T.);
#1561=FACE_OUTER_BOUND('',#2333,.T.);
#1562=FACE_OUTER_BOUND('',#2334,.T.);
#1563=FACE_OUTER_BOUND('',#2335,.T.);
#1564=FACE_OUTER_BOUND('',#2336,.T.);
#1565=FACE_OUTER_BOUND('',#2337,.T.);
#1566=FACE_OUTER_BOUND('',#2338,.T.);
#1567=FACE_OUTER_BOUND('',#2339,.T.);
#1568=FACE_OUTER_BOUND('',#2340,.T.);
#1569=FACE_OUTER_BOUND('',#2341,.T.);
#1570=FACE_OUTER_BOUND('',#2342,.T.);
#1571=FACE_OUTER_BOUND('',#2343,.T.);
#1572=FACE_OUTER_BOUND('',#2344,.T.);
#1573=FACE_OUTER_BOUND('',#2345,.T.);
#1574=FACE_OUTER_BOUND('',#2346,.T.);
#1575=FACE_OUTER_BOUND('',#2347,.T.);
#1576=FACE_OUTER_BOUND('',#2348,.T.);
#1577=FACE_OUTER_BOUND('',#2349,.T.);
#1578=FACE_OUTER_BOUND('',#2350,.T.);
#1579=FACE_OUTER_BOUND('',#2351,.T.);
#1580=FACE_OUTER_BOUND('',#2352,.T.);
#1581=FACE_OUTER_BOUND('',#2353,.T.);
#1582=FACE_OUTER_BOUND('',#2354,.T.);
#1583=FACE_OUTER_BOUND('',#2355,.T.);
#1584=FACE_OUTER_BOUND('',#2356,.T.);
#1585=FACE_OUTER_BOUND('',#2357,.T.);
#1586=FACE_OUTER_BOUND('',#2358,.T.);
#1587=FACE_OUTER_BOUND('',#2359,.T.);
#1588=FACE_OUTER_BOUND('',#2360,.T.);
#1589=FACE_OUTER_BOUND('',#2361,.T.);
#1590=FACE_OUTER_BOUND('',#2362,.T.);
#1591=FACE_OUTER_BOUND('',#2363,.T.);
#1592=FACE_OUTER_BOUND('',#2364,.T.);
#1593=FACE_OUTER_BOUND('',#2365,.T.);
#1594=FACE_OUTER_BOUND('',#2366,.T.);
#1595=FACE_OUTER_BOUND('',#2367,.T.);
#1596=FACE_OUTER_BOUND('',#2368,.T.);
#1597=FACE_OUTER_BOUND('',#2369,.T.);
#1598=FACE_OUTER_BOUND('',#2370,.T.);
#1599=FACE_OUTER_BOUND('',#2371,.T.);
#1600=FACE_OUTER_BOUND('',#2372,.T.);
#1601=FACE_OUTER_BOUND('',#2373,.T.);
#1602=FACE_OUTER_BOUND('',#2374,.T.);
#1603=FACE_OUTER_BOUND('',#2375,.T.);
#1604=FACE_OUTER_BOUND('',#2376,.T.);
#1605=FACE_OUTER_BOUND('',#2377,.T.);
#1606=FACE_OUTER_BOUND('',#2378,.T.);
#1607=FACE_OUTER_BOUND('',#2379,.T.);
#1608=FACE_OUTER_BOUND('',#2380,.T.);
#1609=FACE_OUTER_BOUND('',#2381,.T.);
#1610=FACE_OUTER_BOUND('',#2382,.T.);
#1611=FACE_OUTER_BOUND('',#2383,.T.);
#1612=FACE_OUTER_BOUND('',#2384,.T.);
#1613=FACE_OUTER_BOUND('',#2385,.T.);
#1614=FACE_OUTER_BOUND('',#2386,.T.);
#1615=FACE_OUTER_BOUND('',#2387,.T.);
#1616=FACE_OUTER_BOUND('',#2388,.T.);
#1617=FACE_OUTER_BOUND('',#2389,.T.);
#1618=FACE_OUTER_BOUND('',#2390,.T.);
#1619=FACE_OUTER_BOUND('',#2391,.T.);
#1620=FACE_OUTER_BOUND('',#2392,.T.);
#1621=FACE_OUTER_BOUND('',#2393,.T.);
#1622=FACE_OUTER_BOUND('',#2394,.T.);
#1623=FACE_OUTER_BOUND('',#2395,.T.);
#1624=FACE_OUTER_BOUND('',#2396,.T.);
#1625=FACE_OUTER_BOUND('',#2397,.T.);
#1626=FACE_OUTER_BOUND('',#2398,.T.);
#1627=FACE_OUTER_BOUND('',#2399,.T.);
#1628=FACE_OUTER_BOUND('',#2400,.T.);
#1629=FACE_OUTER_BOUND('',#2401,.T.);
#1630=FACE_OUTER_BOUND('',#2402,.T.);
#1631=FACE_OUTER_BOUND('',#2403,.T.);
#1632=FACE_OUTER_BOUND('',#2404,.T.);
#1633=FACE_OUTER_BOUND('',#2405,.T.);
#1634=FACE_OUTER_BOUND('',#2406,.T.);
#1635=FACE_OUTER_BOUND('',#2407,.T.);
#1636=FACE_OUTER_BOUND('',#2408,.T.);
#1637=FACE_OUTER_BOUND('',#2409,.T.);
#1638=FACE_OUTER_BOUND('',#2410,.T.);
#1639=FACE_OUTER_BOUND('',#2411,.T.);
#1640=FACE_OUTER_BOUND('',#2412,.T.);
#1641=FACE_OUTER_BOUND('',#2413,.T.);
#1642=FACE_OUTER_BOUND('',#2414,.T.);
#1643=FACE_OUTER_BOUND('',#2415,.T.);
#1644=FACE_OUTER_BOUND('',#2416,.T.);
#1645=FACE_OUTER_BOUND('',#2417,.T.);
#1646=FACE_OUTER_BOUND('',#2418,.T.);
#1647=FACE_OUTER_BOUND('',#2419,.T.);
#1648=FACE_OUTER_BOUND('',#2420,.T.);
#1649=FACE_OUTER_BOUND('',#2421,.T.);
#1650=FACE_OUTER_BOUND('',#2422,.T.);
#1651=FACE_OUTER_BOUND('',#2423,.T.);
#1652=FACE_OUTER_BOUND('',#2424,.T.);
#1653=FACE_OUTER_BOUND('',#2425,.T.);
#1654=FACE_OUTER_BOUND('',#2426,.T.);
#1655=FACE_OUTER_BOUND('',#2427,.T.);
#1656=FACE_OUTER_BOUND('',#2428,.T.);
#1657=FACE_OUTER_BOUND('',#2429,.T.);
#1658=FACE_OUTER_BOUND('',#2430,.T.);
#1659=FACE_OUTER_BOUND('',#2431,.T.);
#1660=FACE_OUTER_BOUND('',#2432,.T.);
#1661=FACE_OUTER_BOUND('',#2433,.T.);
#1662=FACE_OUTER_BOUND('',#2434,.T.);
#1663=FACE_OUTER_BOUND('',#2435,.T.);
#1664=FACE_OUTER_BOUND('',#2436,.T.);
#1665=FACE_OUTER_BOUND('',#2437,.T.);
#1666=FACE_OUTER_BOUND('',#2438,.T.);
#1667=FACE_OUTER_BOUND('',#2439,.T.);
#1668=FACE_OUTER_BOUND('',#2440,.T.);
#1669=FACE_OUTER_BOUND('',#2441,.T.);
#1670=FACE_OUTER_BOUND('',#2442,.T.);
#1671=FACE_OUTER_BOUND('',#2443,.T.);
#1672=FACE_OUTER_BOUND('',#2444,.T.);
#1673=FACE_OUTER_BOUND('',#2445,.T.);
#1674=FACE_OUTER_BOUND('',#2446,.T.);
#1675=FACE_OUTER_BOUND('',#2447,.T.);
#1676=FACE_OUTER_BOUND('',#2448,.T.);
#1677=FACE_OUTER_BOUND('',#2449,.T.);
#1678=FACE_OUTER_BOUND('',#2450,.T.);
#1679=FACE_OUTER_BOUND('',#2451,.T.);
#1680=FACE_OUTER_BOUND('',#2452,.T.);
#1681=FACE_OUTER_BOUND('',#2453,.T.);
#1682=FACE_OUTER_BOUND('',#2454,.T.);
#1683=FACE_OUTER_BOUND('',#2455,.T.);
#1684=FACE_OUTER_BOUND('',#2456,.T.);
#1685=FACE_OUTER_BOUND('',#2457,.T.);
#1686=FACE_OUTER_BOUND('',#2458,.T.);
#1687=FACE_OUTER_BOUND('',#2459,.T.);
#1688=FACE_OUTER_BOUND('',#2460,.T.);
#1689=FACE_OUTER_BOUND('',#2461,.T.);
#1690=FACE_OUTER_BOUND('',#2462,.T.);
#1691=FACE_OUTER_BOUND('',#2463,.T.);
#1692=FACE_OUTER_BOUND('',#2464,.T.);
#1693=FACE_OUTER_BOUND('',#2465,.T.);
#1694=FACE_OUTER_BOUND('',#2466,.T.);
#1695=FACE_OUTER_BOUND('',#2467,.T.);
#1696=FACE_OUTER_BOUND('',#2468,.T.);
#1697=FACE_OUTER_BOUND('',#2469,.T.);
#1698=FACE_OUTER_BOUND('',#2470,.T.);
#1699=FACE_OUTER_BOUND('',#2472,.T.);
#1700=FACE_OUTER_BOUND('',#2474,.T.);
#1701=FACE_OUTER_BOUND('',#2476,.T.);
#1702=FACE_OUTER_BOUND('',#2477,.T.);
#1703=FACE_OUTER_BOUND('',#2478,.T.);
#1704=FACE_OUTER_BOUND('',#2479,.T.);
#1705=FACE_OUTER_BOUND('',#2480,.T.);
#1706=FACE_OUTER_BOUND('',#2481,.T.);
#1707=FACE_OUTER_BOUND('',#2482,.T.);
#1708=FACE_OUTER_BOUND('',#2483,.T.);
#1709=FACE_OUTER_BOUND('',#2484,.T.);
#1710=FACE_OUTER_BOUND('',#2485,.T.);
#1711=FACE_OUTER_BOUND('',#2486,.T.);
#1712=FACE_OUTER_BOUND('',#2487,.T.);
#1713=FACE_OUTER_BOUND('',#2488,.T.);
#1714=FACE_OUTER_BOUND('',#2489,.T.);
#1715=FACE_OUTER_BOUND('',#2490,.T.);
#1716=FACE_OUTER_BOUND('',#2491,.T.);
#1717=FACE_OUTER_BOUND('',#2492,.T.);
#1718=FACE_OUTER_BOUND('',#2493,.T.);
#1759=EDGE_LOOP('',(#7051,#7052,#7053,#7054));
#1760=EDGE_LOOP('',(#7055,#7056,#7057,#7058));
#1761=EDGE_LOOP('',(#7059,#7060,#7061,#7062));
#1762=EDGE_LOOP('',(#7063,#7064,#7065,#7066));
#1763=EDGE_LOOP('',(#7067,#7068,#7069,#7070,#7071));
#1764=EDGE_LOOP('',(#7072,#7073,#7074,#7075,#7076));
#1765=EDGE_LOOP('',(#7077,#7078,#7079,#7080));
#1766=EDGE_LOOP('',(#7081,#7082,#7083,#7084,#7085));
#1767=EDGE_LOOP('',(#7086,#7087,#7088,#7089));
#1768=EDGE_LOOP('',(#7090,#7091,#7092,#7093));
#1769=EDGE_LOOP('',(#7094,#7095,#7096,#7097));
#1770=EDGE_LOOP('',(#7098,#7099,#7100,#7101));
#1771=EDGE_LOOP('',(#7102,#7103,#7104,#7105,#7106));
#1772=EDGE_LOOP('',(#7107,#7108,#7109,#7110,#7111));
#1773=EDGE_LOOP('',(#7112,#7113,#7114,#7115,#7116));
#1774=EDGE_LOOP('',(#7117,#7118,#7119,#7120,#7121));
#1775=EDGE_LOOP('',(#7122,#7123,#7124,#7125));
#1776=EDGE_LOOP('',(#7126,#7127,#7128,#7129));
#1777=EDGE_LOOP('',(#7130,#7131,#7132,#7133));
#1778=EDGE_LOOP('',(#7134,#7135,#7136,#7137));
#1779=EDGE_LOOP('',(#7138,#7139,#7140,#7141));
#1780=EDGE_LOOP('',(#7142,#7143,#7144,#7145));
#1781=EDGE_LOOP('',(#7146,#7147,#7148,#7149,#7150));
#1782=EDGE_LOOP('',(#7151,#7152,#7153,#7154));
#1783=EDGE_LOOP('',(#7155,#7156,#7157,#7158));
#1784=EDGE_LOOP('',(#7159,#7160,#7161,#7162));
#1785=EDGE_LOOP('',(#7163,#7164,#7165,#7166,#7167));
#1786=EDGE_LOOP('',(#7168,#7169,#7170,#7171,#7172));
#1787=EDGE_LOOP('',(#7173,#7174,#7175,#7176,#7177));
#1788=EDGE_LOOP('',(#7178,#7179,#7180,#7181,#7182));
#1789=EDGE_LOOP('',(#7183,#7184,#7185,#7186));
#1790=EDGE_LOOP('',(#7187,#7188,#7189,#7190));
#1791=EDGE_LOOP('',(#7191,#7192,#7193,#7194));
#1792=EDGE_LOOP('',(#7195,#7196,#7197,#7198));
#1793=EDGE_LOOP('',(#7199,#7200,#7201,#7202));
#1794=EDGE_LOOP('',(#7203,#7204,#7205,#7206));
#1795=EDGE_LOOP('',(#7207,#7208,#7209,#7210));
#1796=EDGE_LOOP('',(#7211,#7212,#7213,#7214));
#1797=EDGE_LOOP('',(#7215,#7216,#7217,#7218));
#1798=EDGE_LOOP('',(#7219,#7220,#7221,#7222));
#1799=EDGE_LOOP('',(#7223,#7224,#7225,#7226));
#1800=EDGE_LOOP('',(#7227,#7228,#7229,#7230));
#1801=EDGE_LOOP('',(#7231,#7232,#7233,#7234));
#1802=EDGE_LOOP('',(#7235,#7236,#7237,#7238));
#1803=EDGE_LOOP('',(#7239,#7240,#7241,#7242));
#1804=EDGE_LOOP('',(#7243,#7244,#7245,#7246));
#1805=EDGE_LOOP('',(#7247,#7248,#7249,#7250));
#1806=EDGE_LOOP('',(#7251,#7252,#7253,#7254));
#1807=EDGE_LOOP('',(#7255,#7256,#7257,#7258));
#1808=EDGE_LOOP('',(#7259,#7260,#7261,#7262,#7263,#7264));
#1809=EDGE_LOOP('',(#7265,#7266,#7267,#7268,#7269,#7270));
#1810=EDGE_LOOP('',(#7271,#7272,#7273,#7274));
#1811=EDGE_LOOP('',(#7275,#7276,#7277,#7278));
#1812=EDGE_LOOP('',(#7279,#7280,#7281,#7282));
#1813=EDGE_LOOP('',(#7283,#7284,#7285,#7286));
#1814=EDGE_LOOP('',(#7287,#7288,#7289,#7290,#7291));
#1815=EDGE_LOOP('',(#7292,#7293,#7294,#7295,#7296,#7297,#7298));
#1816=EDGE_LOOP('',(#7299,#7300,#7301,#7302));
#1817=EDGE_LOOP('',(#7303,#7304,#7305,#7306));
#1818=EDGE_LOOP('',(#7307,#7308,#7309,#7310));
#1819=EDGE_LOOP('',(#7311,#7312,#7313,#7314,#7315,#7316));
#1820=EDGE_LOOP('',(#7317,#7318,#7319,#7320,#7321,#7322));
#1821=EDGE_LOOP('',(#7323,#7324,#7325,#7326,#7327,#7328,#7329));
#1822=EDGE_LOOP('',(#7330,#7331,#7332,#7333));
#1823=EDGE_LOOP('',(#7334,#7335,#7336,#7337));
#1824=EDGE_LOOP('',(#7338,#7339,#7340,#7341));
#1825=EDGE_LOOP('',(#7342,#7343,#7344,#7345,#7346,#7347,#7348,#7349,#7350,
#7351,#7352,#7353,#7354,#7355,#7356,#7357,#7358,#7359,#7360,#7361,#7362,
#7363,#7364,#7365,#7366,#7367,#7368,#7369,#7370,#7371,#7372,#7373,#7374,
#7375,#7376,#7377,#7378,#7379,#7380,#7381,#7382,#7383,#7384,#7385,#7386,
#7387,#7388,#7389,#7390,#7391,#7392,#7393,#7394,#7395,#7396,#7397,#7398,
#7399,#7400,#7401,#7402,#7403,#7404,#7405,#7406,#7407,#7408,#7409,#7410,
#7411,#7412,#7413,#7414,#7415));
#1826=EDGE_LOOP('',(#7416,#7417,#7418,#7419,#7420,#7421));
#1827=EDGE_LOOP('',(#7422,#7423,#7424,#7425,#7426));
#1828=EDGE_LOOP('',(#7427,#7428,#7429,#7430,#7431,#7432,#7433));
#1829=EDGE_LOOP('',(#7434,#7435,#7436,#7437));
#1830=EDGE_LOOP('',(#7438,#7439,#7440,#7441));
#1831=EDGE_LOOP('',(#7442,#7443,#7444,#7445,#7446,#7447,#7448,#7449,#7450,
#7451,#7452,#7453,#7454,#7455,#7456,#7457,#7458,#7459,#7460,#7461,#7462,
#7463));
#1832=EDGE_LOOP('',(#7464));
#1833=EDGE_LOOP('',(#7465,#7466,#7467,#7468,#7469,#7470,#7471,#7472));
#1834=EDGE_LOOP('',(#7473));
#1835=EDGE_LOOP('',(#7474));
#1836=EDGE_LOOP('',(#7475,#7476,#7477,#7478,#7479,#7480,#7481,#7482));
#1837=EDGE_LOOP('',(#7483,#7484,#7485,#7486,#7487,#7488,#7489,#7490));
#1838=EDGE_LOOP('',(#7491));
#1839=EDGE_LOOP('',(#7492,#7493,#7494,#7495,#7496,#7497,#7498,#7499,#7500,
#7501,#7502,#7503,#7504,#7505,#7506,#7507));
#1840=EDGE_LOOP('',(#7508,#7509,#7510,#7511));
#1841=EDGE_LOOP('',(#7512,#7513,#7514,#7515));
#1842=EDGE_LOOP('',(#7516,#7517,#7518,#7519,#7520,#7521,#7522,#7523,#7524,
#7525,#7526,#7527,#7528,#7529,#7530,#7531,#7532,#7533));
#1843=EDGE_LOOP('',(#7534));
#1844=EDGE_LOOP('',(#7535,#7536,#7537,#7538,#7539,#7540,#7541,#7542,#7543,
#7544,#7545,#7546,#7547,#7548,#7549,#7550));
#1845=EDGE_LOOP('',(#7551));
#1846=EDGE_LOOP('',(#7552,#7553,#7554,#7555));
#1847=EDGE_LOOP('',(#7556,#7557,#7558,#7559));
#1848=EDGE_LOOP('',(#7560,#7561,#7562,#7563));
#1849=EDGE_LOOP('',(#7564,#7565,#7566,#7567));
#1850=EDGE_LOOP('',(#7568,#7569,#7570,#7571));
#1851=EDGE_LOOP('',(#7572,#7573,#7574,#7575));
#1852=EDGE_LOOP('',(#7576,#7577,#7578,#7579));
#1853=EDGE_LOOP('',(#7580,#7581,#7582,#7583));
#1854=EDGE_LOOP('',(#7584,#7585,#7586,#7587));
#1855=EDGE_LOOP('',(#7588,#7589,#7590,#7591));
#1856=EDGE_LOOP('',(#7592,#7593,#7594,#7595,#7596));
#1857=EDGE_LOOP('',(#7597));
#1858=EDGE_LOOP('',(#7598,#7599,#7600,#7601,#7602));
#1859=EDGE_LOOP('',(#7603,#7604,#7605,#7606,#7607));
#1860=EDGE_LOOP('',(#7608,#7609,#7610,#7611,#7612));
#1861=EDGE_LOOP('',(#7613,#7614,#7615,#7616,#7617));
#1862=EDGE_LOOP('',(#7618,#7619,#7620,#7621,#7622,#7623,#7624));
#1863=EDGE_LOOP('',(#7625,#7626,#7627,#7628,#7629,#7630,#7631,#7632,#7633,
#7634,#7635,#7636,#7637,#7638,#7639,#7640,#7641,#7642,#7643,#7644,#7645,
#7646,#7647,#7648,#7649,#7650,#7651,#7652));
#1864=EDGE_LOOP('',(#7653,#7654,#7655,#7656,#7657,#7658,#7659));
#1865=EDGE_LOOP('',(#7660,#7661,#7662,#7663,#7664,#7665,#7666));
#1866=EDGE_LOOP('',(#7667,#7668,#7669,#7670,#7671,#7672,#7673));
#1867=EDGE_LOOP('',(#7674,#7675,#7676,#7677,#7678,#7679));
#1868=EDGE_LOOP('',(#7680,#7681,#7682,#7683));
#1869=EDGE_LOOP('',(#7684,#7685,#7686,#7687));
#1870=EDGE_LOOP('',(#7688,#7689,#7690,#7691,#7692,#7693));
#1871=EDGE_LOOP('',(#7694,#7695,#7696,#7697,#7698,#7699));
#1872=EDGE_LOOP('',(#7700,#7701,#7702,#7703,#7704,#7705,#7706,#7707));
#1873=EDGE_LOOP('',(#7708));
#1874=EDGE_LOOP('',(#7709,#7710,#7711,#7712,#7713,#7714,#7715,#7716));
#1875=EDGE_LOOP('',(#7717));
#1876=EDGE_LOOP('',(#7718,#7719,#7720,#7721,#7722,#7723,#7724,#7725));
#1877=EDGE_LOOP('',(#7726,#7727,#7728,#7729,#7730,#7731,#7732,#7733));
#1878=EDGE_LOOP('',(#7734,#7735,#7736,#7737));
#1879=EDGE_LOOP('',(#7738,#7739,#7740,#7741,#7742,#7743,#7744,#7745));
#1880=EDGE_LOOP('',(#7746,#7747,#7748,#7749,#7750,#7751,#7752,#7753));
#1881=EDGE_LOOP('',(#7754,#7755,#7756,#7757,#7758,#7759,#7760,#7761,#7762,
#7763,#7764,#7765,#7766,#7767,#7768,#7769,#7770,#7771,#7772,#7773,#7774,
#7775,#7776,#7777,#7778,#7779,#7780,#7781,#7782,#7783,#7784));
#1882=EDGE_LOOP('',(#7785));
#1883=EDGE_LOOP('',(#7786));
#1884=EDGE_LOOP('',(#7787,#7788,#7789,#7790,#7791,#7792,#7793,#7794,#7795,
#7796,#7797));
#1885=EDGE_LOOP('',(#7798));
#1886=EDGE_LOOP('',(#7799));
#1887=EDGE_LOOP('',(#7800,#7801,#7802,#7803,#7804,#7805,#7806,#7807,#7808,
#7809,#7810));
#1888=EDGE_LOOP('',(#7811,#7812,#7813,#7814,#7815,#7816,#7817,#7818,#7819,
#7820,#7821));
#1889=EDGE_LOOP('',(#7822));
#1890=EDGE_LOOP('',(#7823,#7824,#7825,#7826));
#1891=EDGE_LOOP('',(#7827,#7828,#7829,#7830));
#1892=EDGE_LOOP('',(#7831,#7832,#7833,#7834,#7835));
#1893=EDGE_LOOP('',(#7836,#7837,#7838,#7839,#7840));
#1894=EDGE_LOOP('',(#7841,#7842,#7843,#7844,#7845,#7846));
#1895=EDGE_LOOP('',(#7847,#7848,#7849,#7850,#7851,#7852));
#1896=EDGE_LOOP('',(#7853,#7854,#7855,#7856));
#1897=EDGE_LOOP('',(#7857,#7858,#7859,#7860));
#1898=EDGE_LOOP('',(#7861,#7862,#7863));
#1899=EDGE_LOOP('',(#7864,#7865,#7866,#7867));
#1900=EDGE_LOOP('',(#7868,#7869,#7870));
#1901=EDGE_LOOP('',(#7871,#7872,#7873,#7874));
#1902=EDGE_LOOP('',(#7875,#7876,#7877,#7878));
#1903=EDGE_LOOP('',(#7879,#7880,#7881,#7882));
#1904=EDGE_LOOP('',(#7883,#7884,#7885,#7886,#7887,#7888,#7889,#7890));
#1905=EDGE_LOOP('',(#7891,#7892,#7893,#7894));
#1906=EDGE_LOOP('',(#7895,#7896,#7897,#7898));
#1907=EDGE_LOOP('',(#7899,#7900,#7901,#7902));
#1908=EDGE_LOOP('',(#7903,#7904,#7905,#7906,#7907,#7908,#7909));
#1909=EDGE_LOOP('',(#7910,#7911,#7912,#7913,#7914,#7915,#7916));
#1910=EDGE_LOOP('',(#7917,#7918,#7919,#7920,#7921,#7922,#7923));
#1911=EDGE_LOOP('',(#7924,#7925,#7926,#7927,#7928,#7929,#7930));
#1912=EDGE_LOOP('',(#7931,#7932,#7933,#7934));
#1913=EDGE_LOOP('',(#7935,#7936,#7937,#7938,#7939,#7940));
#1914=EDGE_LOOP('',(#7941,#7942,#7943,#7944,#7945,#7946,#7947,#7948));
#1915=EDGE_LOOP('',(#7949));
#1916=EDGE_LOOP('',(#7950,#7951,#7952,#7953,#7954,#7955,#7956,#7957));
#1917=EDGE_LOOP('',(#7958));
#1918=EDGE_LOOP('',(#7959,#7960,#7961,#7962,#7963,#7964,#7965,#7966));
#1919=EDGE_LOOP('',(#7967,#7968,#7969,#7970));
#1920=EDGE_LOOP('',(#7971,#7972,#7973,#7974,#7975,#7976,#7977,#7978));
#1921=EDGE_LOOP('',(#7979,#7980,#7981,#7982));
#1922=EDGE_LOOP('',(#7983,#7984,#7985,#7986));
#1923=EDGE_LOOP('',(#7987,#7988,#7989,#7990,#7991));
#1924=EDGE_LOOP('',(#7992,#7993,#7994,#7995,#7996,#7997));
#1925=EDGE_LOOP('',(#7998,#7999,#8000,#8001,#8002,#8003));
#1926=EDGE_LOOP('',(#8004,#8005,#8006,#8007));
#1927=EDGE_LOOP('',(#8008,#8009,#8010,#8011));
#1928=EDGE_LOOP('',(#8012,#8013,#8014));
#1929=EDGE_LOOP('',(#8015,#8016,#8017,#8018));
#1930=EDGE_LOOP('',(#8019,#8020,#8021));
#1931=EDGE_LOOP('',(#8022,#8023,#8024,#8025));
#1932=EDGE_LOOP('',(#8026,#8027,#8028,#8029));
#1933=EDGE_LOOP('',(#8030,#8031,#8032,#8033));
#1934=EDGE_LOOP('',(#8034,#8035,#8036,#8037,#8038,#8039,#8040,#8041));
#1935=EDGE_LOOP('',(#8042,#8043,#8044,#8045));
#1936=EDGE_LOOP('',(#8046,#8047,#8048,#8049));
#1937=EDGE_LOOP('',(#8050,#8051,#8052,#8053));
#1938=EDGE_LOOP('',(#8054,#8055,#8056,#8057,#8058,#8059,#8060));
#1939=EDGE_LOOP('',(#8061,#8062,#8063,#8064,#8065,#8066,#8067));
#1940=EDGE_LOOP('',(#8068,#8069,#8070,#8071,#8072,#8073,#8074));
#1941=EDGE_LOOP('',(#8075,#8076,#8077,#8078,#8079,#8080,#8081));
#1942=EDGE_LOOP('',(#8082,#8083,#8084,#8085));
#1943=EDGE_LOOP('',(#8086,#8087,#8088,#8089,#8090,#8091));
#1944=EDGE_LOOP('',(#8092,#8093,#8094,#8095,#8096,#8097,#8098,#8099));
#1945=EDGE_LOOP('',(#8100,#8101,#8102,#8103));
#1946=EDGE_LOOP('',(#8104,#8105,#8106,#8107,#8108,#8109,#8110,#8111));
#1947=EDGE_LOOP('',(#8112,#8113,#8114,#8115));
#1948=EDGE_LOOP('',(#8116,#8117,#8118,#8119));
#1949=EDGE_LOOP('',(#8120,#8121,#8122,#8123,#8124));
#1950=EDGE_LOOP('',(#8125,#8126,#8127,#8128,#8129,#8130));
#1951=EDGE_LOOP('',(#8131,#8132,#8133,#8134,#8135,#8136));
#1952=EDGE_LOOP('',(#8137,#8138,#8139,#8140));
#1953=EDGE_LOOP('',(#8141,#8142,#8143,#8144));
#1954=EDGE_LOOP('',(#8145,#8146,#8147));
#1955=EDGE_LOOP('',(#8148,#8149,#8150,#8151));
#1956=EDGE_LOOP('',(#8152,#8153,#8154));
#1957=EDGE_LOOP('',(#8155,#8156,#8157,#8158));
#1958=EDGE_LOOP('',(#8159,#8160,#8161,#8162));
#1959=EDGE_LOOP('',(#8163,#8164,#8165,#8166));
#1960=EDGE_LOOP('',(#8167,#8168,#8169,#8170,#8171,#8172,#8173,#8174,#8175,
#8176,#8177,#8178));
#1961=EDGE_LOOP('',(#8179,#8180,#8181,#8182));
#1962=EDGE_LOOP('',(#8183,#8184,#8185,#8186));
#1963=EDGE_LOOP('',(#8187,#8188,#8189,#8190));
#1964=EDGE_LOOP('',(#8191,#8192,#8193,#8194,#8195,#8196,#8197));
#1965=EDGE_LOOP('',(#8198,#8199,#8200,#8201,#8202,#8203,#8204));
#1966=EDGE_LOOP('',(#8205,#8206,#8207,#8208,#8209,#8210,#8211));
#1967=EDGE_LOOP('',(#8212,#8213,#8214,#8215,#8216,#8217,#8218));
#1968=EDGE_LOOP('',(#8219,#8220,#8221,#8222,#8223,#8224,#8225,#8226));
#1969=EDGE_LOOP('',(#8227));
#1970=EDGE_LOOP('',(#8228,#8229,#8230,#8231,#8232,#8233,#8234,#8235));
#1971=EDGE_LOOP('',(#8236));
#1972=EDGE_LOOP('',(#8237,#8238,#8239,#8240));
#1973=EDGE_LOOP('',(#8241,#8242,#8243,#8244));
#1974=EDGE_LOOP('',(#8245,#8246,#8247,#8248));
#1975=EDGE_LOOP('',(#8249,#8250,#8251,#8252,#8253,#8254));
#1976=EDGE_LOOP('',(#8255,#8256,#8257,#8258,#8259,#8260));
#1977=EDGE_LOOP('',(#8261,#8262,#8263,#8264));
#1978=EDGE_LOOP('',(#8265,#8266,#8267,#8268));
#1979=EDGE_LOOP('',(#8269,#8270,#8271));
#1980=EDGE_LOOP('',(#8272,#8273,#8274,#8275));
#1981=EDGE_LOOP('',(#8276,#8277,#8278));
#1982=EDGE_LOOP('',(#8279,#8280,#8281,#8282));
#1983=EDGE_LOOP('',(#8283,#8284,#8285,#8286));
#1984=EDGE_LOOP('',(#8287,#8288,#8289,#8290));
#1985=EDGE_LOOP('',(#8291,#8292,#8293,#8294,#8295,#8296,#8297,#8298));
#1986=EDGE_LOOP('',(#8299,#8300,#8301,#8302));
#1987=EDGE_LOOP('',(#8303,#8304,#8305,#8306));
#1988=EDGE_LOOP('',(#8307,#8308,#8309,#8310));
#1989=EDGE_LOOP('',(#8311,#8312,#8313,#8314));
#1990=EDGE_LOOP('',(#8315,#8316,#8317,#8318));
#1991=EDGE_LOOP('',(#8319,#8320,#8321,#8322));
#1992=EDGE_LOOP('',(#8323,#8324,#8325,#8326));
#1993=EDGE_LOOP('',(#8327,#8328,#8329,#8330));
#1994=EDGE_LOOP('',(#8331,#8332,#8333,#8334));
#1995=EDGE_LOOP('',(#8335,#8336,#8337,#8338));
#1996=EDGE_LOOP('',(#8339,#8340,#8341,#8342));
#1997=EDGE_LOOP('',(#8343,#8344,#8345,#8346));
#1998=EDGE_LOOP('',(#8347,#8348,#8349,#8350));
#1999=EDGE_LOOP('',(#8351,#8352,#8353,#8354));
#2000=EDGE_LOOP('',(#8355,#8356,#8357,#8358));
#2001=EDGE_LOOP('',(#8359,#8360,#8361,#8362));
#2002=EDGE_LOOP('',(#8363,#8364,#8365,#8366));
#2003=EDGE_LOOP('',(#8367,#8368,#8369,#8370));
#2004=EDGE_LOOP('',(#8371,#8372,#8373,#8374));
#2005=EDGE_LOOP('',(#8375,#8376,#8377,#8378));
#2006=EDGE_LOOP('',(#8379,#8380,#8381,#8382));
#2007=EDGE_LOOP('',(#8383,#8384,#8385,#8386));
#2008=EDGE_LOOP('',(#8387,#8388,#8389,#8390));
#2009=EDGE_LOOP('',(#8391,#8392,#8393,#8394));
#2010=EDGE_LOOP('',(#8395,#8396,#8397,#8398));
#2011=EDGE_LOOP('',(#8399,#8400,#8401,#8402));
#2012=EDGE_LOOP('',(#8403,#8404,#8405,#8406));
#2013=EDGE_LOOP('',(#8407,#8408,#8409,#8410));
#2014=EDGE_LOOP('',(#8411,#8412,#8413,#8414));
#2015=EDGE_LOOP('',(#8415,#8416,#8417,#8418));
#2016=EDGE_LOOP('',(#8419,#8420,#8421,#8422));
#2017=EDGE_LOOP('',(#8423,#8424,#8425,#8426));
#2018=EDGE_LOOP('',(#8427,#8428,#8429,#8430));
#2019=EDGE_LOOP('',(#8431,#8432,#8433,#8434));
#2020=EDGE_LOOP('',(#8435,#8436,#8437,#8438));
#2021=EDGE_LOOP('',(#8439,#8440,#8441,#8442));
#2022=EDGE_LOOP('',(#8443,#8444,#8445,#8446));
#2023=EDGE_LOOP('',(#8447,#8448,#8449,#8450));
#2024=EDGE_LOOP('',(#8451,#8452,#8453,#8454));
#2025=EDGE_LOOP('',(#8455,#8456,#8457,#8458));
#2026=EDGE_LOOP('',(#8459,#8460,#8461,#8462));
#2027=EDGE_LOOP('',(#8463,#8464,#8465,#8466));
#2028=EDGE_LOOP('',(#8467,#8468,#8469,#8470));
#2029=EDGE_LOOP('',(#8471,#8472,#8473,#8474,#8475));
#2030=EDGE_LOOP('',(#8476,#8477,#8478,#8479,#8480));
#2031=EDGE_LOOP('',(#8481,#8482,#8483,#8484,#8485));
#2032=EDGE_LOOP('',(#8486,#8487,#8488,#8489));
#2033=EDGE_LOOP('',(#8490,#8491,#8492,#8493));
#2034=EDGE_LOOP('',(#8494,#8495,#8496));
#2035=EDGE_LOOP('',(#8497,#8498,#8499,#8500));
#2036=EDGE_LOOP('',(#8501,#8502,#8503));
#2037=EDGE_LOOP('',(#8504,#8505,#8506,#8507));
#2038=EDGE_LOOP('',(#8508,#8509,#8510,#8511));
#2039=EDGE_LOOP('',(#8512,#8513,#8514,#8515));
#2040=EDGE_LOOP('',(#8516,#8517,#8518,#8519));
#2041=EDGE_LOOP('',(#8520,#8521,#8522,#8523));
#2042=EDGE_LOOP('',(#8524,#8525,#8526,#8527));
#2043=EDGE_LOOP('',(#8528,#8529,#8530,#8531));
#2044=EDGE_LOOP('',(#8532,#8533,#8534,#8535));
#2045=EDGE_LOOP('',(#8536,#8537,#8538,#8539));
#2046=EDGE_LOOP('',(#8540,#8541,#8542,#8543));
#2047=EDGE_LOOP('',(#8544,#8545,#8546,#8547));
#2048=EDGE_LOOP('',(#8548,#8549,#8550,#8551,#8552));
#2049=EDGE_LOOP('',(#8553,#8554,#8555,#8556));
#2050=EDGE_LOOP('',(#8557,#8558,#8559,#8560));
#2051=EDGE_LOOP('',(#8561,#8562,#8563,#8564));
#2052=EDGE_LOOP('',(#8565,#8566,#8567,#8568));
#2053=EDGE_LOOP('',(#8569,#8570,#8571,#8572));
#2054=EDGE_LOOP('',(#8573,#8574,#8575));
#2055=EDGE_LOOP('',(#8576,#8577,#8578));
#2056=EDGE_LOOP('',(#8579,#8580,#8581,#8582));
#2057=EDGE_LOOP('',(#8583,#8584,#8585,#8586));
#2058=EDGE_LOOP('',(#8587,#8588,#8589,#8590,#8591));
#2059=EDGE_LOOP('',(#8592,#8593,#8594,#8595,#8596));
#2060=EDGE_LOOP('',(#8597,#8598,#8599,#8600,#8601));
#2061=EDGE_LOOP('',(#8602,#8603,#8604,#8605));
#2062=EDGE_LOOP('',(#8606,#8607,#8608,#8609));
#2063=EDGE_LOOP('',(#8610,#8611,#8612,#8613));
#2064=EDGE_LOOP('',(#8614,#8615,#8616,#8617));
#2065=EDGE_LOOP('',(#8618,#8619,#8620,#8621));
#2066=EDGE_LOOP('',(#8622,#8623,#8624,#8625));
#2067=EDGE_LOOP('',(#8626,#8627,#8628,#8629));
#2068=EDGE_LOOP('',(#8630,#8631,#8632,#8633));
#2069=EDGE_LOOP('',(#8634,#8635,#8636,#8637));
#2070=EDGE_LOOP('',(#8638,#8639,#8640,#8641));
#2071=EDGE_LOOP('',(#8642,#8643,#8644,#8645));
#2072=EDGE_LOOP('',(#8646,#8647,#8648,#8649));
#2073=EDGE_LOOP('',(#8650,#8651,#8652,#8653));
#2074=EDGE_LOOP('',(#8654,#8655,#8656,#8657));
#2075=EDGE_LOOP('',(#8658,#8659,#8660,#8661));
#2076=EDGE_LOOP('',(#8662,#8663,#8664,#8665));
#2077=EDGE_LOOP('',(#8666,#8667,#8668,#8669));
#2078=EDGE_LOOP('',(#8670,#8671,#8672,#8673));
#2079=EDGE_LOOP('',(#8674,#8675,#8676,#8677));
#2080=EDGE_LOOP('',(#8678,#8679,#8680,#8681));
#2081=EDGE_LOOP('',(#8682,#8683,#8684,#8685));
#2082=EDGE_LOOP('',(#8686,#8687,#8688,#8689));
#2083=EDGE_LOOP('',(#8690,#8691,#8692,#8693,#8694));
#2084=EDGE_LOOP('',(#8695,#8696,#8697));
#2085=EDGE_LOOP('',(#8698,#8699,#8700));
#2086=EDGE_LOOP('',(#8701,#8702,#8703,#8704));
#2087=EDGE_LOOP('',(#8705,#8706,#8707,#8708));
#2088=EDGE_LOOP('',(#8709,#8710,#8711,#8712));
#2089=EDGE_LOOP('',(#8713,#8714,#8715,#8716));
#2090=EDGE_LOOP('',(#8717,#8718,#8719,#8720));
#2091=EDGE_LOOP('',(#8721,#8722,#8723,#8724));
#2092=EDGE_LOOP('',(#8725,#8726,#8727,#8728));
#2093=EDGE_LOOP('',(#8729,#8730,#8731,#8732));
#2094=EDGE_LOOP('',(#8733,#8734,#8735,#8736));
#2095=EDGE_LOOP('',(#8737,#8738,#8739,#8740));
#2096=EDGE_LOOP('',(#8741,#8742,#8743,#8744));
#2097=EDGE_LOOP('',(#8745,#8746,#8747,#8748));
#2098=EDGE_LOOP('',(#8749,#8750,#8751,#8752));
#2099=EDGE_LOOP('',(#8753,#8754,#8755,#8756));
#2100=EDGE_LOOP('',(#8757,#8758,#8759,#8760));
#2101=EDGE_LOOP('',(#8761,#8762,#8763,#8764));
#2102=EDGE_LOOP('',(#8765,#8766,#8767,#8768));
#2103=EDGE_LOOP('',(#8769,#8770,#8771,#8772));
#2104=EDGE_LOOP('',(#8773,#8774,#8775,#8776));
#2105=EDGE_LOOP('',(#8777,#8778,#8779,#8780));
#2106=EDGE_LOOP('',(#8781,#8782,#8783,#8784));
#2107=EDGE_LOOP('',(#8785,#8786,#8787,#8788,#8789));
#2108=EDGE_LOOP('',(#8790,#8791,#8792,#8793,#8794));
#2109=EDGE_LOOP('',(#8795,#8796,#8797,#8798,#8799));
#2110=EDGE_LOOP('',(#8800,#8801,#8802,#8803));
#2111=EDGE_LOOP('',(#8804,#8805,#8806,#8807));
#2112=EDGE_LOOP('',(#8808,#8809,#8810));
#2113=EDGE_LOOP('',(#8811,#8812,#8813));
#2114=EDGE_LOOP('',(#8814,#8815,#8816,#8817));
#2115=EDGE_LOOP('',(#8818,#8819,#8820,#8821));
#2116=EDGE_LOOP('',(#8822,#8823,#8824,#8825));
#2117=EDGE_LOOP('',(#8826,#8827,#8828,#8829));
#2118=EDGE_LOOP('',(#8830,#8831,#8832));
#2119=EDGE_LOOP('',(#8833,#8834,#8835));
#2120=EDGE_LOOP('',(#8836,#8837,#8838,#8839));
#2121=EDGE_LOOP('',(#8840,#8841,#8842,#8843));
#2122=EDGE_LOOP('',(#8844,#8845,#8846,#8847));
#2123=EDGE_LOOP('',(#8848,#8849,#8850,#8851));
#2124=EDGE_LOOP('',(#8852,#8853,#8854,#8855));
#2125=EDGE_LOOP('',(#8856,#8857,#8858,#8859));
#2126=EDGE_LOOP('',(#8860,#8861,#8862,#8863));
#2127=EDGE_LOOP('',(#8864,#8865,#8866,#8867));
#2128=EDGE_LOOP('',(#8868,#8869,#8870,#8871));
#2129=EDGE_LOOP('',(#8872,#8873,#8874,#8875));
#2130=EDGE_LOOP('',(#8876,#8877,#8878,#8879));
#2131=EDGE_LOOP('',(#8880,#8881,#8882,#8883));
#2132=EDGE_LOOP('',(#8884,#8885,#8886,#8887,#8888));
#2133=EDGE_LOOP('',(#8889,#8890,#8891,#8892));
#2134=EDGE_LOOP('',(#8893,#8894,#8895,#8896));
#2135=EDGE_LOOP('',(#8897,#8898,#8899,#8900));
#2136=EDGE_LOOP('',(#8901,#8902,#8903,#8904));
#2137=EDGE_LOOP('',(#8905,#8906,#8907,#8908));
#2138=EDGE_LOOP('',(#8909,#8910,#8911,#8912));
#2139=EDGE_LOOP('',(#8913,#8914,#8915,#8916));
#2140=EDGE_LOOP('',(#8917,#8918,#8919,#8920));
#2141=EDGE_LOOP('',(#8921,#8922,#8923,#8924));
#2142=EDGE_LOOP('',(#8925,#8926,#8927,#8928));
#2143=EDGE_LOOP('',(#8929,#8930,#8931,#8932));
#2144=EDGE_LOOP('',(#8933,#8934,#8935,#8936));
#2145=EDGE_LOOP('',(#8937,#8938,#8939,#8940));
#2146=EDGE_LOOP('',(#8941,#8942,#8943,#8944));
#2147=EDGE_LOOP('',(#8945,#8946,#8947,#8948));
#2148=EDGE_LOOP('',(#8949,#8950,#8951,#8952));
#2149=EDGE_LOOP('',(#8953,#8954,#8955,#8956));
#2150=EDGE_LOOP('',(#8957,#8958,#8959,#8960));
#2151=EDGE_LOOP('',(#8961,#8962,#8963,#8964));
#2152=EDGE_LOOP('',(#8965,#8966,#8967,#8968));
#2153=EDGE_LOOP('',(#8969,#8970,#8971,#8972));
#2154=EDGE_LOOP('',(#8973,#8974,#8975,#8976));
#2155=EDGE_LOOP('',(#8977,#8978,#8979));
#2156=EDGE_LOOP('',(#8980,#8981,#8982));
#2157=EDGE_LOOP('',(#8983,#8984,#8985,#8986));
#2158=EDGE_LOOP('',(#8987,#8988,#8989,#8990));
#2159=EDGE_LOOP('',(#8991,#8992,#8993,#8994));
#2160=EDGE_LOOP('',(#8995,#8996,#8997,#8998));
#2161=EDGE_LOOP('',(#8999,#9000,#9001,#9002));
#2162=EDGE_LOOP('',(#9003,#9004,#9005,#9006));
#2163=EDGE_LOOP('',(#9007,#9008,#9009,#9010));
#2164=EDGE_LOOP('',(#9011,#9012,#9013,#9014));
#2165=EDGE_LOOP('',(#9015,#9016,#9017,#9018));
#2166=EDGE_LOOP('',(#9019,#9020,#9021,#9022));
#2167=EDGE_LOOP('',(#9023,#9024,#9025));
#2168=EDGE_LOOP('',(#9026,#9027,#9028,#9029));
#2169=EDGE_LOOP('',(#9030,#9031,#9032,#9033));
#2170=EDGE_LOOP('',(#9034,#9035,#9036,#9037));
#2171=EDGE_LOOP('',(#9038,#9039,#9040,#9041));
#2172=EDGE_LOOP('',(#9042,#9043,#9044,#9045));
#2173=EDGE_LOOP('',(#9046,#9047,#9048,#9049));
#2174=EDGE_LOOP('',(#9050,#9051,#9052,#9053));
#2175=EDGE_LOOP('',(#9054,#9055,#9056,#9057));
#2176=EDGE_LOOP('',(#9058,#9059,#9060));
#2177=EDGE_LOOP('',(#9061,#9062,#9063,#9064));
#2178=EDGE_LOOP('',(#9065,#9066,#9067,#9068));
#2179=EDGE_LOOP('',(#9069,#9070,#9071,#9072));
#2180=EDGE_LOOP('',(#9073,#9074,#9075,#9076));
#2181=EDGE_LOOP('',(#9077,#9078,#9079,#9080));
#2182=EDGE_LOOP('',(#9081,#9082,#9083,#9084));
#2183=EDGE_LOOP('',(#9085,#9086,#9087,#9088));
#2184=EDGE_LOOP('',(#9089,#9090,#9091,#9092));
#2185=EDGE_LOOP('',(#9093,#9094,#9095,#9096));
#2186=EDGE_LOOP('',(#9097,#9098,#9099,#9100));
#2187=EDGE_LOOP('',(#9101,#9102,#9103,#9104));
#2188=EDGE_LOOP('',(#9105,#9106,#9107,#9108));
#2189=EDGE_LOOP('',(#9109,#9110,#9111,#9112));
#2190=EDGE_LOOP('',(#9113,#9114,#9115,#9116));
#2191=EDGE_LOOP('',(#9117,#9118,#9119,#9120));
#2192=EDGE_LOOP('',(#9121,#9122,#9123,#9124,#9125));
#2193=EDGE_LOOP('',(#9126,#9127,#9128,#9129,#9130));
#2194=EDGE_LOOP('',(#9131,#9132,#9133,#9134,#9135));
#2195=EDGE_LOOP('',(#9136,#9137,#9138,#9139));
#2196=EDGE_LOOP('',(#9140,#9141,#9142,#9143));
#2197=EDGE_LOOP('',(#9144,#9145,#9146,#9147));
#2198=EDGE_LOOP('',(#9148,#9149,#9150,#9151));
#2199=EDGE_LOOP('',(#9152,#9153,#9154,#9155));
#2200=EDGE_LOOP('',(#9156,#9157,#9158,#9159));
#2201=EDGE_LOOP('',(#9160,#9161,#9162,#9163));
#2202=EDGE_LOOP('',(#9164,#9165,#9166,#9167,#9168));
#2203=EDGE_LOOP('',(#9169,#9170,#9171,#9172));
#2204=EDGE_LOOP('',(#9173,#9174,#9175,#9176));
#2205=EDGE_LOOP('',(#9177,#9178,#9179,#9180));
#2206=EDGE_LOOP('',(#9181,#9182,#9183,#9184));
#2207=EDGE_LOOP('',(#9185,#9186,#9187,#9188));
#2208=EDGE_LOOP('',(#9189,#9190,#9191));
#2209=EDGE_LOOP('',(#9192,#9193,#9194,#9195));
#2210=EDGE_LOOP('',(#9196,#9197,#9198,#9199));
#2211=EDGE_LOOP('',(#9200,#9201,#9202,#9203));
#2212=EDGE_LOOP('',(#9204,#9205,#9206,#9207));
#2213=EDGE_LOOP('',(#9208,#9209,#9210));
#2214=EDGE_LOOP('',(#9211,#9212,#9213,#9214));
#2215=EDGE_LOOP('',(#9215,#9216,#9217,#9218));
#2216=EDGE_LOOP('',(#9219,#9220,#9221,#9222));
#2217=EDGE_LOOP('',(#9223,#9224,#9225));
#2218=EDGE_LOOP('',(#9226,#9227,#9228));
#2219=EDGE_LOOP('',(#9229,#9230,#9231,#9232));
#2220=EDGE_LOOP('',(#9233,#9234,#9235,#9236));
#2221=EDGE_LOOP('',(#9237,#9238,#9239,#9240));
#2222=EDGE_LOOP('',(#9241,#9242,#9243));
#2223=EDGE_LOOP('',(#9244,#9245,#9246));
#2224=EDGE_LOOP('',(#9247,#9248,#9249,#9250));
#2225=EDGE_LOOP('',(#9251,#9252,#9253,#9254));
#2226=EDGE_LOOP('',(#9255,#9256,#9257,#9258));
#2227=EDGE_LOOP('',(#9259,#9260,#9261,#9262));
#2228=EDGE_LOOP('',(#9263,#9264,#9265,#9266));
#2229=EDGE_LOOP('',(#9267,#9268,#9269,#9270));
#2230=EDGE_LOOP('',(#9271,#9272,#9273,#9274));
#2231=EDGE_LOOP('',(#9275,#9276,#9277,#9278));
#2232=EDGE_LOOP('',(#9279,#9280,#9281,#9282));
#2233=EDGE_LOOP('',(#9283,#9284,#9285));
#2234=EDGE_LOOP('',(#9286,#9287,#9288));
#2235=EDGE_LOOP('',(#9289,#9290,#9291));
#2236=EDGE_LOOP('',(#9292,#9293,#9294,#9295));
#2237=EDGE_LOOP('',(#9296,#9297,#9298,#9299));
#2238=EDGE_LOOP('',(#9300,#9301,#9302));
#2239=EDGE_LOOP('',(#9303,#9304,#9305,#9306));
#2240=EDGE_LOOP('',(#9307,#9308,#9309,#9310));
#2241=EDGE_LOOP('',(#9311,#9312,#9313,#9314));
#2242=EDGE_LOOP('',(#9315,#9316,#9317,#9318));
#2243=EDGE_LOOP('',(#9319,#9320,#9321,#9322));
#2244=EDGE_LOOP('',(#9323,#9324,#9325,#9326));
#2245=EDGE_LOOP('',(#9327,#9328,#9329,#9330));
#2246=EDGE_LOOP('',(#9331,#9332,#9333,#9334));
#2247=EDGE_LOOP('',(#9335,#9336,#9337,#9338));
#2248=EDGE_LOOP('',(#9339,#9340,#9341));
#2249=EDGE_LOOP('',(#9342,#9343,#9344,#9345));
#2250=EDGE_LOOP('',(#9346,#9347,#9348,#9349));
#2251=EDGE_LOOP('',(#9350,#9351,#9352,#9353));
#2252=EDGE_LOOP('',(#9354,#9355,#9356));
#2253=EDGE_LOOP('',(#9357,#9358,#9359,#9360));
#2254=EDGE_LOOP('',(#9361,#9362,#9363,#9364));
#2255=EDGE_LOOP('',(#9365,#9366,#9367,#9368,#9369));
#2256=EDGE_LOOP('',(#9370,#9371,#9372,#9373));
#2257=EDGE_LOOP('',(#9374,#9375,#9376,#9377));
#2258=EDGE_LOOP('',(#9378,#9379,#9380,#9381));
#2259=EDGE_LOOP('',(#9382,#9383,#9384,#9385));
#2260=EDGE_LOOP('',(#9386,#9387,#9388,#9389));
#2261=EDGE_LOOP('',(#9390,#9391,#9392,#9393));
#2262=EDGE_LOOP('',(#9394,#9395,#9396,#9397));
#2263=EDGE_LOOP('',(#9398,#9399,#9400,#9401));
#2264=EDGE_LOOP('',(#9402,#9403,#9404,#9405));
#2265=EDGE_LOOP('',(#9406,#9407,#9408));
#2266=EDGE_LOOP('',(#9409,#9410,#9411,#9412));
#2267=EDGE_LOOP('',(#9413,#9414,#9415,#9416));
#2268=EDGE_LOOP('',(#9417,#9418,#9419));
#2269=EDGE_LOOP('',(#9420,#9421,#9422,#9423));
#2270=EDGE_LOOP('',(#9424,#9425,#9426,#9427));
#2271=EDGE_LOOP('',(#9428,#9429,#9430));
#2272=EDGE_LOOP('',(#9431,#9432,#9433));
#2273=EDGE_LOOP('',(#9434,#9435,#9436,#9437));
#2274=EDGE_LOOP('',(#9438,#9439,#9440,#9441));
#2275=EDGE_LOOP('',(#9442,#9443,#9444,#9445));
#2276=EDGE_LOOP('',(#9446,#9447,#9448,#9449));
#2277=EDGE_LOOP('',(#9450,#9451,#9452,#9453));
#2278=EDGE_LOOP('',(#9454,#9455,#9456,#9457));
#2279=EDGE_LOOP('',(#9458,#9459,#9460,#9461));
#2280=EDGE_LOOP('',(#9462,#9463,#9464,#9465));
#2281=EDGE_LOOP('',(#9466,#9467,#9468,#9469));
#2282=EDGE_LOOP('',(#9470,#9471,#9472,#9473));
#2283=EDGE_LOOP('',(#9474,#9475,#9476,#9477));
#2284=EDGE_LOOP('',(#9478,#9479,#9480,#9481));
#2285=EDGE_LOOP('',(#9482,#9483,#9484,#9485));
#2286=EDGE_LOOP('',(#9486,#9487,#9488));
#2287=EDGE_LOOP('',(#9489,#9490,#9491));
#2288=EDGE_LOOP('',(#9492,#9493,#9494,#9495));
#2289=EDGE_LOOP('',(#9496,#9497,#9498,#9499));
#2290=EDGE_LOOP('',(#9500,#9501,#9502));
#2291=EDGE_LOOP('',(#9503,#9504,#9505));
#2292=EDGE_LOOP('',(#9506,#9507,#9508,#9509,#9510));
#2293=EDGE_LOOP('',(#9511,#9512,#9513,#9514));
#2294=EDGE_LOOP('',(#9515,#9516,#9517,#9518));
#2295=EDGE_LOOP('',(#9519,#9520,#9521,#9522));
#2296=EDGE_LOOP('',(#9523,#9524,#9525,#9526));
#2297=EDGE_LOOP('',(#9527,#9528,#9529,#9530));
#2298=EDGE_LOOP('',(#9531,#9532,#9533,#9534));
#2299=EDGE_LOOP('',(#9535,#9536,#9537,#9538));
#2300=EDGE_LOOP('',(#9539,#9540,#9541,#9542));
#2301=EDGE_LOOP('',(#9543,#9544,#9545,#9546));
#2302=EDGE_LOOP('',(#9547,#9548,#9549,#9550));
#2303=EDGE_LOOP('',(#9551,#9552,#9553,#9554));
#2304=EDGE_LOOP('',(#9555,#9556,#9557,#9558));
#2305=EDGE_LOOP('',(#9559,#9560,#9561,#9562));
#2306=EDGE_LOOP('',(#9563,#9564,#9565,#9566));
#2307=EDGE_LOOP('',(#9567,#9568,#9569));
#2308=EDGE_LOOP('',(#9570,#9571,#9572));
#2309=EDGE_LOOP('',(#9573,#9574,#9575));
#2310=EDGE_LOOP('',(#9576,#9577,#9578,#9579));
#2311=EDGE_LOOP('',(#9580,#9581,#9582,#9583));
#2312=EDGE_LOOP('',(#9584,#9585,#9586));
#2313=EDGE_LOOP('',(#9587,#9588,#9589,#9590));
#2314=EDGE_LOOP('',(#9591,#9592,#9593,#9594));
#2315=EDGE_LOOP('',(#9595,#9596,#9597,#9598));
#2316=EDGE_LOOP('',(#9599,#9600,#9601,#9602));
#2317=EDGE_LOOP('',(#9603,#9604,#9605,#9606));
#2318=EDGE_LOOP('',(#9607,#9608,#9609,#9610));
#2319=EDGE_LOOP('',(#9611,#9612,#9613,#9614));
#2320=EDGE_LOOP('',(#9615,#9616,#9617,#9618));
#2321=EDGE_LOOP('',(#9619,#9620,#9621,#9622));
#2322=EDGE_LOOP('',(#9623,#9624,#9625,#9626));
#2323=EDGE_LOOP('',(#9627,#9628,#9629,#9630));
#2324=EDGE_LOOP('',(#9631,#9632,#9633,#9634));
#2325=EDGE_LOOP('',(#9635,#9636,#9637));
#2326=EDGE_LOOP('',(#9638,#9639,#9640,#9641));
#2327=EDGE_LOOP('',(#9642,#9643,#9644));
#2328=EDGE_LOOP('',(#9645,#9646,#9647,#9648));
#2329=EDGE_LOOP('',(#9649,#9650,#9651,#9652));
#2330=EDGE_LOOP('',(#9653,#9654,#9655,#9656));
#2331=EDGE_LOOP('',(#9657,#9658,#9659,#9660));
#2332=EDGE_LOOP('',(#9661,#9662,#9663,#9664));
#2333=EDGE_LOOP('',(#9665,#9666,#9667,#9668));
#2334=EDGE_LOOP('',(#9669,#9670,#9671,#9672));
#2335=EDGE_LOOP('',(#9673,#9674,#9675,#9676));
#2336=EDGE_LOOP('',(#9677,#9678,#9679,#9680));
#2337=EDGE_LOOP('',(#9681,#9682,#9683,#9684));
#2338=EDGE_LOOP('',(#9685,#9686,#9687,#9688));
#2339=EDGE_LOOP('',(#9689,#9690,#9691,#9692));
#2340=EDGE_LOOP('',(#9693,#9694,#9695));
#2341=EDGE_LOOP('',(#9696,#9697,#9698));
#2342=EDGE_LOOP('',(#9699,#9700,#9701));
#2343=EDGE_LOOP('',(#9702,#9703,#9704));
#2344=EDGE_LOOP('',(#9705,#9706,#9707,#9708,#9709));
#2345=EDGE_LOOP('',(#9710,#9711,#9712,#9713));
#2346=EDGE_LOOP('',(#9714,#9715,#9716,#9717));
#2347=EDGE_LOOP('',(#9718,#9719,#9720,#9721));
#2348=EDGE_LOOP('',(#9722,#9723,#9724,#9725));
#2349=EDGE_LOOP('',(#9726,#9727,#9728,#9729));
#2350=EDGE_LOOP('',(#9730,#9731,#9732,#9733));
#2351=EDGE_LOOP('',(#9734,#9735,#9736,#9737));
#2352=EDGE_LOOP('',(#9738,#9739,#9740));
#2353=EDGE_LOOP('',(#9741,#9742,#9743));
#2354=EDGE_LOOP('',(#9744,#9745,#9746,#9747));
#2355=EDGE_LOOP('',(#9748,#9749,#9750,#9751));
#2356=EDGE_LOOP('',(#9752,#9753,#9754,#9755));
#2357=EDGE_LOOP('',(#9756,#9757,#9758));
#2358=EDGE_LOOP('',(#9759,#9760,#9761));
#2359=EDGE_LOOP('',(#9762,#9763,#9764,#9765));
#2360=EDGE_LOOP('',(#9766,#9767,#9768,#9769));
#2361=EDGE_LOOP('',(#9770,#9771,#9772,#9773));
#2362=EDGE_LOOP('',(#9774,#9775,#9776,#9777));
#2363=EDGE_LOOP('',(#9778,#9779,#9780,#9781));
#2364=EDGE_LOOP('',(#9782,#9783,#9784,#9785));
#2365=EDGE_LOOP('',(#9786,#9787,#9788,#9789));
#2366=EDGE_LOOP('',(#9790,#9791,#9792,#9793));
#2367=EDGE_LOOP('',(#9794,#9795,#9796,#9797));
#2368=EDGE_LOOP('',(#9798,#9799,#9800,#9801));
#2369=EDGE_LOOP('',(#9802,#9803,#9804,#9805));
#2370=EDGE_LOOP('',(#9806,#9807,#9808,#9809));
#2371=EDGE_LOOP('',(#9810,#9811,#9812,#9813));
#2372=EDGE_LOOP('',(#9814,#9815,#9816,#9817));
#2373=EDGE_LOOP('',(#9818,#9819,#9820,#9821));
#2374=EDGE_LOOP('',(#9822,#9823,#9824,#9825));
#2375=EDGE_LOOP('',(#9826,#9827,#9828,#9829));
#2376=EDGE_LOOP('',(#9830,#9831,#9832,#9833));
#2377=EDGE_LOOP('',(#9834,#9835,#9836,#9837));
#2378=EDGE_LOOP('',(#9838,#9839,#9840,#9841));
#2379=EDGE_LOOP('',(#9842,#9843,#9844,#9845));
#2380=EDGE_LOOP('',(#9846,#9847,#9848,#9849));
#2381=EDGE_LOOP('',(#9850,#9851,#9852,#9853));
#2382=EDGE_LOOP('',(#9854,#9855,#9856,#9857));
#2383=EDGE_LOOP('',(#9858,#9859,#9860,#9861,#9862));
#2384=EDGE_LOOP('',(#9863,#9864,#9865,#9866,#9867));
#2385=EDGE_LOOP('',(#9868,#9869,#9870,#9871));
#2386=EDGE_LOOP('',(#9872,#9873,#9874,#9875));
#2387=EDGE_LOOP('',(#9876,#9877,#9878,#9879));
#2388=EDGE_LOOP('',(#9880,#9881,#9882,#9883));
#2389=EDGE_LOOP('',(#9884,#9885,#9886,#9887));
#2390=EDGE_LOOP('',(#9888,#9889,#9890,#9891));
#2391=EDGE_LOOP('',(#9892,#9893,#9894,#9895));
#2392=EDGE_LOOP('',(#9896,#9897,#9898,#9899,#9900));
#2393=EDGE_LOOP('',(#9901,#9902,#9903,#9904,#9905,#9906));
#2394=EDGE_LOOP('',(#9907,#9908,#9909,#9910,#9911,#9912));
#2395=EDGE_LOOP('',(#9913,#9914,#9915,#9916,#9917));
#2396=EDGE_LOOP('',(#9918,#9919,#9920,#9921,#9922));
#2397=EDGE_LOOP('',(#9923,#9924,#9925,#9926));
#2398=EDGE_LOOP('',(#9927,#9928,#9929,#9930));
#2399=EDGE_LOOP('',(#9931,#9932,#9933,#9934,#9935));
#2400=EDGE_LOOP('',(#9936,#9937,#9938,#9939));
#2401=EDGE_LOOP('',(#9940,#9941,#9942,#9943));
#2402=EDGE_LOOP('',(#9944,#9945,#9946,#9947));
#2403=EDGE_LOOP('',(#9948,#9949,#9950,#9951));
#2404=EDGE_LOOP('',(#9952,#9953,#9954,#9955,#9956,#9957));
#2405=EDGE_LOOP('',(#9958,#9959,#9960,#9961,#9962,#9963));
#2406=EDGE_LOOP('',(#9964,#9965,#9966,#9967,#9968));
#2407=EDGE_LOOP('',(#9969,#9970,#9971,#9972));
#2408=EDGE_LOOP('',(#9973,#9974,#9975,#9976));
#2409=EDGE_LOOP('',(#9977,#9978,#9979,#9980));
#2410=EDGE_LOOP('',(#9981,#9982,#9983,#9984));
#2411=EDGE_LOOP('',(#9985,#9986,#9987,#9988,#9989));
#2412=EDGE_LOOP('',(#9990,#9991,#9992,#9993));
#2413=EDGE_LOOP('',(#9994,#9995,#9996,#9997));
#2414=EDGE_LOOP('',(#9998,#9999,#10000,#10001));
#2415=EDGE_LOOP('',(#10002,#10003,#10004,#10005));
#2416=EDGE_LOOP('',(#10006,#10007,#10008,#10009));
#2417=EDGE_LOOP('',(#10010,#10011,#10012,#10013));
#2418=EDGE_LOOP('',(#10014,#10015,#10016,#10017));
#2419=EDGE_LOOP('',(#10018,#10019,#10020,#10021));
#2420=EDGE_LOOP('',(#10022,#10023,#10024,#10025));
#2421=EDGE_LOOP('',(#10026,#10027,#10028,#10029));
#2422=EDGE_LOOP('',(#10030,#10031,#10032,#10033));
#2423=EDGE_LOOP('',(#10034,#10035,#10036,#10037));
#2424=EDGE_LOOP('',(#10038,#10039,#10040,#10041));
#2425=EDGE_LOOP('',(#10042,#10043,#10044,#10045));
#2426=EDGE_LOOP('',(#10046,#10047,#10048,#10049));
#2427=EDGE_LOOP('',(#10050,#10051,#10052,#10053));
#2428=EDGE_LOOP('',(#10054,#10055,#10056,#10057));
#2429=EDGE_LOOP('',(#10058,#10059,#10060,#10061));
#2430=EDGE_LOOP('',(#10062,#10063,#10064,#10065));
#2431=EDGE_LOOP('',(#10066,#10067,#10068,#10069));
#2432=EDGE_LOOP('',(#10070,#10071,#10072,#10073));
#2433=EDGE_LOOP('',(#10074,#10075,#10076,#10077));
#2434=EDGE_LOOP('',(#10078,#10079,#10080,#10081));
#2435=EDGE_LOOP('',(#10082,#10083,#10084,#10085));
#2436=EDGE_LOOP('',(#10086,#10087,#10088,#10089));
#2437=EDGE_LOOP('',(#10090,#10091,#10092,#10093));
#2438=EDGE_LOOP('',(#10094,#10095,#10096,#10097));
#2439=EDGE_LOOP('',(#10098,#10099,#10100,#10101));
#2440=EDGE_LOOP('',(#10102,#10103,#10104,#10105));
#2441=EDGE_LOOP('',(#10106,#10107,#10108,#10109));
#2442=EDGE_LOOP('',(#10110,#10111,#10112,#10113));
#2443=EDGE_LOOP('',(#10114,#10115,#10116,#10117));
#2444=EDGE_LOOP('',(#10118,#10119,#10120,#10121));
#2445=EDGE_LOOP('',(#10122,#10123,#10124,#10125));
#2446=EDGE_LOOP('',(#10126,#10127,#10128,#10129));
#2447=EDGE_LOOP('',(#10130,#10131,#10132,#10133));
#2448=EDGE_LOOP('',(#10134,#10135,#10136,#10137));
#2449=EDGE_LOOP('',(#10138,#10139,#10140,#10141));
#2450=EDGE_LOOP('',(#10142,#10143,#10144,#10145));
#2451=EDGE_LOOP('',(#10146,#10147,#10148,#10149));
#2452=EDGE_LOOP('',(#10150,#10151,#10152,#10153));
#2453=EDGE_LOOP('',(#10154,#10155,#10156,#10157));
#2454=EDGE_LOOP('',(#10158,#10159,#10160,#10161));
#2455=EDGE_LOOP('',(#10162,#10163,#10164,#10165));
#2456=EDGE_LOOP('',(#10166,#10167,#10168,#10169));
#2457=EDGE_LOOP('',(#10170,#10171,#10172,#10173));
#2458=EDGE_LOOP('',(#10174,#10175,#10176,#10177));
#2459=EDGE_LOOP('',(#10178,#10179,#10180,#10181));
#2460=EDGE_LOOP('',(#10182,#10183,#10184,#10185));
#2461=EDGE_LOOP('',(#10186,#10187,#10188,#10189));
#2462=EDGE_LOOP('',(#10190,#10191,#10192,#10193));
#2463=EDGE_LOOP('',(#10194,#10195,#10196,#10197));
#2464=EDGE_LOOP('',(#10198,#10199,#10200,#10201));
#2465=EDGE_LOOP('',(#10202,#10203,#10204,#10205));
#2466=EDGE_LOOP('',(#10206,#10207,#10208,#10209));
#2467=EDGE_LOOP('',(#10210,#10211,#10212,#10213));
#2468=EDGE_LOOP('',(#10214,#10215,#10216,#10217,#10218,#10219,#10220,#10221,
#10222,#10223));
#2469=EDGE_LOOP('',(#10224,#10225,#10226,#10227));
#2470=EDGE_LOOP('',(#10228));
#2471=EDGE_LOOP('',(#10229));
#2472=EDGE_LOOP('',(#10230));
#2473=EDGE_LOOP('',(#10231));
#2474=EDGE_LOOP('',(#10232));
#2475=EDGE_LOOP('',(#10233));
#2476=EDGE_LOOP('',(#10234,#10235,#10236,#10237,#10238,#10239,#10240,#10241));
#2477=EDGE_LOOP('',(#10242,#10243,#10244,#10245,#10246,#10247,#10248,#10249));
#2478=EDGE_LOOP('',(#10250,#10251,#10252,#10253));
#2479=EDGE_LOOP('',(#10254,#10255,#10256,#10257,#10258,#10259));
#2480=EDGE_LOOP('',(#10260,#10261,#10262,#10263,#10264));
#2481=EDGE_LOOP('',(#10265,#10266,#10267,#10268,#10269,#10270));
#2482=EDGE_LOOP('',(#10271,#10272,#10273,#10274));
#2483=EDGE_LOOP('',(#10275,#10276,#10277,#10278));
#2484=EDGE_LOOP('',(#10279,#10280,#10281,#10282,#10283,#10284));
#2485=EDGE_LOOP('',(#10285,#10286,#10287,#10288));
#2486=EDGE_LOOP('',(#10289,#10290,#10291,#10292,#10293,#10294));
#2487=EDGE_LOOP('',(#10295,#10296,#10297,#10298));
#2488=EDGE_LOOP('',(#10299,#10300,#10301,#10302,#10303,#10304,#10305));
#2489=EDGE_LOOP('',(#10306,#10307,#10308,#10309,#10310,#10311));
#2490=EDGE_LOOP('',(#10312,#10313,#10314,#10315));
#2491=EDGE_LOOP('',(#10316,#10317,#10318,#10319,#10320,#10321,#10322));
#2492=EDGE_LOOP('',(#10323,#10324,#10325,#10326));
#2493=EDGE_LOOP('',(#10327,#10328,#10329,#10330));
#2537=LINE('',#16379,#2975);
#2538=LINE('',#16385,#2976);
#2539=LINE('',#16391,#2977);
#2540=LINE('',#16397,#2978);
#2541=LINE('',#16668,#2979);
#2542=LINE('',#16671,#2980);
#2543=LINE('',#16677,#2981);
#2544=LINE('',#16680,#2982);
#2545=LINE('',#16686,#2983);
#2546=LINE('',#16689,#2984);
#2547=LINE('',#16701,#2985);
#2548=LINE('',#16704,#2986);
#2549=LINE('',#16710,#2987);
#2550=LINE('',#16713,#2988);
#2551=LINE('',#16719,#2989);
#2552=LINE('',#16722,#2990);
#2553=LINE('',#16728,#2991);
#2554=LINE('',#16731,#2992);
#2555=LINE('',#16764,#2993);
#2556=LINE('',#16767,#2994);
#2557=LINE('',#16771,#2995);
#2558=LINE('',#16774,#2996);
#2559=LINE('',#16776,#2997);
#2560=LINE('',#16778,#2998);
#2561=LINE('',#16781,#2999);
#2562=LINE('',#16784,#3000);
#2563=LINE('',#16790,#3001);
#2564=LINE('',#16793,#3002);
#2565=LINE('',#16798,#3003);
#2566=LINE('',#16800,#3004);
#2567=LINE('',#16802,#3005);
#2568=LINE('',#16804,#3006);
#2569=LINE('',#16851,#3007);
#2570=LINE('',#16854,#3008);
#2571=LINE('',#16860,#3009);
#2572=LINE('',#16863,#3010);
#2573=LINE('',#16865,#3011);
#2574=LINE('',#16866,#3012);
#2575=LINE('',#16868,#3013);
#2576=LINE('',#16870,#3014);
#2577=LINE('',#16922,#3015);
#2578=LINE('',#16923,#3016);
#2579=LINE('',#16925,#3017);
#2580=LINE('',#16926,#3018);
#2581=LINE('',#16928,#3019);
#2582=LINE('',#16929,#3020);
#2583=LINE('',#16945,#3021);
#2584=LINE('',#16998,#3022);
#2585=LINE('',#17002,#3023);
#2586=LINE('',#17073,#3024);
#2587=LINE('',#17175,#3025);
#2588=LINE('',#17247,#3026);
#2589=LINE('',#17251,#3027);
#2590=LINE('',#17352,#3028);
#2591=LINE('',#17356,#3029);
#2592=LINE('',#17428,#3030);
#2593=LINE('',#17530,#3031);
#2594=LINE('',#17601,#3032);
#2595=LINE('',#17605,#3033);
#2596=LINE('',#17665,#3034);
#2597=LINE('',#17667,#3035);
#2598=LINE('',#17719,#3036);
#2599=LINE('',#17720,#3037);
#2600=LINE('',#17726,#3038);
#2601=LINE('',#17729,#3039);
#2602=LINE('',#17733,#3040);
#2603=LINE('',#17735,#3041);
#2604=LINE('',#17737,#3042);
#2605=LINE('',#17738,#3043);
#2606=LINE('',#17744,#3044);
#2607=LINE('',#17752,#3045);
#2608=LINE('',#17754,#3046);
#2609=LINE('',#17756,#3047);
#2610=LINE('',#17758,#3048);
#2611=LINE('',#17762,#3049);
#2612=LINE('',#17766,#3050);
#2613=LINE('',#17770,#3051);
#2614=LINE('',#17778,#3052);
#2615=LINE('',#17783,#3053);
#2616=LINE('',#17790,#3054);
#2617=LINE('',#17794,#3055);
#2618=LINE('',#17798,#3056);
#2619=LINE('',#17803,#3057);
#2620=LINE('',#17827,#3058);
#2621=LINE('',#17871,#3059);
#2622=LINE('',#17904,#3060);
#2623=LINE('',#17947,#3061);
#2624=LINE('',#17951,#3062);
#2625=LINE('',#17953,#3063);
#2626=LINE('',#17955,#3064);
#2627=LINE('',#17956,#3065);
#2628=LINE('',#17960,#3066);
#2629=LINE('',#17962,#3067);
#2630=LINE('',#17964,#3068);
#2631=LINE('',#17965,#3069);
#2632=LINE('',#17969,#3070);
#2633=LINE('',#17971,#3071);
#2634=LINE('',#17973,#3072);
#2635=LINE('',#17975,#3073);
#2636=LINE('',#17977,#3074);
#2637=LINE('',#17979,#3075);
#2638=LINE('',#17981,#3076);
#2639=LINE('',#17985,#3077);
#2640=LINE('',#17989,#3078);
#2641=LINE('',#17993,#3079);
#2642=LINE('',#17997,#3080);
#2643=LINE('',#17999,#3081);
#2644=LINE('',#18001,#3082);
#2645=LINE('',#18002,#3083);
#2646=LINE('',#18006,#3084);
#2647=LINE('',#18008,#3085);
#2648=LINE('',#18012,#3086);
#2649=LINE('',#18015,#3087);
#2650=LINE('',#18017,#3088);
#2651=LINE('',#18021,#3089);
#2652=LINE('',#18023,#3090);
#2653=LINE('',#18025,#3091);
#2654=LINE('',#18027,#3092);
#2655=LINE('',#18029,#3093);
#2656=LINE('',#18031,#3094);
#2657=LINE('',#18032,#3095);
#2658=LINE('',#18036,#3096);
#2659=LINE('',#18037,#3097);
#2660=LINE('',#18038,#3098);
#2661=LINE('',#18039,#3099);
#2662=LINE('',#18049,#3100);
#2663=LINE('',#18060,#3101);
#2664=LINE('',#18064,#3102);
#2665=LINE('',#18066,#3103);
#2666=LINE('',#18068,#3104);
#2667=LINE('',#18069,#3105);
#2668=LINE('',#18074,#3106);
#2669=LINE('',#18081,#3107);
#2670=LINE('',#18085,#3108);
#2671=LINE('',#18091,#3109);
#2672=LINE('',#18092,#3110);
#2673=LINE('',#18132,#3111);
#2674=LINE('',#18209,#3112);
#2675=LINE('',#18289,#3113);
#2676=LINE('',#18363,#3114);
#2677=LINE('',#18474,#3115);
#2678=LINE('',#18475,#3116);
#2679=LINE('',#18481,#3117);
#2680=LINE('',#18485,#3118);
#2681=LINE('',#18491,#3119);
#2682=LINE('',#18495,#3120);
#2683=LINE('',#18501,#3121);
#2684=LINE('',#18504,#3122);
#2685=LINE('',#18508,#3123);
#2686=LINE('',#18512,#3124);
#2687=LINE('',#18513,#3125);
#2688=LINE('',#18515,#3126);
#2689=LINE('',#18522,#3127);
#2690=LINE('',#18523,#3128);
#2691=LINE('',#18560,#3129);
#2692=LINE('',#18563,#3130);
#2693=LINE('',#18567,#3131);
#2694=LINE('',#18569,#3132);
#2695=LINE('',#18571,#3133);
#2696=LINE('',#18573,#3134);
#2697=LINE('',#18577,#3135);
#2698=LINE('',#18781,#3136);
#2699=LINE('',#18785,#3137);
#2700=LINE('',#18793,#3138);
#2701=LINE('',#18797,#3139);
#2702=LINE('',#18833,#3140);
#2703=LINE('',#18837,#3141);
#2704=LINE('',#18885,#3142);
#2705=LINE('',#18889,#3143);
#2706=LINE('',#18892,#3144);
#2707=LINE('',#18894,#3145);
#2708=LINE('',#18899,#3146);
#2709=LINE('',#18903,#3147);
#2710=LINE('',#18907,#3148);
#2711=LINE('',#18911,#3149);
#2712=LINE('',#18936,#3150);
#2713=LINE('',#18938,#3151);
#2714=LINE('',#18940,#3152);
#2715=LINE('',#18942,#3153);
#2716=LINE('',#18944,#3154);
#2717=LINE('',#19029,#3155);
#2718=LINE('',#19031,#3156);
#2719=LINE('',#19150,#3157);
#2720=LINE('',#19152,#3158);
#2721=LINE('',#19153,#3159);
#2722=LINE('',#19160,#3160);
#2723=LINE('',#19162,#3161);
#2724=LINE('',#19227,#3162);
#2725=LINE('',#19229,#3163);
#2726=LINE('',#19230,#3164);
#2727=LINE('',#19248,#3165);
#2728=LINE('',#19250,#3166);
#2729=LINE('',#19252,#3167);
#2730=LINE('',#19254,#3168);
#2731=LINE('',#19256,#3169);
#2732=LINE('',#19293,#3170);
#2733=LINE('',#19295,#3171);
#2734=LINE('',#19297,#3172);
#2735=LINE('',#19299,#3173);
#2736=LINE('',#19301,#3174);
#2737=LINE('',#19303,#3175);
#2738=LINE('',#19383,#3176);
#2739=LINE('',#19452,#3177);
#2740=LINE('',#19457,#3178);
#2741=LINE('',#19459,#3179);
#2742=LINE('',#19461,#3180);
#2743=LINE('',#19463,#3181);
#2744=LINE('',#19465,#3182);
#2745=LINE('',#19466,#3183);
#2746=LINE('',#19470,#3184);
#2747=LINE('',#19474,#3185);
#2748=LINE('',#19478,#3186);
#2749=LINE('',#19540,#3187);
#2750=LINE('',#19546,#3188);
#2751=LINE('',#19629,#3189);
#2752=LINE('',#19698,#3190);
#2753=LINE('',#19701,#3191);
#2754=LINE('',#19784,#3192);
#2755=LINE('',#19799,#3193);
#2756=LINE('',#19882,#3194);
#2757=LINE('',#19950,#3195);
#2758=LINE('',#20017,#3196);
#2759=LINE('',#20091,#3197);
#2760=LINE('',#20139,#3198);
#2761=LINE('',#20141,#3199);
#2762=LINE('',#20142,#3200);
#2763=LINE('',#20145,#3201);
#2764=LINE('',#20154,#3202);
#2765=LINE('',#20156,#3203);
#2766=LINE('',#20157,#3204);
#2767=LINE('',#20161,#3205);
#2768=LINE('',#20165,#3206);
#2769=LINE('',#20170,#3207);
#2770=LINE('',#20174,#3208);
#2771=LINE('',#20179,#3209);
#2772=LINE('',#20188,#3210);
#2773=LINE('',#20192,#3211);
#2774=LINE('',#20196,#3212);
#2775=LINE('',#20201,#3213);
#2776=LINE('',#20207,#3214);
#2777=LINE('',#20212,#3215);
#2778=LINE('',#20217,#3216);
#2779=LINE('',#20218,#3217);
#2780=LINE('',#20219,#3218);
#2781=LINE('',#20223,#3219);
#2782=LINE('',#20225,#3220);
#2783=LINE('',#20227,#3221);
#2784=LINE('',#20228,#3222);
#2785=LINE('',#20232,#3223);
#2786=LINE('',#20238,#3224);
#2787=LINE('',#20321,#3225);
#2788=LINE('',#20323,#3226);
#2789=LINE('',#20325,#3227);
#2790=LINE('',#20362,#3228);
#2791=LINE('',#20365,#3229);
#2792=LINE('',#20368,#3230);
#2793=LINE('',#20370,#3231);
#2794=LINE('',#20372,#3232);
#2795=LINE('',#20376,#3233);
#2796=LINE('',#20534,#3234);
#2797=LINE('',#20538,#3235);
#2798=LINE('',#20543,#3236);
#2799=LINE('',#20547,#3237);
#2800=LINE('',#20595,#3238);
#2801=LINE('',#20599,#3239);
#2802=LINE('',#20602,#3240);
#2803=LINE('',#20604,#3241);
#2804=LINE('',#20609,#3242);
#2805=LINE('',#20613,#3243);
#2806=LINE('',#20617,#3244);
#2807=LINE('',#20621,#3245);
#2808=LINE('',#20626,#3246);
#2809=LINE('',#20628,#3247);
#2810=LINE('',#20630,#3248);
#2811=LINE('',#20632,#3249);
#2812=LINE('',#20634,#3250);
#2813=LINE('',#20742,#3251);
#2814=LINE('',#20744,#3252);
#2815=LINE('',#20746,#3253);
#2816=LINE('',#20811,#3254);
#2817=LINE('',#20812,#3255);
#2818=LINE('',#20879,#3256);
#2819=LINE('',#20925,#3257);
#2820=LINE('',#20927,#3258);
#2821=LINE('',#20929,#3259);
#2822=LINE('',#20930,#3260);
#2823=LINE('',#20933,#3261);
#2824=LINE('',#20941,#3262);
#2825=LINE('',#20942,#3263);
#2826=LINE('',#20945,#3264);
#2827=LINE('',#20951,#3265);
#2828=LINE('',#20955,#3266);
#2829=LINE('',#20960,#3267);
#2830=LINE('',#20969,#3268);
#2831=LINE('',#20973,#3269);
#2832=LINE('',#20977,#3270);
#2833=LINE('',#20982,#3271);
#2834=LINE('',#20988,#3272);
#2835=LINE('',#20991,#3273);
#2836=LINE('',#20996,#3274);
#2837=LINE('',#20997,#3275);
#2838=LINE('',#20998,#3276);
#2839=LINE('',#21000,#3277);
#2840=LINE('',#21002,#3278);
#2841=LINE('',#21004,#3279);
#2842=LINE('',#21005,#3280);
#2843=LINE('',#21010,#3281);
#2844=LINE('',#21015,#3282);
#2845=LINE('',#21097,#3283);
#2846=LINE('',#21099,#3284);
#2847=LINE('',#21101,#3285);
#2848=LINE('',#21103,#3286);
#2849=LINE('',#21140,#3287);
#2850=LINE('',#21145,#3288);
#2851=LINE('',#21147,#3289);
#2852=LINE('',#21149,#3290);
#2853=LINE('',#21151,#3291);
#2854=LINE('',#21155,#3292);
#2855=LINE('',#21311,#3293);
#2856=LINE('',#21312,#3294);
#2857=LINE('',#21315,#3295);
#2858=LINE('',#21317,#3296);
#2859=LINE('',#21385,#3297);
#2860=LINE('',#21387,#3298);
#2861=LINE('',#21389,#3299);
#2862=LINE('',#21391,#3300);
#2863=LINE('',#21393,#3301);
#2864=LINE('',#21481,#3302);
#2865=LINE('',#21483,#3303);
#2866=LINE('',#21548,#3304);
#2867=LINE('',#21550,#3305);
#2868=LINE('',#21551,#3306);
#2869=LINE('',#21618,#3307);
#2870=LINE('',#21664,#3308);
#2871=LINE('',#21666,#3309);
#2872=LINE('',#21668,#3310);
#2873=LINE('',#21669,#3311);
#2874=LINE('',#21672,#3312);
#2875=LINE('',#21681,#3313);
#2876=LINE('',#21683,#3314);
#2877=LINE('',#21684,#3315);
#2878=LINE('',#21688,#3316);
#2879=LINE('',#21694,#3317);
#2880=LINE('',#21698,#3318);
#2881=LINE('',#21703,#3319);
#2882=LINE('',#21712,#3320);
#2883=LINE('',#21716,#3321);
#2884=LINE('',#21720,#3322);
#2885=LINE('',#21728,#3323);
#2886=LINE('',#21733,#3324);
#2887=LINE('',#21737,#3325);
#2888=LINE('',#21739,#3326);
#2889=LINE('',#21740,#3327);
#2890=LINE('',#21744,#3328);
#2891=LINE('',#21746,#3329);
#2892=LINE('',#21748,#3330);
#2893=LINE('',#21749,#3331);
#2894=LINE('',#21753,#3332);
#2895=LINE('',#21755,#3333);
#2896=LINE('',#21763,#3334);
#2897=LINE('',#21768,#3335);
#2898=LINE('',#21769,#3336);
#2899=LINE('',#21849,#3337);
#2900=LINE('',#21851,#3338);
#2901=LINE('',#21888,#3339);
#2902=LINE('',#21891,#3340);
#2903=LINE('',#21895,#3341);
#2904=LINE('',#21896,#3342);
#2905=LINE('',#21898,#3343);
#2906=LINE('',#21902,#3344);
#2907=LINE('',#22060,#3345);
#2908=LINE('',#22064,#3346);
#2909=LINE('',#22068,#3347);
#2910=LINE('',#22072,#3348);
#2911=LINE('',#22077,#3349);
#2912=LINE('',#22081,#3350);
#2913=LINE('',#22084,#3351);
#2914=LINE('',#22086,#3352);
#2915=LINE('',#22126,#3353);
#2916=LINE('',#22128,#3354);
#2917=LINE('',#22130,#3355);
#2918=LINE('',#22131,#3356);
#2919=LINE('',#22134,#3357);
#2920=LINE('',#22143,#3358);
#2921=LINE('',#22145,#3359);
#2922=LINE('',#22146,#3360);
#2923=LINE('',#22153,#3361);
#2924=LINE('',#22157,#3362);
#2925=LINE('',#22161,#3363);
#2926=LINE('',#22172,#3364);
#2927=LINE('',#22176,#3365);
#2928=LINE('',#22181,#3366);
#2929=LINE('',#22187,#3367);
#2930=LINE('',#22192,#3368);
#2931=LINE('',#22197,#3369);
#2932=LINE('',#22198,#3370);
#2933=LINE('',#22199,#3371);
#2934=LINE('',#22203,#3372);
#2935=LINE('',#22204,#3373);
#2936=LINE('',#22205,#3374);
#2937=LINE('',#22206,#3375);
#2938=LINE('',#22213,#3376);
#2939=LINE('',#22220,#3377);
#2940=LINE('',#32144,#3378);
#2941=LINE('',#32145,#3379);
#2942=LINE('',#32147,#3380);
#2943=LINE('',#32148,#3381);
#2944=LINE('',#32150,#3382);
#2945=LINE('',#32151,#3383);
#2946=LINE('',#32153,#3384);
#2947=LINE('',#32154,#3385);
#2948=LINE('',#32161,#3386);
#2949=LINE('',#32162,#3387);
#2950=LINE('',#32165,#3388);
#2951=LINE('',#32166,#3389);
#2952=LINE('',#32169,#3390);
#2953=LINE('',#32170,#3391);
#2954=LINE('',#32172,#3392);
#2955=LINE('',#32174,#3393);
#2956=LINE('',#32176,#3394);
#2957=LINE('',#32178,#3395);
#2958=LINE('',#32182,#3396);
#2959=LINE('',#32184,#3397);
#2960=LINE('',#32186,#3398);
#2961=LINE('',#32188,#3399);
#2962=LINE('',#32190,#3400);
#2963=LINE('',#32192,#3401);
#2975=VECTOR('',#13001,2.1875);
#2976=VECTOR('',#13008,2.5625);
#2977=VECTOR('',#13015,3.4375);
#2978=VECTOR('',#13022,1.3125);
#2979=VECTOR('',#13341,1000.);
#2980=VECTOR('',#13344,1000.);
#2981=VECTOR('',#13349,1000.);
#2982=VECTOR('',#13352,1000.);
#2983=VECTOR('',#13357,1000.);
#2984=VECTOR('',#13360,1000.);
#2985=VECTOR('',#13373,1000.);
#2986=VECTOR('',#13376,1000.);
#2987=VECTOR('',#13381,1000.);
#2988=VECTOR('',#13384,1000.);
#2989=VECTOR('',#13389,1000.);
#2990=VECTOR('',#13392,1000.);
#2991=VECTOR('',#13397,1000.);
#2992=VECTOR('',#13400,1000.);
#2993=VECTOR('',#13435,1000.);
#2994=VECTOR('',#13438,1000.);
#2995=VECTOR('',#13443,1000.);
#2996=VECTOR('',#13446,1000.);
#2997=VECTOR('',#13449,2.8125);
#2998=VECTOR('',#13452,2.8125);
#2999=VECTOR('',#13455,1000.);
#3000=VECTOR('',#13458,1000.);
#3001=VECTOR('',#13463,1000.);
#3002=VECTOR('',#13466,1000.);
#3003=VECTOR('',#13471,1000.);
#3004=VECTOR('',#13474,1000.);
#3005=VECTOR('',#13477,2.8125);
#3006=VECTOR('',#13480,2.8125);
#3007=VECTOR('',#13489,1000.);
#3008=VECTOR('',#13492,1000.);
#3009=VECTOR('',#13497,1000.);
#3010=VECTOR('',#13500,1000.);
#3011=VECTOR('',#13503,1000.);
#3012=VECTOR('',#13504,1000.);
#3013=VECTOR('',#13507,2.8125);
#3014=VECTOR('',#13510,2.8125);
#3015=VECTOR('',#13523,1000.);
#3016=VECTOR('',#13524,1000.);
#3017=VECTOR('',#13527,1000.);
#3018=VECTOR('',#13528,1000.);
#3019=VECTOR('',#13531,1000.);
#3020=VECTOR('',#13532,1000.);
#3021=VECTOR('',#13547,48.4375);
#3022=VECTOR('',#13552,1000.);
#3023=VECTOR('',#13555,1000.);
#3024=VECTOR('',#13558,1000.);
#3025=VECTOR('',#13569,1000.);
#3026=VECTOR('',#13574,1000.);
#3027=VECTOR('',#13577,1000.);
#3028=VECTOR('',#13586,1000.);
#3029=VECTOR('',#13589,1000.);
#3030=VECTOR('',#13594,1000.);
#3031=VECTOR('',#13605,1000.);
#3032=VECTOR('',#13608,1000.);
#3033=VECTOR('',#13611,1000.);
#3034=VECTOR('',#13630,2.8125);
#3035=VECTOR('',#13633,2.8125);
#3036=VECTOR('',#13646,1000.);
#3037=VECTOR('',#13647,1000.);
#3038=VECTOR('',#13652,1000.);
#3039=VECTOR('',#13655,1000.);
#3040=VECTOR('',#13658,1000.);
#3041=VECTOR('',#13659,1000.);
#3042=VECTOR('',#13660,1000.);
#3043=VECTOR('',#13661,1000.);
#3044=VECTOR('',#13666,1000.);
#3045=VECTOR('',#13673,1000.);
#3046=VECTOR('',#13674,1000.);
#3047=VECTOR('',#13675,1000.);
#3048=VECTOR('',#13676,1000.);
#3049=VECTOR('',#13679,1000.);
#3050=VECTOR('',#13682,1000.);
#3051=VECTOR('',#13685,1000.);
#3052=VECTOR('',#13692,1000.);
#3053=VECTOR('',#13697,1000.);
#3054=VECTOR('',#13704,1000.);
#3055=VECTOR('',#13709,1000.);
#3056=VECTOR('',#13712,1000.);
#3057=VECTOR('',#13717,1000.);
#3058=VECTOR('',#13722,1000.);
#3059=VECTOR('',#13725,1000.);
#3060=VECTOR('',#13728,1000.);
#3061=VECTOR('',#13731,1000.);
#3062=VECTOR('',#13734,1000.);
#3063=VECTOR('',#13735,1000.);
#3064=VECTOR('',#13736,1000.);
#3065=VECTOR('',#13737,1000.);
#3066=VECTOR('',#13740,1000.);
#3067=VECTOR('',#13741,1000.);
#3068=VECTOR('',#13742,1000.);
#3069=VECTOR('',#13743,1000.);
#3070=VECTOR('',#13746,1000.);
#3071=VECTOR('',#13747,1000.);
#3072=VECTOR('',#13748,1000.);
#3073=VECTOR('',#13749,1000.);
#3074=VECTOR('',#13750,1000.);
#3075=VECTOR('',#13751,1000.);
#3076=VECTOR('',#13752,1000.);
#3077=VECTOR('',#13755,1000.);
#3078=VECTOR('',#13758,1000.);
#3079=VECTOR('',#13761,1000.);
#3080=VECTOR('',#13764,1000.);
#3081=VECTOR('',#13765,1000.);
#3082=VECTOR('',#13766,1000.);
#3083=VECTOR('',#13767,1000.);
#3084=VECTOR('',#13770,1000.);
#3085=VECTOR('',#13771,1000.);
#3086=VECTOR('',#13774,1000.);
#3087=VECTOR('',#13777,1000.);
#3088=VECTOR('',#13778,1000.);
#3089=VECTOR('',#13781,1000.);
#3090=VECTOR('',#13782,1000.);
#3091=VECTOR('',#13783,1000.);
#3092=VECTOR('',#13784,1000.);
#3093=VECTOR('',#13785,1000.);
#3094=VECTOR('',#13786,1000.);
#3095=VECTOR('',#13787,1000.);
#3096=VECTOR('',#13790,1000.);
#3097=VECTOR('',#13791,1000.);
#3098=VECTOR('',#13792,1000.);
#3099=VECTOR('',#13793,1000.);
#3100=VECTOR('',#13808,1000.);
#3101=VECTOR('',#13827,1000.);
#3102=VECTOR('',#13830,1000.);
#3103=VECTOR('',#13831,1000.);
#3104=VECTOR('',#13832,1000.);
#3105=VECTOR('',#13833,1000.);
#3106=VECTOR('',#13838,1000.);
#3107=VECTOR('',#13847,1000.);
#3108=VECTOR('',#13850,1000.);
#3109=VECTOR('',#13855,1000.);
#3110=VECTOR('',#13856,1000.);
#3111=VECTOR('',#13863,1000.);
#3112=VECTOR('',#13870,1000.);
#3113=VECTOR('',#13877,1000.);
#3114=VECTOR('',#13884,1000.);
#3115=VECTOR('',#13899,1000.);
#3116=VECTOR('',#13900,1000.);
#3117=VECTOR('',#13905,1000.);
#3118=VECTOR('',#13908,1000.);
#3119=VECTOR('',#13913,1000.);
#3120=VECTOR('',#13916,1000.);
#3121=VECTOR('',#13921,1000.);
#3122=VECTOR('',#13924,1000.);
#3123=VECTOR('',#13927,1000.);
#3124=VECTOR('',#13930,1000.);
#3125=VECTOR('',#13931,1000.);
#3126=VECTOR('',#13932,1000.);
#3127=VECTOR('',#13939,1000.);
#3128=VECTOR('',#13940,1000.);
#3129=VECTOR('',#13941,1000.);
#3130=VECTOR('',#13944,1000.);
#3131=VECTOR('',#13947,1000.);
#3132=VECTOR('',#13948,1000.);
#3133=VECTOR('',#13949,1000.);
#3134=VECTOR('',#13950,1000.);
#3135=VECTOR('',#13953,1000.);
#3136=VECTOR('',#13974,1000.);
#3137=VECTOR('',#13977,1000.);
#3138=VECTOR('',#13988,10.);
#3139=VECTOR('',#13991,10.);
#3140=VECTOR('',#13998,10.);
#3141=VECTOR('',#14001,10.);
#3142=VECTOR('',#14008,1000.);
#3143=VECTOR('',#14011,1000.);
#3144=VECTOR('',#14014,1000.);
#3145=VECTOR('',#14015,1000.);
#3146=VECTOR('',#14020,1000.);
#3147=VECTOR('',#14023,1000.);
#3148=VECTOR('',#14026,1000.);
#3149=VECTOR('',#14029,1000.);
#3150=VECTOR('',#14034,1000.);
#3151=VECTOR('',#14035,1000.);
#3152=VECTOR('',#14036,1000.);
#3153=VECTOR('',#14037,1000.);
#3154=VECTOR('',#14038,1000.);
#3155=VECTOR('',#14041,1000.);
#3156=VECTOR('',#14042,1000.);
#3157=VECTOR('',#14043,1000.);
#3158=VECTOR('',#14044,1000.);
#3159=VECTOR('',#14045,1000.);
#3160=VECTOR('',#14054,1000.);
#3161=VECTOR('',#14055,1000.);
#3162=VECTOR('',#14056,1000.);
#3163=VECTOR('',#14057,1000.);
#3164=VECTOR('',#14058,1000.);
#3165=VECTOR('',#14061,1000.);
#3166=VECTOR('',#14062,1000.);
#3167=VECTOR('',#14063,1000.);
#3168=VECTOR('',#14064,1000.);
#3169=VECTOR('',#14065,1000.);
#3170=VECTOR('',#14068,1000.);
#3171=VECTOR('',#14069,1000.);
#3172=VECTOR('',#14070,1000.);
#3173=VECTOR('',#14071,1000.);
#3174=VECTOR('',#14072,1000.);
#3175=VECTOR('',#14073,1000.);
#3176=VECTOR('',#14076,1000.);
#3177=VECTOR('',#14079,1000.);
#3178=VECTOR('',#14084,1000.);
#3179=VECTOR('',#14085,1000.);
#3180=VECTOR('',#14086,1000.);
#3181=VECTOR('',#14087,1000.);
#3182=VECTOR('',#14088,1000.);
#3183=VECTOR('',#14089,1000.);
#3184=VECTOR('',#14092,1000.);
#3185=VECTOR('',#14095,1000.);
#3186=VECTOR('',#14098,1000.);
#3187=VECTOR('',#14103,1000.);
#3188=VECTOR('',#14108,1000.);
#3189=VECTOR('',#14111,1000.);
#3190=VECTOR('',#14114,1000.);
#3191=VECTOR('',#14117,1000.);
#3192=VECTOR('',#14120,1000.);
#3193=VECTOR('',#14125,1000.);
#3194=VECTOR('',#14128,1000.);
#3195=VECTOR('',#14131,1000.);
#3196=VECTOR('',#14148,1000.);
#3197=VECTOR('',#14155,1000.);
#3198=VECTOR('',#14160,1000.);
#3199=VECTOR('',#14161,1000.);
#3200=VECTOR('',#14162,10.);
#3201=VECTOR('',#14165,1000.);
#3202=VECTOR('',#14166,1000.);
#3203=VECTOR('',#14167,10.);
#3204=VECTOR('',#14168,1000.);
#3205=VECTOR('',#14171,1000.);
#3206=VECTOR('',#14174,1000.);
#3207=VECTOR('',#14179,1000.);
#3208=VECTOR('',#14182,1000.);
#3209=VECTOR('',#14187,1000.);
#3210=VECTOR('',#14188,1000.);
#3211=VECTOR('',#14191,1000.);
#3212=VECTOR('',#14194,1000.);
#3213=VECTOR('',#14199,1000.);
#3214=VECTOR('',#14200,1000.);
#3215=VECTOR('',#14205,1000.);
#3216=VECTOR('',#14210,1000.);
#3217=VECTOR('',#14211,1000.);
#3218=VECTOR('',#14212,1000.);
#3219=VECTOR('',#14215,1000.);
#3220=VECTOR('',#14216,1000.);
#3221=VECTOR('',#14217,1000.);
#3222=VECTOR('',#14218,1000.);
#3223=VECTOR('',#14223,1000.);
#3224=VECTOR('',#14228,1000.);
#3225=VECTOR('',#14263,1000.);
#3226=VECTOR('',#14264,1000.);
#3227=VECTOR('',#14265,1000.);
#3228=VECTOR('',#14266,1000.);
#3229=VECTOR('',#14269,1000.);
#3230=VECTOR('',#14272,1000.);
#3231=VECTOR('',#14273,1000.);
#3232=VECTOR('',#14274,1000.);
#3233=VECTOR('',#14277,1000.);
#3234=VECTOR('',#14290,1000.);
#3235=VECTOR('',#14293,1000.);
#3236=VECTOR('',#14298,10.);
#3237=VECTOR('',#14301,10.);
#3238=VECTOR('',#14308,1000.);
#3239=VECTOR('',#14311,1000.);
#3240=VECTOR('',#14314,1000.);
#3241=VECTOR('',#14315,1000.);
#3242=VECTOR('',#14320,1000.);
#3243=VECTOR('',#14323,1000.);
#3244=VECTOR('',#14326,1000.);
#3245=VECTOR('',#14329,1000.);
#3246=VECTOR('',#14334,1000.);
#3247=VECTOR('',#14335,1000.);
#3248=VECTOR('',#14336,1000.);
#3249=VECTOR('',#14337,1000.);
#3250=VECTOR('',#14338,1000.);
#3251=VECTOR('',#14347,1000.);
#3252=VECTOR('',#14348,1000.);
#3253=VECTOR('',#14349,1000.);
#3254=VECTOR('',#14350,1000.);
#3255=VECTOR('',#14351,1000.);
#3256=VECTOR('',#14368,1000.);
#3257=VECTOR('',#14373,1000.);
#3258=VECTOR('',#14374,1000.);
#3259=VECTOR('',#14375,10.);
#3260=VECTOR('',#14376,1000.);
#3261=VECTOR('',#14379,1000.);
#3262=VECTOR('',#14380,10.);
#3263=VECTOR('',#14381,1000.);
#3264=VECTOR('',#14384,1000.);
#3265=VECTOR('',#14391,1000.);
#3266=VECTOR('',#14394,1000.);
#3267=VECTOR('',#14399,1000.);
#3268=VECTOR('',#14400,1000.);
#3269=VECTOR('',#14403,1000.);
#3270=VECTOR('',#14406,1000.);
#3271=VECTOR('',#14411,1000.);
#3272=VECTOR('',#14412,1000.);
#3273=VECTOR('',#14417,1000.);
#3274=VECTOR('',#14422,1000.);
#3275=VECTOR('',#14423,1000.);
#3276=VECTOR('',#14424,1000.);
#3277=VECTOR('',#14427,1000.);
#3278=VECTOR('',#14428,1000.);
#3279=VECTOR('',#14429,1000.);
#3280=VECTOR('',#14430,1000.);
#3281=VECTOR('',#14435,1000.);
#3282=VECTOR('',#14440,1000.);
#3283=VECTOR('',#14471,1000.);
#3284=VECTOR('',#14472,1000.);
#3285=VECTOR('',#14473,1000.);
#3286=VECTOR('',#14474,1000.);
#3287=VECTOR('',#14475,1000.);
#3288=VECTOR('',#14480,1000.);
#3289=VECTOR('',#14481,1000.);
#3290=VECTOR('',#14482,1000.);
#3291=VECTOR('',#14483,1000.);
#3292=VECTOR('',#14486,1000.);
#3293=VECTOR('',#14499,1000.);
#3294=VECTOR('',#14500,1000.);
#3295=VECTOR('',#14503,10.);
#3296=VECTOR('',#14504,10.);
#3297=VECTOR('',#14511,1000.);
#3298=VECTOR('',#14512,1000.);
#3299=VECTOR('',#14513,1000.);
#3300=VECTOR('',#14514,1000.);
#3301=VECTOR('',#14515,1000.);
#3302=VECTOR('',#14524,1000.);
#3303=VECTOR('',#14525,1000.);
#3304=VECTOR('',#14526,1000.);
#3305=VECTOR('',#14527,1000.);
#3306=VECTOR('',#14528,1000.);
#3307=VECTOR('',#14545,1000.);
#3308=VECTOR('',#14550,1000.);
#3309=VECTOR('',#14551,1000.);
#3310=VECTOR('',#14552,10.);
#3311=VECTOR('',#14553,1000.);
#3312=VECTOR('',#14556,1000.);
#3313=VECTOR('',#14557,1000.);
#3314=VECTOR('',#14558,10.);
#3315=VECTOR('',#14559,1000.);
#3316=VECTOR('',#14562,1000.);
#3317=VECTOR('',#14569,1000.);
#3318=VECTOR('',#14572,1000.);
#3319=VECTOR('',#14577,1000.);
#3320=VECTOR('',#14578,1000.);
#3321=VECTOR('',#14581,1000.);
#3322=VECTOR('',#14584,1000.);
#3323=VECTOR('',#14589,1000.);
#3324=VECTOR('',#14594,1000.);
#3325=VECTOR('',#14599,1000.);
#3326=VECTOR('',#14600,1000.);
#3327=VECTOR('',#14601,1000.);
#3328=VECTOR('',#14604,1000.);
#3329=VECTOR('',#14605,1000.);
#3330=VECTOR('',#14606,1000.);
#3331=VECTOR('',#14607,1000.);
#3332=VECTOR('',#14610,1000.);
#3333=VECTOR('',#14611,1000.);
#3334=VECTOR('',#14618,1000.);
#3335=VECTOR('',#14623,1000.);
#3336=VECTOR('',#14624,1000.);
#3337=VECTOR('',#14653,1000.);
#3338=VECTOR('',#14654,1000.);
#3339=VECTOR('',#14655,1000.);
#3340=VECTOR('',#14658,1000.);
#3341=VECTOR('',#14661,1000.);
#3342=VECTOR('',#14662,1000.);
#3343=VECTOR('',#14663,1000.);
#3344=VECTOR('',#14666,1000.);
#3345=VECTOR('',#14679,1000.);
#3346=VECTOR('',#14682,1000.);
#3347=VECTOR('',#14685,1000.);
#3348=VECTOR('',#14688,1000.);
#3349=VECTOR('',#14693,1000.);
#3350=VECTOR('',#14696,1000.);
#3351=VECTOR('',#14699,1000.);
#3352=VECTOR('',#14700,1000.);
#3353=VECTOR('',#14723,1000.);
#3354=VECTOR('',#14724,1000.);
#3355=VECTOR('',#14725,10.);
#3356=VECTOR('',#14726,1000.);
#3357=VECTOR('',#14729,1000.);
#3358=VECTOR('',#14730,1000.);
#3359=VECTOR('',#14731,10.);
#3360=VECTOR('',#14732,1000.);
#3361=VECTOR('',#14741,1000.);
#3362=VECTOR('',#14744,1000.);
#3363=VECTOR('',#14749,1000.);
#3364=VECTOR('',#14752,1000.);
#3365=VECTOR('',#14755,1000.);
#3366=VECTOR('',#14760,1000.);
#3367=VECTOR('',#14761,1000.);
#3368=VECTOR('',#14766,1000.);
#3369=VECTOR('',#14771,1000.);
#3370=VECTOR('',#14772,1000.);
#3371=VECTOR('',#14773,1000.);
#3372=VECTOR('',#14776,1000.);
#3373=VECTOR('',#14777,1000.);
#3374=VECTOR('',#14778,1000.);
#3375=VECTOR('',#14779,1000.);
#3376=VECTOR('',#14786,1000.);
#3377=VECTOR('',#14793,1000.);
#3378=VECTOR('',#16204,1000.);
#3379=VECTOR('',#16205,1000.);
#3380=VECTOR('',#16208,1000.);
#3381=VECTOR('',#16209,1000.);
#3382=VECTOR('',#16212,1000.);
#3383=VECTOR('',#16213,1000.);
#3384=VECTOR('',#16214,1000.);
#3385=VECTOR('',#16215,1000.);
#3386=VECTOR('',#16226,1000.);
#3387=VECTOR('',#16227,1000.);
#3388=VECTOR('',#16232,1000.);
#3389=VECTOR('',#16233,1000.);
#3390=VECTOR('',#16236,1000.);
#3391=VECTOR('',#16237,1000.);
#3392=VECTOR('',#16240,1000.);
#3393=VECTOR('',#16243,1000.);
#3394=VECTOR('',#16246,1000.);
#3395=VECTOR('',#16249,1000.);
#3396=VECTOR('',#16256,1000.);
#3397=VECTOR('',#16259,1000.);
#3398=VECTOR('',#16262,1000.);
#3399=VECTOR('',#16265,1000.);
#3400=VECTOR('',#16268,1000.);
#3401=VECTOR('',#16271,1000.);
#3413=CIRCLE('',#11525,2.1875);
#3414=CIRCLE('',#11526,2.1875);
#3415=CIRCLE('',#11528,2.5625);
#3416=CIRCLE('',#11529,2.5625);
#3417=CIRCLE('',#11531,3.4375);
#3418=CIRCLE('',#11532,3.4375);
#3419=CIRCLE('',#11534,1.3125);
#3420=CIRCLE('',#11535,1.3125);
#3421=CIRCLE('',#11537,2.8125);
#3422=CIRCLE('',#11538,2.8125);
#3423=CIRCLE('',#11539,0.3125);
#3424=CIRCLE('',#11540,3.125);
#3425=CIRCLE('',#11542,3.125);
#3426=CIRCLE('',#11543,0.3125);
#3427=CIRCLE('',#11544,2.8125);
#3428=CIRCLE('',#11545,2.8125);
#3429=CIRCLE('',#11547,3.125);
#3430=CIRCLE('',#11548,0.3125);
#3431=CIRCLE('',#11549,2.8125);
#3432=CIRCLE('',#11551,3.125);
#3433=CIRCLE('',#11552,0.3125);
#3434=CIRCLE('',#11553,2.8125);
#3435=CIRCLE('',#11554,2.8125);
#3436=CIRCLE('',#11556,0.625000000000001);
#3437=CIRCLE('',#11557,0.3125);
#3438=CIRCLE('',#11558,0.937500000000001);
#3439=CIRCLE('',#11559,0.312499999999997);
#3440=CIRCLE('',#11561,4.375);
#3441=CIRCLE('',#11562,0.312500000000001);
#3442=CIRCLE('',#11563,4.6875);
#3443=CIRCLE('',#11564,0.312500000000001);
#3444=CIRCLE('',#11566,1.25);
#3445=CIRCLE('',#11567,0.312499999999997);
#3446=CIRCLE('',#11568,0.937500000000001);
#3447=CIRCLE('',#11569,0.3125);
#3448=CIRCLE('',#11571,4.375);
#3449=CIRCLE('',#11572,0.312499999999997);
#3450=CIRCLE('',#11573,4.0625);
#3451=CIRCLE('',#11574,0.312500000000001);
#3452=CIRCLE('',#11576,2.8125);
#3453=CIRCLE('',#11577,2.8125);
#3454=CIRCLE('',#11578,0.3125);
#3455=CIRCLE('',#11579,3.125);
#3456=CIRCLE('',#11581,3.125);
#3457=CIRCLE('',#11582,0.3125);
#3458=CIRCLE('',#11583,2.8125);
#3459=CIRCLE('',#11584,2.8125);
#3460=CIRCLE('',#11586,3.125);
#3461=CIRCLE('',#11587,0.3125);
#3462=CIRCLE('',#11588,2.8125);
#3463=CIRCLE('',#11589,2.8125);
#3464=CIRCLE('',#11591,3.125);
#3465=CIRCLE('',#11592,0.3125);
#3466=CIRCLE('',#11593,2.8125);
#3467=CIRCLE('',#11594,2.8125);
#3468=CIRCLE('',#11596,0.625000000000001);
#3469=CIRCLE('',#11597,0.312499999999997);
#3470=CIRCLE('',#11598,0.937500000000001);
#3471=CIRCLE('',#11599,0.3125);
#3472=CIRCLE('',#11601,4.375);
#3473=CIRCLE('',#11602,0.312500000000001);
#3474=CIRCLE('',#11603,4.6875);
#3475=CIRCLE('',#11604,0.312500000000001);
#3476=CIRCLE('',#11606,1.25);
#3477=CIRCLE('',#11607,0.3125);
#3478=CIRCLE('',#11608,0.937500000000001);
#3479=CIRCLE('',#11609,0.312499999999997);
#3480=CIRCLE('',#11611,4.375);
#3481=CIRCLE('',#11612,0.312500000000001);
#3482=CIRCLE('',#11613,4.0625);
#3483=CIRCLE('',#11614,0.312500000000001);
#3484=CIRCLE('',#11616,2.8125);
#3485=CIRCLE('',#11617,0.3125);
#3486=CIRCLE('',#11618,3.125);
#3487=CIRCLE('',#11620,3.125);
#3488=CIRCLE('',#11621,0.3125);
#3489=CIRCLE('',#11622,2.8125);
#3490=CIRCLE('',#11624,3.125);
#3491=CIRCLE('',#11625,0.3125);
#3492=CIRCLE('',#11626,2.8125);
#3493=CIRCLE('',#11627,2.8125);
#3494=CIRCLE('',#11629,3.125);
#3495=CIRCLE('',#11630,0.3125);
#3496=CIRCLE('',#11631,2.8125);
#3497=CIRCLE('',#11633,0.625000000000001);
#3498=CIRCLE('',#11634,0.312500000000001);
#3499=CIRCLE('',#11635,0.937500000000001);
#3500=CIRCLE('',#11636,0.3125);
#3501=CIRCLE('',#11638,1.25);
#3502=CIRCLE('',#11639,0.3125);
#3503=CIRCLE('',#11640,0.937500000000001);
#3504=CIRCLE('',#11641,0.312500000000001);
#3505=CIRCLE('',#11643,2.8125);
#3506=CIRCLE('',#11644,0.3125);
#3507=CIRCLE('',#11645,3.125);
#3508=CIRCLE('',#11646,2.8125);
#3509=CIRCLE('',#11648,3.125);
#3510=CIRCLE('',#11649,0.3125);
#3511=CIRCLE('',#11650,2.8125);
#3512=CIRCLE('',#11651,2.8125);
#3513=CIRCLE('',#11653,3.125);
#3514=CIRCLE('',#11654,0.3125);
#3515=CIRCLE('',#11655,2.8125);
#3516=CIRCLE('',#11656,2.8125);
#3517=CIRCLE('',#11658,3.125);
#3518=CIRCLE('',#11659,0.3125);
#3519=CIRCLE('',#11660,2.8125);
#3520=CIRCLE('',#11661,2.8125);
#3521=CIRCLE('',#11663,49.6875);
#3522=CIRCLE('',#11664,0.312499999999998);
#3523=CIRCLE('',#11665,49.7790291308792);
#3524=CIRCLE('',#11666,0.312500000000003);
#3525=CIRCLE('',#11668,49.7790291308792);
#3526=CIRCLE('',#11669,0.312499999999998);
#3527=CIRCLE('',#11670,49.6875);
#3528=CIRCLE('',#11671,0.312499999999998);
#3529=CIRCLE('',#11673,1.25);
#3530=CIRCLE('',#11674,0.312500000000001);
#3531=CIRCLE('',#11675,0.937500000000001);
#3532=CIRCLE('',#11676,0.312500000000001);
#3533=CIRCLE('',#11678,1.25);
#3534=CIRCLE('',#11679,0.312500000000001);
#3535=CIRCLE('',#11680,0.937500000000001);
#3536=CIRCLE('',#11681,0.312500000000001);
#3537=CIRCLE('',#11683,1.25);
#3538=CIRCLE('',#11684,0.312500000000001);
#3539=CIRCLE('',#11685,0.937500000000001);
#3540=CIRCLE('',#11686,0.312500000000001);
#3541=CIRCLE('',#11688,1.25);
#3542=CIRCLE('',#11689,0.312500000000001);
#3543=CIRCLE('',#11690,0.937500000000001);
#3544=CIRCLE('',#11691,0.312499999999996);
#3545=CIRCLE('',#11693,0.3125);
#3546=CIRCLE('',#11694,0.3125);
#3547=CIRCLE('',#11696,0.3125);
#3548=CIRCLE('',#11697,0.3125);
#3549=CIRCLE('',#11699,0.3125);
#3550=CIRCLE('',#11700,0.3125);
#3551=CIRCLE('',#11702,0.3125);
#3552=CIRCLE('',#11703,0.625000000000001);
#3553=CIRCLE('',#11704,0.3125);
#3554=CIRCLE('',#11706,0.3125);
#3555=CIRCLE('',#11707,0.3125);
#3556=CIRCLE('',#11709,0.3125);
#3557=CIRCLE('',#11710,0.3125);
#3558=CIRCLE('',#11712,0.3125);
#3559=CIRCLE('',#11713,0.3125);
#3560=CIRCLE('',#11715,0.3125);
#3561=CIRCLE('',#11716,0.3125);
#3562=CIRCLE('',#11718,0.3125);
#3563=CIRCLE('',#11719,0.312499999999999);
#3564=CIRCLE('',#11720,0.625000000000001);
#3565=CIRCLE('',#11721,0.312500000000001);
#3566=CIRCLE('',#11723,0.625000000000001);
#3567=CIRCLE('',#11724,0.3125);
#3568=CIRCLE('',#11725,0.937500000000001);
#3569=CIRCLE('',#11726,0.312500000000001);
#3570=CIRCLE('',#11728,1.25);
#3571=CIRCLE('',#11729,0.312500000000001);
#3572=CIRCLE('',#11730,0.937500000000001);
#3573=CIRCLE('',#11731,0.3125);
#3574=CIRCLE('',#11733,0.937500000000001);
#3575=CIRCLE('',#11734,0.937500000000001);
#3576=CIRCLE('',#11736,4.375);
#3577=CIRCLE('',#11737,4.375);
#3578=CIRCLE('',#11741,0.937500000000001);
#3579=CIRCLE('',#11743,0.937500000000001);
#3580=CIRCLE('',#11744,0.937500000000001);
#3581=CIRCLE('',#11746,4.375);
#3582=CIRCLE('',#11747,4.375);
#3583=CIRCLE('',#11751,54.4084708691208);
#3584=CIRCLE('',#11752,54.4084708691208);
#3585=CIRCLE('',#11754,0.937500000000001);
#3586=CIRCLE('',#11756,0.937500000000001);
#3587=CIRCLE('',#11757,0.937500000000001);
#3588=CIRCLE('',#11762,49.7790291308792);
#3589=CIRCLE('',#11763,54.4084708691208);
#3590=CIRCLE('',#11764,54.4084708691208);
#3591=CIRCLE('',#11766,0.937500000000001);
#3592=CIRCLE('',#11770,48.4374999999919);
#3593=CIRCLE('',#11771,48.4375);
#3594=CIRCLE('',#11772,48.4374999999962);
#3595=CIRCLE('',#11773,48.4374999999878);
#3596=CIRCLE('',#11774,48.4375);
#3597=CIRCLE('',#11775,48.4374999999957);
#3598=CIRCLE('',#11776,48.4375000000006);
#3599=CIRCLE('',#11777,48.4375);
#3600=CIRCLE('',#11778,48.4375);
#3601=CIRCLE('',#11779,48.4375);
#3602=CIRCLE('',#11780,48.4375);
#3603=CIRCLE('',#11781,48.4375);
#3604=CIRCLE('',#11782,48.4374999999921);
#3605=CIRCLE('',#11783,48.4375000000018);
#3606=CIRCLE('',#11784,48.4375);
#3607=CIRCLE('',#11785,48.4375);
#3608=CIRCLE('',#11786,48.4375);
#3609=CIRCLE('',#11787,48.4375);
#3610=CIRCLE('',#11788,48.4375);
#3611=CIRCLE('',#11789,48.4374999999846);
#3612=CIRCLE('',#11790,48.4375000000085);
#3613=CIRCLE('',#11791,48.4375);
#3614=CIRCLE('',#11792,48.4375);
#3615=CIRCLE('',#11793,48.4375);
#3616=CIRCLE('',#11794,48.4375);
#3617=CIRCLE('',#11795,48.4375);
#3618=CIRCLE('',#11796,48.4374999999955);
#3619=CIRCLE('',#11797,48.4374999999898);
#3620=CIRCLE('',#11798,48.4375);
#3621=CIRCLE('',#11799,48.4375);
#3622=CIRCLE('',#11800,48.4375);
#3623=CIRCLE('',#11801,48.4375);
#3624=CIRCLE('',#11802,48.4375);
#3625=CIRCLE('',#11803,48.4375000000021);
#3626=CIRCLE('',#11804,48.4375000000048);
#3627=CIRCLE('',#11805,48.4375);
#3628=CIRCLE('',#11806,48.4375000000005);
#3629=CIRCLE('',#11807,48.4374999999868);
#3630=CIRCLE('',#11808,48.4375);
#3631=CIRCLE('',#11809,48.4375000000012);
#3632=CIRCLE('',#11813,49.7790291308792);
#3633=CIRCLE('',#11814,54.4084708691208);
#3634=CIRCLE('',#11815,54.4084708691208);
#3635=CIRCLE('',#11817,0.937500000000001);
#3636=CIRCLE('',#11819,1.25);
#3637=CIRCLE('',#11820,1.25);
#3638=CIRCLE('',#11822,4.0625);
#3639=CIRCLE('',#11823,1.25);
#3640=CIRCLE('',#11824,1.25);
#3641=CIRCLE('',#11825,54.6875);
#3642=CIRCLE('',#11826,1.25);
#3643=CIRCLE('',#11827,5.3125);
#3644=CIRCLE('',#11828,5.3125);
#3645=CIRCLE('',#11829,5.3125);
#3646=CIRCLE('',#11830,5.3125);
#3647=CIRCLE('',#11831,54.6875);
#3648=CIRCLE('',#11832,1.25);
#3649=CIRCLE('',#11833,1.25);
#3650=CIRCLE('',#11834,4.0625);
#3651=CIRCLE('',#11835,1.25);
#3652=CIRCLE('',#11836,54.6875);
#3653=CIRCLE('',#11837,1.25);
#3654=CIRCLE('',#11838,1.25);
#3655=CIRCLE('',#11839,1.25);
#3656=CIRCLE('',#11840,54.6875);
#3657=CIRCLE('',#11841,1.25);
#3658=CIRCLE('',#11842,1.25);
#3659=CIRCLE('',#11843,1.25);
#3660=CIRCLE('',#11844,53.5669417382416);
#3661=CIRCLE('',#11845,53.5669417382416);
#3662=CIRCLE('',#11846,53.5669417382416);
#3663=CIRCLE('',#11847,53.5669417382416);
#3664=CIRCLE('',#11851,54.6294417382416);
#3665=CIRCLE('',#11852,1.25);
#3666=CIRCLE('',#11853,54.6294417382416);
#3667=CIRCLE('',#11854,5.3125);
#3668=CIRCLE('',#11856,5.3125);
#3669=CIRCLE('',#11857,50.8794417382416);
#3670=CIRCLE('',#11858,50.8794417382416);
#3671=CIRCLE('',#11861,0.3125);
#3672=CIRCLE('',#11862,0.3125);
#3673=CIRCLE('',#11864,0.3125);
#3674=CIRCLE('',#11865,0.3125);
#3675=CIRCLE('',#11867,0.3125);
#3676=CIRCLE('',#11868,0.3125);
#3677=CIRCLE('',#11870,0.3125);
#3678=CIRCLE('',#11871,0.3125);
#3679=CIRCLE('',#11873,0.3125);
#3680=CIRCLE('',#11875,0.3125);
#3681=CIRCLE('',#11878,0.312499999999999);
#3682=CIRCLE('',#11879,0.312499999999999);
#3683=CIRCLE('',#11881,0.312499999999999);
#3684=CIRCLE('',#11882,0.3125);
#3685=CIRCLE('',#11884,1.25);
#3686=CIRCLE('',#11885,20.);
#3687=CIRCLE('',#11899,55.7165291308792);
#3688=CIRCLE('',#11901,48.5290291308792);
#3689=CIRCLE('',#11902,57.0959708691208);
#3690=CIRCLE('',#11903,1927.031520572);
#3691=CIRCLE('',#11905,0.625000000000001);
#3692=CIRCLE('',#11906,21.5625);
#3693=CIRCLE('',#11907,48.125);
#3694=CIRCLE('',#11908,0.625000000000001);
#3695=CIRCLE('',#11909,21.5625);
#3696=CIRCLE('',#11910,48.125);
#3697=CIRCLE('',#11911,0.625000000000001);
#3698=CIRCLE('',#11912,21.5625);
#3699=CIRCLE('',#11913,48.125);
#3700=CIRCLE('',#11914,21.5625);
#3701=CIRCLE('',#11915,48.125);
#3702=CIRCLE('',#11916,20.);
#3703=CIRCLE('',#11917,1.25);
#3704=CIRCLE('',#11919,1924.96574975015);
#3705=CIRCLE('',#11921,890.503059959066);
#3706=CIRCLE('',#11923,48.5290291308792);
#3707=CIRCLE('',#11924,55.7165291308792);
#3708=CIRCLE('',#11925,893.129292938247);
#3709=CIRCLE('',#11926,57.0959708691208);
#3710=CIRCLE('',#11928,49.7790291308792);
#3711=CIRCLE('',#11929,54.4084708691208);
#3712=CIRCLE('',#11930,54.4084708691208);
#3713=CIRCLE('',#11932,49.6875);
#3714=CIRCLE('',#11933,49.6875);
#3715=CIRCLE('',#11935,49.6875);
#3716=CIRCLE('',#11936,49.6875);
#3717=CIRCLE('',#11938,49.7790291308792);
#3718=CIRCLE('',#11939,50.6584708691208);
#3719=CIRCLE('',#11940,50.6584708691208);
#3720=CIRCLE('',#11942,49.7790291308792);
#3721=CIRCLE('',#11943,50.6584708691208);
#3722=CIRCLE('',#11944,50.6584708691208);
#3723=CIRCLE('',#11946,5.3125);
#3724=CIRCLE('',#11947,54.6294417382416);
#3725=CIRCLE('',#11948,54.6294417382416);
#3726=CIRCLE('',#11950,5.3125);
#3727=CIRCLE('',#11951,50.8794417382416);
#3728=CIRCLE('',#11952,1.25);
#3729=CIRCLE('',#11953,50.8794417382416);
#3730=CIRCLE('',#11957,5.625);
#3731=CIRCLE('',#11958,5.625);
#3732=CIRCLE('',#11962,57.3169417382416);
#3733=CIRCLE('',#11963,57.3169417382416);
#3734=CIRCLE('',#11964,21.5625);
#3735=CIRCLE('',#11965,0.625000000000001);
#3736=CIRCLE('',#11966,5.3125);
#3737=CIRCLE('',#11967,5.3125);
#3738=CIRCLE('',#11968,5.3125);
#3739=CIRCLE('',#11969,5.3125);
#3740=CIRCLE('',#11970,57.3169417382416);
#3741=CIRCLE('',#11971,21.5625);
#3742=CIRCLE('',#11972,0.625000000000001);
#3743=CIRCLE('',#11973,57.3169417382416);
#3744=CIRCLE('',#11974,57.3169417382416);
#3745=CIRCLE('',#11975,21.5625);
#3746=CIRCLE('',#11976,57.3169417382416);
#3747=CIRCLE('',#11977,21.5625);
#3748=CIRCLE('',#11978,0.625000000000001);
#3749=CIRCLE('',#11979,57.3169417382416);
#3750=CIRCLE('',#11980,57.3169417382416);
#3751=CIRCLE('',#11982,5.625);
#3752=CIRCLE('',#11983,5.625);
#3753=CIRCLE('',#11985,48.5290291308792);
#3754=CIRCLE('',#11986,53.3459708691208);
#3755=CIRCLE('',#11996,21.875);
#3756=CIRCLE('',#11997,21.875);
#3757=CIRCLE('',#11999,55.4955582617584);
#3758=CIRCLE('',#12000,48.75);
#3759=CIRCLE('',#12003,55.4955582617584);
#3760=CIRCLE('',#12004,48.75);
#3761=CIRCLE('',#12007,55.);
#3762=CIRCLE('',#12008,55.);
#3763=CIRCLE('',#12012,0.625000000000001);
#3764=CIRCLE('',#12013,55.3125);
#3765=CIRCLE('',#12014,0.625000000000001);
#3766=CIRCLE('',#12015,0.625000000000001);
#3767=CIRCLE('',#12017,0.937500000000001);
#3768=CIRCLE('',#12018,0.937500000000001);
#3769=CIRCLE('',#12020,0.937500000000001);
#3770=CIRCLE('',#12021,0.937500000000001);
#3771=CIRCLE('',#12023,0.937500000000001);
#3772=CIRCLE('',#12024,0.937500000000001);
#3773=CIRCLE('',#12026,55.7165291308792);
#3774=CIRCLE('',#12028,48.5290291308792);
#3775=CIRCLE('',#12029,57.0959708691208);
#3776=CIRCLE('',#12030,1927.03152059917);
#3777=CIRCLE('',#12032,1924.96575403414);
#3778=CIRCLE('',#12034,890.503063305381);
#3779=CIRCLE('',#12036,48.5290291308792);
#3780=CIRCLE('',#12037,55.7165291308792);
#3781=CIRCLE('',#12038,893.129293181156);
#3782=CIRCLE('',#12039,57.0959708691208);
#3783=CIRCLE('',#12041,49.6875);
#3784=CIRCLE('',#12042,49.6875);
#3785=CIRCLE('',#12044,49.7790291308792);
#3786=CIRCLE('',#12045,50.6584708691208);
#3787=CIRCLE('',#12046,50.6584708691208);
#3788=CIRCLE('',#12048,5.3125);
#3789=CIRCLE('',#12049,54.6294417382416);
#3790=CIRCLE('',#12050,54.6294417382416);
#3791=CIRCLE('',#12052,5.3125);
#3792=CIRCLE('',#12053,50.8794417382416);
#3793=CIRCLE('',#12054,1.25);
#3794=CIRCLE('',#12055,50.8794417382416);
#3795=CIRCLE('',#12058,5.625);
#3796=CIRCLE('',#12059,5.625);
#3797=CIRCLE('',#12062,5.625);
#3798=CIRCLE('',#12063,5.625);
#3799=CIRCLE('',#12065,48.5290291308792);
#3800=CIRCLE('',#12066,53.3459708691208);
#3801=CIRCLE('',#12073,21.875);
#3802=CIRCLE('',#12074,21.875);
#3803=CIRCLE('',#12076,55.4955582617584);
#3804=CIRCLE('',#12077,48.75);
#3805=CIRCLE('',#12080,55.4955582617584);
#3806=CIRCLE('',#12081,48.75);
#3807=CIRCLE('',#12084,55.);
#3808=CIRCLE('',#12085,55.);
#3809=CIRCLE('',#12089,0.625000000000001);
#3810=CIRCLE('',#12090,0.625000000000001);
#3811=CIRCLE('',#12091,55.3125);
#3812=CIRCLE('',#12092,0.625000000000001);
#3813=CIRCLE('',#12095,0.937500000000001);
#3814=CIRCLE('',#12096,0.937500000000001);
#3815=CIRCLE('',#12098,0.937500000000001);
#3816=CIRCLE('',#12099,0.937500000000001);
#3817=CIRCLE('',#12101,55.7165291308792);
#3818=CIRCLE('',#12103,48.5290291308792);
#3819=CIRCLE('',#12104,57.0959708691208);
#3820=CIRCLE('',#12105,1927.031520572);
#3821=CIRCLE('',#12107,1924.96571317355);
#3822=CIRCLE('',#12109,890.503061246252);
#3823=CIRCLE('',#12111,48.5290291308792);
#3824=CIRCLE('',#12112,55.7165291308792);
#3825=CIRCLE('',#12113,893.129292782135);
#3826=CIRCLE('',#12114,57.0959708691208);
#3827=CIRCLE('',#12117,50.6584708691208);
#3828=CIRCLE('',#12118,50.6584708691208);
#3829=CIRCLE('',#12121,5.625);
#3830=CIRCLE('',#12122,5.625);
#3831=CIRCLE('',#12125,5.625);
#3832=CIRCLE('',#12126,5.625);
#3833=CIRCLE('',#12128,48.5290291308792);
#3834=CIRCLE('',#12129,53.3459708691208);
#3835=CIRCLE('',#12136,21.875);
#3836=CIRCLE('',#12137,21.875);
#3837=CIRCLE('',#12139,55.4955582617584);
#3838=CIRCLE('',#12140,48.75);
#3839=CIRCLE('',#12143,55.4955582617584);
#3840=CIRCLE('',#12144,48.75);
#3841=CIRCLE('',#12147,55.);
#3842=CIRCLE('',#12148,55.);
#3843=CIRCLE('',#12152,0.625000000000001);
#3844=CIRCLE('',#12153,55.3125);
#3845=CIRCLE('',#12154,0.625000000000001);
#3846=CIRCLE('',#12155,0.625000000000001);
#3847=CIRCLE('',#12156,4.6875);
#3848=CIRCLE('',#12158,0.937500000000001);
#3849=CIRCLE('',#12159,0.937500000000001);
#3850=CIRCLE('',#12162,0.937500000000001);
#3851=CIRCLE('',#12163,0.937500000000001);
#3852=CIRCLE('',#12165,55.7165291308792);
#3853=CIRCLE('',#12167,48.5290291308792);
#3854=CIRCLE('',#12168,57.0959708691208);
#3855=CIRCLE('',#12169,1927.03152058192);
#3856=CIRCLE('',#12171,1924.9657347274);
#3857=CIRCLE('',#12173,890.503062314187);
#3858=CIRCLE('',#12175,48.5290291308792);
#3859=CIRCLE('',#12176,55.7165291308792);
#3860=CIRCLE('',#12177,893.129296310679);
#3861=CIRCLE('',#12178,57.0959708691208);
#3862=CIRCLE('',#12180,5.3125);
#3863=CIRCLE('',#12181,54.6294417382416);
#3864=CIRCLE('',#12182,1.25);
#3865=CIRCLE('',#12183,54.6294417382416);
#3866=CIRCLE('',#12185,5.3125);
#3867=CIRCLE('',#12186,50.8794417382416);
#3868=CIRCLE('',#12187,50.8794417382416);
#3869=CIRCLE('',#12189,5.625);
#3870=CIRCLE('',#12190,5.625);
#3871=CIRCLE('',#12192,5.625);
#3872=CIRCLE('',#12193,5.625);
#3873=CIRCLE('',#12195,48.5290291308792);
#3874=CIRCLE('',#12196,53.3459708691208);
#3875=CIRCLE('',#12200,21.875);
#3876=CIRCLE('',#12201,21.875);
#3877=CIRCLE('',#12203,55.4955582617584);
#3878=CIRCLE('',#12204,48.75);
#3879=CIRCLE('',#12207,55.4955582617584);
#3880=CIRCLE('',#12208,48.75);
#3881=CIRCLE('',#12211,55.);
#3882=CIRCLE('',#12212,55.);
#3883=CIRCLE('',#12216,4.6875);
#3884=CIRCLE('',#12217,0.625000000000001);
#3885=CIRCLE('',#12218,0.625000000000001);
#3886=CIRCLE('',#12219,55.3125);
#3887=CIRCLE('',#12220,0.625000000000001);
#3888=CIRCLE('',#12222,0.937500000000001);
#3889=CIRCLE('',#12223,0.937500000000001);
#3890=CIRCLE('',#12225,0.937500000000001);
#3891=CIRCLE('',#12226,0.937500000000001);
#3892=CIRCLE('',#12229,0.3125);
#3893=CIRCLE('',#12231,0.3125);
#3894=CIRCLE('',#12233,0.3125);
#3895=CIRCLE('',#12235,0.3125);
#3896=CIRCLE('',#12237,0.312499999999999);
#3897=CIRCLE('',#12239,0.312499999999997);
#3898=CIRCLE('',#12242,0.3125);
#3899=CIRCLE('',#12244,0.3125);
#3900=CIRCLE('',#12246,0.3125);
#3901=CIRCLE('',#12248,0.3125);
#3902=CIRCLE('',#12250,0.312499999999999);
#3903=CIRCLE('',#12252,0.312499999999997);
#3904=CIRCLE('',#12254,0.313663740331856);
#3905=CIRCLE('',#12255,0.313663740332209);
#3906=CIRCLE('',#12256,0.3125);
#3907=CIRCLE('',#12257,0.312500000000002);
#3908=CIRCLE('',#12258,0.312500000000002);
#3909=CIRCLE('',#12259,0.3125);
#3910=CIRCLE('',#12261,0.312499999999997);
#3911=CIRCLE('',#12263,0.312499999999999);
#3912=CIRCLE('',#12265,0.3125);
#3913=CIRCLE('',#12268,0.3125);
#3914=CIRCLE('',#12269,0.3125);
#3915=CIRCLE('',#12270,0.312500000000003);
#3916=CIRCLE('',#12272,0.312500000000002);
#3917=CIRCLE('',#12273,0.312500000000001);
#3918=CIRCLE('',#12274,0.312499999999996);
#3919=CIRCLE('',#12275,0.312499999999999);
#3920=CIRCLE('',#12277,0.312500000000002);
#3921=CIRCLE('',#12278,0.312500000000003);
#3922=CIRCLE('',#12280,0.312499999999998);
#3923=CIRCLE('',#12282,0.312499999999999);
#3924=CIRCLE('',#12285,0.3125);
#3925=CIRCLE('',#12286,0.3125);
#3926=CIRCLE('',#12288,0.3125);
#3927=CIRCLE('',#12290,0.312499999999999);
#3928=CIRCLE('',#12291,0.312499999999999);
#3929=CIRCLE('',#12293,0.312499999999999);
#3930=CIRCLE('',#12294,0.312499999999999);
#3931=CIRCLE('',#12296,0.312500000000001);
#3932=CIRCLE('',#12298,0.312499999999998);
#3933=CIRCLE('',#12299,0.312500000000002);
#3934=CIRCLE('',#12300,0.312500000000002);
#3935=CIRCLE('',#12301,0.3125);
#3936=CIRCLE('',#12303,0.312499999999997);
#3937=CIRCLE('',#12305,0.312500000000002);
#3938=CIRCLE('',#12306,0.312500000000002);
#3939=CIRCLE('',#12307,0.3125);
#3940=CIRCLE('',#12308,0.3125);
#3941=CIRCLE('',#12310,0.3125);
#3942=CIRCLE('',#12312,0.3125);
#3943=CIRCLE('',#12313,0.312499999999996);
#3944=CIRCLE('',#12317,0.3125);
#3945=CIRCLE('',#12320,0.312500000000002);
#3946=CIRCLE('',#12322,0.3125);
#3947=CIRCLE('',#12323,0.312500000000003);
#3948=CIRCLE('',#12324,0.313663740332281);
#3949=CIRCLE('',#12326,0.3125);
#3950=CIRCLE('',#12328,0.312500000000002);
#3951=CIRCLE('',#12330,0.312499999999999);
#3952=CIRCLE('',#12331,0.312500000000002);
#3953=CIRCLE('',#12332,0.312500000000001);
#3954=CIRCLE('',#12333,0.312500000000002);
#3955=CIRCLE('',#12335,0.312499999999998);
#3956=CIRCLE('',#12336,0.3125);
#3957=CIRCLE('',#12337,0.3125);
#3958=CIRCLE('',#12339,0.312500000000002);
#3959=CIRCLE('',#12341,0.312499999999997);
#3960=CIRCLE('',#12343,0.312500000000002);
#3961=CIRCLE('',#12345,0.3125);
#3962=CIRCLE('',#12347,0.312499999999999);
#3963=CIRCLE('',#12349,0.312499999999997);
#3964=CIRCLE('',#12351,0.312499999999999);
#3965=CIRCLE('',#12352,0.312500000000002);
#3966=CIRCLE('',#12353,0.312500000000002);
#3967=CIRCLE('',#12354,0.312500000000002);
#3968=CIRCLE('',#12355,0.312500000000002);
#3969=CIRCLE('',#12356,0.3125);
#3970=CIRCLE('',#12358,0.312499999999999);
#3971=CIRCLE('',#12360,0.312499999999999);
#3972=CIRCLE('',#12362,0.3125);
#3973=CIRCLE('',#12365,0.312500000000002);
#3974=CIRCLE('',#12367,0.3125);
#3975=CIRCLE('',#12369,0.312500000000001);
#3976=CIRCLE('',#12371,0.312499999999999);
#3977=CIRCLE('',#12372,0.312500000000003);
#3978=CIRCLE('',#12374,0.312500000000001);
#3979=CIRCLE('',#12376,0.312499999999999);
#3980=CIRCLE('',#12379,0.3125);
#3981=CIRCLE('',#12380,0.3125);
#3982=CIRCLE('',#12381,0.312500000000003);
#3983=CIRCLE('',#12383,0.312500000000002);
#3984=CIRCLE('',#12384,0.312500000000001);
#3985=CIRCLE('',#12386,0.3125);
#3986=CIRCLE('',#12387,0.3125);
#3987=CIRCLE('',#12389,0.312499999999999);
#3988=CIRCLE('',#12391,0.312499999999999);
#3989=CIRCLE('',#12393,0.3125);
#3990=CIRCLE('',#12395,0.312500000000002);
#3991=CIRCLE('',#12397,0.3125);
#3992=CIRCLE('',#12398,0.312500000000003);
#3993=CIRCLE('',#12400,0.312499999999998);
#3994=CIRCLE('',#12402,0.312499999999999);
#3995=CIRCLE('',#12405,0.3125);
#3996=CIRCLE('',#12408,0.312500000000001);
#3997=CIRCLE('',#12410,0.3125);
#3998=CIRCLE('',#12412,0.312499999999999);
#3999=CIRCLE('',#12415,0.312499999999999);
#4000=CIRCLE('',#12416,0.312500000000002);
#4001=CIRCLE('',#12418,0.3125);
#4002=CIRCLE('',#12420,0.312499999999999);
#4003=CIRCLE('',#12421,0.312500000000002);
#4004=CIRCLE('',#12422,0.312500000000002);
#4005=CIRCLE('',#12423,0.312499999999997);
#4006=CIRCLE('',#12425,0.3125);
#4007=CIRCLE('',#12426,0.312500000000001);
#4008=CIRCLE('',#12428,0.312500000000001);
#4009=CIRCLE('',#12430,0.312499999999999);
#4010=CIRCLE('',#12432,0.312500000000002);
#4011=CIRCLE('',#12434,0.312499999999999);
#4012=CIRCLE('',#12436,0.3125);
#4013=CIRCLE('',#12438,0.312500000000002);
#4014=CIRCLE('',#12440,0.312499999999999);
#4015=CIRCLE('',#12441,0.312500000000002);
#4016=CIRCLE('',#12443,0.3125);
#4017=CIRCLE('',#12444,0.312500000000002);
#4018=CIRCLE('',#12446,0.312500000000002);
#4019=CIRCLE('',#12448,0.312500000000002);
#4020=CIRCLE('',#12450,0.3125);
#4021=CIRCLE('',#12452,0.3125);
#4022=CIRCLE('',#12454,0.312499999999997);
#4023=CIRCLE('',#12456,0.3125);
#4024=CIRCLE('',#12457,0.3125);
#4025=CIRCLE('',#12459,0.312500000000002);
#4026=CIRCLE('',#12460,0.312500000000002);
#4027=CIRCLE('',#12463,0.312499999999997);
#4028=CIRCLE('',#12465,0.312500000000001);
#4029=CIRCLE('',#12467,0.312499999999999);
#4030=CIRCLE('',#12468,0.312499999999999);
#4031=CIRCLE('',#12470,0.312499999999996);
#4032=CIRCLE('',#12472,0.312500000000002);
#4033=CIRCLE('',#12474,0.312499999999997);
#4034=CIRCLE('',#12475,0.3125);
#4035=CIRCLE('',#12477,0.3125);
#4036=CIRCLE('',#12479,0.312499999999999);
#4037=CIRCLE('',#12480,0.312499999999999);
#4038=CIRCLE('',#12482,0.3125);
#4039=CIRCLE('',#12484,0.3125);
#4040=CIRCLE('',#12487,0.312500000000002);
#4041=CIRCLE('',#12488,0.312500000000001);
#4042=CIRCLE('',#12490,0.312500000000003);
#4043=CIRCLE('',#12492,0.3125);
#4044=CIRCLE('',#12493,0.312499999999997);
#4045=CIRCLE('',#12495,0.312499999999999);
#4046=CIRCLE('',#12496,0.3125);
#4047=CIRCLE('',#12497,0.312499999999999);
#4048=CIRCLE('',#12499,0.312500000000001);
#4049=CIRCLE('',#12502,0.3125);
#4050=CIRCLE('',#12504,0.3125);
#4051=CIRCLE('',#12506,0.3125);
#4052=CIRCLE('',#12508,0.3125);
#4053=CIRCLE('',#12509,0.312500000000003);
#4054=CIRCLE('',#12510,0.313663740331845);
#4055=CIRCLE('',#12512,0.3125);
#4056=CIRCLE('',#12514,0.312500000000002);
#4057=CIRCLE('',#12516,0.312499999999998);
#4058=CIRCLE('',#12518,0.312499999999998);
#4059=CIRCLE('',#12520,0.3125);
#4060=CIRCLE('',#12521,0.3125);
#4061=CIRCLE('',#12523,0.312500000000002);
#4062=CIRCLE('',#12524,0.312500000000001);
#4063=CIRCLE('',#12526,0.312499999999999);
#4064=CIRCLE('',#12528,0.312500000000002);
#4065=CIRCLE('',#12529,0.312499999999999);
#4066=CIRCLE('',#12530,0.312500000000001);
#4067=CIRCLE('',#12533,0.312499999999997);
#4068=CIRCLE('',#12534,0.312500000000002);
#4069=CIRCLE('',#12537,0.312500000000003);
#4070=CIRCLE('',#12538,0.312499999999999);
#4071=CIRCLE('',#12540,0.312500000000003);
#4072=CIRCLE('',#12542,0.312499999999996);
#4073=CIRCLE('',#12543,0.312499999999999);
#4074=CIRCLE('',#12545,0.312499999999998);
#4075=CIRCLE('',#12548,0.312500000000001);
#4076=CIRCLE('',#12550,0.312500000000003);
#4077=CIRCLE('',#12551,0.3125);
#4078=CIRCLE('',#12553,0.312500000000003);
#4079=CIRCLE('',#12554,0.3125);
#4080=CIRCLE('',#12555,0.3125);
#4081=CIRCLE('',#12557,0.312500000000001);
#4082=CIRCLE('',#12558,0.312499999999999);
#4083=CIRCLE('',#12560,0.312500000000003);
#4084=CIRCLE('',#12562,0.312500000000002);
#4085=CIRCLE('',#12564,0.312500000000004);
#4086=CIRCLE('',#12565,0.3125);
#4087=CIRCLE('',#12567,0.3125);
#4088=CIRCLE('',#12569,0.312500000000001);
#4089=CIRCLE('',#12571,0.3125);
#4090=CIRCLE('',#12572,0.312500000000001);
#4091=CIRCLE('',#12574,0.312500000000003);
#4092=CIRCLE('',#12576,0.312500000000001);
#4093=CIRCLE('',#12577,0.3125);
#4094=CIRCLE('',#12579,0.3125);
#4095=CIRCLE('',#12581,0.312499999999997);
#4096=CIRCLE('',#12582,0.312499999999999);
#4097=CIRCLE('',#12585,0.312499999999998);
#4098=CIRCLE('',#12587,0.312500000000001);
#4099=CIRCLE('',#12589,0.3125);
#4100=CIRCLE('',#12591,0.3125);
#4101=CIRCLE('',#12594,0.312499999999998);
#4102=CIRCLE('',#12595,0.3125);
#4103=CIRCLE('',#12596,0.3125);
#4104=CIRCLE('',#12598,0.312500000000001);
#4105=CIRCLE('',#12599,0.3125);
#4106=CIRCLE('',#12601,0.312499999999996);
#4107=CIRCLE('',#12603,0.3125);
#4108=CIRCLE('',#12604,0.3125);
#4109=CIRCLE('',#12606,0.3125);
#4110=CIRCLE('',#12607,0.312500000000003);
#4111=CIRCLE('',#12609,0.312500000000001);
#4112=CIRCLE('',#12611,0.3125);
#4113=CIRCLE('',#12612,0.3125);
#4114=CIRCLE('',#12616,0.312500000000001);
#4115=CIRCLE('',#12618,0.312499999999999);
#4116=CIRCLE('',#12620,0.3125);
#4117=CIRCLE('',#12621,0.3125);
#4118=CIRCLE('',#12623,0.312500000000003);
#4119=CIRCLE('',#12625,0.3125);
#4120=CIRCLE('',#12626,0.312500000000002);
#4121=CIRCLE('',#12627,0.312500000000001);
#4122=CIRCLE('',#12629,0.3125);
#4123=CIRCLE('',#12631,0.3125);
#4124=CIRCLE('',#12632,0.3125);
#4125=CIRCLE('',#12634,0.312500000000002);
#4126=CIRCLE('',#12635,0.3125);
#4127=CIRCLE('',#12636,0.3125);
#4128=CIRCLE('',#12638,0.3125);
#4129=CIRCLE('',#12639,0.312500000000003);
#4130=CIRCLE('',#12641,0.312499999999998);
#4131=CIRCLE('',#12644,0.3125);
#4132=CIRCLE('',#12646,0.3125);
#4133=CIRCLE('',#12648,0.312500000000001);
#4134=CIRCLE('',#12650,0.312500000000003);
#4135=CIRCLE('',#12651,0.3125);
#4136=CIRCLE('',#12653,0.3125);
#4137=CIRCLE('',#12655,0.312499999999999);
#4138=CIRCLE('',#12657,0.312500000000002);
#4139=CIRCLE('',#12659,0.3125);
#4140=CIRCLE('',#12661,0.312499999999998);
#4141=CIRCLE('',#12662,0.3125);
#4142=CIRCLE('',#12664,0.3125);
#4143=CIRCLE('',#12666,0.312500000000001);
#4144=CIRCLE('',#12667,0.3125);
#4145=CIRCLE('',#12669,0.312500000000003);
#4146=CIRCLE('',#12670,0.3125);
#4147=CIRCLE('',#12671,0.3125);
#4148=CIRCLE('',#12673,0.3125);
#4149=CIRCLE('',#12675,0.312500000000001);
#4150=CIRCLE('',#12677,0.3125);
#4151=CIRCLE('',#12678,0.3125);
#4152=CIRCLE('',#12680,0.3125);
#4153=CIRCLE('',#12682,0.312499999999999);
#4154=CIRCLE('',#12684,0.3125);
#4155=CIRCLE('',#12686,0.312499999999998);
#4156=CIRCLE('',#12688,0.312499999999998);
#4157=CIRCLE('',#12689,0.312499999999999);
#4158=CIRCLE('',#12691,0.312499999999999);
#4159=CIRCLE('',#12693,0.3125);
#4160=CIRCLE('',#12695,0.3125);
#4161=CIRCLE('',#12697,0.312499999999998);
#4162=CIRCLE('',#12699,0.3125);
#4163=CIRCLE('',#12700,0.3125);
#4164=CIRCLE('',#12701,0.3125);
#4165=CIRCLE('',#12703,0.312499999999998);
#4166=CIRCLE('',#12705,0.3125);
#4167=CIRCLE('',#12707,0.312500000000001);
#4168=CIRCLE('',#12709,0.3125);
#4169=CIRCLE('',#12710,0.3125);
#4170=CIRCLE('',#12712,0.312500000000001);
#4171=CIRCLE('',#12714,0.3125);
#4172=CIRCLE('',#12715,0.3125);
#4173=CIRCLE('',#12717,0.312499999999998);
#4174=CIRCLE('',#12719,0.3125);
#4175=CIRCLE('',#12722,0.3125);
#4176=CIRCLE('',#12723,0.3125);
#4177=CIRCLE('',#12725,0.312500000000004);
#4178=CIRCLE('',#12727,0.312500000000001);
#4179=CIRCLE('',#12729,0.312500000000001);
#4180=CIRCLE('',#12731,0.3125);
#4181=CIRCLE('',#12732,0.3125);
#4182=CIRCLE('',#12734,0.312499999999997);
#4183=CIRCLE('',#12736,0.312500000000002);
#4184=CIRCLE('',#12738,0.312499999999997);
#4185=CIRCLE('',#12740,0.3125);
#4186=CIRCLE('',#12742,0.3125);
#4187=CIRCLE('',#12744,0.312500000000001);
#4188=CIRCLE('',#12745,0.312499999999999);
#4189=CIRCLE('',#12747,0.312500000000001);
#4190=CIRCLE('',#12749,0.312499999999999);
#4191=CIRCLE('',#12751,0.312499999999999);
#4192=CIRCLE('',#12753,0.312500000000001);
#4193=CIRCLE('',#12755,0.3125);
#4194=CIRCLE('',#12756,0.3125);
#4195=CIRCLE('',#12758,0.3125);
#4196=CIRCLE('',#12760,0.312500000000001);
#4197=CIRCLE('',#12762,0.312499999999999);
#4198=CIRCLE('',#12764,0.3125);
#4199=CIRCLE('',#12766,0.312499999999998);
#4200=CIRCLE('',#12767,0.3125);
#4201=CIRCLE('',#12769,0.3125);
#4202=CIRCLE('',#12771,0.312500000000001);
#4203=CIRCLE('',#12773,0.312499999999997);
#4204=CIRCLE('',#12775,0.3125);
#4205=CIRCLE('',#12776,0.312500000000003);
#4206=CIRCLE('',#12778,0.312500000000001);
#4207=CIRCLE('',#12780,0.3125);
#4208=CIRCLE('',#12783,0.3125);
#4209=CIRCLE('',#12785,0.312500000000001);
#4210=CIRCLE('',#12787,0.3125);
#4211=CIRCLE('',#12789,0.312499999999999);
#4212=CIRCLE('',#12791,0.312499999999997);
#4213=CIRCLE('',#12792,0.31366374033177);
#4214=CIRCLE('',#12793,0.313663740332204);
#4215=CIRCLE('',#12794,0.313663740331843);
#4216=CIRCLE('',#12796,0.3125);
#4217=CIRCLE('',#12797,0.3125);
#4218=CIRCLE('',#12798,0.312500000000001);
#4219=CIRCLE('',#12799,0.312500000000001);
#4220=CIRCLE('',#12801,0.312500000000001);
#4221=CIRCLE('',#12803,0.3125);
#4222=CIRCLE('',#12804,0.3125);
#4223=CIRCLE('',#12806,0.312500000000001);
#4224=CIRCLE('',#12807,0.312500000000001);
#4225=CIRCLE('',#12808,0.3125);
#4226=CIRCLE('',#12812,0.312500000000001);
#4227=CIRCLE('',#12814,0.3125);
#4228=CIRCLE('',#12815,0.313663740332451);
#4229=CIRCLE('',#12816,0.3125);
#4230=CIRCLE('',#12817,0.312500000000001);
#4231=CIRCLE('',#12821,0.3125);
#4232=CIRCLE('',#12823,0.312500000000001);
#4233=CIRCLE('',#12824,0.313672771251787);
#4234=CIRCLE('',#12826,0.3125);
#4235=CIRCLE('',#12827,0.3125);
#4236=CIRCLE('',#12829,0.3125);
#4237=CIRCLE('',#12831,0.3125);
#4238=CIRCLE('',#12833,0.3125);
#4239=CIRCLE('',#12835,0.3125);
#4240=CIRCLE('',#12837,0.3125);
#4241=CIRCLE('',#12839,0.3125);
#4242=CIRCLE('',#12842,0.3125);
#4243=CIRCLE('',#12843,0.3125);
#4244=CIRCLE('',#12845,0.3125);
#4245=CIRCLE('',#12847,0.3125);
#4246=CIRCLE('',#12849,0.3125);
#4247=CIRCLE('',#12851,0.3125);
#4248=CIRCLE('',#12853,0.3125);
#4249=CIRCLE('',#12855,0.3125);
#4250=CIRCLE('',#12858,0.312499999999997);
#4251=CIRCLE('',#12860,0.3125);
#4252=CIRCLE('',#12862,0.3125);
#4253=CIRCLE('',#12863,0.3125);
#4254=CIRCLE('',#12865,0.3125);
#4255=CIRCLE('',#12867,0.312499999999997);
#4256=CIRCLE('',#12869,0.312499999999997);
#4257=CIRCLE('',#12872,0.312500000000001);
#4258=CIRCLE('',#12874,0.3125);
#4259=CIRCLE('',#12876,0.3125);
#4260=CIRCLE('',#12877,0.3125);
#4261=CIRCLE('',#12879,0.3125);
#4262=CIRCLE('',#12881,0.312499999999997);
#4263=CIRCLE('',#12883,0.312499999999997);
#4264=CIRCLE('',#12886,0.3125);
#4265=CIRCLE('',#12888,0.3125);
#4266=CIRCLE('',#12890,0.3125);
#4267=CIRCLE('',#12893,0.312499999999997);
#4268=CIRCLE('',#12896,0.3125);
#4269=CIRCLE('',#12898,0.3125);
#4270=CIRCLE('',#12900,0.3125);
#4271=CIRCLE('',#12903,0.312499999999997);
#4272=CIRCLE('',#12906,0.3125);
#4273=CIRCLE('',#12908,0.3125);
#4274=CIRCLE('',#12911,0.3125);
#4275=CIRCLE('',#12913,0.312499999999997);
#4276=CIRCLE('',#12916,0.3125);
#4277=CIRCLE('',#12918,0.3125);
#4278=CIRCLE('',#12921,0.3125);
#4279=CIRCLE('',#12923,0.312499999999997);
#4301=VERTEX_POINT('',#16376);
#4302=VERTEX_POINT('',#16378);
#4303=VERTEX_POINT('',#16382);
#4304=VERTEX_POINT('',#16384);
#4305=VERTEX_POINT('',#16388);
#4306=VERTEX_POINT('',#16390);
#4307=VERTEX_POINT('',#16394);
#4308=VERTEX_POINT('',#16396);
#4309=VERTEX_POINT('',#16400);
#4310=VERTEX_POINT('',#16401);
#4311=VERTEX_POINT('',#16404);
#4312=VERTEX_POINT('',#16408);
#4313=VERTEX_POINT('',#16410);
#4314=VERTEX_POINT('',#16412);
#4315=VERTEX_POINT('',#16416);
#4316=VERTEX_POINT('',#16418);
#4317=VERTEX_POINT('',#16422);
#4318=VERTEX_POINT('',#16424);
#4319=VERTEX_POINT('',#16426);
#4320=VERTEX_POINT('',#16430);
#4321=VERTEX_POINT('',#16431);
#4322=VERTEX_POINT('',#16433);
#4323=VERTEX_POINT('',#16435);
#4324=VERTEX_POINT('',#16439);
#4325=VERTEX_POINT('',#16440);
#4326=VERTEX_POINT('',#16442);
#4327=VERTEX_POINT('',#16444);
#4328=VERTEX_POINT('',#16448);
#4329=VERTEX_POINT('',#16449);
#4330=VERTEX_POINT('',#16451);
#4331=VERTEX_POINT('',#16453);
#4332=VERTEX_POINT('',#16457);
#4333=VERTEX_POINT('',#16458);
#4334=VERTEX_POINT('',#16460);
#4335=VERTEX_POINT('',#16462);
#4336=VERTEX_POINT('',#16466);
#4337=VERTEX_POINT('',#16467);
#4338=VERTEX_POINT('',#16470);
#4339=VERTEX_POINT('',#16474);
#4340=VERTEX_POINT('',#16476);
#4341=VERTEX_POINT('',#16478);
#4342=VERTEX_POINT('',#16482);
#4343=VERTEX_POINT('',#16484);
#4344=VERTEX_POINT('',#16486);
#4345=VERTEX_POINT('',#16490);
#4346=VERTEX_POINT('',#16492);
#4347=VERTEX_POINT('',#16494);
#4348=VERTEX_POINT('',#16498);
#4349=VERTEX_POINT('',#16499);
#4350=VERTEX_POINT('',#16501);
#4351=VERTEX_POINT('',#16503);
#4352=VERTEX_POINT('',#16507);
#4353=VERTEX_POINT('',#16508);
#4354=VERTEX_POINT('',#16510);
#4355=VERTEX_POINT('',#16512);
#4356=VERTEX_POINT('',#16516);
#4357=VERTEX_POINT('',#16517);
#4358=VERTEX_POINT('',#16519);
#4359=VERTEX_POINT('',#16521);
#4360=VERTEX_POINT('',#16525);
#4361=VERTEX_POINT('',#16526);
#4362=VERTEX_POINT('',#16528);
#4363=VERTEX_POINT('',#16530);
#4364=VERTEX_POINT('',#16534);
#4365=VERTEX_POINT('',#16536);
#4366=VERTEX_POINT('',#16540);
#4367=VERTEX_POINT('',#16542);
#4368=VERTEX_POINT('',#16546);
#4369=VERTEX_POINT('',#16548);
#4370=VERTEX_POINT('',#16550);
#4371=VERTEX_POINT('',#16554);
#4372=VERTEX_POINT('',#16556);
#4373=VERTEX_POINT('',#16560);
#4374=VERTEX_POINT('',#16561);
#4375=VERTEX_POINT('',#16563);
#4376=VERTEX_POINT('',#16565);
#4377=VERTEX_POINT('',#16569);
#4378=VERTEX_POINT('',#16570);
#4379=VERTEX_POINT('',#16572);
#4380=VERTEX_POINT('',#16574);
#4381=VERTEX_POINT('',#16578);
#4382=VERTEX_POINT('',#16579);
#4383=VERTEX_POINT('',#16581);
#4384=VERTEX_POINT('',#16586);
#4385=VERTEX_POINT('',#16588);
#4386=VERTEX_POINT('',#16590);
#4387=VERTEX_POINT('',#16594);
#4388=VERTEX_POINT('',#16596);
#4389=VERTEX_POINT('',#16598);
#4390=VERTEX_POINT('',#16602);
#4391=VERTEX_POINT('',#16604);
#4392=VERTEX_POINT('',#16606);
#4393=VERTEX_POINT('',#16610);
#4394=VERTEX_POINT('',#16611);
#4395=VERTEX_POINT('',#16613);
#4396=VERTEX_POINT('',#16615);
#4397=VERTEX_POINT('',#16619);
#4398=VERTEX_POINT('',#16620);
#4399=VERTEX_POINT('',#16622);
#4400=VERTEX_POINT('',#16624);
#4401=VERTEX_POINT('',#16628);
#4402=VERTEX_POINT('',#16629);
#4403=VERTEX_POINT('',#16631);
#4404=VERTEX_POINT('',#16633);
#4405=VERTEX_POINT('',#16637);
#4406=VERTEX_POINT('',#16638);
#4407=VERTEX_POINT('',#16640);
#4408=VERTEX_POINT('',#16642);
#4409=VERTEX_POINT('',#16646);
#4410=VERTEX_POINT('',#16647);
#4411=VERTEX_POINT('',#16649);
#4412=VERTEX_POINT('',#16651);
#4413=VERTEX_POINT('',#16655);
#4414=VERTEX_POINT('',#16656);
#4415=VERTEX_POINT('',#16658);
#4416=VERTEX_POINT('',#16660);
#4417=VERTEX_POINT('',#16664);
#4418=VERTEX_POINT('',#16665);
#4419=VERTEX_POINT('',#16667);
#4420=VERTEX_POINT('',#16669);
#4421=VERTEX_POINT('',#16673);
#4422=VERTEX_POINT('',#16674);
#4423=VERTEX_POINT('',#16676);
#4424=VERTEX_POINT('',#16678);
#4425=VERTEX_POINT('',#16682);
#4426=VERTEX_POINT('',#16683);
#4427=VERTEX_POINT('',#16685);
#4428=VERTEX_POINT('',#16687);
#4429=VERTEX_POINT('',#16691);
#4430=VERTEX_POINT('',#16693);
#4431=VERTEX_POINT('',#16697);
#4432=VERTEX_POINT('',#16698);
#4433=VERTEX_POINT('',#16700);
#4434=VERTEX_POINT('',#16702);
#4435=VERTEX_POINT('',#16706);
#4436=VERTEX_POINT('',#16707);
#4437=VERTEX_POINT('',#16709);
#4438=VERTEX_POINT('',#16711);
#4439=VERTEX_POINT('',#16715);
#4440=VERTEX_POINT('',#16716);
#4441=VERTEX_POINT('',#16718);
#4442=VERTEX_POINT('',#16720);
#4443=VERTEX_POINT('',#16724);
#4444=VERTEX_POINT('',#16725);
#4445=VERTEX_POINT('',#16727);
#4446=VERTEX_POINT('',#16729);
#4447=VERTEX_POINT('',#16733);
#4448=VERTEX_POINT('',#16734);
#4449=VERTEX_POINT('',#16736);
#4450=VERTEX_POINT('',#16738);
#4451=VERTEX_POINT('',#16742);
#4452=VERTEX_POINT('',#16743);
#4453=VERTEX_POINT('',#16745);
#4454=VERTEX_POINT('',#16747);
#4455=VERTEX_POINT('',#16751);
#4456=VERTEX_POINT('',#16752);
#4457=VERTEX_POINT('',#16754);
#4458=VERTEX_POINT('',#16756);
#4459=VERTEX_POINT('',#16760);
#4460=VERTEX_POINT('',#16761);
#4461=VERTEX_POINT('',#16763);
#4462=VERTEX_POINT('',#16765);
#4463=VERTEX_POINT('',#16769);
#4464=VERTEX_POINT('',#16772);
#4465=VERTEX_POINT('',#16780);
#4466=VERTEX_POINT('',#16782);
#4467=VERTEX_POINT('',#16786);
#4468=VERTEX_POINT('',#16787);
#4469=VERTEX_POINT('',#16789);
#4470=VERTEX_POINT('',#16791);
#4471=VERTEX_POINT('',#16795);
#4472=VERTEX_POINT('',#16797);
#4473=VERTEX_POINT('',#16806);
#4474=VERTEX_POINT('',#16815);
#4475=VERTEX_POINT('',#16817);
#4476=VERTEX_POINT('',#16828);
#4477=VERTEX_POINT('',#16839);
#4478=VERTEX_POINT('',#16850);
#4479=VERTEX_POINT('',#16852);
#4480=VERTEX_POINT('',#16856);
#4481=VERTEX_POINT('',#16857);
#4482=VERTEX_POINT('',#16859);
#4483=VERTEX_POINT('',#16861);
#4484=VERTEX_POINT('',#16872);
#4485=VERTEX_POINT('',#16873);
#4486=VERTEX_POINT('',#16875);
#4487=VERTEX_POINT('',#16884);
#4488=VERTEX_POINT('',#16886);
#4489=VERTEX_POINT('',#16897);
#4490=VERTEX_POINT('',#16908);
#4491=VERTEX_POINT('',#16919);
#4492=VERTEX_POINT('',#16920);
#4493=VERTEX_POINT('',#16931);
#4494=VERTEX_POINT('',#16932);
#4495=VERTEX_POINT('',#16934);
#4496=VERTEX_POINT('',#16936);
#4497=VERTEX_POINT('',#16938);
#4498=VERTEX_POINT('',#16940);
#4499=VERTEX_POINT('',#16942);
#4500=VERTEX_POINT('',#16944);
#4501=VERTEX_POINT('',#16946);
#4502=VERTEX_POINT('',#16948);
#4503=VERTEX_POINT('',#16950);
#4504=VERTEX_POINT('',#16997);
#4505=VERTEX_POINT('',#16999);
#4506=VERTEX_POINT('',#17001);
#4507=VERTEX_POINT('',#17003);
#4508=VERTEX_POINT('',#17035);
#4509=VERTEX_POINT('',#17037);
#4510=VERTEX_POINT('',#17072);
#4511=VERTEX_POINT('',#17075);
#4512=VERTEX_POINT('',#17119);
#4513=VERTEX_POINT('',#17121);
#4514=VERTEX_POINT('',#17123);
#4515=VERTEX_POINT('',#17125);
#4516=VERTEX_POINT('',#17127);
#4517=VERTEX_POINT('',#17174);
#4518=VERTEX_POINT('',#17177);
#4519=VERTEX_POINT('',#17209);
#4520=VERTEX_POINT('',#17211);
#4521=VERTEX_POINT('',#17246);
#4522=VERTEX_POINT('',#17248);
#4523=VERTEX_POINT('',#17250);
#4524=VERTEX_POINT('',#17252);
#4525=VERTEX_POINT('',#17296);
#4526=VERTEX_POINT('',#17298);
#4527=VERTEX_POINT('',#17300);
#4528=VERTEX_POINT('',#17302);
#4529=VERTEX_POINT('',#17304);
#4530=VERTEX_POINT('',#17351);
#4531=VERTEX_POINT('',#17353);
#4532=VERTEX_POINT('',#17355);
#4533=VERTEX_POINT('',#17357);
#4534=VERTEX_POINT('',#17389);
#4535=VERTEX_POINT('',#17425);
#4536=VERTEX_POINT('',#17427);
#4537=VERTEX_POINT('',#17429);
#4538=VERTEX_POINT('',#17473);
#4539=VERTEX_POINT('',#17475);
#4540=VERTEX_POINT('',#17477);
#4541=VERTEX_POINT('',#17479);
#4542=VERTEX_POINT('',#17527);
#4543=VERTEX_POINT('',#17529);
#4544=VERTEX_POINT('',#17531);
#4545=VERTEX_POINT('',#17563);
#4546=VERTEX_POINT('',#17565);
#4547=VERTEX_POINT('',#17600);
#4548=VERTEX_POINT('',#17602);
#4549=VERTEX_POINT('',#17604);
#4550=VERTEX_POINT('',#17606);
#4551=VERTEX_POINT('',#17650);
#4552=VERTEX_POINT('',#17653);
#4553=VERTEX_POINT('',#17655);
#4554=VERTEX_POINT('',#17657);
#4555=VERTEX_POINT('',#17659);
#4556=VERTEX_POINT('',#17661);
#4557=VERTEX_POINT('',#17669);
#4558=VERTEX_POINT('',#17670);
#4559=VERTEX_POINT('',#17672);
#4560=VERTEX_POINT('',#17681);
#4561=VERTEX_POINT('',#17683);
#4562=VERTEX_POINT('',#17694);
#4563=VERTEX_POINT('',#17705);
#4564=VERTEX_POINT('',#17716);
#4565=VERTEX_POINT('',#17717);
#4566=VERTEX_POINT('',#17722);
#4567=VERTEX_POINT('',#17723);
#4568=VERTEX_POINT('',#17725);
#4569=VERTEX_POINT('',#17727);
#4570=VERTEX_POINT('',#17731);
#4571=VERTEX_POINT('',#17732);
#4572=VERTEX_POINT('',#17734);
#4573=VERTEX_POINT('',#17736);
#4574=VERTEX_POINT('',#17739);
#4575=VERTEX_POINT('',#17741);
#4576=VERTEX_POINT('',#17743);
#4577=VERTEX_POINT('',#17745);
#4578=VERTEX_POINT('',#17747);
#4579=VERTEX_POINT('',#17749);
#4580=VERTEX_POINT('',#17751);
#4581=VERTEX_POINT('',#17753);
#4582=VERTEX_POINT('',#17755);
#4583=VERTEX_POINT('',#17757);
#4584=VERTEX_POINT('',#17759);
#4585=VERTEX_POINT('',#17761);
#4586=VERTEX_POINT('',#17763);
#4587=VERTEX_POINT('',#17765);
#4588=VERTEX_POINT('',#17767);
#4589=VERTEX_POINT('',#17769);
#4590=VERTEX_POINT('',#17772);
#4591=VERTEX_POINT('',#17773);
#4592=VERTEX_POINT('',#17775);
#4593=VERTEX_POINT('',#17777);
#4594=VERTEX_POINT('',#17779);
#4595=VERTEX_POINT('',#17782);
#4596=VERTEX_POINT('',#17785);
#4597=VERTEX_POINT('',#17787);
#4598=VERTEX_POINT('',#17789);
#4599=VERTEX_POINT('',#17792);
#4600=VERTEX_POINT('',#17795);
#4601=VERTEX_POINT('',#17797);
#4602=VERTEX_POINT('',#17800);
#4603=VERTEX_POINT('',#17802);
#4604=VERTEX_POINT('',#17805);
#4605=VERTEX_POINT('',#17806);
#4606=VERTEX_POINT('',#17815);
#4607=VERTEX_POINT('',#17817);
#4608=VERTEX_POINT('',#17826);
#4609=VERTEX_POINT('',#17828);
#4610=VERTEX_POINT('',#17848);
#4611=VERTEX_POINT('',#17850);
#4612=VERTEX_POINT('',#17870);
#4613=VERTEX_POINT('',#17872);
#4614=VERTEX_POINT('',#17892);
#4615=VERTEX_POINT('',#17894);
#4616=VERTEX_POINT('',#17903);
#4617=VERTEX_POINT('',#17905);
#4618=VERTEX_POINT('',#17925);
#4619=VERTEX_POINT('',#17927);
#4620=VERTEX_POINT('',#17949);
#4621=VERTEX_POINT('',#17950);
#4622=VERTEX_POINT('',#17952);
#4623=VERTEX_POINT('',#17954);
#4624=VERTEX_POINT('',#17958);
#4625=VERTEX_POINT('',#17959);
#4626=VERTEX_POINT('',#17961);
#4627=VERTEX_POINT('',#17963);
#4628=VERTEX_POINT('',#17967);
#4629=VERTEX_POINT('',#17968);
#4630=VERTEX_POINT('',#17970);
#4631=VERTEX_POINT('',#17972);
#4632=VERTEX_POINT('',#17974);
#4633=VERTEX_POINT('',#17976);
#4634=VERTEX_POINT('',#17978);
#4635=VERTEX_POINT('',#17980);
#4636=VERTEX_POINT('',#17982);
#4637=VERTEX_POINT('',#17984);
#4638=VERTEX_POINT('',#17986);
#4639=VERTEX_POINT('',#17988);
#4640=VERTEX_POINT('',#17990);
#4641=VERTEX_POINT('',#17992);
#4642=VERTEX_POINT('',#17994);
#4643=VERTEX_POINT('',#17996);
#4644=VERTEX_POINT('',#17998);
#4645=VERTEX_POINT('',#18000);
#4646=VERTEX_POINT('',#18004);
#4647=VERTEX_POINT('',#18005);
#4648=VERTEX_POINT('',#18007);
#4649=VERTEX_POINT('',#18009);
#4650=VERTEX_POINT('',#18011);
#4651=VERTEX_POINT('',#18013);
#4652=VERTEX_POINT('',#18016);
#4653=VERTEX_POINT('',#18018);
#4654=VERTEX_POINT('',#18020);
#4655=VERTEX_POINT('',#18022);
#4656=VERTEX_POINT('',#18024);
#4657=VERTEX_POINT('',#18026);
#4658=VERTEX_POINT('',#18028);
#4659=VERTEX_POINT('',#18030);
#4660=VERTEX_POINT('',#18034);
#4661=VERTEX_POINT('',#18035);
#4662=VERTEX_POINT('',#18047);
#4663=VERTEX_POINT('',#18048);
#4664=VERTEX_POINT('',#18058);
#4665=VERTEX_POINT('',#18062);
#4666=VERTEX_POINT('',#18063);
#4667=VERTEX_POINT('',#18065);
#4668=VERTEX_POINT('',#18067);
#4669=VERTEX_POINT('',#18071);
#4670=VERTEX_POINT('',#18073);
#4671=VERTEX_POINT('',#18077);
#4672=VERTEX_POINT('',#18079);
#4673=VERTEX_POINT('',#18083);
#4674=VERTEX_POINT('',#18084);
#4675=VERTEX_POINT('',#18086);
#4676=VERTEX_POINT('',#18088);
#4677=VERTEX_POINT('',#18090);
#4678=VERTEX_POINT('',#18094);
#4679=VERTEX_POINT('',#18095);
#4680=VERTEX_POINT('',#18097);
#4681=VERTEX_POINT('',#18099);
#4682=VERTEX_POINT('',#18131);
#4683=VERTEX_POINT('',#18171);
#4684=VERTEX_POINT('',#18172);
#4685=VERTEX_POINT('',#18174);
#4686=VERTEX_POINT('',#18176);
#4687=VERTEX_POINT('',#18208);
#4688=VERTEX_POINT('',#18248);
#4689=VERTEX_POINT('',#18249);
#4690=VERTEX_POINT('',#18251);
#4691=VERTEX_POINT('',#18253);
#4692=VERTEX_POINT('',#18288);
#4693=VERTEX_POINT('',#18325);
#4694=VERTEX_POINT('',#18326);
#4695=VERTEX_POINT('',#18328);
#4696=VERTEX_POINT('',#18330);
#4697=VERTEX_POINT('',#18362);
#4698=VERTEX_POINT('',#18402);
#4699=VERTEX_POINT('',#18403);
#4700=VERTEX_POINT('',#18405);
#4701=VERTEX_POINT('',#18455);
#4702=VERTEX_POINT('',#18457);
#4703=VERTEX_POINT('',#18459);
#4704=VERTEX_POINT('',#18468);
#4705=VERTEX_POINT('',#18472);
#4706=VERTEX_POINT('',#18473);
#4707=VERTEX_POINT('',#18476);
#4708=VERTEX_POINT('',#18478);
#4709=VERTEX_POINT('',#18480);
#4710=VERTEX_POINT('',#18482);
#4711=VERTEX_POINT('',#18484);
#4712=VERTEX_POINT('',#18486);
#4713=VERTEX_POINT('',#18488);
#4714=VERTEX_POINT('',#18490);
#4715=VERTEX_POINT('',#18492);
#4716=VERTEX_POINT('',#18494);
#4717=VERTEX_POINT('',#18496);
#4718=VERTEX_POINT('',#18498);
#4719=VERTEX_POINT('',#18500);
#4720=VERTEX_POINT('',#18502);
#4721=VERTEX_POINT('',#18505);
#4722=VERTEX_POINT('',#18507);
#4723=VERTEX_POINT('',#18509);
#4724=VERTEX_POINT('',#18511);
#4725=VERTEX_POINT('',#18514);
#4726=VERTEX_POINT('',#18516);
#4727=VERTEX_POINT('',#18520);
#4728=VERTEX_POINT('',#18521);
#4729=VERTEX_POINT('',#18524);
#4730=VERTEX_POINT('',#18559);
#4731=VERTEX_POINT('',#18561);
#4732=VERTEX_POINT('',#18565);
#4733=VERTEX_POINT('',#18566);
#4734=VERTEX_POINT('',#18568);
#4735=VERTEX_POINT('',#18570);
#4736=VERTEX_POINT('',#18572);
#4737=VERTEX_POINT('',#18574);
#4738=VERTEX_POINT('',#18576);
#4739=VERTEX_POINT('',#18607);
#4740=VERTEX_POINT('',#18608);
#4741=VERTEX_POINT('',#18610);
#4742=VERTEX_POINT('',#18627);
#4743=VERTEX_POINT('',#18671);
#4744=VERTEX_POINT('',#18673);
#4745=VERTEX_POINT('',#18675);
#4746=VERTEX_POINT('',#18733);
#4747=VERTEX_POINT('',#18734);
#4748=VERTEX_POINT('',#18743);
#4749=VERTEX_POINT('',#18745);
#4750=VERTEX_POINT('',#18754);
#4751=VERTEX_POINT('',#18756);
#4752=VERTEX_POINT('',#18779);
#4753=VERTEX_POINT('',#18780);
#4754=VERTEX_POINT('',#18782);
#4755=VERTEX_POINT('',#18784);
#4756=VERTEX_POINT('',#18791);
#4757=VERTEX_POINT('',#18792);
#4758=VERTEX_POINT('',#18794);
#4759=VERTEX_POINT('',#18796);
#4760=VERTEX_POINT('',#18798);
#4761=VERTEX_POINT('',#18800);
#4762=VERTEX_POINT('',#18831);
#4763=VERTEX_POINT('',#18832);
#4764=VERTEX_POINT('',#18834);
#4765=VERTEX_POINT('',#18836);
#4766=VERTEX_POINT('',#18838);
#4767=VERTEX_POINT('',#18840);
#4768=VERTEX_POINT('',#18883);
#4769=VERTEX_POINT('',#18884);
#4770=VERTEX_POINT('',#18886);
#4771=VERTEX_POINT('',#18888);
#4772=VERTEX_POINT('',#18890);
#4773=VERTEX_POINT('',#18893);
#4774=VERTEX_POINT('',#18897);
#4775=VERTEX_POINT('',#18898);
#4776=VERTEX_POINT('',#18900);
#4777=VERTEX_POINT('',#18902);
#4778=VERTEX_POINT('',#18904);
#4779=VERTEX_POINT('',#18906);
#4780=VERTEX_POINT('',#18908);
#4781=VERTEX_POINT('',#18910);
#4782=VERTEX_POINT('',#18914);
#4783=VERTEX_POINT('',#18915);
#4784=VERTEX_POINT('',#18935);
#4785=VERTEX_POINT('',#18937);
#4786=VERTEX_POINT('',#18939);
#4787=VERTEX_POINT('',#18941);
#4788=VERTEX_POINT('',#18943);
#4789=VERTEX_POINT('',#18945);
#4790=VERTEX_POINT('',#19027);
#4791=VERTEX_POINT('',#19028);
#4792=VERTEX_POINT('',#19030);
#4793=VERTEX_POINT('',#19032);
#4794=VERTEX_POINT('',#19046);
#4795=VERTEX_POINT('',#19129);
#4796=VERTEX_POINT('',#19149);
#4797=VERTEX_POINT('',#19151);
#4798=VERTEX_POINT('',#19158);
#4799=VERTEX_POINT('',#19159);
#4800=VERTEX_POINT('',#19161);
#4801=VERTEX_POINT('',#19163);
#4802=VERTEX_POINT('',#19177);
#4803=VERTEX_POINT('',#19212);
#4804=VERTEX_POINT('',#19226);
#4805=VERTEX_POINT('',#19228);
#4806=VERTEX_POINT('',#19232);
#4807=VERTEX_POINT('',#19233);
#4808=VERTEX_POINT('',#19247);
#4809=VERTEX_POINT('',#19249);
#4810=VERTEX_POINT('',#19251);
#4811=VERTEX_POINT('',#19253);
#4812=VERTEX_POINT('',#19255);
#4813=VERTEX_POINT('',#19257);
#4814=VERTEX_POINT('',#19291);
#4815=VERTEX_POINT('',#19292);
#4816=VERTEX_POINT('',#19294);
#4817=VERTEX_POINT('',#19296);
#4818=VERTEX_POINT('',#19298);
#4819=VERTEX_POINT('',#19300);
#4820=VERTEX_POINT('',#19302);
#4821=VERTEX_POINT('',#19304);
#4822=VERTEX_POINT('',#19360);
#4823=VERTEX_POINT('',#19362);
#4824=VERTEX_POINT('',#19382);
#4825=VERTEX_POINT('',#19384);
#4826=VERTEX_POINT('',#19393);
#4827=VERTEX_POINT('',#19395);
#4828=VERTEX_POINT('',#19451);
#4829=VERTEX_POINT('',#19453);
#4830=VERTEX_POINT('',#19456);
#4831=VERTEX_POINT('',#19458);
#4832=VERTEX_POINT('',#19460);
#4833=VERTEX_POINT('',#19462);
#4834=VERTEX_POINT('',#19464);
#4835=VERTEX_POINT('',#19467);
#4836=VERTEX_POINT('',#19469);
#4837=VERTEX_POINT('',#19471);
#4838=VERTEX_POINT('',#19473);
#4839=VERTEX_POINT('',#19475);
#4840=VERTEX_POINT('',#19477);
#4841=VERTEX_POINT('',#19480);
#4842=VERTEX_POINT('',#19481);
#4843=VERTEX_POINT('',#19483);
#4844=VERTEX_POINT('',#19539);
#4845=VERTEX_POINT('',#19541);
#4846=VERTEX_POINT('',#19543);
#4847=VERTEX_POINT('',#19545);
#4848=VERTEX_POINT('',#19547);
#4849=VERTEX_POINT('',#19603);
#4850=VERTEX_POINT('',#19605);
#4851=VERTEX_POINT('',#19628);
#4852=VERTEX_POINT('',#19638);
#4853=VERTEX_POINT('',#19639);
#4854=VERTEX_POINT('',#19641);
#4855=VERTEX_POINT('',#19697);
#4856=VERTEX_POINT('',#19700);
#4857=VERTEX_POINT('',#19702);
#4858=VERTEX_POINT('',#19758);
#4859=VERTEX_POINT('',#19760);
#4860=VERTEX_POINT('',#19783);
#4861=VERTEX_POINT('',#19793);
#4862=VERTEX_POINT('',#19794);
#4863=VERTEX_POINT('',#19796);
#4864=VERTEX_POINT('',#19798);
#4865=VERTEX_POINT('',#19800);
#4866=VERTEX_POINT('',#19856);
#4867=VERTEX_POINT('',#19858);
#4868=VERTEX_POINT('',#19881);
#4869=VERTEX_POINT('',#19883);
#4870=VERTEX_POINT('',#19892);
#4871=VERTEX_POINT('',#19894);
#4872=VERTEX_POINT('',#19955);
#4873=VERTEX_POINT('',#19956);
#4874=VERTEX_POINT('',#19965);
#4875=VERTEX_POINT('',#19967);
#4876=VERTEX_POINT('',#19978);
#4877=VERTEX_POINT('',#19979);
#4878=VERTEX_POINT('',#19981);
#4879=VERTEX_POINT('',#20016);
#4880=VERTEX_POINT('',#20018);
#4881=VERTEX_POINT('',#20055);
#4882=VERTEX_POINT('',#20056);
#4883=VERTEX_POINT('',#20058);
#4884=VERTEX_POINT('',#20090);
#4885=VERTEX_POINT('',#20092);
#4886=VERTEX_POINT('',#20132);
#4887=VERTEX_POINT('',#20140);
#4888=VERTEX_POINT('',#20144);
#4889=VERTEX_POINT('',#20146);
#4890=VERTEX_POINT('',#20153);
#4891=VERTEX_POINT('',#20155);
#4892=VERTEX_POINT('',#20159);
#4893=VERTEX_POINT('',#20160);
#4894=VERTEX_POINT('',#20162);
#4895=VERTEX_POINT('',#20164);
#4896=VERTEX_POINT('',#20168);
#4897=VERTEX_POINT('',#20169);
#4898=VERTEX_POINT('',#20171);
#4899=VERTEX_POINT('',#20173);
#4900=VERTEX_POINT('',#20177);
#4901=VERTEX_POINT('',#20178);
#4902=VERTEX_POINT('',#20180);
#4903=VERTEX_POINT('',#20190);
#4904=VERTEX_POINT('',#20191);
#4905=VERTEX_POINT('',#20193);
#4906=VERTEX_POINT('',#20195);
#4907=VERTEX_POINT('',#20199);
#4908=VERTEX_POINT('',#20200);
#4909=VERTEX_POINT('',#20202);
#4910=VERTEX_POINT('',#20209);
#4911=VERTEX_POINT('',#20211);
#4912=VERTEX_POINT('',#20215);
#4913=VERTEX_POINT('',#20216);
#4914=VERTEX_POINT('',#20221);
#4915=VERTEX_POINT('',#20222);
#4916=VERTEX_POINT('',#20224);
#4917=VERTEX_POINT('',#20226);
#4918=VERTEX_POINT('',#20230);
#4919=VERTEX_POINT('',#20233);
#4920=VERTEX_POINT('',#20235);
#4921=VERTEX_POINT('',#20237);
#4922=VERTEX_POINT('',#20250);
#4923=VERTEX_POINT('',#20251);
#4924=VERTEX_POINT('',#20253);
#4925=VERTEX_POINT('',#20303);
#4926=VERTEX_POINT('',#20305);
#4927=VERTEX_POINT('',#20307);
#4928=VERTEX_POINT('',#20316);
#4929=VERTEX_POINT('',#20320);
#4930=VERTEX_POINT('',#20322);
#4931=VERTEX_POINT('',#20324);
#4932=VERTEX_POINT('',#20326);
#4933=VERTEX_POINT('',#20361);
#4934=VERTEX_POINT('',#20363);
#4935=VERTEX_POINT('',#20367);
#4936=VERTEX_POINT('',#20369);
#4937=VERTEX_POINT('',#20371);
#4938=VERTEX_POINT('',#20373);
#4939=VERTEX_POINT('',#20375);
#4940=VERTEX_POINT('',#20406);
#4941=VERTEX_POINT('',#20407);
#4942=VERTEX_POINT('',#20409);
#4943=VERTEX_POINT('',#20426);
#4944=VERTEX_POINT('',#20470);
#4945=VERTEX_POINT('',#20472);
#4946=VERTEX_POINT('',#20474);
#4947=VERTEX_POINT('',#20532);
#4948=VERTEX_POINT('',#20533);
#4949=VERTEX_POINT('',#20535);
#4950=VERTEX_POINT('',#20537);
#4951=VERTEX_POINT('',#20541);
#4952=VERTEX_POINT('',#20542);
#4953=VERTEX_POINT('',#20544);
#4954=VERTEX_POINT('',#20546);
#4955=VERTEX_POINT('',#20548);
#4956=VERTEX_POINT('',#20550);
#4957=VERTEX_POINT('',#20593);
#4958=VERTEX_POINT('',#20594);
#4959=VERTEX_POINT('',#20596);
#4960=VERTEX_POINT('',#20598);
#4961=VERTEX_POINT('',#20600);
#4962=VERTEX_POINT('',#20603);
#4963=VERTEX_POINT('',#20607);
#4964=VERTEX_POINT('',#20608);
#4965=VERTEX_POINT('',#20610);
#4966=VERTEX_POINT('',#20612);
#4967=VERTEX_POINT('',#20614);
#4968=VERTEX_POINT('',#20616);
#4969=VERTEX_POINT('',#20618);
#4970=VERTEX_POINT('',#20620);
#4971=VERTEX_POINT('',#20624);
#4972=VERTEX_POINT('',#20625);
#4973=VERTEX_POINT('',#20627);
#4974=VERTEX_POINT('',#20629);
#4975=VERTEX_POINT('',#20631);
#4976=VERTEX_POINT('',#20633);
#4977=VERTEX_POINT('',#20635);
#4978=VERTEX_POINT('',#20649);
#4979=VERTEX_POINT('',#20740);
#4980=VERTEX_POINT('',#20741);
#4981=VERTEX_POINT('',#20743);
#4982=VERTEX_POINT('',#20745);
#4983=VERTEX_POINT('',#20747);
#4984=VERTEX_POINT('',#20761);
#4985=VERTEX_POINT('',#20796);
#4986=VERTEX_POINT('',#20810);
#4987=VERTEX_POINT('',#20817);
#4988=VERTEX_POINT('',#20818);
#4989=VERTEX_POINT('',#20827);
#4990=VERTEX_POINT('',#20829);
#4991=VERTEX_POINT('',#20840);
#4992=VERTEX_POINT('',#20841);
#4993=VERTEX_POINT('',#20843);
#4994=VERTEX_POINT('',#20878);
#4995=VERTEX_POINT('',#20880);
#4996=VERTEX_POINT('',#20917);
#4997=VERTEX_POINT('',#20918);
#4998=VERTEX_POINT('',#20926);
#4999=VERTEX_POINT('',#20928);
#5000=VERTEX_POINT('',#20932);
#5001=VERTEX_POINT('',#20940);
#5002=VERTEX_POINT('',#20944);
#5003=VERTEX_POINT('',#20949);
#5004=VERTEX_POINT('',#20950);
#5005=VERTEX_POINT('',#20952);
#5006=VERTEX_POINT('',#20954);
#5007=VERTEX_POINT('',#20958);
#5008=VERTEX_POINT('',#20959);
#5009=VERTEX_POINT('',#20961);
#5010=VERTEX_POINT('',#20971);
#5011=VERTEX_POINT('',#20972);
#5012=VERTEX_POINT('',#20974);
#5013=VERTEX_POINT('',#20976);
#5014=VERTEX_POINT('',#20980);
#5015=VERTEX_POINT('',#20981);
#5016=VERTEX_POINT('',#20983);
#5017=VERTEX_POINT('',#20994);
#5018=VERTEX_POINT('',#20995);
#5019=VERTEX_POINT('',#21001);
#5020=VERTEX_POINT('',#21003);
#5021=VERTEX_POINT('',#21007);
#5022=VERTEX_POINT('',#21009);
#5023=VERTEX_POINT('',#21011);
#5024=VERTEX_POINT('',#21014);
#5025=VERTEX_POINT('',#21025);
#5026=VERTEX_POINT('',#21026);
#5027=VERTEX_POINT('',#21028);
#5028=VERTEX_POINT('',#21078);
#5029=VERTEX_POINT('',#21080);
#5030=VERTEX_POINT('',#21082);
#5031=VERTEX_POINT('',#21091);
#5032=VERTEX_POINT('',#21095);
#5033=VERTEX_POINT('',#21096);
#5034=VERTEX_POINT('',#21098);
#5035=VERTEX_POINT('',#21100);
#5036=VERTEX_POINT('',#21102);
#5037=VERTEX_POINT('',#21104);
#5038=VERTEX_POINT('',#21139);
#5039=VERTEX_POINT('',#21143);
#5040=VERTEX_POINT('',#21144);
#5041=VERTEX_POINT('',#21146);
#5042=VERTEX_POINT('',#21148);
#5043=VERTEX_POINT('',#21150);
#5044=VERTEX_POINT('',#21152);
#5045=VERTEX_POINT('',#21154);
#5046=VERTEX_POINT('',#21185);
#5047=VERTEX_POINT('',#21186);
#5048=VERTEX_POINT('',#21188);
#5049=VERTEX_POINT('',#21205);
#5050=VERTEX_POINT('',#21249);
#5051=VERTEX_POINT('',#21251);
#5052=VERTEX_POINT('',#21253);
#5053=VERTEX_POINT('',#21314);
#5054=VERTEX_POINT('',#21316);
#5055=VERTEX_POINT('',#21318);
#5056=VERTEX_POINT('',#21320);
#5057=VERTEX_POINT('',#21363);
#5058=VERTEX_POINT('',#21364);
#5059=VERTEX_POINT('',#21384);
#5060=VERTEX_POINT('',#21386);
#5061=VERTEX_POINT('',#21388);
#5062=VERTEX_POINT('',#21390);
#5063=VERTEX_POINT('',#21392);
#5064=VERTEX_POINT('',#21394);
#5065=VERTEX_POINT('',#21479);
#5066=VERTEX_POINT('',#21480);
#5067=VERTEX_POINT('',#21482);
#5068=VERTEX_POINT('',#21484);
#5069=VERTEX_POINT('',#21498);
#5070=VERTEX_POINT('',#21533);
#5071=VERTEX_POINT('',#21547);
#5072=VERTEX_POINT('',#21549);
#5073=VERTEX_POINT('',#21556);
#5074=VERTEX_POINT('',#21557);
#5075=VERTEX_POINT('',#21566);
#5076=VERTEX_POINT('',#21568);
#5077=VERTEX_POINT('',#21579);
#5078=VERTEX_POINT('',#21580);
#5079=VERTEX_POINT('',#21582);
#5080=VERTEX_POINT('',#21617);
#5081=VERTEX_POINT('',#21619);
#5082=VERTEX_POINT('',#21656);
#5083=VERTEX_POINT('',#21657);
#5084=VERTEX_POINT('',#21665);
#5085=VERTEX_POINT('',#21667);
#5086=VERTEX_POINT('',#21671);
#5087=VERTEX_POINT('',#21673);
#5088=VERTEX_POINT('',#21680);
#5089=VERTEX_POINT('',#21682);
#5090=VERTEX_POINT('',#21686);
#5091=VERTEX_POINT('',#21687);
#5092=VERTEX_POINT('',#21692);
#5093=VERTEX_POINT('',#21693);
#5094=VERTEX_POINT('',#21695);
#5095=VERTEX_POINT('',#21697);
#5096=VERTEX_POINT('',#21701);
#5097=VERTEX_POINT('',#21702);
#5098=VERTEX_POINT('',#21704);
#5099=VERTEX_POINT('',#21714);
#5100=VERTEX_POINT('',#21715);
#5101=VERTEX_POINT('',#21717);
#5102=VERTEX_POINT('',#21719);
#5103=VERTEX_POINT('',#21723);
#5104=VERTEX_POINT('',#21730);
#5105=VERTEX_POINT('',#21732);
#5106=VERTEX_POINT('',#21736);
#5107=VERTEX_POINT('',#21738);
#5108=VERTEX_POINT('',#21742);
#5109=VERTEX_POINT('',#21743);
#5110=VERTEX_POINT('',#21745);
#5111=VERTEX_POINT('',#21747);
#5112=VERTEX_POINT('',#21751);
#5113=VERTEX_POINT('',#21752);
#5114=VERTEX_POINT('',#21754);
#5115=VERTEX_POINT('',#21756);
#5116=VERTEX_POINT('',#21758);
#5117=VERTEX_POINT('',#21760);
#5118=VERTEX_POINT('',#21762);
#5119=VERTEX_POINT('',#21764);
#5120=VERTEX_POINT('',#21767);
#5121=VERTEX_POINT('',#21778);
#5122=VERTEX_POINT('',#21779);
#5123=VERTEX_POINT('',#21781);
#5124=VERTEX_POINT('',#21831);
#5125=VERTEX_POINT('',#21833);
#5126=VERTEX_POINT('',#21835);
#5127=VERTEX_POINT('',#21844);
#5128=VERTEX_POINT('',#21848);
#5129=VERTEX_POINT('',#21850);
#5130=VERTEX_POINT('',#21852);
#5131=VERTEX_POINT('',#21887);
#5132=VERTEX_POINT('',#21889);
#5133=VERTEX_POINT('',#21893);
#5134=VERTEX_POINT('',#21894);
#5135=VERTEX_POINT('',#21897);
#5136=VERTEX_POINT('',#21899);
#5137=VERTEX_POINT('',#21901);
#5138=VERTEX_POINT('',#21932);
#5139=VERTEX_POINT('',#21933);
#5140=VERTEX_POINT('',#21935);
#5141=VERTEX_POINT('',#21952);
#5142=VERTEX_POINT('',#21996);
#5143=VERTEX_POINT('',#21998);
#5144=VERTEX_POINT('',#22000);
#5145=VERTEX_POINT('',#22058);
#5146=VERTEX_POINT('',#22059);
#5147=VERTEX_POINT('',#22061);
#5148=VERTEX_POINT('',#22063);
#5149=VERTEX_POINT('',#22065);
#5150=VERTEX_POINT('',#22067);
#5151=VERTEX_POINT('',#22069);
#5152=VERTEX_POINT('',#22071);
#5153=VERTEX_POINT('',#22075);
#5154=VERTEX_POINT('',#22076);
#5155=VERTEX_POINT('',#22078);
#5156=VERTEX_POINT('',#22080);
#5157=VERTEX_POINT('',#22082);
#5158=VERTEX_POINT('',#22085);
#5159=VERTEX_POINT('',#22095);
#5160=VERTEX_POINT('',#22096);
#5161=VERTEX_POINT('',#22105);
#5162=VERTEX_POINT('',#22107);
#5163=VERTEX_POINT('',#22118);
#5164=VERTEX_POINT('',#22119);
#5165=VERTEX_POINT('',#22127);
#5166=VERTEX_POINT('',#22129);
#5167=VERTEX_POINT('',#22133);
#5168=VERTEX_POINT('',#22135);
#5169=VERTEX_POINT('',#22142);
#5170=VERTEX_POINT('',#22144);
#5171=VERTEX_POINT('',#22151);
#5172=VERTEX_POINT('',#22152);
#5173=VERTEX_POINT('',#22154);
#5174=VERTEX_POINT('',#22156);
#5175=VERTEX_POINT('',#22160);
#5176=VERTEX_POINT('',#22170);
#5177=VERTEX_POINT('',#22171);
#5178=VERTEX_POINT('',#22173);
#5179=VERTEX_POINT('',#22175);
#5180=VERTEX_POINT('',#22179);
#5181=VERTEX_POINT('',#22180);
#5182=VERTEX_POINT('',#22182);
#5183=VERTEX_POINT('',#22189);
#5184=VERTEX_POINT('',#22191);
#5185=VERTEX_POINT('',#22195);
#5186=VERTEX_POINT('',#22196);
#5187=VERTEX_POINT('',#22201);
#5188=VERTEX_POINT('',#22202);
#5189=VERTEX_POINT('',#22208);
#5190=VERTEX_POINT('',#22210);
#5191=VERTEX_POINT('',#22212);
#5192=VERTEX_POINT('',#22214);
#5193=VERTEX_POINT('',#22216);
#5194=VERTEX_POINT('',#22218);
#5195=VERTEX_POINT('',#22314);
#5196=VERTEX_POINT('',#22321);
#5197=VERTEX_POINT('',#22412);
#5198=VERTEX_POINT('',#22543);
#5199=VERTEX_POINT('',#22636);
#5200=VERTEX_POINT('',#22746);
#5201=VERTEX_POINT('',#22747);
#5202=VERTEX_POINT('',#22824);
#5203=VERTEX_POINT('',#22917);
#5204=VERTEX_POINT('',#23067);
#5205=VERTEX_POINT('',#23135);
#5206=VERTEX_POINT('',#23142);
#5207=VERTEX_POINT('',#23233);
#5208=VERTEX_POINT('',#23364);
#5209=VERTEX_POINT('',#23457);
#5210=VERTEX_POINT('',#23567);
#5211=VERTEX_POINT('',#23568);
#5212=VERTEX_POINT('',#23645);
#5213=VERTEX_POINT('',#23738);
#5214=VERTEX_POINT('',#23888);
#5215=VERTEX_POINT('',#29491);
#5216=VERTEX_POINT('',#29498);
#5217=VERTEX_POINT('',#29591);
#5218=VERTEX_POINT('',#29741);
#5219=VERTEX_POINT('',#29832);
#5220=VERTEX_POINT('',#29951);
#5221=VERTEX_POINT('',#29952);
#5222=VERTEX_POINT('',#30029);
#5223=VERTEX_POINT('',#30122);
#5224=VERTEX_POINT('',#30272);
#5225=VERTEX_POINT('',#30340);
#5226=VERTEX_POINT('',#30347);
#5227=VERTEX_POINT('',#30438);
#5228=VERTEX_POINT('',#30569);
#5229=VERTEX_POINT('',#30662);
#5230=VERTEX_POINT('',#30772);
#5231=VERTEX_POINT('',#30773);
#5232=VERTEX_POINT('',#30850);
#5233=VERTEX_POINT('',#30943);
#5234=VERTEX_POINT('',#31132);
#5235=VERTEX_POINT('',#32152);
#5236=VERTEX_POINT('',#32160);
#5237=VERTEX_POINT('',#32168);
#5307=EDGE_CURVE('',#4301,#4301,#3413,.T.);
#5308=EDGE_CURVE('',#4301,#4302,#2537,.T.);
#5309=EDGE_CURVE('',#4302,#4302,#3414,.T.);
#5310=EDGE_CURVE('',#4303,#4303,#3415,.T.);
#5311=EDGE_CURVE('',#4303,#4304,#2538,.T.);
#5312=EDGE_CURVE('',#4304,#4304,#3416,.T.);
#5313=EDGE_CURVE('',#4305,#4305,#3417,.T.);
#5314=EDGE_CURVE('',#4305,#4306,#2539,.T.);
#5315=EDGE_CURVE('',#4306,#4306,#3418,.T.);
#5316=EDGE_CURVE('',#4307,#4307,#3419,.T.);
#5317=EDGE_CURVE('',#4307,#4308,#2540,.T.);
#5318=EDGE_CURVE('',#4308,#4308,#3420,.T.);
#5319=EDGE_CURVE('',#4309,#4310,#3421,.T.);
#5320=EDGE_CURVE('',#4310,#4309,#3422,.T.);
#5321=EDGE_CURVE('',#4310,#4311,#3423,.T.);
#5322=EDGE_CURVE('',#4311,#4311,#3424,.T.);
#5323=EDGE_CURVE('',#4312,#4312,#3425,.T.);
#5324=EDGE_CURVE('',#4312,#4313,#3426,.T.);
#5325=EDGE_CURVE('',#4314,#4313,#3427,.T.);
#5326=EDGE_CURVE('',#4313,#4314,#3428,.T.);
#5327=EDGE_CURVE('',#4315,#4315,#3429,.T.);
#5328=EDGE_CURVE('',#4315,#4316,#3430,.T.);
#5329=EDGE_CURVE('',#4316,#4316,#3431,.T.);
#5330=EDGE_CURVE('',#4317,#4317,#3432,.T.);
#5331=EDGE_CURVE('',#4317,#4318,#3433,.T.);
#5332=EDGE_CURVE('',#4319,#4318,#3434,.T.);
#5333=EDGE_CURVE('',#4318,#4319,#3435,.T.);
#5334=EDGE_CURVE('',#4320,#4321,#3436,.T.);
#5335=EDGE_CURVE('',#4320,#4322,#3437,.T.);
#5336=EDGE_CURVE('',#4323,#4322,#3438,.T.);
#5337=EDGE_CURVE('',#4321,#4323,#3439,.T.);
#5338=EDGE_CURVE('',#4324,#4325,#3440,.T.);
#5339=EDGE_CURVE('',#4326,#4324,#3441,.T.);
#5340=EDGE_CURVE('',#4327,#4326,#3442,.T.);
#5341=EDGE_CURVE('',#4325,#4327,#3443,.T.);
#5342=EDGE_CURVE('',#4328,#4329,#3444,.T.);
#5343=EDGE_CURVE('',#4330,#4328,#3445,.T.);
#5344=EDGE_CURVE('',#4331,#4330,#3446,.T.);
#5345=EDGE_CURVE('',#4331,#4329,#3447,.T.);
#5346=EDGE_CURVE('',#4332,#4333,#3448,.T.);
#5347=EDGE_CURVE('',#4334,#4332,#3449,.T.);
#5348=EDGE_CURVE('',#4335,#4334,#3450,.T.);
#5349=EDGE_CURVE('',#4333,#4335,#3451,.T.);
#5350=EDGE_CURVE('',#4336,#4337,#3452,.T.);
#5351=EDGE_CURVE('',#4337,#4336,#3453,.T.);
#5352=EDGE_CURVE('',#4337,#4338,#3454,.T.);
#5353=EDGE_CURVE('',#4338,#4338,#3455,.T.);
#5354=EDGE_CURVE('',#4339,#4339,#3456,.T.);
#5355=EDGE_CURVE('',#4339,#4340,#3457,.T.);
#5356=EDGE_CURVE('',#4341,#4340,#3458,.T.);
#5357=EDGE_CURVE('',#4340,#4341,#3459,.T.);
#5358=EDGE_CURVE('',#4342,#4342,#3460,.T.);
#5359=EDGE_CURVE('',#4342,#4343,#3461,.T.);
#5360=EDGE_CURVE('',#4344,#4343,#3462,.T.);
#5361=EDGE_CURVE('',#4343,#4344,#3463,.T.);
#5362=EDGE_CURVE('',#4345,#4345,#3464,.T.);
#5363=EDGE_CURVE('',#4345,#4346,#3465,.T.);
#5364=EDGE_CURVE('',#4347,#4346,#3466,.T.);
#5365=EDGE_CURVE('',#4346,#4347,#3467,.T.);
#5366=EDGE_CURVE('',#4348,#4349,#3468,.T.);
#5367=EDGE_CURVE('',#4350,#4348,#3469,.T.);
#5368=EDGE_CURVE('',#4351,#4350,#3470,.T.);
#5369=EDGE_CURVE('',#4351,#4349,#3471,.T.);
#5370=EDGE_CURVE('',#4352,#4353,#3472,.T.);
#5371=EDGE_CURVE('',#4354,#4352,#3473,.T.);
#5372=EDGE_CURVE('',#4355,#4354,#3474,.T.);
#5373=EDGE_CURVE('',#4353,#4355,#3475,.T.);
#5374=EDGE_CURVE('',#4356,#4357,#3476,.T.);
#5375=EDGE_CURVE('',#4356,#4358,#3477,.T.);
#5376=EDGE_CURVE('',#4359,#4358,#3478,.T.);
#5377=EDGE_CURVE('',#4357,#4359,#3479,.T.);
#5378=EDGE_CURVE('',#4360,#4361,#3480,.T.);
#5379=EDGE_CURVE('',#4362,#4360,#3481,.T.);
#5380=EDGE_CURVE('',#4363,#4362,#3482,.T.);
#5381=EDGE_CURVE('',#4361,#4363,#3483,.T.);
#5382=EDGE_CURVE('',#4364,#4364,#3484,.T.);
#5383=EDGE_CURVE('',#4364,#4365,#3485,.T.);
#5384=EDGE_CURVE('',#4365,#4365,#3486,.T.);
#5385=EDGE_CURVE('',#4366,#4366,#3487,.T.);
#5386=EDGE_CURVE('',#4366,#4367,#3488,.T.);
#5387=EDGE_CURVE('',#4367,#4367,#3489,.T.);
#5388=EDGE_CURVE('',#4368,#4368,#3490,.T.);
#5389=EDGE_CURVE('',#4368,#4369,#3491,.T.);
#5390=EDGE_CURVE('',#4370,#4369,#3492,.T.);
#5391=EDGE_CURVE('',#4369,#4370,#3493,.T.);
#5392=EDGE_CURVE('',#4371,#4371,#3494,.T.);
#5393=EDGE_CURVE('',#4371,#4372,#3495,.T.);
#5394=EDGE_CURVE('',#4372,#4372,#3496,.T.);
#5395=EDGE_CURVE('',#4373,#4374,#3497,.T.);
#5396=EDGE_CURVE('',#4373,#4375,#3498,.T.);
#5397=EDGE_CURVE('',#4376,#4375,#3499,.T.);
#5398=EDGE_CURVE('',#4374,#4376,#3500,.T.);
#5399=EDGE_CURVE('',#4377,#4378,#3501,.T.);
#5400=EDGE_CURVE('',#4379,#4377,#3502,.T.);
#5401=EDGE_CURVE('',#4380,#4379,#3503,.T.);
#5402=EDGE_CURVE('',#4380,#4378,#3504,.T.);
#5403=EDGE_CURVE('',#4381,#4382,#3505,.T.);
#5404=EDGE_CURVE('',#4381,#4383,#3506,.T.);
#5405=EDGE_CURVE('',#4383,#4383,#3507,.T.);
#5406=EDGE_CURVE('',#4382,#4381,#3508,.T.);
#5407=EDGE_CURVE('',#4384,#4384,#3509,.T.);
#5408=EDGE_CURVE('',#4384,#4385,#3510,.T.);
#5409=EDGE_CURVE('',#4386,#4385,#3511,.T.);
#5410=EDGE_CURVE('',#4385,#4386,#3512,.T.);
#5411=EDGE_CURVE('',#4387,#4387,#3513,.T.);
#5412=EDGE_CURVE('',#4387,#4388,#3514,.T.);
#5413=EDGE_CURVE('',#4389,#4388,#3515,.T.);
#5414=EDGE_CURVE('',#4388,#4389,#3516,.T.);
#5415=EDGE_CURVE('',#4390,#4390,#3517,.T.);
#5416=EDGE_CURVE('',#4390,#4391,#3518,.T.);
#5417=EDGE_CURVE('',#4392,#4391,#3519,.T.);
#5418=EDGE_CURVE('',#4391,#4392,#3520,.T.);
#5419=EDGE_CURVE('',#4393,#4394,#3521,.T.);
#5420=EDGE_CURVE('',#4395,#4393,#3522,.T.);
#5421=EDGE_CURVE('',#4396,#4395,#3523,.T.);
#5422=EDGE_CURVE('',#4396,#4394,#3524,.T.);
#5423=EDGE_CURVE('',#4397,#4398,#3525,.T.);
#5424=EDGE_CURVE('',#4399,#4397,#3526,.T.);
#5425=EDGE_CURVE('',#4400,#4399,#3527,.T.);
#5426=EDGE_CURVE('',#4400,#4398,#3528,.T.);
#5427=EDGE_CURVE('',#4401,#4402,#3529,.T.);
#5428=EDGE_CURVE('',#4401,#4403,#3530,.T.);
#5429=EDGE_CURVE('',#4404,#4403,#3531,.T.);
#5430=EDGE_CURVE('',#4402,#4404,#3532,.T.);
#5431=EDGE_CURVE('',#4405,#4406,#3533,.T.);
#5432=EDGE_CURVE('',#4407,#4405,#3534,.T.);
#5433=EDGE_CURVE('',#4408,#4407,#3535,.T.);
#5434=EDGE_CURVE('',#4408,#4406,#3536,.T.);
#5435=EDGE_CURVE('',#4409,#4410,#3537,.T.);
#5436=EDGE_CURVE('',#4411,#4409,#3538,.T.);
#5437=EDGE_CURVE('',#4412,#4411,#3539,.T.);
#5438=EDGE_CURVE('',#4412,#4410,#3540,.T.);
#5439=EDGE_CURVE('',#4413,#4414,#3541,.T.);
#5440=EDGE_CURVE('',#4413,#4415,#3542,.T.);
#5441=EDGE_CURVE('',#4416,#4415,#3543,.T.);
#5442=EDGE_CURVE('',#4414,#4416,#3544,.T.);
#5443=EDGE_CURVE('',#4417,#4418,#3545,.T.);
#5444=EDGE_CURVE('',#4419,#4417,#2541,.T.);
#5445=EDGE_CURVE('',#4419,#4420,#3546,.T.);
#5446=EDGE_CURVE('',#4418,#4420,#2542,.T.);
#5447=EDGE_CURVE('',#4421,#4422,#3547,.T.);
#5448=EDGE_CURVE('',#4423,#4421,#2543,.T.);
#5449=EDGE_CURVE('',#4423,#4424,#3548,.T.);
#5450=EDGE_CURVE('',#4422,#4424,#2544,.T.);
#5451=EDGE_CURVE('',#4425,#4426,#3549,.T.);
#5452=EDGE_CURVE('',#4427,#4426,#2545,.T.);
#5453=EDGE_CURVE('',#4428,#4427,#3550,.T.);
#5454=EDGE_CURVE('',#4425,#4428,#2546,.T.);
#5455=EDGE_CURVE('',#4425,#4429,#3551,.T.);
#5456=EDGE_CURVE('',#4430,#4429,#3552,.T.);
#5457=EDGE_CURVE('',#4426,#4430,#3553,.T.);
#5458=EDGE_CURVE('',#4431,#4432,#3554,.T.);
#5459=EDGE_CURVE('',#4433,#4432,#2547,.T.);
#5460=EDGE_CURVE('',#4434,#4433,#3555,.T.);
#5461=EDGE_CURVE('',#4431,#4434,#2548,.T.);
#5462=EDGE_CURVE('',#4435,#4436,#3556,.T.);
#5463=EDGE_CURVE('',#4437,#4435,#2549,.T.);
#5464=EDGE_CURVE('',#4437,#4438,#3557,.T.);
#5465=EDGE_CURVE('',#4436,#4438,#2550,.T.);
#5466=EDGE_CURVE('',#4439,#4440,#3558,.T.);
#5467=EDGE_CURVE('',#4441,#4440,#2551,.T.);
#5468=EDGE_CURVE('',#4442,#4441,#3559,.T.);
#5469=EDGE_CURVE('',#4439,#4442,#2552,.T.);
#5470=EDGE_CURVE('',#4443,#4444,#3560,.T.);
#5471=EDGE_CURVE('',#4445,#4443,#2553,.T.);
#5472=EDGE_CURVE('',#4445,#4446,#3561,.T.);
#5473=EDGE_CURVE('',#4444,#4446,#2554,.T.);
#5474=EDGE_CURVE('',#4447,#4448,#3562,.T.);
#5475=EDGE_CURVE('',#4447,#4449,#3563,.T.);
#5476=EDGE_CURVE('',#4450,#4449,#3564,.T.);
#5477=EDGE_CURVE('',#4450,#4448,#3565,.T.);
#5478=EDGE_CURVE('',#4451,#4452,#3566,.T.);
#5479=EDGE_CURVE('',#4453,#4451,#3567,.T.);
#5480=EDGE_CURVE('',#4454,#4453,#3568,.T.);
#5481=EDGE_CURVE('',#4454,#4452,#3569,.T.);
#5482=EDGE_CURVE('',#4455,#4456,#3570,.T.);
#5483=EDGE_CURVE('',#4455,#4457,#3571,.T.);
#5484=EDGE_CURVE('',#4458,#4457,#3572,.T.);
#5485=EDGE_CURVE('',#4456,#4458,#3573,.T.);
#5486=EDGE_CURVE('',#4459,#4460,#3574,.T.);
#5487=EDGE_CURVE('',#4461,#4460,#2555,.T.);
#5488=EDGE_CURVE('',#4461,#4462,#3575,.T.);
#5489=EDGE_CURVE('',#4459,#4462,#2556,.T.);
#5490=EDGE_CURVE('',#4463,#4454,#3576,.T.);
#5491=EDGE_CURVE('',#4454,#4457,#2557,.T.);
#5492=EDGE_CURVE('',#4457,#4464,#3577,.T.);
#5493=EDGE_CURVE('',#4464,#4463,#2558,.T.);
#5494=EDGE_CURVE('',#4382,#4392,#2559,.T.);
#5495=EDGE_CURVE('',#4389,#4386,#2560,.T.);
#5496=EDGE_CURVE('',#4465,#4403,#2561,.T.);
#5497=EDGE_CURVE('',#4465,#4466,#3578,.T.);
#5498=EDGE_CURVE('',#4404,#4466,#2562,.T.);
#5499=EDGE_CURVE('',#4467,#4468,#3579,.T.);
#5500=EDGE_CURVE('',#4469,#4468,#2563,.T.);
#5501=EDGE_CURVE('',#4469,#4470,#3580,.T.);
#5502=EDGE_CURVE('',#4467,#4470,#2564,.T.);
#5503=EDGE_CURVE('',#4375,#4471,#3581,.T.);
#5504=EDGE_CURVE('',#4471,#4472,#2565,.T.);
#5505=EDGE_CURVE('',#4472,#4380,#3582,.T.);
#5506=EDGE_CURVE('',#4380,#4375,#2566,.T.);
#5507=EDGE_CURVE('',#4364,#4372,#2567,.T.);
#5508=EDGE_CURVE('',#4370,#4367,#2568,.T.);
#5509=EDGE_CURVE('',#4395,#4473,#419,.T.);
#5510=EDGE_CURVE('',#4473,#4474,#3583,.T.);
#5511=EDGE_CURVE('',#4474,#4475,#420,.T.);
#5512=EDGE_CURVE('',#4475,#4476,#421,.T.);
#5513=EDGE_CURVE('',#4476,#4477,#3584,.T.);
#5514=EDGE_CURVE('',#4477,#4396,#422,.T.);
#5515=EDGE_CURVE('',#4478,#4407,#2569,.T.);
#5516=EDGE_CURVE('',#4478,#4479,#3585,.T.);
#5517=EDGE_CURVE('',#4408,#4479,#2570,.T.);
#5518=EDGE_CURVE('',#4480,#4481,#3586,.T.);
#5519=EDGE_CURVE('',#4482,#4481,#2571,.T.);
#5520=EDGE_CURVE('',#4482,#4483,#3587,.T.);
#5521=EDGE_CURVE('',#4480,#4483,#2572,.T.);
#5522=EDGE_CURVE('',#4353,#4360,#2573,.T.);
#5523=EDGE_CURVE('',#4361,#4352,#2574,.T.);
#5524=EDGE_CURVE('',#4336,#4347,#2575,.T.);
#5525=EDGE_CURVE('',#4344,#4341,#2576,.T.);
#5526=EDGE_CURVE('',#4484,#4485,#3588,.T.);
#5527=EDGE_CURVE('',#4485,#4486,#423,.T.);
#5528=EDGE_CURVE('',#4486,#4487,#3589,.T.);
#5529=EDGE_CURVE('',#4487,#4488,#424,.T.);
#5530=EDGE_CURVE('',#4488,#4489,#425,.T.);
#5531=EDGE_CURVE('',#4489,#4490,#3590,.T.);
#5532=EDGE_CURVE('',#4490,#4484,#426,.T.);
#5533=EDGE_CURVE('',#4491,#4492,#3591,.T.);
#5534=EDGE_CURVE('',#4416,#4492,#2577,.T.);
#5535=EDGE_CURVE('',#4491,#4415,#2578,.T.);
#5536=EDGE_CURVE('',#4331,#4322,#2579,.T.);
#5537=EDGE_CURVE('',#4323,#4330,#2580,.T.);
#5538=EDGE_CURVE('',#4325,#4332,#2581,.T.);
#5539=EDGE_CURVE('',#4333,#4324,#2582,.T.);
#5540=EDGE_CURVE('',#4493,#4494,#3592,.T.);
#5541=EDGE_CURVE('',#4493,#4495,#3593,.T.);
#5542=EDGE_CURVE('',#4496,#4495,#3594,.T.);
#5543=EDGE_CURVE('',#4497,#4496,#3595,.T.);
#5544=EDGE_CURVE('',#4497,#4498,#3596,.T.);
#5545=EDGE_CURVE('',#4499,#4498,#3597,.T.);
#5546=EDGE_CURVE('',#4499,#4500,#2583,.T.);
#5547=EDGE_CURVE('',#4501,#4500,#3598,.T.);
#5548=EDGE_CURVE('',#4501,#4502,#3599,.T.);
#5549=EDGE_CURVE('',#4503,#4502,#427,.T.);
#5550=EDGE_CURVE('',#4503,#4504,#2584,.T.);
#5551=EDGE_CURVE('',#4504,#4505,#3600,.T.);
#5552=EDGE_CURVE('',#4505,#4506,#2585,.T.);
#5553=EDGE_CURVE('',#4507,#4506,#428,.T.);
#5554=EDGE_CURVE('',#4507,#4508,#3601,.T.);
#5555=EDGE_CURVE('',#4509,#4508,#429,.T.);
#5556=EDGE_CURVE('',#4509,#4510,#2586,.T.);
#5557=EDGE_CURVE('',#4510,#4433,#3602,.T.);
#5558=EDGE_CURVE('',#4432,#4511,#430,.T.);
#5559=EDGE_CURVE('',#4511,#4512,#3603,.T.);
#5560=EDGE_CURVE('',#4513,#4512,#3604,.T.);
#5561=EDGE_CURVE('',#4514,#4513,#3605,.T.);
#5562=EDGE_CURVE('',#4514,#4515,#3606,.T.);
#5563=EDGE_CURVE('',#4516,#4515,#431,.T.);
#5564=EDGE_CURVE('',#4516,#4517,#2587,.T.);
#5565=EDGE_CURVE('',#4517,#4437,#3607,.T.);
#5566=EDGE_CURVE('',#4518,#4435,#432,.T.);
#5567=EDGE_CURVE('',#4518,#4519,#3608,.T.);
#5568=EDGE_CURVE('',#4520,#4519,#433,.T.);
#5569=EDGE_CURVE('',#4520,#4521,#2588,.T.);
#5570=EDGE_CURVE('',#4521,#4522,#3609,.T.);
#5571=EDGE_CURVE('',#4522,#4523,#2589,.T.);
#5572=EDGE_CURVE('',#4523,#4524,#434,.T.);
#5573=EDGE_CURVE('',#4524,#4525,#3610,.T.);
#5574=EDGE_CURVE('',#4526,#4525,#3611,.T.);
#5575=EDGE_CURVE('',#4527,#4526,#3612,.T.);
#5576=EDGE_CURVE('',#4527,#4528,#3613,.T.);
#5577=EDGE_CURVE('',#4529,#4528,#435,.T.);
#5578=EDGE_CURVE('',#4529,#4530,#2590,.T.);
#5579=EDGE_CURVE('',#4530,#4531,#3614,.T.);
#5580=EDGE_CURVE('',#4531,#4532,#2591,.T.);
#5581=EDGE_CURVE('',#4533,#4532,#436,.T.);
#5582=EDGE_CURVE('',#4533,#4534,#3615,.T.);
#5583=EDGE_CURVE('',#4444,#4534,#437,.T.);
#5584=EDGE_CURVE('',#4446,#4535,#3616,.T.);
#5585=EDGE_CURVE('',#4535,#4536,#2592,.T.);
#5586=EDGE_CURVE('',#4536,#4537,#438,.T.);
#5587=EDGE_CURVE('',#4537,#4538,#3617,.T.);
#5588=EDGE_CURVE('',#4539,#4538,#3618,.T.);
#5589=EDGE_CURVE('',#4540,#4539,#3619,.T.);
#5590=EDGE_CURVE('',#4540,#4541,#3620,.T.);
#5591=EDGE_CURVE('',#4439,#4541,#439,.T.);
#5592=EDGE_CURVE('',#4442,#4542,#3621,.T.);
#5593=EDGE_CURVE('',#4542,#4543,#2593,.T.);
#5594=EDGE_CURVE('',#4544,#4543,#440,.T.);
#5595=EDGE_CURVE('',#4544,#4545,#3622,.T.);
#5596=EDGE_CURVE('',#4546,#4545,#441,.T.);
#5597=EDGE_CURVE('',#4546,#4547,#2594,.T.);
#5598=EDGE_CURVE('',#4547,#4548,#3623,.T.);
#5599=EDGE_CURVE('',#4548,#4549,#2595,.T.);
#5600=EDGE_CURVE('',#4549,#4550,#442,.T.);
#5601=EDGE_CURVE('',#4550,#4551,#3624,.T.);
#5602=EDGE_CURVE('',#4500,#4551,#3625,.T.);
#5603=EDGE_CURVE('',#4552,#4499,#3626,.T.);
#5604=EDGE_CURVE('',#4552,#4553,#3627,.T.);
#5605=EDGE_CURVE('',#4554,#4553,#3628,.T.);
#5606=EDGE_CURVE('',#4555,#4554,#3629,.T.);
#5607=EDGE_CURVE('',#4555,#4556,#3630,.T.);
#5608=EDGE_CURVE('',#4494,#4556,#3631,.T.);
#5609=EDGE_CURVE('',#4309,#4319,#2596,.T.);
#5610=EDGE_CURVE('',#4316,#4314,#2597,.T.);
#5611=EDGE_CURVE('',#4557,#4558,#3632,.T.);
#5612=EDGE_CURVE('',#4558,#4559,#443,.T.);
#5613=EDGE_CURVE('',#4559,#4560,#3633,.T.);
#5614=EDGE_CURVE('',#4560,#4561,#444,.T.);
#5615=EDGE_CURVE('',#4561,#4562,#445,.T.);
#5616=EDGE_CURVE('',#4562,#4563,#3634,.T.);
#5617=EDGE_CURVE('',#4563,#4557,#446,.T.);
#5618=EDGE_CURVE('',#4564,#4565,#3635,.T.);
#5619=EDGE_CURVE('',#4412,#4565,#2598,.T.);
#5620=EDGE_CURVE('',#4564,#4411,#2599,.T.);
#5621=EDGE_CURVE('',#4566,#4567,#3636,.T.);
#5622=EDGE_CURVE('',#4566,#4568,#2600,.T.);
#5623=EDGE_CURVE('',#4568,#4569,#3637,.T.);
#5624=EDGE_CURVE('',#4567,#4569,#2601,.T.);
#5625=EDGE_CURVE('',#4570,#4571,#2602,.T.);
#5626=EDGE_CURVE('',#4572,#4571,#2603,.T.);
#5627=EDGE_CURVE('',#4573,#4572,#2604,.T.);
#5628=EDGE_CURVE('',#4573,#4377,#2605,.T.);
#5629=EDGE_CURVE('',#4378,#4574,#3638,.T.);
#5630=EDGE_CURVE('',#4574,#4575,#3639,.T.);
#5631=EDGE_CURVE('',#4575,#4576,#2606,.T.);
#5632=EDGE_CURVE('',#4576,#4577,#3640,.T.);
#5633=EDGE_CURVE('',#4577,#4578,#3641,.T.);
#5634=EDGE_CURVE('',#4578,#4579,#3642,.T.);
#5635=EDGE_CURVE('',#4579,#4580,#2607,.T.);
#5636=EDGE_CURVE('',#4581,#4580,#2608,.T.);
#5637=EDGE_CURVE('',#4581,#4582,#2609,.T.);
#5638=EDGE_CURVE('',#4582,#4583,#2610,.T.);
#5639=EDGE_CURVE('',#4583,#4584,#3643,.T.);
#5640=EDGE_CURVE('',#4584,#4585,#2611,.T.);
#5641=EDGE_CURVE('',#4585,#4586,#3644,.T.);
#5642=EDGE_CURVE('',#4586,#4587,#2612,.T.);
#5643=EDGE_CURVE('',#4587,#4588,#3645,.T.);
#5644=EDGE_CURVE('',#4588,#4589,#2613,.T.);
#5645=EDGE_CURVE('',#4589,#4570,#3646,.T.);
#5646=EDGE_CURVE('',#4590,#4591,#3647,.T.);
#5647=EDGE_CURVE('',#4591,#4592,#3648,.T.);
#5648=EDGE_CURVE('',#4592,#4593,#2614,.T.);
#5649=EDGE_CURVE('',#4593,#4594,#3649,.T.);
#5650=EDGE_CURVE('',#4594,#4455,#3650,.T.);
#5651=EDGE_CURVE('',#4456,#4595,#2615,.T.);
#5652=EDGE_CURVE('',#4595,#4590,#3651,.T.);
#5653=EDGE_CURVE('',#4357,#4596,#3652,.T.);
#5654=EDGE_CURVE('',#4596,#4597,#3653,.T.);
#5655=EDGE_CURVE('',#4597,#4598,#2616,.T.);
#5656=EDGE_CURVE('',#4598,#4363,#3654,.T.);
#5657=EDGE_CURVE('',#4362,#4599,#3655,.T.);
#5658=EDGE_CURVE('',#4599,#4356,#2617,.T.);
#5659=EDGE_CURVE('',#4600,#4328,#3656,.T.);
#5660=EDGE_CURVE('',#4329,#4601,#2618,.T.);
#5661=EDGE_CURVE('',#4601,#4335,#3657,.T.);
#5662=EDGE_CURVE('',#4334,#4602,#3658,.T.);
#5663=EDGE_CURVE('',#4602,#4603,#2619,.T.);
#5664=EDGE_CURVE('',#4603,#4600,#3659,.T.);
#5665=EDGE_CURVE('',#4604,#4605,#447,.T.);
#5666=EDGE_CURVE('',#4604,#4606,#3660,.T.);
#5667=EDGE_CURVE('',#4607,#4606,#448,.T.);
#5668=EDGE_CURVE('',#4607,#4608,#2620,.T.);
#5669=EDGE_CURVE('',#4609,#4608,#449,.T.);
#5670=EDGE_CURVE('',#4609,#4610,#3661,.T.);
#5671=EDGE_CURVE('',#4611,#4610,#450,.T.);
#5672=EDGE_CURVE('',#4611,#4612,#2621,.T.);
#5673=EDGE_CURVE('',#4613,#4612,#451,.T.);
#5674=EDGE_CURVE('',#4613,#4614,#3662,.T.);
#5675=EDGE_CURVE('',#4615,#4614,#452,.T.);
#5676=EDGE_CURVE('',#4615,#4616,#2622,.T.);
#5677=EDGE_CURVE('',#4617,#4616,#453,.T.);
#5678=EDGE_CURVE('',#4617,#4618,#3663,.T.);
#5679=EDGE_CURVE('',#4619,#4618,#454,.T.);
#5680=EDGE_CURVE('',#4619,#4605,#2623,.T.);
#5681=EDGE_CURVE('',#4620,#4621,#2624,.T.);
#5682=EDGE_CURVE('',#4620,#4622,#2625,.T.);
#5683=EDGE_CURVE('',#4622,#4623,#2626,.T.);
#5684=EDGE_CURVE('',#4623,#4621,#2627,.T.);
#5685=EDGE_CURVE('',#4624,#4625,#2628,.T.);
#5686=EDGE_CURVE('',#4624,#4626,#2629,.T.);
#5687=EDGE_CURVE('',#4626,#4627,#2630,.T.);
#5688=EDGE_CURVE('',#4627,#4625,#2631,.T.);
#5689=EDGE_CURVE('',#4628,#4629,#2632,.T.);
#5690=EDGE_CURVE('',#4630,#4629,#2633,.T.);
#5691=EDGE_CURVE('',#4631,#4630,#2634,.T.);
#5692=EDGE_CURVE('',#4632,#4631,#2635,.T.);
#5693=EDGE_CURVE('',#4633,#4632,#2636,.T.);
#5694=EDGE_CURVE('',#4633,#4634,#2637,.T.);
#5695=EDGE_CURVE('',#4634,#4635,#2638,.T.);
#5696=EDGE_CURVE('',#4635,#4636,#3664,.T.);
#5697=EDGE_CURVE('',#4636,#4637,#2639,.T.);
#5698=EDGE_CURVE('',#4637,#4638,#3665,.T.);
#5699=EDGE_CURVE('',#4638,#4639,#2640,.T.);
#5700=EDGE_CURVE('',#4639,#4640,#3666,.T.);
#5701=EDGE_CURVE('',#4640,#4641,#2641,.T.);
#5702=EDGE_CURVE('',#4641,#4642,#3667,.T.);
#5703=EDGE_CURVE('',#4642,#4643,#2642,.T.);
#5704=EDGE_CURVE('',#4644,#4643,#2643,.T.);
#5705=EDGE_CURVE('',#4645,#4644,#2644,.T.);
#5706=EDGE_CURVE('',#4628,#4645,#2645,.T.);
#5707=EDGE_CURVE('',#4646,#4647,#2646,.T.);
#5708=EDGE_CURVE('',#4646,#4648,#2647,.T.);
#5709=EDGE_CURVE('',#4648,#4649,#3668,.T.);
#5710=EDGE_CURVE('',#4649,#4650,#2648,.T.);
#5711=EDGE_CURVE('',#4650,#4651,#3669,.T.);
#5712=EDGE_CURVE('',#4651,#4405,#2649,.T.);
#5713=EDGE_CURVE('',#4406,#4652,#2650,.T.);
#5714=EDGE_CURVE('',#4652,#4653,#3670,.T.);
#5715=EDGE_CURVE('',#4653,#4654,#2651,.T.);
#5716=EDGE_CURVE('',#4654,#4655,#2652,.T.);
#5717=EDGE_CURVE('',#4656,#4655,#2653,.T.);
#5718=EDGE_CURVE('',#4656,#4657,#2654,.T.);
#5719=EDGE_CURVE('',#4657,#4658,#2655,.T.);
#5720=EDGE_CURVE('',#4659,#4658,#2656,.T.);
#5721=EDGE_CURVE('',#4647,#4659,#2657,.T.);
#5722=EDGE_CURVE('',#4660,#4661,#2658,.T.);
#5723=EDGE_CURVE('',#4660,#4376,#2659,.T.);
#5724=EDGE_CURVE('',#4376,#4379,#2660,.T.);
#5725=EDGE_CURVE('',#4379,#4661,#2661,.T.);
#5726=EDGE_CURVE('',#4646,#4625,#3671,.T.);
#5727=EDGE_CURVE('',#4648,#4627,#3672,.T.);
#5728=EDGE_CURVE('',#4620,#4643,#3673,.T.);
#5729=EDGE_CURVE('',#4622,#4642,#3674,.T.);
#5730=EDGE_CURVE('',#4662,#4663,#2662,.T.);
#5731=EDGE_CURVE('',#4662,#4621,#3675,.T.);
#5732=EDGE_CURVE('',#4663,#4623,#3676,.T.);
#5733=EDGE_CURVE('',#4624,#4571,#3677,.T.);
#5734=EDGE_CURVE('',#4626,#4570,#3678,.T.);
#5735=EDGE_CURVE('',#4573,#4661,#3679,.T.);
#5736=EDGE_CURVE('',#4664,#4660,#3680,.T.);
#5737=EDGE_CURVE('',#4374,#4664,#2663,.T.);
#5738=EDGE_CURVE('',#4665,#4666,#2664,.T.);
#5739=EDGE_CURVE('',#4666,#4667,#2665,.T.);
#5740=EDGE_CURVE('',#4667,#4668,#2666,.T.);
#5741=EDGE_CURVE('',#4668,#4665,#2667,.T.);
#5742=EDGE_CURVE('',#4669,#4667,#3681,.T.);
#5743=EDGE_CURVE('',#4670,#4669,#2668,.T.);
#5744=EDGE_CURVE('',#4668,#4670,#3682,.T.);
#5745=EDGE_CURVE('',#4666,#4671,#3683,.T.);
#5746=EDGE_CURVE('',#4665,#4672,#3684,.T.);
#5747=EDGE_CURVE('',#4671,#4672,#2669,.T.);
#5748=EDGE_CURVE('',#4673,#4674,#2670,.T.);
#5749=EDGE_CURVE('',#4674,#4675,#3685,.T.);
#5750=EDGE_CURVE('',#4675,#4676,#3686,.T.);
#5751=EDGE_CURVE('',#4677,#4676,#2671,.T.);
#5752=EDGE_CURVE('',#4673,#4677,#2672,.T.);
#5753=EDGE_CURVE('',#4678,#4679,#264,.T.);
#5754=EDGE_CURVE('',#4680,#4678,#265,.T.);
#5755=EDGE_CURVE('',#4680,#4681,#455,.T.);
#5756=EDGE_CURVE('',#4681,#4682,#2673,.T.);
#5757=EDGE_CURVE('',#4682,#4679,#456,.T.);
#5758=EDGE_CURVE('',#4683,#4684,#266,.T.);
#5759=EDGE_CURVE('',#4685,#4683,#267,.T.);
#5760=EDGE_CURVE('',#4685,#4686,#457,.T.);
#5761=EDGE_CURVE('',#4686,#4687,#2674,.T.);
#5762=EDGE_CURVE('',#4687,#4684,#458,.T.);
#5763=EDGE_CURVE('',#4688,#4689,#268,.T.);
#5764=EDGE_CURVE('',#4690,#4688,#269,.T.);
#5765=EDGE_CURVE('',#4690,#4691,#459,.T.);
#5766=EDGE_CURVE('',#4691,#4692,#2675,.T.);
#5767=EDGE_CURVE('',#4692,#4689,#460,.T.);
#5768=EDGE_CURVE('',#4693,#4694,#270,.T.);
#5769=EDGE_CURVE('',#4695,#4693,#271,.T.);
#5770=EDGE_CURVE('',#4695,#4696,#461,.T.);
#5771=EDGE_CURVE('',#4696,#4697,#2676,.T.);
#5772=EDGE_CURVE('',#4697,#4694,#462,.T.);
#5773=EDGE_CURVE('',#4698,#4699,#3687,.T.);
#5774=EDGE_CURVE('',#4699,#4700,#463,.T.);
#5775=EDGE_CURVE('',#4700,#4701,#272,.T.);
#5776=EDGE_CURVE('',#4701,#4702,#3688,.T.);
#5777=EDGE_CURVE('',#4702,#4703,#464,.T.);
#5778=EDGE_CURVE('',#4703,#4704,#3689,.T.);
#5779=EDGE_CURVE('',#4704,#4698,#3690,.T.);
#5780=EDGE_CURVE('',#4705,#4706,#2677,.T.);
#5781=EDGE_CURVE('',#4671,#4705,#2678,.T.);
#5782=EDGE_CURVE('',#4672,#4707,#3691,.T.);
#5783=EDGE_CURVE('',#4707,#4708,#3692,.T.);
#5784=EDGE_CURVE('',#4708,#4709,#2679,.T.);
#5785=EDGE_CURVE('',#4709,#4710,#3693,.T.);
#5786=EDGE_CURVE('',#4710,#4711,#2680,.T.);
#5787=EDGE_CURVE('',#4711,#4712,#3694,.T.);
#5788=EDGE_CURVE('',#4712,#4713,#3695,.T.);
#5789=EDGE_CURVE('',#4713,#4714,#2681,.T.);
#5790=EDGE_CURVE('',#4714,#4715,#3696,.T.);
#5791=EDGE_CURVE('',#4715,#4716,#2682,.T.);
#5792=EDGE_CURVE('',#4716,#4717,#3697,.T.);
#5793=EDGE_CURVE('',#4717,#4718,#3698,.T.);
#5794=EDGE_CURVE('',#4718,#4719,#2683,.T.);
#5795=EDGE_CURVE('',#4719,#4720,#3699,.T.);
#5796=EDGE_CURVE('',#4720,#4430,#2684,.T.);
#5797=EDGE_CURVE('',#4429,#4721,#3700,.T.);
#5798=EDGE_CURVE('',#4721,#4722,#2685,.T.);
#5799=EDGE_CURVE('',#4722,#4723,#3701,.T.);
#5800=EDGE_CURVE('',#4723,#4724,#2686,.T.);
#5801=EDGE_CURVE('',#4569,#4724,#2687,.T.);
#5802=EDGE_CURVE('',#4568,#4725,#2688,.T.);
#5803=EDGE_CURVE('',#4726,#4725,#3702,.T.);
#5804=EDGE_CURVE('',#4726,#4706,#3703,.T.);
#5805=EDGE_CURVE('',#4727,#4728,#2689,.T.);
#5806=EDGE_CURVE('',#4728,#4436,#2690,.T.);
#5807=EDGE_CURVE('',#4729,#4438,#465,.T.);
#5808=EDGE_CURVE('',#4729,#4730,#2691,.T.);
#5809=EDGE_CURVE('',#4730,#4731,#3704,.T.);
#5810=EDGE_CURVE('',#4731,#4727,#2692,.T.);
#5811=EDGE_CURVE('',#4732,#4733,#2693,.T.);
#5812=EDGE_CURVE('',#4733,#4734,#2694,.T.);
#5813=EDGE_CURVE('',#4734,#4735,#2695,.T.);
#5814=EDGE_CURVE('',#4735,#4736,#2696,.T.);
#5815=EDGE_CURVE('',#4736,#4737,#3705,.T.);
#5816=EDGE_CURVE('',#4737,#4738,#2697,.T.);
#5817=EDGE_CURVE('',#4732,#4738,#466,.T.);
#5818=EDGE_CURVE('',#4739,#4740,#3706,.T.);
#5819=EDGE_CURVE('',#4740,#4741,#467,.T.);
#5820=EDGE_CURVE('',#4742,#4741,#468,.T.);
#5821=EDGE_CURVE('',#4742,#4743,#3707,.T.);
#5822=EDGE_CURVE('',#4743,#4744,#3708,.T.);
#5823=EDGE_CURVE('',#4744,#4745,#3709,.T.);
#5824=EDGE_CURVE('',#4745,#4739,#469,.T.);
#5825=EDGE_CURVE('',#4746,#4747,#470,.T.);
#5826=EDGE_CURVE('',#4747,#4748,#3710,.T.);
#5827=EDGE_CURVE('',#4748,#4749,#471,.T.);
#5828=EDGE_CURVE('',#4749,#4750,#3711,.T.);
#5829=EDGE_CURVE('',#4750,#4751,#472,.T.);
#5830=EDGE_CURVE('',#4751,#4746,#3712,.T.);
#5831=EDGE_CURVE('',#4752,#4753,#2698,.T.);
#5832=EDGE_CURVE('',#4753,#4754,#3713,.T.);
#5833=EDGE_CURVE('',#4754,#4755,#2699,.T.);
#5834=EDGE_CURVE('',#4755,#4752,#3714,.T.);
#5835=EDGE_CURVE('',#4420,#4423,#3715,.T.);
#5836=EDGE_CURVE('',#4421,#4418,#3716,.T.);
#5837=EDGE_CURVE('',#4756,#4757,#2700,.T.);
#5838=EDGE_CURVE('',#4757,#4758,#3717,.T.);
#5839=EDGE_CURVE('',#4758,#4759,#2701,.T.);
#5840=EDGE_CURVE('',#4759,#4760,#3718,.T.);
#5841=EDGE_CURVE('',#4760,#4761,#473,.T.);
#5842=EDGE_CURVE('',#4761,#4756,#3719,.T.);
#5843=EDGE_CURVE('',#4762,#4763,#2702,.T.);
#5844=EDGE_CURVE('',#4763,#4764,#3720,.T.);
#5845=EDGE_CURVE('',#4764,#4765,#2703,.T.);
#5846=EDGE_CURVE('',#4765,#4766,#3721,.T.);
#5847=EDGE_CURVE('',#4766,#4767,#474,.T.);
#5848=EDGE_CURVE('',#4767,#4762,#3722,.T.);
#5849=EDGE_CURVE('',#4768,#4769,#2704,.T.);
#5850=EDGE_CURVE('',#4769,#4770,#3723,.T.);
#5851=EDGE_CURVE('',#4770,#4771,#2705,.T.);
#5852=EDGE_CURVE('',#4771,#4772,#3724,.T.);
#5853=EDGE_CURVE('',#4772,#4409,#2706,.T.);
#5854=EDGE_CURVE('',#4410,#4773,#2707,.T.);
#5855=EDGE_CURVE('',#4773,#4768,#3725,.T.);
#5856=EDGE_CURVE('',#4774,#4775,#2708,.T.);
#5857=EDGE_CURVE('',#4775,#4776,#3726,.T.);
#5858=EDGE_CURVE('',#4776,#4777,#2709,.T.);
#5859=EDGE_CURVE('',#4777,#4778,#3727,.T.);
#5860=EDGE_CURVE('',#4778,#4779,#2710,.T.);
#5861=EDGE_CURVE('',#4779,#4780,#3728,.T.);
#5862=EDGE_CURVE('',#4780,#4781,#2711,.T.);
#5863=EDGE_CURVE('',#4781,#4774,#3729,.T.);
#5864=EDGE_CURVE('',#4782,#4783,#475,.T.);
#5865=EDGE_CURVE('',#4782,#4784,#2712,.T.);
#5866=EDGE_CURVE('',#4784,#4785,#2713,.T.);
#5867=EDGE_CURVE('',#4785,#4786,#2714,.T.);
#5868=EDGE_CURVE('',#4787,#4786,#2715,.T.);
#5869=EDGE_CURVE('',#4787,#4788,#2716,.T.);
#5870=EDGE_CURVE('',#4789,#4788,#476,.T.);
#5871=EDGE_CURVE('',#4789,#4783,#477,.T.);
#5872=EDGE_CURVE('',#4790,#4791,#2717,.T.);
#5873=EDGE_CURVE('',#4790,#4792,#2718,.T.);
#5874=EDGE_CURVE('',#4793,#4792,#478,.T.);
#5875=EDGE_CURVE('',#4793,#4794,#479,.T.);
#5876=EDGE_CURVE('',#4795,#4794,#480,.T.);
#5877=EDGE_CURVE('',#4795,#4796,#2719,.T.);
#5878=EDGE_CURVE('',#4796,#4797,#2720,.T.);
#5879=EDGE_CURVE('',#4797,#4791,#2721,.T.);
#5880=EDGE_CURVE('',#4796,#4787,#3730,.T.);
#5881=EDGE_CURVE('',#4786,#4797,#3731,.T.);
#5882=EDGE_CURVE('',#4798,#4799,#2722,.T.);
#5883=EDGE_CURVE('',#4799,#4800,#2723,.T.);
#5884=EDGE_CURVE('',#4801,#4800,#481,.T.);
#5885=EDGE_CURVE('',#4801,#4802,#482,.T.);
#5886=EDGE_CURVE('',#4803,#4802,#483,.T.);
#5887=EDGE_CURVE('',#4803,#4804,#2724,.T.);
#5888=EDGE_CURVE('',#4805,#4804,#2725,.T.);
#5889=EDGE_CURVE('',#4805,#4798,#2726,.T.);
#5890=EDGE_CURVE('',#4806,#4807,#484,.T.);
#5891=EDGE_CURVE('',#4806,#4808,#2727,.T.);
#5892=EDGE_CURVE('',#4809,#4808,#2728,.T.);
#5893=EDGE_CURVE('',#4809,#4810,#2729,.T.);
#5894=EDGE_CURVE('',#4810,#4811,#2730,.T.);
#5895=EDGE_CURVE('',#4811,#4812,#2731,.T.);
#5896=EDGE_CURVE('',#4813,#4812,#485,.T.);
#5897=EDGE_CURVE('',#4813,#4807,#486,.T.);
#5898=EDGE_CURVE('',#4814,#4815,#2732,.T.);
#5899=EDGE_CURVE('',#4816,#4815,#2733,.T.);
#5900=EDGE_CURVE('',#4817,#4816,#2734,.T.);
#5901=EDGE_CURVE('',#4818,#4817,#2735,.T.);
#5902=EDGE_CURVE('',#4818,#4819,#2736,.T.);
#5903=EDGE_CURVE('',#4819,#4820,#2737,.T.);
#5904=EDGE_CURVE('',#4821,#4820,#487,.T.);
#5905=EDGE_CURVE('',#4821,#4822,#3732,.T.);
#5906=EDGE_CURVE('',#4823,#4822,#488,.T.);
#5907=EDGE_CURVE('',#4823,#4824,#2738,.T.);
#5908=EDGE_CURVE('',#4825,#4824,#489,.T.);
#5909=EDGE_CURVE('',#4825,#4826,#3733,.T.);
#5910=EDGE_CURVE('',#4826,#4827,#490,.T.);
#5911=EDGE_CURVE('',#4827,#4828,#2739,.T.);
#5912=EDGE_CURVE('',#4828,#4829,#3734,.T.);
#5913=EDGE_CURVE('',#4829,#4670,#3735,.T.);
#5914=EDGE_CURVE('',#4669,#4830,#2740,.T.);
#5915=EDGE_CURVE('',#4830,#4831,#2741,.T.);
#5916=EDGE_CURVE('',#4832,#4831,#2742,.T.);
#5917=EDGE_CURVE('',#4832,#4833,#2743,.T.);
#5918=EDGE_CURVE('',#4833,#4834,#2744,.T.);
#5919=EDGE_CURVE('',#4834,#4662,#2745,.T.);
#5920=EDGE_CURVE('',#4663,#4835,#3736,.T.);
#5921=EDGE_CURVE('',#4835,#4836,#2746,.T.);
#5922=EDGE_CURVE('',#4836,#4837,#3737,.T.);
#5923=EDGE_CURVE('',#4837,#4838,#2747,.T.);
#5924=EDGE_CURVE('',#4838,#4839,#3738,.T.);
#5925=EDGE_CURVE('',#4839,#4840,#2748,.T.);
#5926=EDGE_CURVE('',#4840,#4814,#3739,.T.);
#5927=EDGE_CURVE('',#4841,#4842,#3740,.T.);
#5928=EDGE_CURVE('',#4842,#4843,#491,.T.);
#5929=EDGE_CURVE('',#4843,#4844,#2749,.T.);
#5930=EDGE_CURVE('',#4844,#4845,#3741,.T.);
#5931=EDGE_CURVE('',#4845,#4846,#3742,.T.);
#5932=EDGE_CURVE('',#4846,#4847,#2750,.T.);
#5933=EDGE_CURVE('',#4848,#4847,#492,.T.);
#5934=EDGE_CURVE('',#4848,#4849,#3743,.T.);
#5935=EDGE_CURVE('',#4850,#4849,#493,.T.);
#5936=EDGE_CURVE('',#4850,#4851,#2751,.T.);
#5937=EDGE_CURVE('',#4841,#4851,#494,.T.);
#5938=EDGE_CURVE('',#4852,#4853,#3744,.T.);
#5939=EDGE_CURVE('',#4853,#4854,#495,.T.);
#5940=EDGE_CURVE('',#4854,#4855,#2752,.T.);
#5941=EDGE_CURVE('',#4855,#4450,#3745,.T.);
#5942=EDGE_CURVE('',#4449,#4856,#2753,.T.);
#5943=EDGE_CURVE('',#4857,#4856,#496,.T.);
#5944=EDGE_CURVE('',#4857,#4858,#3746,.T.);
#5945=EDGE_CURVE('',#4859,#4858,#497,.T.);
#5946=EDGE_CURVE('',#4859,#4860,#2754,.T.);
#5947=EDGE_CURVE('',#4852,#4860,#498,.T.);
#5948=EDGE_CURVE('',#4861,#4862,#3747,.T.);
#5949=EDGE_CURVE('',#4862,#4863,#3748,.T.);
#5950=EDGE_CURVE('',#4863,#4864,#2755,.T.);
#5951=EDGE_CURVE('',#4865,#4864,#499,.T.);
#5952=EDGE_CURVE('',#4865,#4866,#3749,.T.);
#5953=EDGE_CURVE('',#4867,#4866,#500,.T.);
#5954=EDGE_CURVE('',#4867,#4868,#2756,.T.);
#5955=EDGE_CURVE('',#4869,#4868,#501,.T.);
#5956=EDGE_CURVE('',#4869,#4870,#3750,.T.);
#5957=EDGE_CURVE('',#4870,#4871,#502,.T.);
#5958=EDGE_CURVE('',#4871,#4861,#2757,.T.);
#5959=EDGE_CURVE('',#4804,#4811,#3751,.T.);
#5960=EDGE_CURVE('',#4810,#4805,#3752,.T.);
#5961=EDGE_CURVE('',#4872,#4873,#503,.T.);
#5962=EDGE_CURVE('',#4873,#4874,#3753,.T.);
#5963=EDGE_CURVE('',#4874,#4875,#504,.T.);
#5964=EDGE_CURVE('',#4875,#4872,#3754,.T.);
#5965=EDGE_CURVE('',#4876,#4877,#273,.T.);
#5966=EDGE_CURVE('',#4876,#4878,#505,.T.);
#5967=EDGE_CURVE('',#4878,#4879,#2758,.T.);
#5968=EDGE_CURVE('',#4879,#4880,#506,.T.);
#5969=EDGE_CURVE('',#4877,#4880,#274,.T.);
#5970=EDGE_CURVE('',#4881,#4882,#275,.T.);
#5971=EDGE_CURVE('',#4881,#4883,#507,.T.);
#5972=EDGE_CURVE('',#4883,#4884,#2759,.T.);
#5973=EDGE_CURVE('',#4884,#4885,#508,.T.);
#5974=EDGE_CURVE('',#4882,#4885,#276,.T.);
#5975=EDGE_CURVE('',#4417,#4886,#509,.T.);
#5976=EDGE_CURVE('',#4886,#4412,#2760,.T.);
#5977=EDGE_CURVE('',#4565,#4887,#2761,.T.);
#5978=EDGE_CURVE('',#4887,#4419,#2762,.T.);
#5979=EDGE_CURVE('',#4411,#4888,#2763,.T.);
#5980=EDGE_CURVE('',#4888,#4889,#510,.T.);
#5981=EDGE_CURVE('',#4889,#4890,#2764,.T.);
#5982=EDGE_CURVE('',#4890,#4891,#2765,.T.);
#5983=EDGE_CURVE('',#4891,#4564,#2766,.T.);
#5984=EDGE_CURVE('',#4892,#4893,#2767,.T.);
#5985=EDGE_CURVE('',#4893,#4894,#3755,.T.);
#5986=EDGE_CURVE('',#4895,#4894,#2768,.T.);
#5987=EDGE_CURVE('',#4895,#4892,#3756,.T.);
#5988=EDGE_CURVE('',#4896,#4897,#2769,.T.);
#5989=EDGE_CURVE('',#4897,#4898,#3757,.T.);
#5990=EDGE_CURVE('',#4898,#4899,#2770,.T.);
#5991=EDGE_CURVE('',#4899,#4896,#3758,.T.);
#5992=EDGE_CURVE('',#4900,#4901,#2771,.T.);
#5993=EDGE_CURVE('',#4901,#4902,#511,.T.);
#5994=EDGE_CURVE('',#4902,#4900,#2772,.T.);
#5995=EDGE_CURVE('',#4903,#4904,#2773,.T.);
#5996=EDGE_CURVE('',#4904,#4905,#3759,.T.);
#5997=EDGE_CURVE('',#4905,#4906,#2774,.T.);
#5998=EDGE_CURVE('',#4906,#4903,#3760,.T.);
#5999=EDGE_CURVE('',#4907,#4908,#2775,.T.);
#6000=EDGE_CURVE('',#4908,#4909,#512,.T.);
#6001=EDGE_CURVE('',#4909,#4907,#2776,.T.);
#6002=EDGE_CURVE('',#4330,#4910,#3761,.T.);
#6003=EDGE_CURVE('',#4910,#4911,#2777,.T.);
#6004=EDGE_CURVE('',#4911,#4323,#3762,.T.);
#6005=EDGE_CURVE('',#4912,#4913,#2778,.T.);
#6006=EDGE_CURVE('',#4913,#4331,#2779,.T.);
#6007=EDGE_CURVE('',#4322,#4912,#2780,.T.);
#6008=EDGE_CURVE('',#4914,#4915,#2781,.T.);
#6009=EDGE_CURVE('',#4915,#4916,#2782,.T.);
#6010=EDGE_CURVE('',#4916,#4917,#2783,.T.);
#6011=EDGE_CURVE('',#4917,#4914,#2784,.T.);
#6012=EDGE_CURVE('',#4326,#4918,#3763,.T.);
#6013=EDGE_CURVE('',#4918,#4320,#2785,.T.);
#6014=EDGE_CURVE('',#4321,#4919,#3764,.T.);
#6015=EDGE_CURVE('',#4919,#4920,#3765,.T.);
#6016=EDGE_CURVE('',#4920,#4921,#2786,.T.);
#6017=EDGE_CURVE('',#4921,#4327,#3766,.T.);
#6018=EDGE_CURVE('',#4914,#4911,#3767,.T.);
#6019=EDGE_CURVE('',#4910,#4915,#3768,.T.);
#6020=EDGE_CURVE('',#4912,#4324,#3769,.T.);
#6021=EDGE_CURVE('',#4333,#4913,#3770,.T.);
#6022=EDGE_CURVE('',#4325,#4917,#3771,.T.);
#6023=EDGE_CURVE('',#4916,#4332,#3772,.T.);
#6024=EDGE_CURVE('',#4922,#4923,#3773,.T.);
#6025=EDGE_CURVE('',#4923,#4924,#513,.T.);
#6026=EDGE_CURVE('',#4924,#4925,#277,.T.);
#6027=EDGE_CURVE('',#4925,#4926,#3774,.T.);
#6028=EDGE_CURVE('',#4926,#4927,#514,.T.);
#6029=EDGE_CURVE('',#4927,#4928,#3775,.T.);
#6030=EDGE_CURVE('',#4928,#4922,#3776,.T.);
#6031=EDGE_CURVE('',#4447,#4929,#2787,.T.);
#6032=EDGE_CURVE('',#4929,#4930,#2788,.T.);
#6033=EDGE_CURVE('',#4930,#4931,#2789,.T.);
#6034=EDGE_CURVE('',#4932,#4931,#515,.T.);
#6035=EDGE_CURVE('',#4932,#4933,#2790,.T.);
#6036=EDGE_CURVE('',#4933,#4934,#3777,.T.);
#6037=EDGE_CURVE('',#4934,#4447,#2791,.T.);
#6038=EDGE_CURVE('',#4443,#4935,#2792,.T.);
#6039=EDGE_CURVE('',#4935,#4936,#2793,.T.);
#6040=EDGE_CURVE('',#4936,#4937,#2794,.T.);
#6041=EDGE_CURVE('',#4937,#4938,#3778,.T.);
#6042=EDGE_CURVE('',#4938,#4939,#2795,.T.);
#6043=EDGE_CURVE('',#4445,#4939,#516,.T.);
#6044=EDGE_CURVE('',#4940,#4941,#3779,.T.);
#6045=EDGE_CURVE('',#4941,#4942,#517,.T.);
#6046=EDGE_CURVE('',#4943,#4942,#518,.T.);
#6047=EDGE_CURVE('',#4943,#4944,#3780,.T.);
#6048=EDGE_CURVE('',#4944,#4945,#3781,.T.);
#6049=EDGE_CURVE('',#4945,#4946,#3782,.T.);
#6050=EDGE_CURVE('',#4946,#4940,#519,.T.);
#6051=EDGE_CURVE('',#4947,#4948,#2796,.T.);
#6052=EDGE_CURVE('',#4948,#4949,#3783,.T.);
#6053=EDGE_CURVE('',#4949,#4950,#2797,.T.);
#6054=EDGE_CURVE('',#4950,#4947,#3784,.T.);
#6055=EDGE_CURVE('',#4951,#4952,#2798,.T.);
#6056=EDGE_CURVE('',#4952,#4953,#3785,.T.);
#6057=EDGE_CURVE('',#4953,#4954,#2799,.T.);
#6058=EDGE_CURVE('',#4954,#4955,#3786,.T.);
#6059=EDGE_CURVE('',#4955,#4956,#520,.T.);
#6060=EDGE_CURVE('',#4956,#4951,#3787,.T.);
#6061=EDGE_CURVE('',#4957,#4958,#2800,.T.);
#6062=EDGE_CURVE('',#4958,#4959,#3788,.T.);
#6063=EDGE_CURVE('',#4959,#4960,#2801,.T.);
#6064=EDGE_CURVE('',#4960,#4961,#3789,.T.);
#6065=EDGE_CURVE('',#4961,#4413,#2802,.T.);
#6066=EDGE_CURVE('',#4414,#4962,#2803,.T.);
#6067=EDGE_CURVE('',#4962,#4957,#3790,.T.);
#6068=EDGE_CURVE('',#4963,#4964,#2804,.T.);
#6069=EDGE_CURVE('',#4964,#4965,#3791,.T.);
#6070=EDGE_CURVE('',#4965,#4966,#2805,.T.);
#6071=EDGE_CURVE('',#4966,#4967,#3792,.T.);
#6072=EDGE_CURVE('',#4967,#4968,#2806,.T.);
#6073=EDGE_CURVE('',#4968,#4969,#3793,.T.);
#6074=EDGE_CURVE('',#4969,#4970,#2807,.T.);
#6075=EDGE_CURVE('',#4970,#4963,#3794,.T.);
#6076=EDGE_CURVE('',#4971,#4972,#2808,.T.);
#6077=EDGE_CURVE('',#4972,#4973,#2809,.T.);
#6078=EDGE_CURVE('',#4973,#4974,#2810,.T.);
#6079=EDGE_CURVE('',#4975,#4974,#2811,.T.);
#6080=EDGE_CURVE('',#4975,#4976,#2812,.T.);
#6081=EDGE_CURVE('',#4977,#4976,#521,.T.);
#6082=EDGE_CURVE('',#4977,#4978,#522,.T.);
#6083=EDGE_CURVE('',#4971,#4978,#523,.T.);
#6084=EDGE_CURVE('',#4784,#4975,#3795,.T.);
#6085=EDGE_CURVE('',#4974,#4785,#3796,.T.);
#6086=EDGE_CURVE('',#4979,#4980,#2813,.T.);
#6087=EDGE_CURVE('',#4980,#4981,#2814,.T.);
#6088=EDGE_CURVE('',#4981,#4982,#2815,.T.);
#6089=EDGE_CURVE('',#4983,#4982,#524,.T.);
#6090=EDGE_CURVE('',#4983,#4984,#525,.T.);
#6091=EDGE_CURVE('',#4985,#4984,#526,.T.);
#6092=EDGE_CURVE('',#4985,#4986,#2816,.T.);
#6093=EDGE_CURVE('',#4979,#4986,#2817,.T.);
#6094=EDGE_CURVE('',#4986,#4799,#3797,.T.);
#6095=EDGE_CURVE('',#4798,#4979,#3798,.T.);
#6096=EDGE_CURVE('',#4987,#4988,#527,.T.);
#6097=EDGE_CURVE('',#4988,#4989,#3799,.T.);
#6098=EDGE_CURVE('',#4989,#4990,#528,.T.);
#6099=EDGE_CURVE('',#4990,#4987,#3800,.T.);
#6100=EDGE_CURVE('',#4991,#4992,#278,.T.);
#6101=EDGE_CURVE('',#4991,#4993,#529,.T.);
#6102=EDGE_CURVE('',#4993,#4994,#2818,.T.);
#6103=EDGE_CURVE('',#4994,#4995,#530,.T.);
#6104=EDGE_CURVE('',#4992,#4995,#279,.T.);
#6105=EDGE_CURVE('',#4996,#4997,#531,.T.);
#6106=EDGE_CURVE('',#4997,#4416,#2819,.T.);
#6107=EDGE_CURVE('',#4492,#4998,#2820,.T.);
#6108=EDGE_CURVE('',#4998,#4999,#2821,.T.);
#6109=EDGE_CURVE('',#4999,#4996,#2822,.T.);
#6110=EDGE_CURVE('',#4415,#5000,#2823,.T.);
#6111=EDGE_CURVE('',#5000,#4422,#532,.T.);
#6112=EDGE_CURVE('',#4424,#5001,#2824,.T.);
#6113=EDGE_CURVE('',#5001,#4491,#2825,.T.);
#6114=EDGE_CURVE('',#5002,#4448,#2826,.T.);
#6115=EDGE_CURVE('',#4448,#4735,#3801,.T.);
#6116=EDGE_CURVE('',#4734,#5002,#3802,.T.);
#6117=EDGE_CURVE('',#5003,#5004,#2827,.T.);
#6118=EDGE_CURVE('',#5004,#5005,#3803,.T.);
#6119=EDGE_CURVE('',#5005,#5006,#2828,.T.);
#6120=EDGE_CURVE('',#5006,#5003,#3804,.T.);
#6121=EDGE_CURVE('',#5007,#5008,#2829,.T.);
#6122=EDGE_CURVE('',#5008,#5009,#533,.T.);
#6123=EDGE_CURVE('',#5009,#5007,#2830,.T.);
#6124=EDGE_CURVE('',#5010,#5011,#2831,.T.);
#6125=EDGE_CURVE('',#5011,#5012,#3805,.T.);
#6126=EDGE_CURVE('',#5012,#5013,#2832,.T.);
#6127=EDGE_CURVE('',#5013,#5010,#3806,.T.);
#6128=EDGE_CURVE('',#5014,#5015,#2833,.T.);
#6129=EDGE_CURVE('',#5015,#5016,#534,.T.);
#6130=EDGE_CURVE('',#5016,#5014,#2834,.T.);
#6131=EDGE_CURVE('',#4483,#4359,#3807,.T.);
#6132=EDGE_CURVE('',#4359,#4350,#2835,.T.);
#6133=EDGE_CURVE('',#4350,#4480,#3808,.T.);
#6134=EDGE_CURVE('',#5017,#5018,#2836,.T.);
#6135=EDGE_CURVE('',#5018,#4482,#2837,.T.);
#6136=EDGE_CURVE('',#4481,#5017,#2838,.T.);
#6137=EDGE_CURVE('',#4351,#4358,#2839,.T.);
#6138=EDGE_CURVE('',#4358,#5019,#2840,.T.);
#6139=EDGE_CURVE('',#5019,#5020,#2841,.T.);
#6140=EDGE_CURVE('',#5020,#4351,#2842,.T.);
#6141=EDGE_CURVE('',#4354,#5021,#3809,.T.);
#6142=EDGE_CURVE('',#5021,#5022,#2843,.T.);
#6143=EDGE_CURVE('',#5022,#5023,#3810,.T.);
#6144=EDGE_CURVE('',#5023,#4348,#3811,.T.);
#6145=EDGE_CURVE('',#4349,#5024,#2844,.T.);
#6146=EDGE_CURVE('',#5024,#4355,#3812,.T.);
#6147=EDGE_CURVE('',#5017,#4352,#3813,.T.);
#6148=EDGE_CURVE('',#4361,#5018,#3814,.T.);
#6149=EDGE_CURVE('',#4353,#5020,#3815,.T.);
#6150=EDGE_CURVE('',#5019,#4360,#3816,.T.);
#6151=EDGE_CURVE('',#5025,#5026,#3817,.T.);
#6152=EDGE_CURVE('',#5026,#5027,#535,.T.);
#6153=EDGE_CURVE('',#5027,#5028,#280,.T.);
#6154=EDGE_CURVE('',#5028,#5029,#3818,.T.);
#6155=EDGE_CURVE('',#5029,#5030,#536,.T.);
#6156=EDGE_CURVE('',#5030,#5031,#3819,.T.);
#6157=EDGE_CURVE('',#5031,#5025,#3820,.T.);
#6158=EDGE_CURVE('',#5032,#5033,#2845,.T.);
#6159=EDGE_CURVE('',#5033,#5034,#2846,.T.);
#6160=EDGE_CURVE('',#5034,#5035,#2847,.T.);
#6161=EDGE_CURVE('',#5035,#5036,#2848,.T.);
#6162=EDGE_CURVE('',#5037,#5036,#537,.T.);
#6163=EDGE_CURVE('',#5037,#5038,#2849,.T.);
#6164=EDGE_CURVE('',#5038,#5032,#3821,.T.);
#6165=EDGE_CURVE('',#5039,#5040,#2850,.T.);
#6166=EDGE_CURVE('',#5040,#5041,#2851,.T.);
#6167=EDGE_CURVE('',#5041,#5042,#2852,.T.);
#6168=EDGE_CURVE('',#5042,#5043,#2853,.T.);
#6169=EDGE_CURVE('',#5043,#5044,#3822,.T.);
#6170=EDGE_CURVE('',#5044,#5045,#2854,.T.);
#6171=EDGE_CURVE('',#5039,#5045,#538,.T.);
#6172=EDGE_CURVE('',#5046,#5047,#3823,.T.);
#6173=EDGE_CURVE('',#5047,#5048,#539,.T.);
#6174=EDGE_CURVE('',#5049,#5048,#540,.T.);
#6175=EDGE_CURVE('',#5049,#5050,#3824,.T.);
#6176=EDGE_CURVE('',#5050,#5051,#3825,.T.);
#6177=EDGE_CURVE('',#5051,#5052,#3826,.T.);
#6178=EDGE_CURVE('',#5052,#5046,#541,.T.);
#6179=EDGE_CURVE('',#4394,#4400,#2855,.T.);
#6180=EDGE_CURVE('',#4399,#4393,#2856,.T.);
#6181=EDGE_CURVE('',#5053,#4397,#2857,.T.);
#6182=EDGE_CURVE('',#4398,#5054,#2858,.T.);
#6183=EDGE_CURVE('',#5054,#5055,#3827,.T.);
#6184=EDGE_CURVE('',#5055,#5056,#542,.T.);
#6185=EDGE_CURVE('',#5056,#5053,#3828,.T.);
#6186=EDGE_CURVE('',#5057,#5058,#543,.T.);
#6187=EDGE_CURVE('',#5057,#5059,#2859,.T.);
#6188=EDGE_CURVE('',#5059,#5060,#2860,.T.);
#6189=EDGE_CURVE('',#5060,#5061,#2861,.T.);
#6190=EDGE_CURVE('',#5062,#5061,#2862,.T.);
#6191=EDGE_CURVE('',#5062,#5063,#2863,.T.);
#6192=EDGE_CURVE('',#5064,#5063,#544,.T.);
#6193=EDGE_CURVE('',#5064,#5058,#545,.T.);
#6194=EDGE_CURVE('',#4622,#5062,#3829,.T.);
#6195=EDGE_CURVE('',#5061,#4623,#3830,.T.);
#6196=EDGE_CURVE('',#5065,#5066,#2864,.T.);
#6197=EDGE_CURVE('',#5066,#5067,#2865,.T.);
#6198=EDGE_CURVE('',#5068,#5067,#546,.T.);
#6199=EDGE_CURVE('',#5068,#5069,#547,.T.);
#6200=EDGE_CURVE('',#5070,#5069,#548,.T.);
#6201=EDGE_CURVE('',#5070,#5071,#2866,.T.);
#6202=EDGE_CURVE('',#5072,#5071,#2867,.T.);
#6203=EDGE_CURVE('',#5072,#5065,#2868,.T.);
#6204=EDGE_CURVE('',#5071,#4627,#3831,.T.);
#6205=EDGE_CURVE('',#4626,#5072,#3832,.T.);
#6206=EDGE_CURVE('',#5073,#5074,#549,.T.);
#6207=EDGE_CURVE('',#5074,#5075,#3833,.T.);
#6208=EDGE_CURVE('',#5075,#5076,#550,.T.);
#6209=EDGE_CURVE('',#5076,#5073,#3834,.T.);
#6210=EDGE_CURVE('',#5077,#5078,#281,.T.);
#6211=EDGE_CURVE('',#5077,#5079,#551,.T.);
#6212=EDGE_CURVE('',#5079,#5080,#2869,.T.);
#6213=EDGE_CURVE('',#5080,#5081,#552,.T.);
#6214=EDGE_CURVE('',#5078,#5081,#282,.T.);
#6215=EDGE_CURVE('',#5082,#5083,#553,.T.);
#6216=EDGE_CURVE('',#5083,#4478,#2870,.T.);
#6217=EDGE_CURVE('',#4407,#5084,#2871,.T.);
#6218=EDGE_CURVE('',#5084,#5085,#2872,.T.);
#6219=EDGE_CURVE('',#5085,#5082,#2873,.T.);
#6220=EDGE_CURVE('',#4479,#5086,#2874,.T.);
#6221=EDGE_CURVE('',#5086,#5087,#554,.T.);
#6222=EDGE_CURVE('',#5087,#5088,#2875,.T.);
#6223=EDGE_CURVE('',#5088,#5089,#2876,.T.);
#6224=EDGE_CURVE('',#5089,#4408,#2877,.T.);
#6225=EDGE_CURVE('',#5090,#5091,#2878,.T.);
#6226=EDGE_CURVE('',#5091,#4936,#3835,.T.);
#6227=EDGE_CURVE('',#4935,#5090,#3836,.T.);
#6228=EDGE_CURVE('',#5092,#5093,#2879,.T.);
#6229=EDGE_CURVE('',#5093,#5094,#3837,.T.);
#6230=EDGE_CURVE('',#5094,#5095,#2880,.T.);
#6231=EDGE_CURVE('',#5095,#5092,#3838,.T.);
#6232=EDGE_CURVE('',#5096,#5097,#2881,.T.);
#6233=EDGE_CURVE('',#5097,#5098,#555,.T.);
#6234=EDGE_CURVE('',#5098,#5096,#2882,.T.);
#6235=EDGE_CURVE('',#5099,#5100,#2883,.T.);
#6236=EDGE_CURVE('',#5100,#5101,#3839,.T.);
#6237=EDGE_CURVE('',#5101,#5102,#2884,.T.);
#6238=EDGE_CURVE('',#5102,#5099,#3840,.T.);
#6239=EDGE_CURVE('',#4440,#5103,#556,.T.);
#6240=EDGE_CURVE('',#5103,#4441,#2885,.T.);
#6241=EDGE_CURVE('',#4470,#5104,#3841,.T.);
#6242=EDGE_CURVE('',#5104,#5105,#2886,.T.);
#6243=EDGE_CURVE('',#5105,#4467,#3842,.T.);
#6244=EDGE_CURVE('',#4468,#5106,#2887,.T.);
#6245=EDGE_CURVE('',#5106,#5107,#2888,.T.);
#6246=EDGE_CURVE('',#5107,#4469,#2889,.T.);
#6247=EDGE_CURVE('',#5108,#5109,#2890,.T.);
#6248=EDGE_CURVE('',#5109,#5110,#2891,.T.);
#6249=EDGE_CURVE('',#5110,#5111,#2892,.T.);
#6250=EDGE_CURVE('',#5111,#5108,#2893,.T.);
#6251=EDGE_CURVE('',#5112,#5113,#2894,.T.);
#6252=EDGE_CURVE('',#5112,#5114,#2895,.T.);
#6253=EDGE_CURVE('',#5114,#5115,#3843,.T.);
#6254=EDGE_CURVE('',#5115,#5116,#3844,.T.);
#6255=EDGE_CURVE('',#5116,#5117,#3845,.T.);
#6256=EDGE_CURVE('',#5117,#5118,#2896,.T.);
#6257=EDGE_CURVE('',#5118,#5119,#3846,.T.);
#6258=EDGE_CURVE('',#5119,#4373,#3847,.T.);
#6259=EDGE_CURVE('',#4664,#5120,#2897,.T.);
#6260=EDGE_CURVE('',#5113,#5120,#2898,.T.);
#6261=EDGE_CURVE('',#5108,#5105,#3848,.T.);
#6262=EDGE_CURVE('',#5104,#5109,#3849,.T.);
#6263=EDGE_CURVE('',#4471,#5111,#3850,.T.);
#6264=EDGE_CURVE('',#5110,#4472,#3851,.T.);
#6265=EDGE_CURVE('',#5121,#5122,#3852,.T.);
#6266=EDGE_CURVE('',#5122,#5123,#557,.T.);
#6267=EDGE_CURVE('',#5123,#5124,#283,.T.);
#6268=EDGE_CURVE('',#5124,#5125,#3853,.T.);
#6269=EDGE_CURVE('',#5125,#5126,#558,.T.);
#6270=EDGE_CURVE('',#5126,#5127,#3854,.T.);
#6271=EDGE_CURVE('',#5127,#5121,#3855,.T.);
#6272=EDGE_CURVE('',#4426,#5128,#2899,.T.);
#6273=EDGE_CURVE('',#5128,#5129,#2900,.T.);
#6274=EDGE_CURVE('',#5130,#5129,#559,.T.);
#6275=EDGE_CURVE('',#5130,#5131,#2901,.T.);
#6276=EDGE_CURVE('',#5131,#5132,#3856,.T.);
#6277=EDGE_CURVE('',#5132,#4427,#2902,.T.);
#6278=EDGE_CURVE('',#5133,#5134,#2903,.T.);
#6279=EDGE_CURVE('',#5134,#4895,#2904,.T.);
#6280=EDGE_CURVE('',#4894,#5135,#2905,.T.);
#6281=EDGE_CURVE('',#5135,#5136,#3857,.T.);
#6282=EDGE_CURVE('',#5136,#5137,#2906,.T.);
#6283=EDGE_CURVE('',#5133,#5137,#560,.T.);
#6284=EDGE_CURVE('',#5138,#5139,#3858,.T.);
#6285=EDGE_CURVE('',#5139,#5140,#561,.T.);
#6286=EDGE_CURVE('',#5141,#5140,#562,.T.);
#6287=EDGE_CURVE('',#5141,#5142,#3859,.T.);
#6288=EDGE_CURVE('',#5142,#5143,#3860,.T.);
#6289=EDGE_CURVE('',#5143,#5144,#3861,.T.);
#6290=EDGE_CURVE('',#5144,#5138,#563,.T.);
#6291=EDGE_CURVE('',#5145,#5146,#2907,.T.);
#6292=EDGE_CURVE('',#5146,#5147,#3862,.T.);
#6293=EDGE_CURVE('',#5147,#5148,#2908,.T.);
#6294=EDGE_CURVE('',#5148,#5149,#3863,.T.);
#6295=EDGE_CURVE('',#5149,#5150,#2909,.T.);
#6296=EDGE_CURVE('',#5150,#5151,#3864,.T.);
#6297=EDGE_CURVE('',#5151,#5152,#2910,.T.);
#6298=EDGE_CURVE('',#5152,#5145,#3865,.T.);
#6299=EDGE_CURVE('',#5153,#5154,#2911,.T.);
#6300=EDGE_CURVE('',#5154,#5155,#3866,.T.);
#6301=EDGE_CURVE('',#5155,#5156,#2912,.T.);
#6302=EDGE_CURVE('',#5156,#5157,#3867,.T.);
#6303=EDGE_CURVE('',#5157,#4401,#2913,.T.);
#6304=EDGE_CURVE('',#4402,#5158,#2914,.T.);
#6305=EDGE_CURVE('',#5158,#5153,#3868,.T.);
#6306=EDGE_CURVE('',#5059,#4790,#3869,.T.);
#6307=EDGE_CURVE('',#4791,#5060,#3870,.T.);
#6308=EDGE_CURVE('',#4808,#5066,#3871,.T.);
#6309=EDGE_CURVE('',#5065,#4809,#3872,.T.);
#6310=EDGE_CURVE('',#5159,#5160,#564,.T.);
#6311=EDGE_CURVE('',#5160,#5161,#3873,.T.);
#6312=EDGE_CURVE('',#5161,#5162,#565,.T.);
#6313=EDGE_CURVE('',#5162,#5159,#3874,.T.);
#6314=EDGE_CURVE('',#5163,#5164,#566,.T.);
#6315=EDGE_CURVE('',#5164,#4465,#2915,.T.);
#6316=EDGE_CURVE('',#4403,#5165,#2916,.T.);
#6317=EDGE_CURVE('',#5165,#5166,#2917,.T.);
#6318=EDGE_CURVE('',#5166,#5163,#2918,.T.);
#6319=EDGE_CURVE('',#4466,#5167,#2919,.T.);
#6320=EDGE_CURVE('',#5167,#5168,#567,.T.);
#6321=EDGE_CURVE('',#5168,#5169,#2920,.T.);
#6322=EDGE_CURVE('',#5169,#5170,#2921,.T.);
#6323=EDGE_CURVE('',#5170,#4404,#2922,.T.);
#6324=EDGE_CURVE('',#4428,#5042,#3875,.T.);
#6325=EDGE_CURVE('',#5041,#4425,#3876,.T.);
#6326=EDGE_CURVE('',#5171,#5172,#2923,.T.);
#6327=EDGE_CURVE('',#5172,#5173,#3877,.T.);
#6328=EDGE_CURVE('',#5173,#5174,#2924,.T.);
#6329=EDGE_CURVE('',#5174,#5171,#3878,.T.);
#6330=EDGE_CURVE('',#4434,#5175,#2925,.T.);
#6331=EDGE_CURVE('',#5175,#4431,#568,.T.);
#6332=EDGE_CURVE('',#5176,#5177,#2926,.T.);
#6333=EDGE_CURVE('',#5177,#5178,#3879,.T.);
#6334=EDGE_CURVE('',#5178,#5179,#2927,.T.);
#6335=EDGE_CURVE('',#5179,#5176,#3880,.T.);
#6336=EDGE_CURVE('',#5180,#5181,#2928,.T.);
#6337=EDGE_CURVE('',#5181,#5182,#569,.T.);
#6338=EDGE_CURVE('',#5182,#5180,#2929,.T.);
#6339=EDGE_CURVE('',#4462,#5183,#3881,.T.);
#6340=EDGE_CURVE('',#5183,#5184,#2930,.T.);
#6341=EDGE_CURVE('',#5184,#4459,#3882,.T.);
#6342=EDGE_CURVE('',#5185,#5186,#2931,.T.);
#6343=EDGE_CURVE('',#5186,#4461,#2932,.T.);
#6344=EDGE_CURVE('',#4460,#5185,#2933,.T.);
#6345=EDGE_CURVE('',#5187,#5188,#2934,.T.);
#6346=EDGE_CURVE('',#5188,#4458,#2935,.T.);
#6347=EDGE_CURVE('',#4458,#4453,#2936,.T.);
#6348=EDGE_CURVE('',#4453,#5187,#2937,.T.);
#6349=EDGE_CURVE('',#4452,#5189,#3883,.T.);
#6350=EDGE_CURVE('',#5189,#5190,#3884,.T.);
#6351=EDGE_CURVE('',#5190,#5191,#2938,.T.);
#6352=EDGE_CURVE('',#5191,#5192,#3885,.T.);
#6353=EDGE_CURVE('',#5192,#5193,#3886,.T.);
#6354=EDGE_CURVE('',#5193,#5194,#3887,.T.);
#6355=EDGE_CURVE('',#5194,#4451,#2939,.T.);
#6356=EDGE_CURVE('',#5187,#5184,#3888,.T.);
#6357=EDGE_CURVE('',#5183,#5188,#3889,.T.);
#6358=EDGE_CURVE('',#5185,#4463,#3890,.T.);
#6359=EDGE_CURVE('',#4464,#5186,#3891,.T.);
#6360=EDGE_CURVE('',#4464,#4594,#3892,.T.);
#6361=EDGE_CURVE('',#5186,#4593,#3893,.T.);
#6362=EDGE_CURVE('',#4461,#4592,#3894,.T.);
#6363=EDGE_CURVE('',#4595,#5188,#3895,.T.);
#6364=EDGE_CURVE('',#4462,#4591,#3896,.T.);
#6365=EDGE_CURVE('',#4590,#5183,#3897,.T.);
#6366=EDGE_CURVE('',#5189,#4463,#3898,.T.);
#6367=EDGE_CURVE('',#5190,#5185,#3899,.T.);
#6368=EDGE_CURVE('',#5191,#4460,#3900,.T.);
#6369=EDGE_CURVE('',#5187,#5194,#3901,.T.);
#6370=EDGE_CURVE('',#5192,#4459,#3902,.T.);
#6371=EDGE_CURVE('',#5184,#5193,#3903,.T.);
#6372=EDGE_CURVE('',#4500,#5195,#570,.T.);
#6373=EDGE_CURVE('',#4551,#5196,#571,.T.);
#6374=EDGE_CURVE('',#5196,#5195,#572,.T.);
#6375=EDGE_CURVE('',#5196,#5046,#573,.T.);
#6376=EDGE_CURVE('',#5046,#5197,#574,.T.);
#6377=EDGE_CURVE('',#5197,#5195,#575,.T.);
#6378=EDGE_CURVE('',#5197,#4695,#576,.T.);
#6379=EDGE_CURVE('',#4693,#5195,#577,.T.);
#6380=EDGE_CURVE('',#4694,#5198,#578,.T.);
#6381=EDGE_CURVE('',#5198,#5195,#579,.T.);
#6382=EDGE_CURVE('',#5198,#5125,#580,.T.);
#6383=EDGE_CURVE('',#5199,#5125,#581,.T.);
#6384=EDGE_CURVE('',#5199,#5195,#582,.T.);
#6385=EDGE_CURVE('',#5200,#5201,#583,.T.);
#6386=EDGE_CURVE('',#5200,#4881,#584,.T.);
#6387=EDGE_CURVE('',#4882,#5201,#585,.T.);
#6388=EDGE_CURVE('',#4885,#5202,#586,.T.);
#6389=EDGE_CURVE('',#5202,#5201,#587,.T.);
#6390=EDGE_CURVE('',#5202,#4702,#588,.T.);
#6391=EDGE_CURVE('',#4702,#5203,#589,.T.);
#6392=EDGE_CURVE('',#5203,#5201,#590,.T.);
#6393=EDGE_CURVE('',#5203,#4514,#591,.T.);
#6394=EDGE_CURVE('',#4513,#5201,#592,.T.);
#6395=EDGE_CURVE('',#5204,#4512,#3904,.T.);
#6396=EDGE_CURVE('',#5204,#5201,#593,.T.);
#6397=EDGE_CURVE('',#4539,#5205,#594,.T.);
#6398=EDGE_CURVE('',#4538,#5206,#595,.T.);
#6399=EDGE_CURVE('',#5206,#5205,#596,.T.);
#6400=EDGE_CURVE('',#5206,#4940,#597,.T.);
#6401=EDGE_CURVE('',#4940,#5207,#598,.T.);
#6402=EDGE_CURVE('',#5207,#5205,#599,.T.);
#6403=EDGE_CURVE('',#5207,#4685,#600,.T.);
#6404=EDGE_CURVE('',#4683,#5205,#601,.T.);
#6405=EDGE_CURVE('',#4684,#5208,#602,.T.);
#6406=EDGE_CURVE('',#5208,#5205,#603,.T.);
#6407=EDGE_CURVE('',#5208,#5029,#604,.T.);
#6408=EDGE_CURVE('',#5209,#5029,#605,.T.);
#6409=EDGE_CURVE('',#5209,#5205,#606,.T.);
#6410=EDGE_CURVE('',#5210,#5211,#607,.T.);
#6411=EDGE_CURVE('',#5210,#4680,#608,.T.);
#6412=EDGE_CURVE('',#4678,#5211,#609,.T.);
#6413=EDGE_CURVE('',#4679,#5212,#610,.T.);
#6414=EDGE_CURVE('',#5212,#5211,#611,.T.);
#6415=EDGE_CURVE('',#5212,#4926,#612,.T.);
#6416=EDGE_CURVE('',#4926,#5213,#613,.T.);
#6417=EDGE_CURVE('',#5213,#5211,#614,.T.);
#6418=EDGE_CURVE('',#5213,#4527,#615,.T.);
#6419=EDGE_CURVE('',#4526,#5211,#616,.T.);
#6420=EDGE_CURVE('',#5214,#4525,#3905,.T.);
#6421=EDGE_CURVE('',#5214,#5211,#617,.T.);
#6422=EDGE_CURVE('',#4925,#5015,#618,.T.);
#6423=EDGE_CURVE('',#5016,#4924,#3906,.T.);
#6424=EDGE_CURVE('',#5011,#4923,#3907,.T.);
#6425=EDGE_CURVE('',#5016,#5011,#619,.T.);
#6426=EDGE_CURVE('',#4925,#4528,#3908,.T.);
#6427=EDGE_CURVE('',#4529,#5015,#3909,.T.);
#6428=EDGE_CURVE('',#5012,#4922,#3910,.T.);
#6429=EDGE_CURVE('',#5014,#5010,#3911,.T.);
#6430=EDGE_CURVE('',#4530,#5014,#3912,.T.);
#6431=EDGE_CURVE('',#4927,#4682,#620,.T.);
#6432=EDGE_CURVE('',#4681,#4745,#621,.T.);
#6433=EDGE_CURVE('',#4739,#5210,#622,.T.);
#6434=EDGE_CURVE('',#4860,#4681,#3913,.T.);
#6435=EDGE_CURVE('',#4682,#4859,#3914,.T.);
#6436=EDGE_CURVE('',#4927,#4858,#3915,.T.);
#6437=EDGE_CURVE('',#5012,#4933,#3916,.T.);
#6438=EDGE_CURVE('',#4933,#4922,#3917,.T.);
#6439=EDGE_CURVE('',#4943,#5005,#3918,.T.);
#6440=EDGE_CURVE('',#5008,#4942,#3919,.T.);
#6441=EDGE_CURVE('',#5005,#5008,#623,.T.);
#6442=EDGE_CURVE('',#4530,#5010,#3920,.T.);
#6443=EDGE_CURVE('',#4739,#5214,#624,.T.);
#6444=EDGE_CURVE('',#4852,#4745,#3921,.T.);
#6445=EDGE_CURVE('',#4928,#4857,#3922,.T.);
#6446=EDGE_CURVE('',#4934,#4928,#625,.T.);
#6447=EDGE_CURVE('',#5013,#4932,#3923,.T.);
#6448=EDGE_CURVE('',#4531,#5013,#626,.T.);
#6449=EDGE_CURVE('',#5009,#4941,#627,.T.);
#6450=EDGE_CURVE('',#5007,#4535,#3924,.T.);
#6451=EDGE_CURVE('',#4536,#5009,#3925,.T.);
#6452=EDGE_CURVE('',#5006,#5007,#3926,.T.);
#6453=EDGE_CURVE('',#4944,#5004,#3927,.T.);
#6454=EDGE_CURVE('',#4537,#4941,#3928,.T.);
#6455=EDGE_CURVE('',#4740,#4524,#3929,.T.);
#6456=EDGE_CURVE('',#4741,#4901,#3930,.T.);
#6457=EDGE_CURVE('',#4902,#4740,#628,.T.);
#6458=EDGE_CURVE('',#4853,#4744,#3931,.T.);
#6459=EDGE_CURVE('',#4855,#4735,#3932,.T.);
#6460=EDGE_CURVE('',#4736,#4854,#3933,.T.);
#6461=EDGE_CURVE('',#4934,#4856,#3934,.T.);
#6462=EDGE_CURVE('',#4531,#4931,#3935,.T.);
#6463=EDGE_CURVE('',#5006,#4535,#3936,.T.);
#6464=EDGE_CURVE('',#4944,#4938,#3937,.T.);
#6465=EDGE_CURVE('',#4938,#5004,#3938,.T.);
#6466=EDGE_CURVE('',#4825,#4946,#3939,.T.);
#6467=EDGE_CURVE('',#4686,#4824,#3940,.T.);
#6468=EDGE_CURVE('',#4946,#4686,#629,.T.);
#6469=EDGE_CURVE('',#4687,#4823,#3941,.T.);
#6470=EDGE_CURVE('',#5030,#4687,#630,.T.);
#6471=EDGE_CURVE('',#4902,#4523,#3942,.T.);
#6472=EDGE_CURVE('',#4898,#4901,#631,.T.);
#6473=EDGE_CURVE('',#4742,#4898,#3943,.T.);
#6474=EDGE_CURVE('',#4736,#4744,#632,.T.);
#6475=EDGE_CURVE('',#4532,#4930,#3944,.T.);
#6476=EDGE_CURVE('',#5003,#4446,#633,.T.);
#6477=EDGE_CURVE('',#4939,#5003,#3945,.T.);
#6478=EDGE_CURVE('',#4945,#4937,#634,.T.);
#6479=EDGE_CURVE('',#4826,#4945,#3946,.T.);
#6480=EDGE_CURVE('',#5030,#4822,#3947,.T.);
#6481=EDGE_CURVE('',#4540,#5209,#3948,.T.);
#6482=EDGE_CURVE('',#4900,#4522,#3949,.T.);
#6483=EDGE_CURVE('',#4899,#4900,#3950,.T.);
#6484=EDGE_CURVE('',#4743,#4897,#3951,.T.);
#6485=EDGE_CURVE('',#4737,#4743,#3952,.T.);
#6486=EDGE_CURVE('',#4710,#4930,#635,.T.);
#6487=EDGE_CURVE('',#4533,#4710,#3953,.T.);
#6488=EDGE_CURVE('',#4827,#4937,#3954,.T.);
#6489=EDGE_CURVE('',#5031,#4821,#3955,.T.);
#6490=EDGE_CURVE('',#5028,#4440,#636,.T.);
#6491=EDGE_CURVE('',#5103,#5027,#3956,.T.);
#6492=EDGE_CURVE('',#4701,#4908,#637,.T.);
#6493=EDGE_CURVE('',#4909,#4700,#3957,.T.);
#6494=EDGE_CURVE('',#4541,#5028,#3958,.T.);
#6495=EDGE_CURVE('',#4899,#4522,#3959,.T.);
#6496=EDGE_CURVE('',#4737,#4897,#3960,.T.);
#6497=EDGE_CURVE('',#4929,#5002,#3961,.T.);
#6498=EDGE_CURVE('',#4711,#4929,#3962,.T.);
#6499=EDGE_CURVE('',#4534,#4709,#3963,.T.);
#6500=EDGE_CURVE('',#4828,#4936,#3964,.T.);
#6501=EDGE_CURVE('',#5032,#4820,#3965,.T.);
#6502=EDGE_CURVE('',#5031,#5032,#638,.T.);
#6503=EDGE_CURVE('',#5100,#5026,#3966,.T.);
#6504=EDGE_CURVE('',#5103,#5100,#639,.T.);
#6505=EDGE_CURVE('',#4904,#4699,#3967,.T.);
#6506=EDGE_CURVE('',#4909,#4904,#640,.T.);
#6507=EDGE_CURVE('',#4701,#4515,#3968,.T.);
#6508=EDGE_CURVE('',#4516,#4908,#3969,.T.);
#6509=EDGE_CURVE('',#4905,#4698,#3970,.T.);
#6510=EDGE_CURVE('',#4907,#4903,#3971,.T.);
#6511=EDGE_CURVE('',#4517,#4907,#3972,.T.);
#6512=EDGE_CURVE('',#4896,#4521,#641,.T.);
#6513=EDGE_CURVE('',#4738,#4896,#3973,.T.);
#6514=EDGE_CURVE('',#4712,#5002,#3974,.T.);
#6515=EDGE_CURVE('',#4443,#4709,#642,.T.);
#6516=EDGE_CURVE('',#4829,#5091,#3975,.T.);
#6517=EDGE_CURVE('',#5033,#4819,#3976,.T.);
#6518=EDGE_CURVE('',#5025,#5038,#3977,.T.);
#6519=EDGE_CURVE('',#5101,#5025,#3978,.T.);
#6520=EDGE_CURVE('',#4441,#5099,#3979,.T.);
#6521=EDGE_CURVE('',#4703,#4884,#643,.T.);
#6522=EDGE_CURVE('',#4883,#5144,#644,.T.);
#6523=EDGE_CURVE('',#5138,#5200,#645,.T.);
#6524=EDGE_CURVE('',#4868,#4883,#3980,.T.);
#6525=EDGE_CURVE('',#4884,#4867,#3981,.T.);
#6526=EDGE_CURVE('',#4703,#4866,#3982,.T.);
#6527=EDGE_CURVE('',#4905,#4730,#3983,.T.);
#6528=EDGE_CURVE('',#4730,#4698,#3984,.T.);
#6529=EDGE_CURVE('',#4517,#4903,#3985,.T.);
#6530=EDGE_CURVE('',#4732,#4521,#3986,.T.);
#6531=EDGE_CURVE('',#4713,#4734,#3987,.T.);
#6532=EDGE_CURVE('',#4935,#4708,#3988,.T.);
#6533=EDGE_CURVE('',#4668,#5091,#3989,.T.);
#6534=EDGE_CURVE('',#5101,#5038,#3990,.T.);
#6535=EDGE_CURVE('',#4442,#5099,#3991,.T.);
#6536=EDGE_CURVE('',#5138,#5204,#646,.T.);
#6537=EDGE_CURVE('',#4869,#5144,#3992,.T.);
#6538=EDGE_CURVE('',#4704,#4865,#3993,.T.);
#6539=EDGE_CURVE('',#4731,#4704,#647,.T.);
#6540=EDGE_CURVE('',#4906,#4729,#3994,.T.);
#6541=EDGE_CURVE('',#4437,#4906,#648,.T.);
#6542=EDGE_CURVE('',#4733,#4520,#3995,.T.);
#6543=EDGE_CURVE('',#4714,#4733,#649,.T.);
#6544=EDGE_CURVE('',#5090,#4707,#3996,.T.);
#6545=EDGE_CURVE('',#4665,#5090,#3997,.T.);
#6546=EDGE_CURVE('',#5102,#5037,#3998,.T.);
#6547=EDGE_CURVE('',#4542,#5102,#650,.T.);
#6548=EDGE_CURVE('',#5139,#4511,#3999,.T.);
#6549=EDGE_CURVE('',#5140,#5175,#4000,.T.);
#6550=EDGE_CURVE('',#4431,#5139,#651,.T.);
#6551=EDGE_CURVE('',#4870,#5143,#4001,.T.);
#6552=EDGE_CURVE('',#4861,#4894,#4002,.T.);
#6553=EDGE_CURVE('',#5135,#4871,#4003,.T.);
#6554=EDGE_CURVE('',#4731,#4864,#4004,.T.);
#6555=EDGE_CURVE('',#4714,#4519,#4005,.T.);
#6556=EDGE_CURVE('',#4542,#5036,#4006,.T.);
#6557=EDGE_CURVE('',#5173,#5175,#652,.T.);
#6558=EDGE_CURVE('',#5141,#5173,#4007,.T.);
#6559=EDGE_CURVE('',#5135,#5143,#653,.T.);
#6560=EDGE_CURVE('',#4862,#4893,#4008,.T.);
#6561=EDGE_CURVE('',#4727,#4863,#4009,.T.);
#6562=EDGE_CURVE('',#4715,#4518,#4010,.T.);
#6563=EDGE_CURVE('',#4724,#5034,#4011,.T.);
#6564=EDGE_CURVE('',#5035,#4723,#654,.T.);
#6565=EDGE_CURVE('',#4543,#5035,#4012,.T.);
#6566=EDGE_CURVE('',#5174,#4434,#4013,.T.);
#6567=EDGE_CURVE('',#5142,#5172,#4014,.T.);
#6568=EDGE_CURVE('',#5136,#5142,#4015,.T.);
#6569=EDGE_CURVE('',#4727,#4893,#4016,.T.);
#6570=EDGE_CURVE('',#4715,#4436,#655,.T.);
#6571=EDGE_CURVE('',#4544,#4723,#4017,.T.);
#6572=EDGE_CURVE('',#5174,#4433,#4018,.T.);
#6573=EDGE_CURVE('',#5136,#5172,#4019,.T.);
#6574=EDGE_CURVE('',#4728,#4892,#4020,.T.);
#6575=EDGE_CURVE('',#4716,#4728,#4021,.T.);
#6576=EDGE_CURVE('',#4545,#4722,#4022,.T.);
#6577=EDGE_CURVE('',#5040,#4546,#4023,.T.);
#6578=EDGE_CURVE('',#4547,#5039,#4024,.T.);
#6579=EDGE_CURVE('',#5045,#5092,#4025,.T.);
#6580=EDGE_CURVE('',#5093,#5044,#4026,.T.);
#6581=EDGE_CURVE('',#4547,#5092,#656,.T.);
#6582=EDGE_CURVE('',#5171,#4510,#657,.T.);
#6583=EDGE_CURVE('',#5137,#5171,#4027,.T.);
#6584=EDGE_CURVE('',#4717,#4892,#4028,.T.);
#6585=EDGE_CURVE('',#5040,#4722,#658,.T.);
#6586=EDGE_CURVE('',#5050,#5044,#4029,.T.);
#6587=EDGE_CURVE('',#5093,#5050,#4030,.T.);
#6588=EDGE_CURVE('',#5094,#5049,#4031,.T.);
#6589=EDGE_CURVE('',#5095,#5096,#4032,.T.);
#6590=EDGE_CURVE('',#5097,#5094,#659,.T.);
#6591=EDGE_CURVE('',#4548,#5095,#4033,.T.);
#6592=EDGE_CURVE('',#5133,#4510,#4034,.T.);
#6593=EDGE_CURVE('',#4718,#4895,#4035,.T.);
#6594=EDGE_CURVE('',#5041,#4721,#4036,.T.);
#6595=EDGE_CURVE('',#5051,#5043,#660,.T.);
#6596=EDGE_CURVE('',#5097,#5048,#4037,.T.);
#6597=EDGE_CURVE('',#4548,#5096,#4038,.T.);
#6598=EDGE_CURVE('',#5134,#4509,#4039,.T.);
#6599=EDGE_CURVE('',#4719,#5134,#661,.T.);
#6600=EDGE_CURVE('',#4843,#5043,#4040,.T.);
#6601=EDGE_CURVE('',#5051,#4842,#4041,.T.);
#6602=EDGE_CURVE('',#5052,#4841,#4042,.T.);
#6603=EDGE_CURVE('',#5098,#5047,#662,.T.);
#6604=EDGE_CURVE('',#4549,#5098,#4043,.T.);
#6605=EDGE_CURVE('',#4719,#4508,#4044,.T.);
#6606=EDGE_CURVE('',#4844,#5042,#4045,.T.);
#6607=EDGE_CURVE('',#4696,#4851,#4046,.T.);
#6608=EDGE_CURVE('',#5052,#4696,#663,.T.);
#6609=EDGE_CURVE('',#4550,#5047,#4047,.T.);
#6610=EDGE_CURVE('',#4720,#4507,#4048,.T.);
#6611=EDGE_CURVE('',#5128,#4720,#664,.T.);
#6612=EDGE_CURVE('',#4845,#4428,#4049,.T.);
#6613=EDGE_CURVE('',#4697,#4850,#4050,.T.);
#6614=EDGE_CURVE('',#5126,#4697,#665,.T.);
#6615=EDGE_CURVE('',#5128,#4506,#4051,.T.);
#6616=EDGE_CURVE('',#4846,#4427,#4052,.T.);
#6617=EDGE_CURVE('',#5126,#4849,#4053,.T.);
#6618=EDGE_CURVE('',#4501,#5199,#4054,.T.);
#6619=EDGE_CURVE('',#5129,#4505,#4055,.T.);
#6620=EDGE_CURVE('',#4847,#5132,#4056,.T.);
#6621=EDGE_CURVE('',#5127,#4848,#4057,.T.);
#6622=EDGE_CURVE('',#4502,#5124,#4058,.T.);
#6623=EDGE_CURVE('',#4504,#5180,#4059,.T.);
#6624=EDGE_CURVE('',#5181,#4503,#4060,.T.);
#6625=EDGE_CURVE('',#4505,#5179,#666,.T.);
#6626=EDGE_CURVE('',#5176,#4504,#4061,.T.);
#6627=EDGE_CURVE('',#5130,#5179,#4062,.T.);
#6628=EDGE_CURVE('',#5127,#5132,#667,.T.);
#6629=EDGE_CURVE('',#5181,#5124,#668,.T.);
#6630=EDGE_CURVE('',#5176,#5180,#4063,.T.);
#6631=EDGE_CURVE('',#5131,#5178,#4064,.T.);
#6632=EDGE_CURVE('',#5121,#5131,#4065,.T.);
#6633=EDGE_CURVE('',#5182,#5123,#4066,.T.);
#6634=EDGE_CURVE('',#5177,#5182,#669,.T.);
#6635=EDGE_CURVE('',#5121,#5178,#4067,.T.);
#6636=EDGE_CURVE('',#5177,#5122,#4068,.T.);
#6637=EDGE_CURVE('',#4763,#4424,#4069,.T.);
#6638=EDGE_CURVE('',#5001,#4762,#4070,.T.);
#6639=EDGE_CURVE('',#4763,#4423,#4071,.T.);
#6640=EDGE_CURVE('',#5001,#4970,#4072,.T.);
#6641=EDGE_CURVE('',#4970,#4762,#4073,.T.);
#6642=EDGE_CURVE('',#4764,#4420,#4074,.T.);
#6643=EDGE_CURVE('',#4963,#4767,#670,.T.);
#6644=EDGE_CURVE('',#4491,#4969,#4075,.T.);
#6645=EDGE_CURVE('',#4421,#4558,#4076,.T.);
#6646=EDGE_CURVE('',#4558,#4422,#4077,.T.);
#6647=EDGE_CURVE('',#4764,#4419,#4078,.T.);
#6648=EDGE_CURVE('',#4963,#4800,#4079,.T.);
#6649=EDGE_CURVE('',#4801,#4767,#4080,.T.);
#6650=EDGE_CURVE('',#4492,#4968,#4081,.T.);
#6651=EDGE_CURVE('',#4559,#5000,#4082,.T.);
#6652=EDGE_CURVE('',#4418,#4557,#4083,.T.);
#6653=EDGE_CURVE('',#4765,#4887,#4084,.T.);
#6654=EDGE_CURVE('',#4766,#4777,#671,.T.);
#6655=EDGE_CURVE('',#4778,#4765,#4085,.T.);
#6656=EDGE_CURVE('',#4802,#4766,#4086,.T.);
#6657=EDGE_CURVE('',#4964,#4799,#4087,.T.);
#6658=EDGE_CURVE('',#4998,#4967,#4088,.T.);
#6659=EDGE_CURVE('',#4559,#4961,#4089,.T.);
#6660=EDGE_CURVE('',#4961,#5000,#4090,.T.);
#6661=EDGE_CURVE('',#4417,#4557,#4091,.T.);
#6662=EDGE_CURVE('',#4778,#4887,#4092,.T.);
#6663=EDGE_CURVE('',#4803,#4777,#4093,.T.);
#6664=EDGE_CURVE('',#4965,#4986,#4094,.T.);
#6665=EDGE_CURVE('',#4998,#4954,#4095,.T.);
#6666=EDGE_CURVE('',#4954,#4967,#4096,.T.);
#6667=EDGE_CURVE('',#4560,#4960,#672,.T.);
#6668=EDGE_CURVE('',#4886,#4563,#4097,.T.);
#6669=EDGE_CURVE('',#4779,#4565,#4098,.T.);
#6670=EDGE_CURVE('',#4804,#4776,#4099,.T.);
#6671=EDGE_CURVE('',#4966,#4985,#4100,.T.);
#6672=EDGE_CURVE('',#4955,#4966,#673,.T.);
#6673=EDGE_CURVE('',#4999,#4953,#4101,.T.);
#6674=EDGE_CURVE('',#4560,#4783,#4102,.T.);
#6675=EDGE_CURVE('',#4782,#4960,#4103,.T.);
#6676=EDGE_CURVE('',#4886,#4773,#4104,.T.);
#6677=EDGE_CURVE('',#4773,#4563,#4105,.T.);
#6678=EDGE_CURVE('',#4780,#4564,#4106,.T.);
#6679=EDGE_CURVE('',#4811,#4775,#4107,.T.);
#6680=EDGE_CURVE('',#4955,#4984,#4108,.T.);
#6681=EDGE_CURVE('',#4999,#4948,#4109,.T.);
#6682=EDGE_CURVE('',#4948,#4953,#4110,.T.);
#6683=EDGE_CURVE('',#4962,#4997,#4111,.T.);
#6684=EDGE_CURVE('',#4784,#4959,#4112,.T.);
#6685=EDGE_CURVE('',#4562,#4789,#4113,.T.);
#6686=EDGE_CURVE('',#4768,#4562,#674,.T.);
#6687=EDGE_CURVE('',#4781,#4891,#4114,.T.);
#6688=EDGE_CURVE('',#4774,#4761,#675,.T.);
#6689=EDGE_CURVE('',#4756,#4781,#4115,.T.);
#6690=EDGE_CURVE('',#4812,#4774,#4116,.T.);
#6691=EDGE_CURVE('',#4956,#4983,#4117,.T.);
#6692=EDGE_CURVE('',#4949,#4952,#4118,.T.);
#6693=EDGE_CURVE('',#4996,#4947,#4119,.T.);
#6694=EDGE_CURVE('',#4997,#4490,#4120,.T.);
#6695=EDGE_CURVE('',#4484,#4996,#4121,.T.);
#6696=EDGE_CURVE('',#4962,#4490,#4122,.T.);
#6697=EDGE_CURVE('',#4975,#4958,#4123,.T.);
#6698=EDGE_CURVE('',#4768,#4788,#4124,.T.);
#6699=EDGE_CURVE('',#4756,#4891,#4125,.T.);
#6700=EDGE_CURVE('',#4813,#4761,#4126,.T.);
#6701=EDGE_CURVE('',#4653,#4982,#4127,.T.);
#6702=EDGE_CURVE('',#4956,#4653,#676,.T.);
#6703=EDGE_CURVE('',#4949,#5088,#4128,.T.);
#6704=EDGE_CURVE('',#5088,#4952,#4129,.T.);
#6705=EDGE_CURVE('',#4484,#4947,#4130,.T.);
#6706=EDGE_CURVE('',#4957,#4489,#677,.T.);
#6707=EDGE_CURVE('',#4976,#4957,#4131,.T.);
#6708=EDGE_CURVE('',#4769,#4787,#4132,.T.);
#6709=EDGE_CURVE('',#4888,#4772,#4133,.T.);
#6710=EDGE_CURVE('',#4757,#4890,#4134,.T.);
#6711=EDGE_CURVE('',#4807,#4760,#4135,.T.);
#6712=EDGE_CURVE('',#4654,#4981,#4136,.T.);
#6713=EDGE_CURVE('',#4951,#4652,#4137,.T.);
#6714=EDGE_CURVE('',#5089,#4951,#4138,.T.);
#6715=EDGE_CURVE('',#4950,#5087,#4139,.T.);
#6716=EDGE_CURVE('',#4485,#4950,#4140,.T.);
#6717=EDGE_CURVE('',#4977,#4489,#4141,.T.);
#6718=EDGE_CURVE('',#4770,#4796,#4142,.T.);
#6719=EDGE_CURVE('',#4888,#4749,#4143,.T.);
#6720=EDGE_CURVE('',#4749,#4772,#4144,.T.);
#6721=EDGE_CURVE('',#4757,#4754,#4145,.T.);
#6722=EDGE_CURVE('',#4754,#4890,#4146,.T.);
#6723=EDGE_CURVE('',#5156,#4760,#678,.T.);
#6724=EDGE_CURVE('',#4806,#5156,#4147,.T.);
#6725=EDGE_CURVE('',#4649,#5071,#4148,.T.);
#6726=EDGE_CURVE('',#5089,#4652,#4149,.T.);
#6727=EDGE_CURVE('',#4485,#5087,#4150,.T.);
#6728=EDGE_CURVE('',#4978,#4487,#4151,.T.);
#6729=EDGE_CURVE('',#4771,#4795,#4152,.T.);
#6730=EDGE_CURVE('',#4750,#4771,#679,.T.);
#6731=EDGE_CURVE('',#4889,#4748,#4153,.T.);
#6732=EDGE_CURVE('',#4755,#4889,#4154,.T.);
#6733=EDGE_CURVE('',#4758,#4753,#4155,.T.);
#6734=EDGE_CURVE('',#4759,#5165,#4156,.T.);
#6735=EDGE_CURVE('',#5166,#4758,#4157,.T.);
#6736=EDGE_CURVE('',#5157,#4759,#4158,.T.);
#6737=EDGE_CURVE('',#4808,#5155,#4159,.T.);
#6738=EDGE_CURVE('',#4650,#5070,#4160,.T.);
#6739=EDGE_CURVE('',#4486,#5086,#4161,.T.);
#6740=EDGE_CURVE('',#4487,#4635,#680,.T.);
#6741=EDGE_CURVE('',#4636,#4486,#4162,.T.);
#6742=EDGE_CURVE('',#4971,#4635,#4163,.T.);
#6743=EDGE_CURVE('',#4750,#4794,#4164,.T.);
#6744=EDGE_CURVE('',#4755,#4748,#4165,.T.);
#6745=EDGE_CURVE('',#5166,#4753,#4166,.T.);
#6746=EDGE_CURVE('',#5157,#5165,#4167,.T.);
#6747=EDGE_CURVE('',#5066,#5154,#4168,.T.);
#6748=EDGE_CURVE('',#5055,#5069,#4169,.T.);
#6749=EDGE_CURVE('',#4650,#5055,#681,.T.);
#6750=EDGE_CURVE('',#4636,#5086,#4170,.T.);
#6751=EDGE_CURVE('',#4972,#4634,#4171,.T.);
#6752=EDGE_CURVE('',#4751,#4793,#4172,.T.);
#6753=EDGE_CURVE('',#4752,#4747,#4173,.T.);
#6754=EDGE_CURVE('',#5163,#4752,#4174,.T.);
#6755=EDGE_CURVE('',#5067,#5153,#4175,.T.);
#6756=EDGE_CURVE('',#5056,#5068,#4176,.T.);
#6757=EDGE_CURVE('',#4651,#5054,#4177,.T.);
#6758=EDGE_CURVE('',#5084,#4651,#4178,.T.);
#6759=EDGE_CURVE('',#4637,#4479,#4179,.T.);
#6760=EDGE_CURVE('',#5062,#4641,#4180,.T.);
#6761=EDGE_CURVE('',#5145,#4792,#4181,.T.);
#6762=EDGE_CURVE('',#4751,#5145,#682,.T.);
#6763=EDGE_CURVE('',#5163,#4747,#4182,.T.);
#6764=EDGE_CURVE('',#5056,#5153,#683,.T.);
#6765=EDGE_CURVE('',#5084,#5054,#4183,.T.);
#6766=EDGE_CURVE('',#4638,#4478,#4184,.T.);
#6767=EDGE_CURVE('',#5063,#4640,#4185,.T.);
#6768=EDGE_CURVE('',#5146,#4790,#4186,.T.);
#6769=EDGE_CURVE('',#4746,#5152,#4187,.T.);
#6770=EDGE_CURVE('',#5164,#4746,#4188,.T.);
#6771=EDGE_CURVE('',#5158,#5170,#4189,.T.);
#6772=EDGE_CURVE('',#5053,#5158,#4190,.T.);
#6773=EDGE_CURVE('',#5085,#4398,#4191,.T.);
#6774=EDGE_CURVE('',#4639,#5083,#4192,.T.);
#6775=EDGE_CURVE('',#4640,#4476,#684,.T.);
#6776=EDGE_CURVE('',#4477,#4639,#4193,.T.);
#6777=EDGE_CURVE('',#5064,#4476,#4194,.T.);
#6778=EDGE_CURVE('',#5147,#5059,#4195,.T.);
#6779=EDGE_CURVE('',#5164,#5152,#4196,.T.);
#6780=EDGE_CURVE('',#5053,#5170,#4197,.T.);
#6781=EDGE_CURVE('',#5085,#4400,#4198,.T.);
#6782=EDGE_CURVE('',#4477,#5083,#4199,.T.);
#6783=EDGE_CURVE('',#5058,#4474,#4200,.T.);
#6784=EDGE_CURVE('',#5148,#5057,#4201,.T.);
#6785=EDGE_CURVE('',#4465,#5151,#4202,.T.);
#6786=EDGE_CURVE('',#4397,#5169,#4203,.T.);
#6787=EDGE_CURVE('',#5082,#4394,#4204,.T.);
#6788=EDGE_CURVE('',#4396,#5082,#4205,.T.);
#6789=EDGE_CURVE('',#5148,#4474,#685,.T.);
#6790=EDGE_CURVE('',#4466,#5150,#4206,.T.);
#6791=EDGE_CURVE('',#4399,#5169,#4207,.T.);
#6792=EDGE_CURVE('',#5149,#4473,#4208,.T.);
#6793=EDGE_CURVE('',#5167,#5149,#4209,.T.);
#6794=EDGE_CURVE('',#4393,#5168,#4210,.T.);
#6795=EDGE_CURVE('',#5167,#4473,#4211,.T.);
#6796=EDGE_CURVE('',#4395,#5168,#4212,.T.);
#6797=EDGE_CURVE('',#5078,#5215,#686,.T.);
#6798=EDGE_CURVE('',#5081,#5216,#687,.T.);
#6799=EDGE_CURVE('',#5216,#5215,#688,.T.);
#6800=EDGE_CURVE('',#5216,#5075,#689,.T.);
#6801=EDGE_CURVE('',#5075,#5217,#690,.T.);
#6802=EDGE_CURVE('',#5217,#5215,#691,.T.);
#6803=EDGE_CURVE('',#5217,#4552,#692,.T.);
#6804=EDGE_CURVE('',#4499,#5215,#693,.T.);
#6805=EDGE_CURVE('',#4498,#5218,#694,.T.);
#6806=EDGE_CURVE('',#5218,#5215,#695,.T.);
#6807=EDGE_CURVE('',#5218,#5160,#696,.T.);
#6808=EDGE_CURVE('',#5219,#5160,#697,.T.);
#6809=EDGE_CURVE('',#5219,#5215,#698,.T.);
#6810=EDGE_CURVE('',#5220,#5221,#699,.T.);
#6811=EDGE_CURVE('',#5220,#4991,#700,.T.);
#6812=EDGE_CURVE('',#4992,#5221,#701,.T.);
#6813=EDGE_CURVE('',#4995,#5222,#702,.T.);
#6814=EDGE_CURVE('',#5222,#5221,#703,.T.);
#6815=EDGE_CURVE('',#5222,#4989,#704,.T.);
#6816=EDGE_CURVE('',#4989,#5223,#705,.T.);
#6817=EDGE_CURVE('',#5223,#5221,#706,.T.);
#6818=EDGE_CURVE('',#5223,#4555,#707,.T.);
#6819=EDGE_CURVE('',#4554,#5221,#708,.T.);
#6820=EDGE_CURVE('',#5224,#4553,#4213,.T.);
#6821=EDGE_CURVE('',#5224,#5221,#709,.T.);
#6822=EDGE_CURVE('',#4496,#5225,#710,.T.);
#6823=EDGE_CURVE('',#4495,#5226,#711,.T.);
#6824=EDGE_CURVE('',#5226,#5225,#712,.T.);
#6825=EDGE_CURVE('',#5226,#4873,#713,.T.);
#6826=EDGE_CURVE('',#4873,#5227,#714,.T.);
#6827=EDGE_CURVE('',#5227,#5225,#715,.T.);
#6828=EDGE_CURVE('',#5227,#4690,#716,.T.);
#6829=EDGE_CURVE('',#4688,#5225,#717,.T.);
#6830=EDGE_CURVE('',#4689,#5228,#718,.T.);
#6831=EDGE_CURVE('',#5228,#5225,#719,.T.);
#6832=EDGE_CURVE('',#5228,#5161,#720,.T.);
#6833=EDGE_CURVE('',#5229,#5161,#721,.T.);
#6834=EDGE_CURVE('',#5229,#5225,#722,.T.);
#6835=EDGE_CURVE('',#5230,#5231,#723,.T.);
#6836=EDGE_CURVE('',#5230,#4876,#724,.T.);
#6837=EDGE_CURVE('',#4877,#5231,#725,.T.);
#6838=EDGE_CURVE('',#4880,#5232,#726,.T.);
#6839=EDGE_CURVE('',#5232,#5231,#727,.T.);
#6840=EDGE_CURVE('',#5232,#4874,#728,.T.);
#6841=EDGE_CURVE('',#5233,#4874,#729,.T.);
#6842=EDGE_CURVE('',#5233,#5231,#730,.T.);
#6843=EDGE_CURVE('',#4493,#5233,#4214,.T.);
#6844=EDGE_CURVE('',#4494,#5231,#731,.T.);
#6845=EDGE_CURVE('',#5234,#4556,#4215,.T.);
#6846=EDGE_CURVE('',#5234,#5231,#732,.T.);
#6847=EDGE_CURVE('',#4616,#4878,#4216,.T.);
#6848=EDGE_CURVE('',#4879,#4615,#4217,.T.);
#6849=EDGE_CURVE('',#4987,#4878,#733,.T.);
#6850=EDGE_CURVE('',#4617,#4987,#4218,.T.);
#6851=EDGE_CURVE('',#4875,#4614,#4219,.T.);
#6852=EDGE_CURVE('',#4879,#4875,#734,.T.);
#6853=EDGE_CURVE('',#4988,#5230,#735,.T.);
#6854=EDGE_CURVE('',#4618,#4990,#4220,.T.);
#6855=EDGE_CURVE('',#4605,#4993,#4221,.T.);
#6856=EDGE_CURVE('',#4994,#4619,#4222,.T.);
#6857=EDGE_CURVE('',#4872,#4613,#4223,.T.);
#6858=EDGE_CURVE('',#4988,#5234,#736,.T.);
#6859=EDGE_CURVE('',#4994,#4990,#737,.T.);
#6860=EDGE_CURVE('',#5073,#4993,#738,.T.);
#6861=EDGE_CURVE('',#4604,#5073,#4224,.T.);
#6862=EDGE_CURVE('',#4691,#4612,#4225,.T.);
#6863=EDGE_CURVE('',#4872,#4691,#739,.T.);
#6864=EDGE_CURVE('',#5074,#5220,#740,.T.);
#6865=EDGE_CURVE('',#4606,#5076,#4226,.T.);
#6866=EDGE_CURVE('',#4692,#4611,#4227,.T.);
#6867=EDGE_CURVE('',#5162,#4692,#741,.T.);
#6868=EDGE_CURVE('',#4497,#5229,#4228,.T.);
#6869=EDGE_CURVE('',#5074,#5224,#742,.T.);
#6870=EDGE_CURVE('',#5080,#5076,#743,.T.);
#6871=EDGE_CURVE('',#4607,#5080,#4229,.T.);
#6872=EDGE_CURVE('',#5162,#4610,#4230,.T.);
#6873=EDGE_CURVE('',#4608,#5079,#4231,.T.);
#6874=EDGE_CURVE('',#5159,#4609,#4232,.T.);
#6875=EDGE_CURVE('',#5077,#5219,#4233,.T.);
#6876=EDGE_CURVE('',#5159,#5079,#744,.T.);
#6877=EDGE_CURVE('',#4814,#4974,#4234,.T.);
#6878=EDGE_CURVE('',#4785,#4840,#4235,.T.);
#6879=EDGE_CURVE('',#4786,#4839,#4236,.T.);
#6880=EDGE_CURVE('',#4815,#4973,#4237,.T.);
#6881=EDGE_CURVE('',#4797,#4838,#4238,.T.);
#6882=EDGE_CURVE('',#4835,#5061,#4239,.T.);
#6883=EDGE_CURVE('',#4791,#4837,#4240,.T.);
#6884=EDGE_CURVE('',#4836,#5060,#4241,.T.);
#6885=EDGE_CURVE('',#4979,#4583,#4242,.T.);
#6886=EDGE_CURVE('',#4584,#4798,#4243,.T.);
#6887=EDGE_CURVE('',#4585,#4805,#4244,.T.);
#6888=EDGE_CURVE('',#4980,#4582,#4245,.T.);
#6889=EDGE_CURVE('',#4586,#4810,#4246,.T.);
#6890=EDGE_CURVE('',#5072,#4589,#4247,.T.);
#6891=EDGE_CURVE('',#4587,#4809,#4248,.T.);
#6892=EDGE_CURVE('',#5065,#4588,#4249,.T.);
#6893=EDGE_CURVE('',#4574,#4472,#4250,.T.);
#6894=EDGE_CURVE('',#4575,#5110,#4251,.T.);
#6895=EDGE_CURVE('',#4580,#5107,#4252,.T.);
#6896=EDGE_CURVE('',#4469,#4579,#4253,.T.);
#6897=EDGE_CURVE('',#4576,#5109,#4254,.T.);
#6898=EDGE_CURVE('',#4470,#4578,#4255,.T.);
#6899=EDGE_CURVE('',#4577,#5104,#4256,.T.);
#6900=EDGE_CURVE('',#4471,#5119,#4257,.T.);
#6901=EDGE_CURVE('',#5111,#5118,#4258,.T.);
#6902=EDGE_CURVE('',#5112,#5106,#4259,.T.);
#6903=EDGE_CURVE('',#5114,#4468,#4260,.T.);
#6904=EDGE_CURVE('',#5108,#5117,#4261,.T.);
#6905=EDGE_CURVE('',#5115,#4467,#4262,.T.);
#6906=EDGE_CURVE('',#5105,#5116,#4263,.T.);
#6907=EDGE_CURVE('',#5018,#4598,#4264,.T.);
#6908=EDGE_CURVE('',#4599,#5019,#4265,.T.);
#6909=EDGE_CURVE('',#4482,#4597,#4266,.T.);
#6910=EDGE_CURVE('',#4483,#4596,#4267,.T.);
#6911=EDGE_CURVE('',#5021,#5017,#4268,.T.);
#6912=EDGE_CURVE('',#5020,#5024,#4269,.T.);
#6913=EDGE_CURVE('',#5022,#4481,#4270,.T.);
#6914=EDGE_CURVE('',#5023,#4480,#4271,.T.);
#6915=EDGE_CURVE('',#4913,#4601,#4272,.T.);
#6916=EDGE_CURVE('',#4602,#4916,#4273,.T.);
#6917=EDGE_CURVE('',#4603,#4915,#4274,.T.);
#6918=EDGE_CURVE('',#4600,#4910,#4275,.T.);
#6919=EDGE_CURVE('',#4918,#4912,#4276,.T.);
#6920=EDGE_CURVE('',#4917,#4921,#4277,.T.);
#6921=EDGE_CURVE('',#4914,#4920,#4278,.T.);
#6922=EDGE_CURVE('',#4911,#4919,#4279,.T.);
#6923=EDGE_CURVE('',#4675,#4726,#2940,.T.);
#6924=EDGE_CURVE('',#4676,#4725,#2941,.T.);
#6925=EDGE_CURVE('',#4706,#4674,#2942,.T.);
#6926=EDGE_CURVE('',#4673,#4705,#2943,.T.);
#6927=EDGE_CURVE('',#4831,#4629,#2944,.T.);
#6928=EDGE_CURVE('',#4830,#4677,#2945,.T.);
#6929=EDGE_CURVE('',#5235,#4566,#2946,.T.);
#6930=EDGE_CURVE('',#4630,#5235,#2947,.T.);
#6931=EDGE_CURVE('',#5236,#4818,#2948,.T.);
#6932=EDGE_CURVE('',#4567,#5236,#2949,.T.);
#6933=EDGE_CURVE('',#4633,#4816,#2950,.T.);
#6934=EDGE_CURVE('',#4632,#4817,#2951,.T.);
#6935=EDGE_CURVE('',#4631,#5237,#2952,.T.);
#6936=EDGE_CURVE('',#5236,#5237,#2953,.T.);
#6937=EDGE_CURVE('',#5235,#5237,#2954,.T.);
#6938=EDGE_CURVE('',#4644,#4834,#2955,.T.);
#6939=EDGE_CURVE('',#4645,#4833,#2956,.T.);
#6940=EDGE_CURVE('',#4628,#4832,#2957,.T.);
#6941=EDGE_CURVE('',#4572,#4647,#2958,.T.);
#6942=EDGE_CURVE('',#4573,#4659,#2959,.T.);
#6943=EDGE_CURVE('',#5120,#4658,#2960,.T.);
#6944=EDGE_CURVE('',#4581,#4655,#2961,.T.);
#6945=EDGE_CURVE('',#4580,#4656,#2962,.T.);
#6946=EDGE_CURVE('',#5113,#4657,#2963,.T.);
#7051=ORIENTED_EDGE('',*,*,#5307,.F.);
#7052=ORIENTED_EDGE('',*,*,#5308,.T.);
#7053=ORIENTED_EDGE('',*,*,#5309,.T.);
#7054=ORIENTED_EDGE('',*,*,#5308,.F.);
#7055=ORIENTED_EDGE('',*,*,#5310,.F.);
#7056=ORIENTED_EDGE('',*,*,#5311,.T.);
#7057=ORIENTED_EDGE('',*,*,#5312,.T.);
#7058=ORIENTED_EDGE('',*,*,#5311,.F.);
#7059=ORIENTED_EDGE('',*,*,#5313,.F.);
#7060=ORIENTED_EDGE('',*,*,#5314,.T.);
#7061=ORIENTED_EDGE('',*,*,#5315,.T.);
#7062=ORIENTED_EDGE('',*,*,#5314,.F.);
#7063=ORIENTED_EDGE('',*,*,#5316,.F.);
#7064=ORIENTED_EDGE('',*,*,#5317,.T.);
#7065=ORIENTED_EDGE('',*,*,#5318,.T.);
#7066=ORIENTED_EDGE('',*,*,#5317,.F.);
#7067=ORIENTED_EDGE('',*,*,#5319,.F.);
#7068=ORIENTED_EDGE('',*,*,#5320,.F.);
#7069=ORIENTED_EDGE('',*,*,#5321,.T.);
#7070=ORIENTED_EDGE('',*,*,#5322,.F.);
#7071=ORIENTED_EDGE('',*,*,#5321,.F.);
#7072=ORIENTED_EDGE('',*,*,#5323,.F.);
#7073=ORIENTED_EDGE('',*,*,#5324,.T.);
#7074=ORIENTED_EDGE('',*,*,#5325,.F.);
#7075=ORIENTED_EDGE('',*,*,#5326,.F.);
#7076=ORIENTED_EDGE('',*,*,#5324,.F.);
#7077=ORIENTED_EDGE('',*,*,#5327,.F.);
#7078=ORIENTED_EDGE('',*,*,#5328,.T.);
#7079=ORIENTED_EDGE('',*,*,#5329,.F.);
#7080=ORIENTED_EDGE('',*,*,#5328,.F.);
#7081=ORIENTED_EDGE('',*,*,#5330,.F.);
#7082=ORIENTED_EDGE('',*,*,#5331,.T.);
#7083=ORIENTED_EDGE('',*,*,#5332,.F.);
#7084=ORIENTED_EDGE('',*,*,#5333,.F.);
#7085=ORIENTED_EDGE('',*,*,#5331,.F.);
#7086=ORIENTED_EDGE('',*,*,#5334,.F.);
#7087=ORIENTED_EDGE('',*,*,#5335,.T.);
#7088=ORIENTED_EDGE('',*,*,#5336,.F.);
#7089=ORIENTED_EDGE('',*,*,#5337,.F.);
#7090=ORIENTED_EDGE('',*,*,#5338,.F.);
#7091=ORIENTED_EDGE('',*,*,#5339,.F.);
#7092=ORIENTED_EDGE('',*,*,#5340,.F.);
#7093=ORIENTED_EDGE('',*,*,#5341,.F.);
#7094=ORIENTED_EDGE('',*,*,#5342,.F.);
#7095=ORIENTED_EDGE('',*,*,#5343,.F.);
#7096=ORIENTED_EDGE('',*,*,#5344,.F.);
#7097=ORIENTED_EDGE('',*,*,#5345,.T.);
#7098=ORIENTED_EDGE('',*,*,#5346,.F.);
#7099=ORIENTED_EDGE('',*,*,#5347,.F.);
#7100=ORIENTED_EDGE('',*,*,#5348,.F.);
#7101=ORIENTED_EDGE('',*,*,#5349,.F.);
#7102=ORIENTED_EDGE('',*,*,#5350,.F.);
#7103=ORIENTED_EDGE('',*,*,#5351,.F.);
#7104=ORIENTED_EDGE('',*,*,#5352,.T.);
#7105=ORIENTED_EDGE('',*,*,#5353,.F.);
#7106=ORIENTED_EDGE('',*,*,#5352,.F.);
#7107=ORIENTED_EDGE('',*,*,#5354,.F.);
#7108=ORIENTED_EDGE('',*,*,#5355,.T.);
#7109=ORIENTED_EDGE('',*,*,#5356,.F.);
#7110=ORIENTED_EDGE('',*,*,#5357,.F.);
#7111=ORIENTED_EDGE('',*,*,#5355,.F.);
#7112=ORIENTED_EDGE('',*,*,#5358,.F.);
#7113=ORIENTED_EDGE('',*,*,#5359,.T.);
#7114=ORIENTED_EDGE('',*,*,#5360,.F.);
#7115=ORIENTED_EDGE('',*,*,#5361,.F.);
#7116=ORIENTED_EDGE('',*,*,#5359,.F.);
#7117=ORIENTED_EDGE('',*,*,#5362,.F.);
#7118=ORIENTED_EDGE('',*,*,#5363,.T.);
#7119=ORIENTED_EDGE('',*,*,#5364,.F.);
#7120=ORIENTED_EDGE('',*,*,#5365,.F.);
#7121=ORIENTED_EDGE('',*,*,#5363,.F.);
#7122=ORIENTED_EDGE('',*,*,#5366,.F.);
#7123=ORIENTED_EDGE('',*,*,#5367,.F.);
#7124=ORIENTED_EDGE('',*,*,#5368,.F.);
#7125=ORIENTED_EDGE('',*,*,#5369,.T.);
#7126=ORIENTED_EDGE('',*,*,#5370,.F.);
#7127=ORIENTED_EDGE('',*,*,#5371,.F.);
#7128=ORIENTED_EDGE('',*,*,#5372,.F.);
#7129=ORIENTED_EDGE('',*,*,#5373,.F.);
#7130=ORIENTED_EDGE('',*,*,#5374,.F.);
#7131=ORIENTED_EDGE('',*,*,#5375,.T.);
#7132=ORIENTED_EDGE('',*,*,#5376,.F.);
#7133=ORIENTED_EDGE('',*,*,#5377,.F.);
#7134=ORIENTED_EDGE('',*,*,#5378,.F.);
#7135=ORIENTED_EDGE('',*,*,#5379,.F.);
#7136=ORIENTED_EDGE('',*,*,#5380,.F.);
#7137=ORIENTED_EDGE('',*,*,#5381,.F.);
#7138=ORIENTED_EDGE('',*,*,#5382,.F.);
#7139=ORIENTED_EDGE('',*,*,#5383,.T.);
#7140=ORIENTED_EDGE('',*,*,#5384,.F.);
#7141=ORIENTED_EDGE('',*,*,#5383,.F.);
#7142=ORIENTED_EDGE('',*,*,#5385,.F.);
#7143=ORIENTED_EDGE('',*,*,#5386,.T.);
#7144=ORIENTED_EDGE('',*,*,#5387,.F.);
#7145=ORIENTED_EDGE('',*,*,#5386,.F.);
#7146=ORIENTED_EDGE('',*,*,#5388,.F.);
#7147=ORIENTED_EDGE('',*,*,#5389,.T.);
#7148=ORIENTED_EDGE('',*,*,#5390,.F.);
#7149=ORIENTED_EDGE('',*,*,#5391,.F.);
#7150=ORIENTED_EDGE('',*,*,#5389,.F.);
#7151=ORIENTED_EDGE('',*,*,#5392,.F.);
#7152=ORIENTED_EDGE('',*,*,#5393,.T.);
#7153=ORIENTED_EDGE('',*,*,#5394,.F.);
#7154=ORIENTED_EDGE('',*,*,#5393,.F.);
#7155=ORIENTED_EDGE('',*,*,#5395,.F.);
#7156=ORIENTED_EDGE('',*,*,#5396,.T.);
#7157=ORIENTED_EDGE('',*,*,#5397,.F.);
#7158=ORIENTED_EDGE('',*,*,#5398,.F.);
#7159=ORIENTED_EDGE('',*,*,#5399,.F.);
#7160=ORIENTED_EDGE('',*,*,#5400,.F.);
#7161=ORIENTED_EDGE('',*,*,#5401,.F.);
#7162=ORIENTED_EDGE('',*,*,#5402,.T.);
#7163=ORIENTED_EDGE('',*,*,#5403,.F.);
#7164=ORIENTED_EDGE('',*,*,#5404,.T.);
#7165=ORIENTED_EDGE('',*,*,#5405,.F.);
#7166=ORIENTED_EDGE('',*,*,#5404,.F.);
#7167=ORIENTED_EDGE('',*,*,#5406,.F.);
#7168=ORIENTED_EDGE('',*,*,#5407,.F.);
#7169=ORIENTED_EDGE('',*,*,#5408,.T.);
#7170=ORIENTED_EDGE('',*,*,#5409,.F.);
#7171=ORIENTED_EDGE('',*,*,#5410,.F.);
#7172=ORIENTED_EDGE('',*,*,#5408,.F.);
#7173=ORIENTED_EDGE('',*,*,#5411,.F.);
#7174=ORIENTED_EDGE('',*,*,#5412,.T.);
#7175=ORIENTED_EDGE('',*,*,#5413,.F.);
#7176=ORIENTED_EDGE('',*,*,#5414,.F.);
#7177=ORIENTED_EDGE('',*,*,#5412,.F.);
#7178=ORIENTED_EDGE('',*,*,#5415,.F.);
#7179=ORIENTED_EDGE('',*,*,#5416,.T.);
#7180=ORIENTED_EDGE('',*,*,#5417,.F.);
#7181=ORIENTED_EDGE('',*,*,#5418,.F.);
#7182=ORIENTED_EDGE('',*,*,#5416,.F.);
#7183=ORIENTED_EDGE('',*,*,#5419,.F.);
#7184=ORIENTED_EDGE('',*,*,#5420,.F.);
#7185=ORIENTED_EDGE('',*,*,#5421,.F.);
#7186=ORIENTED_EDGE('',*,*,#5422,.T.);
#7187=ORIENTED_EDGE('',*,*,#5423,.F.);
#7188=ORIENTED_EDGE('',*,*,#5424,.F.);
#7189=ORIENTED_EDGE('',*,*,#5425,.F.);
#7190=ORIENTED_EDGE('',*,*,#5426,.T.);
#7191=ORIENTED_EDGE('',*,*,#5427,.F.);
#7192=ORIENTED_EDGE('',*,*,#5428,.T.);
#7193=ORIENTED_EDGE('',*,*,#5429,.F.);
#7194=ORIENTED_EDGE('',*,*,#5430,.F.);
#7195=ORIENTED_EDGE('',*,*,#5431,.F.);
#7196=ORIENTED_EDGE('',*,*,#5432,.F.);
#7197=ORIENTED_EDGE('',*,*,#5433,.F.);
#7198=ORIENTED_EDGE('',*,*,#5434,.T.);
#7199=ORIENTED_EDGE('',*,*,#5435,.F.);
#7200=ORIENTED_EDGE('',*,*,#5436,.F.);
#7201=ORIENTED_EDGE('',*,*,#5437,.F.);
#7202=ORIENTED_EDGE('',*,*,#5438,.T.);
#7203=ORIENTED_EDGE('',*,*,#5439,.F.);
#7204=ORIENTED_EDGE('',*,*,#5440,.T.);
#7205=ORIENTED_EDGE('',*,*,#5441,.F.);
#7206=ORIENTED_EDGE('',*,*,#5442,.F.);
#7207=ORIENTED_EDGE('',*,*,#5443,.F.);
#7208=ORIENTED_EDGE('',*,*,#5444,.F.);
#7209=ORIENTED_EDGE('',*,*,#5445,.T.);
#7210=ORIENTED_EDGE('',*,*,#5446,.F.);
#7211=ORIENTED_EDGE('',*,*,#5447,.F.);
#7212=ORIENTED_EDGE('',*,*,#5448,.F.);
#7213=ORIENTED_EDGE('',*,*,#5449,.T.);
#7214=ORIENTED_EDGE('',*,*,#5450,.F.);
#7215=ORIENTED_EDGE('',*,*,#5451,.T.);
#7216=ORIENTED_EDGE('',*,*,#5452,.F.);
#7217=ORIENTED_EDGE('',*,*,#5453,.F.);
#7218=ORIENTED_EDGE('',*,*,#5454,.F.);
#7219=ORIENTED_EDGE('',*,*,#5451,.F.);
#7220=ORIENTED_EDGE('',*,*,#5455,.T.);
#7221=ORIENTED_EDGE('',*,*,#5456,.F.);
#7222=ORIENTED_EDGE('',*,*,#5457,.F.);
#7223=ORIENTED_EDGE('',*,*,#5458,.T.);
#7224=ORIENTED_EDGE('',*,*,#5459,.F.);
#7225=ORIENTED_EDGE('',*,*,#5460,.F.);
#7226=ORIENTED_EDGE('',*,*,#5461,.F.);
#7227=ORIENTED_EDGE('',*,*,#5462,.F.);
#7228=ORIENTED_EDGE('',*,*,#5463,.F.);
#7229=ORIENTED_EDGE('',*,*,#5464,.T.);
#7230=ORIENTED_EDGE('',*,*,#5465,.F.);
#7231=ORIENTED_EDGE('',*,*,#5466,.T.);
#7232=ORIENTED_EDGE('',*,*,#5467,.F.);
#7233=ORIENTED_EDGE('',*,*,#5468,.F.);
#7234=ORIENTED_EDGE('',*,*,#5469,.F.);
#7235=ORIENTED_EDGE('',*,*,#5470,.F.);
#7236=ORIENTED_EDGE('',*,*,#5471,.F.);
#7237=ORIENTED_EDGE('',*,*,#5472,.T.);
#7238=ORIENTED_EDGE('',*,*,#5473,.F.);
#7239=ORIENTED_EDGE('',*,*,#5474,.F.);
#7240=ORIENTED_EDGE('',*,*,#5475,.T.);
#7241=ORIENTED_EDGE('',*,*,#5476,.F.);
#7242=ORIENTED_EDGE('',*,*,#5477,.T.);
#7243=ORIENTED_EDGE('',*,*,#5478,.F.);
#7244=ORIENTED_EDGE('',*,*,#5479,.F.);
#7245=ORIENTED_EDGE('',*,*,#5480,.F.);
#7246=ORIENTED_EDGE('',*,*,#5481,.T.);
#7247=ORIENTED_EDGE('',*,*,#5482,.F.);
#7248=ORIENTED_EDGE('',*,*,#5483,.T.);
#7249=ORIENTED_EDGE('',*,*,#5484,.F.);
#7250=ORIENTED_EDGE('',*,*,#5485,.F.);
#7251=ORIENTED_EDGE('',*,*,#5486,.T.);
#7252=ORIENTED_EDGE('',*,*,#5487,.F.);
#7253=ORIENTED_EDGE('',*,*,#5488,.T.);
#7254=ORIENTED_EDGE('',*,*,#5489,.F.);
#7255=ORIENTED_EDGE('',*,*,#5490,.T.);
#7256=ORIENTED_EDGE('',*,*,#5491,.T.);
#7257=ORIENTED_EDGE('',*,*,#5492,.T.);
#7258=ORIENTED_EDGE('',*,*,#5493,.T.);
#7259=ORIENTED_EDGE('',*,*,#5403,.T.);
#7260=ORIENTED_EDGE('',*,*,#5494,.T.);
#7261=ORIENTED_EDGE('',*,*,#5417,.T.);
#7262=ORIENTED_EDGE('',*,*,#5418,.T.);
#7263=ORIENTED_EDGE('',*,*,#5494,.F.);
#7264=ORIENTED_EDGE('',*,*,#5406,.T.);
#7265=ORIENTED_EDGE('',*,*,#5413,.T.);
#7266=ORIENTED_EDGE('',*,*,#5414,.T.);
#7267=ORIENTED_EDGE('',*,*,#5495,.T.);
#7268=ORIENTED_EDGE('',*,*,#5409,.T.);
#7269=ORIENTED_EDGE('',*,*,#5410,.T.);
#7270=ORIENTED_EDGE('',*,*,#5495,.F.);
#7271=ORIENTED_EDGE('',*,*,#5429,.T.);
#7272=ORIENTED_EDGE('',*,*,#5496,.F.);
#7273=ORIENTED_EDGE('',*,*,#5497,.T.);
#7274=ORIENTED_EDGE('',*,*,#5498,.F.);
#7275=ORIENTED_EDGE('',*,*,#5499,.T.);
#7276=ORIENTED_EDGE('',*,*,#5500,.F.);
#7277=ORIENTED_EDGE('',*,*,#5501,.T.);
#7278=ORIENTED_EDGE('',*,*,#5502,.F.);
#7279=ORIENTED_EDGE('',*,*,#5503,.T.);
#7280=ORIENTED_EDGE('',*,*,#5504,.T.);
#7281=ORIENTED_EDGE('',*,*,#5505,.T.);
#7282=ORIENTED_EDGE('',*,*,#5506,.T.);
#7283=ORIENTED_EDGE('',*,*,#5382,.T.);
#7284=ORIENTED_EDGE('',*,*,#5507,.T.);
#7285=ORIENTED_EDGE('',*,*,#5394,.T.);
#7286=ORIENTED_EDGE('',*,*,#5507,.F.);
#7287=ORIENTED_EDGE('',*,*,#5390,.T.);
#7288=ORIENTED_EDGE('',*,*,#5391,.T.);
#7289=ORIENTED_EDGE('',*,*,#5508,.T.);
#7290=ORIENTED_EDGE('',*,*,#5387,.T.);
#7291=ORIENTED_EDGE('',*,*,#5508,.F.);
#7292=ORIENTED_EDGE('',*,*,#5421,.T.);
#7293=ORIENTED_EDGE('',*,*,#5509,.T.);
#7294=ORIENTED_EDGE('',*,*,#5510,.T.);
#7295=ORIENTED_EDGE('',*,*,#5511,.T.);
#7296=ORIENTED_EDGE('',*,*,#5512,.T.);
#7297=ORIENTED_EDGE('',*,*,#5513,.T.);
#7298=ORIENTED_EDGE('',*,*,#5514,.T.);
#7299=ORIENTED_EDGE('',*,*,#5433,.T.);
#7300=ORIENTED_EDGE('',*,*,#5515,.F.);
#7301=ORIENTED_EDGE('',*,*,#5516,.T.);
#7302=ORIENTED_EDGE('',*,*,#5517,.F.);
#7303=ORIENTED_EDGE('',*,*,#5518,.T.);
#7304=ORIENTED_EDGE('',*,*,#5519,.F.);
#7305=ORIENTED_EDGE('',*,*,#5520,.T.);
#7306=ORIENTED_EDGE('',*,*,#5521,.F.);
#7307=ORIENTED_EDGE('',*,*,#5370,.T.);
#7308=ORIENTED_EDGE('',*,*,#5522,.T.);
#7309=ORIENTED_EDGE('',*,*,#5378,.T.);
#7310=ORIENTED_EDGE('',*,*,#5523,.T.);
#7311=ORIENTED_EDGE('',*,*,#5350,.T.);
#7312=ORIENTED_EDGE('',*,*,#5351,.T.);
#7313=ORIENTED_EDGE('',*,*,#5524,.T.);
#7314=ORIENTED_EDGE('',*,*,#5364,.T.);
#7315=ORIENTED_EDGE('',*,*,#5365,.T.);
#7316=ORIENTED_EDGE('',*,*,#5524,.F.);
#7317=ORIENTED_EDGE('',*,*,#5361,.T.);
#7318=ORIENTED_EDGE('',*,*,#5525,.T.);
#7319=ORIENTED_EDGE('',*,*,#5356,.T.);
#7320=ORIENTED_EDGE('',*,*,#5357,.T.);
#7321=ORIENTED_EDGE('',*,*,#5525,.F.);
#7322=ORIENTED_EDGE('',*,*,#5360,.T.);
#7323=ORIENTED_EDGE('',*,*,#5526,.T.);
#7324=ORIENTED_EDGE('',*,*,#5527,.T.);
#7325=ORIENTED_EDGE('',*,*,#5528,.T.);
#7326=ORIENTED_EDGE('',*,*,#5529,.T.);
#7327=ORIENTED_EDGE('',*,*,#5530,.T.);
#7328=ORIENTED_EDGE('',*,*,#5531,.T.);
#7329=ORIENTED_EDGE('',*,*,#5532,.T.);
#7330=ORIENTED_EDGE('',*,*,#5533,.T.);
#7331=ORIENTED_EDGE('',*,*,#5534,.F.);
#7332=ORIENTED_EDGE('',*,*,#5441,.T.);
#7333=ORIENTED_EDGE('',*,*,#5535,.F.);
#7334=ORIENTED_EDGE('',*,*,#5336,.T.);
#7335=ORIENTED_EDGE('',*,*,#5536,.F.);
#7336=ORIENTED_EDGE('',*,*,#5344,.T.);
#7337=ORIENTED_EDGE('',*,*,#5537,.F.);
#7338=ORIENTED_EDGE('',*,*,#5338,.T.);
#7339=ORIENTED_EDGE('',*,*,#5538,.T.);
#7340=ORIENTED_EDGE('',*,*,#5346,.T.);
#7341=ORIENTED_EDGE('',*,*,#5539,.T.);
#7342=ORIENTED_EDGE('',*,*,#5540,.F.);
#7343=ORIENTED_EDGE('',*,*,#5541,.T.);
#7344=ORIENTED_EDGE('',*,*,#5542,.F.);
#7345=ORIENTED_EDGE('',*,*,#5543,.F.);
#7346=ORIENTED_EDGE('',*,*,#5544,.T.);
#7347=ORIENTED_EDGE('',*,*,#5545,.F.);
#7348=ORIENTED_EDGE('',*,*,#5546,.T.);
#7349=ORIENTED_EDGE('',*,*,#5547,.F.);
#7350=ORIENTED_EDGE('',*,*,#5548,.T.);
#7351=ORIENTED_EDGE('',*,*,#5549,.F.);
#7352=ORIENTED_EDGE('',*,*,#5550,.T.);
#7353=ORIENTED_EDGE('',*,*,#5551,.T.);
#7354=ORIENTED_EDGE('',*,*,#5552,.T.);
#7355=ORIENTED_EDGE('',*,*,#5553,.F.);
#7356=ORIENTED_EDGE('',*,*,#5554,.T.);
#7357=ORIENTED_EDGE('',*,*,#5555,.F.);
#7358=ORIENTED_EDGE('',*,*,#5556,.T.);
#7359=ORIENTED_EDGE('',*,*,#5557,.T.);
#7360=ORIENTED_EDGE('',*,*,#5459,.T.);
#7361=ORIENTED_EDGE('',*,*,#5558,.T.);
#7362=ORIENTED_EDGE('',*,*,#5559,.T.);
#7363=ORIENTED_EDGE('',*,*,#5560,.F.);
#7364=ORIENTED_EDGE('',*,*,#5561,.F.);
#7365=ORIENTED_EDGE('',*,*,#5562,.T.);
#7366=ORIENTED_EDGE('',*,*,#5563,.F.);
#7367=ORIENTED_EDGE('',*,*,#5564,.T.);
#7368=ORIENTED_EDGE('',*,*,#5565,.T.);
#7369=ORIENTED_EDGE('',*,*,#5463,.T.);
#7370=ORIENTED_EDGE('',*,*,#5566,.F.);
#7371=ORIENTED_EDGE('',*,*,#5567,.T.);
#7372=ORIENTED_EDGE('',*,*,#5568,.F.);
#7373=ORIENTED_EDGE('',*,*,#5569,.T.);
#7374=ORIENTED_EDGE('',*,*,#5570,.T.);
#7375=ORIENTED_EDGE('',*,*,#5571,.T.);
#7376=ORIENTED_EDGE('',*,*,#5572,.T.);
#7377=ORIENTED_EDGE('',*,*,#5573,.T.);
#7378=ORIENTED_EDGE('',*,*,#5574,.F.);
#7379=ORIENTED_EDGE('',*,*,#5575,.F.);
#7380=ORIENTED_EDGE('',*,*,#5576,.T.);
#7381=ORIENTED_EDGE('',*,*,#5577,.F.);
#7382=ORIENTED_EDGE('',*,*,#5578,.T.);
#7383=ORIENTED_EDGE('',*,*,#5579,.T.);
#7384=ORIENTED_EDGE('',*,*,#5580,.T.);
#7385=ORIENTED_EDGE('',*,*,#5581,.F.);
#7386=ORIENTED_EDGE('',*,*,#5582,.T.);
#7387=ORIENTED_EDGE('',*,*,#5583,.F.);
#7388=ORIENTED_EDGE('',*,*,#5473,.T.);
#7389=ORIENTED_EDGE('',*,*,#5584,.T.);
#7390=ORIENTED_EDGE('',*,*,#5585,.T.);
#7391=ORIENTED_EDGE('',*,*,#5586,.T.);
#7392=ORIENTED_EDGE('',*,*,#5587,.T.);
#7393=ORIENTED_EDGE('',*,*,#5588,.F.);
#7394=ORIENTED_EDGE('',*,*,#5589,.F.);
#7395=ORIENTED_EDGE('',*,*,#5590,.T.);
#7396=ORIENTED_EDGE('',*,*,#5591,.F.);
#7397=ORIENTED_EDGE('',*,*,#5469,.T.);
#7398=ORIENTED_EDGE('',*,*,#5592,.T.);
#7399=ORIENTED_EDGE('',*,*,#5593,.T.);
#7400=ORIENTED_EDGE('',*,*,#5594,.F.);
#7401=ORIENTED_EDGE('',*,*,#5595,.T.);
#7402=ORIENTED_EDGE('',*,*,#5596,.F.);
#7403=ORIENTED_EDGE('',*,*,#5597,.T.);
#7404=ORIENTED_EDGE('',*,*,#5598,.T.);
#7405=ORIENTED_EDGE('',*,*,#5599,.T.);
#7406=ORIENTED_EDGE('',*,*,#5600,.T.);
#7407=ORIENTED_EDGE('',*,*,#5601,.T.);
#7408=ORIENTED_EDGE('',*,*,#5602,.F.);
#7409=ORIENTED_EDGE('',*,*,#5546,.F.);
#7410=ORIENTED_EDGE('',*,*,#5603,.F.);
#7411=ORIENTED_EDGE('',*,*,#5604,.T.);
#7412=ORIENTED_EDGE('',*,*,#5605,.F.);
#7413=ORIENTED_EDGE('',*,*,#5606,.F.);
#7414=ORIENTED_EDGE('',*,*,#5607,.T.);
#7415=ORIENTED_EDGE('',*,*,#5608,.F.);
#7416=ORIENTED_EDGE('',*,*,#5319,.T.);
#7417=ORIENTED_EDGE('',*,*,#5320,.T.);
#7418=ORIENTED_EDGE('',*,*,#5609,.T.);
#7419=ORIENTED_EDGE('',*,*,#5332,.T.);
#7420=ORIENTED_EDGE('',*,*,#5333,.T.);
#7421=ORIENTED_EDGE('',*,*,#5609,.F.);
#7422=ORIENTED_EDGE('',*,*,#5329,.T.);
#7423=ORIENTED_EDGE('',*,*,#5610,.T.);
#7424=ORIENTED_EDGE('',*,*,#5325,.T.);
#7425=ORIENTED_EDGE('',*,*,#5326,.T.);
#7426=ORIENTED_EDGE('',*,*,#5610,.F.);
#7427=ORIENTED_EDGE('',*,*,#5611,.T.);
#7428=ORIENTED_EDGE('',*,*,#5612,.T.);
#7429=ORIENTED_EDGE('',*,*,#5613,.T.);
#7430=ORIENTED_EDGE('',*,*,#5614,.T.);
#7431=ORIENTED_EDGE('',*,*,#5615,.T.);
#7432=ORIENTED_EDGE('',*,*,#5616,.T.);
#7433=ORIENTED_EDGE('',*,*,#5617,.T.);
#7434=ORIENTED_EDGE('',*,*,#5618,.T.);
#7435=ORIENTED_EDGE('',*,*,#5619,.F.);
#7436=ORIENTED_EDGE('',*,*,#5437,.T.);
#7437=ORIENTED_EDGE('',*,*,#5620,.F.);
#7438=ORIENTED_EDGE('',*,*,#5621,.F.);
#7439=ORIENTED_EDGE('',*,*,#5622,.T.);
#7440=ORIENTED_EDGE('',*,*,#5623,.T.);
#7441=ORIENTED_EDGE('',*,*,#5624,.F.);
#7442=ORIENTED_EDGE('',*,*,#5625,.T.);
#7443=ORIENTED_EDGE('',*,*,#5626,.F.);
#7444=ORIENTED_EDGE('',*,*,#5627,.F.);
#7445=ORIENTED_EDGE('',*,*,#5628,.T.);
#7446=ORIENTED_EDGE('',*,*,#5399,.T.);
#7447=ORIENTED_EDGE('',*,*,#5629,.T.);
#7448=ORIENTED_EDGE('',*,*,#5630,.T.);
#7449=ORIENTED_EDGE('',*,*,#5631,.T.);
#7450=ORIENTED_EDGE('',*,*,#5632,.T.);
#7451=ORIENTED_EDGE('',*,*,#5633,.T.);
#7452=ORIENTED_EDGE('',*,*,#5634,.T.);
#7453=ORIENTED_EDGE('',*,*,#5635,.T.);
#7454=ORIENTED_EDGE('',*,*,#5636,.F.);
#7455=ORIENTED_EDGE('',*,*,#5637,.T.);
#7456=ORIENTED_EDGE('',*,*,#5638,.T.);
#7457=ORIENTED_EDGE('',*,*,#5639,.T.);
#7458=ORIENTED_EDGE('',*,*,#5640,.T.);
#7459=ORIENTED_EDGE('',*,*,#5641,.T.);
#7460=ORIENTED_EDGE('',*,*,#5642,.T.);
#7461=ORIENTED_EDGE('',*,*,#5643,.T.);
#7462=ORIENTED_EDGE('',*,*,#5644,.T.);
#7463=ORIENTED_EDGE('',*,*,#5645,.T.);
#7464=ORIENTED_EDGE('',*,*,#5405,.T.);
#7465=ORIENTED_EDGE('',*,*,#5646,.T.);
#7466=ORIENTED_EDGE('',*,*,#5647,.T.);
#7467=ORIENTED_EDGE('',*,*,#5648,.T.);
#7468=ORIENTED_EDGE('',*,*,#5649,.T.);
#7469=ORIENTED_EDGE('',*,*,#5650,.T.);
#7470=ORIENTED_EDGE('',*,*,#5482,.T.);
#7471=ORIENTED_EDGE('',*,*,#5651,.T.);
#7472=ORIENTED_EDGE('',*,*,#5652,.T.);
#7473=ORIENTED_EDGE('',*,*,#5384,.T.);
#7474=ORIENTED_EDGE('',*,*,#5353,.T.);
#7475=ORIENTED_EDGE('',*,*,#5653,.T.);
#7476=ORIENTED_EDGE('',*,*,#5654,.T.);
#7477=ORIENTED_EDGE('',*,*,#5655,.T.);
#7478=ORIENTED_EDGE('',*,*,#5656,.T.);
#7479=ORIENTED_EDGE('',*,*,#5380,.T.);
#7480=ORIENTED_EDGE('',*,*,#5657,.T.);
#7481=ORIENTED_EDGE('',*,*,#5658,.T.);
#7482=ORIENTED_EDGE('',*,*,#5374,.T.);
#7483=ORIENTED_EDGE('',*,*,#5659,.T.);
#7484=ORIENTED_EDGE('',*,*,#5342,.T.);
#7485=ORIENTED_EDGE('',*,*,#5660,.T.);
#7486=ORIENTED_EDGE('',*,*,#5661,.T.);
#7487=ORIENTED_EDGE('',*,*,#5348,.T.);
#7488=ORIENTED_EDGE('',*,*,#5662,.T.);
#7489=ORIENTED_EDGE('',*,*,#5663,.T.);
#7490=ORIENTED_EDGE('',*,*,#5664,.T.);
#7491=ORIENTED_EDGE('',*,*,#5322,.T.);
#7492=ORIENTED_EDGE('',*,*,#5665,.F.);
#7493=ORIENTED_EDGE('',*,*,#5666,.T.);
#7494=ORIENTED_EDGE('',*,*,#5667,.F.);
#7495=ORIENTED_EDGE('',*,*,#5668,.T.);
#7496=ORIENTED_EDGE('',*,*,#5669,.F.);
#7497=ORIENTED_EDGE('',*,*,#5670,.T.);
#7498=ORIENTED_EDGE('',*,*,#5671,.F.);
#7499=ORIENTED_EDGE('',*,*,#5672,.T.);
#7500=ORIENTED_EDGE('',*,*,#5673,.F.);
#7501=ORIENTED_EDGE('',*,*,#5674,.T.);
#7502=ORIENTED_EDGE('',*,*,#5675,.F.);
#7503=ORIENTED_EDGE('',*,*,#5676,.T.);
#7504=ORIENTED_EDGE('',*,*,#5677,.F.);
#7505=ORIENTED_EDGE('',*,*,#5678,.T.);
#7506=ORIENTED_EDGE('',*,*,#5679,.F.);
#7507=ORIENTED_EDGE('',*,*,#5680,.T.);
#7508=ORIENTED_EDGE('',*,*,#5681,.F.);
#7509=ORIENTED_EDGE('',*,*,#5682,.T.);
#7510=ORIENTED_EDGE('',*,*,#5683,.T.);
#7511=ORIENTED_EDGE('',*,*,#5684,.T.);
#7512=ORIENTED_EDGE('',*,*,#5685,.F.);
#7513=ORIENTED_EDGE('',*,*,#5686,.T.);
#7514=ORIENTED_EDGE('',*,*,#5687,.T.);
#7515=ORIENTED_EDGE('',*,*,#5688,.T.);
#7516=ORIENTED_EDGE('',*,*,#5689,.T.);
#7517=ORIENTED_EDGE('',*,*,#5690,.F.);
#7518=ORIENTED_EDGE('',*,*,#5691,.F.);
#7519=ORIENTED_EDGE('',*,*,#5692,.F.);
#7520=ORIENTED_EDGE('',*,*,#5693,.F.);
#7521=ORIENTED_EDGE('',*,*,#5694,.T.);
#7522=ORIENTED_EDGE('',*,*,#5695,.T.);
#7523=ORIENTED_EDGE('',*,*,#5696,.T.);
#7524=ORIENTED_EDGE('',*,*,#5697,.T.);
#7525=ORIENTED_EDGE('',*,*,#5698,.T.);
#7526=ORIENTED_EDGE('',*,*,#5699,.T.);
#7527=ORIENTED_EDGE('',*,*,#5700,.T.);
#7528=ORIENTED_EDGE('',*,*,#5701,.T.);
#7529=ORIENTED_EDGE('',*,*,#5702,.T.);
#7530=ORIENTED_EDGE('',*,*,#5703,.T.);
#7531=ORIENTED_EDGE('',*,*,#5704,.F.);
#7532=ORIENTED_EDGE('',*,*,#5705,.F.);
#7533=ORIENTED_EDGE('',*,*,#5706,.F.);
#7534=ORIENTED_EDGE('',*,*,#5388,.T.);
#7535=ORIENTED_EDGE('',*,*,#5707,.F.);
#7536=ORIENTED_EDGE('',*,*,#5708,.T.);
#7537=ORIENTED_EDGE('',*,*,#5709,.T.);
#7538=ORIENTED_EDGE('',*,*,#5710,.T.);
#7539=ORIENTED_EDGE('',*,*,#5711,.T.);
#7540=ORIENTED_EDGE('',*,*,#5712,.T.);
#7541=ORIENTED_EDGE('',*,*,#5431,.T.);
#7542=ORIENTED_EDGE('',*,*,#5713,.T.);
#7543=ORIENTED_EDGE('',*,*,#5714,.T.);
#7544=ORIENTED_EDGE('',*,*,#5715,.T.);
#7545=ORIENTED_EDGE('',*,*,#5716,.T.);
#7546=ORIENTED_EDGE('',*,*,#5717,.F.);
#7547=ORIENTED_EDGE('',*,*,#5718,.T.);
#7548=ORIENTED_EDGE('',*,*,#5719,.T.);
#7549=ORIENTED_EDGE('',*,*,#5720,.F.);
#7550=ORIENTED_EDGE('',*,*,#5721,.F.);
#7551=ORIENTED_EDGE('',*,*,#5392,.T.);
#7552=ORIENTED_EDGE('',*,*,#5722,.F.);
#7553=ORIENTED_EDGE('',*,*,#5723,.T.);
#7554=ORIENTED_EDGE('',*,*,#5724,.T.);
#7555=ORIENTED_EDGE('',*,*,#5725,.T.);
#7556=ORIENTED_EDGE('',*,*,#5708,.F.);
#7557=ORIENTED_EDGE('',*,*,#5726,.T.);
#7558=ORIENTED_EDGE('',*,*,#5688,.F.);
#7559=ORIENTED_EDGE('',*,*,#5727,.F.);
#7560=ORIENTED_EDGE('',*,*,#5682,.F.);
#7561=ORIENTED_EDGE('',*,*,#5728,.T.);
#7562=ORIENTED_EDGE('',*,*,#5703,.F.);
#7563=ORIENTED_EDGE('',*,*,#5729,.F.);
#7564=ORIENTED_EDGE('',*,*,#5730,.F.);
#7565=ORIENTED_EDGE('',*,*,#5731,.T.);
#7566=ORIENTED_EDGE('',*,*,#5684,.F.);
#7567=ORIENTED_EDGE('',*,*,#5732,.F.);
#7568=ORIENTED_EDGE('',*,*,#5686,.F.);
#7569=ORIENTED_EDGE('',*,*,#5733,.T.);
#7570=ORIENTED_EDGE('',*,*,#5625,.F.);
#7571=ORIENTED_EDGE('',*,*,#5734,.F.);
#7572=ORIENTED_EDGE('',*,*,#5628,.F.);
#7573=ORIENTED_EDGE('',*,*,#5735,.T.);
#7574=ORIENTED_EDGE('',*,*,#5725,.F.);
#7575=ORIENTED_EDGE('',*,*,#5400,.T.);
#7576=ORIENTED_EDGE('',*,*,#5736,.F.);
#7577=ORIENTED_EDGE('',*,*,#5737,.F.);
#7578=ORIENTED_EDGE('',*,*,#5398,.T.);
#7579=ORIENTED_EDGE('',*,*,#5723,.F.);
#7580=ORIENTED_EDGE('',*,*,#5738,.T.);
#7581=ORIENTED_EDGE('',*,*,#5739,.T.);
#7582=ORIENTED_EDGE('',*,*,#5740,.T.);
#7583=ORIENTED_EDGE('',*,*,#5741,.T.);
#7584=ORIENTED_EDGE('',*,*,#5742,.F.);
#7585=ORIENTED_EDGE('',*,*,#5743,.F.);
#7586=ORIENTED_EDGE('',*,*,#5744,.F.);
#7587=ORIENTED_EDGE('',*,*,#5740,.F.);
#7588=ORIENTED_EDGE('',*,*,#5745,.F.);
#7589=ORIENTED_EDGE('',*,*,#5738,.F.);
#7590=ORIENTED_EDGE('',*,*,#5746,.T.);
#7591=ORIENTED_EDGE('',*,*,#5747,.F.);
#7592=ORIENTED_EDGE('',*,*,#5748,.T.);
#7593=ORIENTED_EDGE('',*,*,#5749,.T.);
#7594=ORIENTED_EDGE('',*,*,#5750,.T.);
#7595=ORIENTED_EDGE('',*,*,#5751,.F.);
#7596=ORIENTED_EDGE('',*,*,#5752,.F.);
#7597=ORIENTED_EDGE('',*,*,#5315,.F.);
#7598=ORIENTED_EDGE('',*,*,#5753,.F.);
#7599=ORIENTED_EDGE('',*,*,#5754,.F.);
#7600=ORIENTED_EDGE('',*,*,#5755,.T.);
#7601=ORIENTED_EDGE('',*,*,#5756,.T.);
#7602=ORIENTED_EDGE('',*,*,#5757,.T.);
#7603=ORIENTED_EDGE('',*,*,#5758,.F.);
#7604=ORIENTED_EDGE('',*,*,#5759,.F.);
#7605=ORIENTED_EDGE('',*,*,#5760,.T.);
#7606=ORIENTED_EDGE('',*,*,#5761,.T.);
#7607=ORIENTED_EDGE('',*,*,#5762,.T.);
#7608=ORIENTED_EDGE('',*,*,#5763,.F.);
#7609=ORIENTED_EDGE('',*,*,#5764,.F.);
#7610=ORIENTED_EDGE('',*,*,#5765,.T.);
#7611=ORIENTED_EDGE('',*,*,#5766,.T.);
#7612=ORIENTED_EDGE('',*,*,#5767,.T.);
#7613=ORIENTED_EDGE('',*,*,#5768,.F.);
#7614=ORIENTED_EDGE('',*,*,#5769,.F.);
#7615=ORIENTED_EDGE('',*,*,#5770,.T.);
#7616=ORIENTED_EDGE('',*,*,#5771,.T.);
#7617=ORIENTED_EDGE('',*,*,#5772,.T.);
#7618=ORIENTED_EDGE('',*,*,#5773,.T.);
#7619=ORIENTED_EDGE('',*,*,#5774,.T.);
#7620=ORIENTED_EDGE('',*,*,#5775,.T.);
#7621=ORIENTED_EDGE('',*,*,#5776,.T.);
#7622=ORIENTED_EDGE('',*,*,#5777,.T.);
#7623=ORIENTED_EDGE('',*,*,#5778,.T.);
#7624=ORIENTED_EDGE('',*,*,#5779,.T.);
#7625=ORIENTED_EDGE('',*,*,#5780,.F.);
#7626=ORIENTED_EDGE('',*,*,#5781,.F.);
#7627=ORIENTED_EDGE('',*,*,#5747,.T.);
#7628=ORIENTED_EDGE('',*,*,#5782,.T.);
#7629=ORIENTED_EDGE('',*,*,#5783,.T.);
#7630=ORIENTED_EDGE('',*,*,#5784,.T.);
#7631=ORIENTED_EDGE('',*,*,#5785,.T.);
#7632=ORIENTED_EDGE('',*,*,#5786,.T.);
#7633=ORIENTED_EDGE('',*,*,#5787,.T.);
#7634=ORIENTED_EDGE('',*,*,#5788,.T.);
#7635=ORIENTED_EDGE('',*,*,#5789,.T.);
#7636=ORIENTED_EDGE('',*,*,#5790,.T.);
#7637=ORIENTED_EDGE('',*,*,#5791,.T.);
#7638=ORIENTED_EDGE('',*,*,#5792,.T.);
#7639=ORIENTED_EDGE('',*,*,#5793,.T.);
#7640=ORIENTED_EDGE('',*,*,#5794,.T.);
#7641=ORIENTED_EDGE('',*,*,#5795,.T.);
#7642=ORIENTED_EDGE('',*,*,#5796,.T.);
#7643=ORIENTED_EDGE('',*,*,#5456,.T.);
#7644=ORIENTED_EDGE('',*,*,#5797,.T.);
#7645=ORIENTED_EDGE('',*,*,#5798,.T.);
#7646=ORIENTED_EDGE('',*,*,#5799,.T.);
#7647=ORIENTED_EDGE('',*,*,#5800,.T.);
#7648=ORIENTED_EDGE('',*,*,#5801,.F.);
#7649=ORIENTED_EDGE('',*,*,#5623,.F.);
#7650=ORIENTED_EDGE('',*,*,#5802,.T.);
#7651=ORIENTED_EDGE('',*,*,#5803,.F.);
#7652=ORIENTED_EDGE('',*,*,#5804,.T.);
#7653=ORIENTED_EDGE('',*,*,#5805,.T.);
#7654=ORIENTED_EDGE('',*,*,#5806,.T.);
#7655=ORIENTED_EDGE('',*,*,#5465,.T.);
#7656=ORIENTED_EDGE('',*,*,#5807,.F.);
#7657=ORIENTED_EDGE('',*,*,#5808,.T.);
#7658=ORIENTED_EDGE('',*,*,#5809,.T.);
#7659=ORIENTED_EDGE('',*,*,#5810,.T.);
#7660=ORIENTED_EDGE('',*,*,#5811,.T.);
#7661=ORIENTED_EDGE('',*,*,#5812,.T.);
#7662=ORIENTED_EDGE('',*,*,#5813,.T.);
#7663=ORIENTED_EDGE('',*,*,#5814,.T.);
#7664=ORIENTED_EDGE('',*,*,#5815,.T.);
#7665=ORIENTED_EDGE('',*,*,#5816,.T.);
#7666=ORIENTED_EDGE('',*,*,#5817,.F.);
#7667=ORIENTED_EDGE('',*,*,#5818,.T.);
#7668=ORIENTED_EDGE('',*,*,#5819,.T.);
#7669=ORIENTED_EDGE('',*,*,#5820,.F.);
#7670=ORIENTED_EDGE('',*,*,#5821,.T.);
#7671=ORIENTED_EDGE('',*,*,#5822,.T.);
#7672=ORIENTED_EDGE('',*,*,#5823,.T.);
#7673=ORIENTED_EDGE('',*,*,#5824,.T.);
#7674=ORIENTED_EDGE('',*,*,#5825,.T.);
#7675=ORIENTED_EDGE('',*,*,#5826,.T.);
#7676=ORIENTED_EDGE('',*,*,#5827,.T.);
#7677=ORIENTED_EDGE('',*,*,#5828,.T.);
#7678=ORIENTED_EDGE('',*,*,#5829,.T.);
#7679=ORIENTED_EDGE('',*,*,#5830,.T.);
#7680=ORIENTED_EDGE('',*,*,#5831,.T.);
#7681=ORIENTED_EDGE('',*,*,#5832,.T.);
#7682=ORIENTED_EDGE('',*,*,#5833,.T.);
#7683=ORIENTED_EDGE('',*,*,#5834,.T.);
#7684=ORIENTED_EDGE('',*,*,#5446,.T.);
#7685=ORIENTED_EDGE('',*,*,#5835,.T.);
#7686=ORIENTED_EDGE('',*,*,#5448,.T.);
#7687=ORIENTED_EDGE('',*,*,#5836,.T.);
#7688=ORIENTED_EDGE('',*,*,#5837,.T.);
#7689=ORIENTED_EDGE('',*,*,#5838,.T.);
#7690=ORIENTED_EDGE('',*,*,#5839,.T.);
#7691=ORIENTED_EDGE('',*,*,#5840,.T.);
#7692=ORIENTED_EDGE('',*,*,#5841,.T.);
#7693=ORIENTED_EDGE('',*,*,#5842,.T.);
#7694=ORIENTED_EDGE('',*,*,#5843,.T.);
#7695=ORIENTED_EDGE('',*,*,#5844,.T.);
#7696=ORIENTED_EDGE('',*,*,#5845,.T.);
#7697=ORIENTED_EDGE('',*,*,#5846,.T.);
#7698=ORIENTED_EDGE('',*,*,#5847,.T.);
#7699=ORIENTED_EDGE('',*,*,#5848,.T.);
#7700=ORIENTED_EDGE('',*,*,#5849,.T.);
#7701=ORIENTED_EDGE('',*,*,#5850,.T.);
#7702=ORIENTED_EDGE('',*,*,#5851,.T.);
#7703=ORIENTED_EDGE('',*,*,#5852,.T.);
#7704=ORIENTED_EDGE('',*,*,#5853,.T.);
#7705=ORIENTED_EDGE('',*,*,#5435,.T.);
#7706=ORIENTED_EDGE('',*,*,#5854,.T.);
#7707=ORIENTED_EDGE('',*,*,#5855,.T.);
#7708=ORIENTED_EDGE('',*,*,#5327,.T.);
#7709=ORIENTED_EDGE('',*,*,#5856,.T.);
#7710=ORIENTED_EDGE('',*,*,#5857,.T.);
#7711=ORIENTED_EDGE('',*,*,#5858,.T.);
#7712=ORIENTED_EDGE('',*,*,#5859,.T.);
#7713=ORIENTED_EDGE('',*,*,#5860,.T.);
#7714=ORIENTED_EDGE('',*,*,#5861,.T.);
#7715=ORIENTED_EDGE('',*,*,#5862,.T.);
#7716=ORIENTED_EDGE('',*,*,#5863,.T.);
#7717=ORIENTED_EDGE('',*,*,#5330,.T.);
#7718=ORIENTED_EDGE('',*,*,#5864,.F.);
#7719=ORIENTED_EDGE('',*,*,#5865,.T.);
#7720=ORIENTED_EDGE('',*,*,#5866,.T.);
#7721=ORIENTED_EDGE('',*,*,#5867,.T.);
#7722=ORIENTED_EDGE('',*,*,#5868,.F.);
#7723=ORIENTED_EDGE('',*,*,#5869,.T.);
#7724=ORIENTED_EDGE('',*,*,#5870,.F.);
#7725=ORIENTED_EDGE('',*,*,#5871,.T.);
#7726=ORIENTED_EDGE('',*,*,#5872,.F.);
#7727=ORIENTED_EDGE('',*,*,#5873,.T.);
#7728=ORIENTED_EDGE('',*,*,#5874,.F.);
#7729=ORIENTED_EDGE('',*,*,#5875,.T.);
#7730=ORIENTED_EDGE('',*,*,#5876,.F.);
#7731=ORIENTED_EDGE('',*,*,#5877,.T.);
#7732=ORIENTED_EDGE('',*,*,#5878,.T.);
#7733=ORIENTED_EDGE('',*,*,#5879,.T.);
#7734=ORIENTED_EDGE('',*,*,#5878,.F.);
#7735=ORIENTED_EDGE('',*,*,#5880,.T.);
#7736=ORIENTED_EDGE('',*,*,#5868,.T.);
#7737=ORIENTED_EDGE('',*,*,#5881,.T.);
#7738=ORIENTED_EDGE('',*,*,#5882,.T.);
#7739=ORIENTED_EDGE('',*,*,#5883,.T.);
#7740=ORIENTED_EDGE('',*,*,#5884,.F.);
#7741=ORIENTED_EDGE('',*,*,#5885,.T.);
#7742=ORIENTED_EDGE('',*,*,#5886,.F.);
#7743=ORIENTED_EDGE('',*,*,#5887,.T.);
#7744=ORIENTED_EDGE('',*,*,#5888,.F.);
#7745=ORIENTED_EDGE('',*,*,#5889,.T.);
#7746=ORIENTED_EDGE('',*,*,#5890,.F.);
#7747=ORIENTED_EDGE('',*,*,#5891,.T.);
#7748=ORIENTED_EDGE('',*,*,#5892,.F.);
#7749=ORIENTED_EDGE('',*,*,#5893,.T.);
#7750=ORIENTED_EDGE('',*,*,#5894,.T.);
#7751=ORIENTED_EDGE('',*,*,#5895,.T.);
#7752=ORIENTED_EDGE('',*,*,#5896,.F.);
#7753=ORIENTED_EDGE('',*,*,#5897,.T.);
#7754=ORIENTED_EDGE('',*,*,#5898,.T.);
#7755=ORIENTED_EDGE('',*,*,#5899,.F.);
#7756=ORIENTED_EDGE('',*,*,#5900,.F.);
#7757=ORIENTED_EDGE('',*,*,#5901,.F.);
#7758=ORIENTED_EDGE('',*,*,#5902,.T.);
#7759=ORIENTED_EDGE('',*,*,#5903,.T.);
#7760=ORIENTED_EDGE('',*,*,#5904,.F.);
#7761=ORIENTED_EDGE('',*,*,#5905,.T.);
#7762=ORIENTED_EDGE('',*,*,#5906,.F.);
#7763=ORIENTED_EDGE('',*,*,#5907,.T.);
#7764=ORIENTED_EDGE('',*,*,#5908,.F.);
#7765=ORIENTED_EDGE('',*,*,#5909,.T.);
#7766=ORIENTED_EDGE('',*,*,#5910,.T.);
#7767=ORIENTED_EDGE('',*,*,#5911,.T.);
#7768=ORIENTED_EDGE('',*,*,#5912,.T.);
#7769=ORIENTED_EDGE('',*,*,#5913,.T.);
#7770=ORIENTED_EDGE('',*,*,#5743,.T.);
#7771=ORIENTED_EDGE('',*,*,#5914,.T.);
#7772=ORIENTED_EDGE('',*,*,#5915,.T.);
#7773=ORIENTED_EDGE('',*,*,#5916,.F.);
#7774=ORIENTED_EDGE('',*,*,#5917,.T.);
#7775=ORIENTED_EDGE('',*,*,#5918,.T.);
#7776=ORIENTED_EDGE('',*,*,#5919,.T.);
#7777=ORIENTED_EDGE('',*,*,#5730,.T.);
#7778=ORIENTED_EDGE('',*,*,#5920,.T.);
#7779=ORIENTED_EDGE('',*,*,#5921,.T.);
#7780=ORIENTED_EDGE('',*,*,#5922,.T.);
#7781=ORIENTED_EDGE('',*,*,#5923,.T.);
#7782=ORIENTED_EDGE('',*,*,#5924,.T.);
#7783=ORIENTED_EDGE('',*,*,#5925,.T.);
#7784=ORIENTED_EDGE('',*,*,#5926,.T.);
#7785=ORIENTED_EDGE('',*,*,#5307,.T.);
#7786=ORIENTED_EDGE('',*,*,#5407,.T.);
#7787=ORIENTED_EDGE('',*,*,#5927,.T.);
#7788=ORIENTED_EDGE('',*,*,#5928,.T.);
#7789=ORIENTED_EDGE('',*,*,#5929,.T.);
#7790=ORIENTED_EDGE('',*,*,#5930,.T.);
#7791=ORIENTED_EDGE('',*,*,#5931,.T.);
#7792=ORIENTED_EDGE('',*,*,#5932,.T.);
#7793=ORIENTED_EDGE('',*,*,#5933,.F.);
#7794=ORIENTED_EDGE('',*,*,#5934,.T.);
#7795=ORIENTED_EDGE('',*,*,#5935,.F.);
#7796=ORIENTED_EDGE('',*,*,#5936,.T.);
#7797=ORIENTED_EDGE('',*,*,#5937,.F.);
#7798=ORIENTED_EDGE('',*,*,#5385,.T.);
#7799=ORIENTED_EDGE('',*,*,#5354,.T.);
#7800=ORIENTED_EDGE('',*,*,#5938,.T.);
#7801=ORIENTED_EDGE('',*,*,#5939,.T.);
#7802=ORIENTED_EDGE('',*,*,#5940,.T.);
#7803=ORIENTED_EDGE('',*,*,#5941,.T.);
#7804=ORIENTED_EDGE('',*,*,#5476,.T.);
#7805=ORIENTED_EDGE('',*,*,#5942,.T.);
#7806=ORIENTED_EDGE('',*,*,#5943,.F.);
#7807=ORIENTED_EDGE('',*,*,#5944,.T.);
#7808=ORIENTED_EDGE('',*,*,#5945,.F.);
#7809=ORIENTED_EDGE('',*,*,#5946,.T.);
#7810=ORIENTED_EDGE('',*,*,#5947,.F.);
#7811=ORIENTED_EDGE('',*,*,#5948,.T.);
#7812=ORIENTED_EDGE('',*,*,#5949,.T.);
#7813=ORIENTED_EDGE('',*,*,#5950,.T.);
#7814=ORIENTED_EDGE('',*,*,#5951,.F.);
#7815=ORIENTED_EDGE('',*,*,#5952,.T.);
#7816=ORIENTED_EDGE('',*,*,#5953,.F.);
#7817=ORIENTED_EDGE('',*,*,#5954,.T.);
#7818=ORIENTED_EDGE('',*,*,#5955,.F.);
#7819=ORIENTED_EDGE('',*,*,#5956,.T.);
#7820=ORIENTED_EDGE('',*,*,#5957,.T.);
#7821=ORIENTED_EDGE('',*,*,#5958,.T.);
#7822=ORIENTED_EDGE('',*,*,#5323,.T.);
#7823=ORIENTED_EDGE('',*,*,#5888,.T.);
#7824=ORIENTED_EDGE('',*,*,#5959,.T.);
#7825=ORIENTED_EDGE('',*,*,#5894,.F.);
#7826=ORIENTED_EDGE('',*,*,#5960,.T.);
#7827=ORIENTED_EDGE('',*,*,#5961,.T.);
#7828=ORIENTED_EDGE('',*,*,#5962,.T.);
#7829=ORIENTED_EDGE('',*,*,#5963,.T.);
#7830=ORIENTED_EDGE('',*,*,#5964,.T.);
#7831=ORIENTED_EDGE('',*,*,#5965,.F.);
#7832=ORIENTED_EDGE('',*,*,#5966,.T.);
#7833=ORIENTED_EDGE('',*,*,#5967,.T.);
#7834=ORIENTED_EDGE('',*,*,#5968,.T.);
#7835=ORIENTED_EDGE('',*,*,#5969,.F.);
#7836=ORIENTED_EDGE('',*,*,#5970,.F.);
#7837=ORIENTED_EDGE('',*,*,#5971,.T.);
#7838=ORIENTED_EDGE('',*,*,#5972,.T.);
#7839=ORIENTED_EDGE('',*,*,#5973,.T.);
#7840=ORIENTED_EDGE('',*,*,#5974,.F.);
#7841=ORIENTED_EDGE('',*,*,#5975,.T.);
#7842=ORIENTED_EDGE('',*,*,#5976,.T.);
#7843=ORIENTED_EDGE('',*,*,#5619,.T.);
#7844=ORIENTED_EDGE('',*,*,#5977,.T.);
#7845=ORIENTED_EDGE('',*,*,#5978,.T.);
#7846=ORIENTED_EDGE('',*,*,#5444,.T.);
#7847=ORIENTED_EDGE('',*,*,#5620,.T.);
#7848=ORIENTED_EDGE('',*,*,#5979,.T.);
#7849=ORIENTED_EDGE('',*,*,#5980,.T.);
#7850=ORIENTED_EDGE('',*,*,#5981,.T.);
#7851=ORIENTED_EDGE('',*,*,#5982,.T.);
#7852=ORIENTED_EDGE('',*,*,#5983,.T.);
#7853=ORIENTED_EDGE('',*,*,#5984,.T.);
#7854=ORIENTED_EDGE('',*,*,#5985,.T.);
#7855=ORIENTED_EDGE('',*,*,#5986,.F.);
#7856=ORIENTED_EDGE('',*,*,#5987,.T.);
#7857=ORIENTED_EDGE('',*,*,#5988,.T.);
#7858=ORIENTED_EDGE('',*,*,#5989,.T.);
#7859=ORIENTED_EDGE('',*,*,#5990,.T.);
#7860=ORIENTED_EDGE('',*,*,#5991,.T.);
#7861=ORIENTED_EDGE('',*,*,#5992,.T.);
#7862=ORIENTED_EDGE('',*,*,#5993,.T.);
#7863=ORIENTED_EDGE('',*,*,#5994,.T.);
#7864=ORIENTED_EDGE('',*,*,#5995,.T.);
#7865=ORIENTED_EDGE('',*,*,#5996,.T.);
#7866=ORIENTED_EDGE('',*,*,#5997,.T.);
#7867=ORIENTED_EDGE('',*,*,#5998,.T.);
#7868=ORIENTED_EDGE('',*,*,#5999,.T.);
#7869=ORIENTED_EDGE('',*,*,#6000,.T.);
#7870=ORIENTED_EDGE('',*,*,#6001,.T.);
#7871=ORIENTED_EDGE('',*,*,#5537,.T.);
#7872=ORIENTED_EDGE('',*,*,#6002,.T.);
#7873=ORIENTED_EDGE('',*,*,#6003,.T.);
#7874=ORIENTED_EDGE('',*,*,#6004,.T.);
#7875=ORIENTED_EDGE('',*,*,#6005,.T.);
#7876=ORIENTED_EDGE('',*,*,#6006,.T.);
#7877=ORIENTED_EDGE('',*,*,#5536,.T.);
#7878=ORIENTED_EDGE('',*,*,#6007,.T.);
#7879=ORIENTED_EDGE('',*,*,#6008,.T.);
#7880=ORIENTED_EDGE('',*,*,#6009,.T.);
#7881=ORIENTED_EDGE('',*,*,#6010,.T.);
#7882=ORIENTED_EDGE('',*,*,#6011,.T.);
#7883=ORIENTED_EDGE('',*,*,#5340,.T.);
#7884=ORIENTED_EDGE('',*,*,#6012,.T.);
#7885=ORIENTED_EDGE('',*,*,#6013,.T.);
#7886=ORIENTED_EDGE('',*,*,#5334,.T.);
#7887=ORIENTED_EDGE('',*,*,#6014,.T.);
#7888=ORIENTED_EDGE('',*,*,#6015,.T.);
#7889=ORIENTED_EDGE('',*,*,#6016,.T.);
#7890=ORIENTED_EDGE('',*,*,#6017,.T.);
#7891=ORIENTED_EDGE('',*,*,#6008,.F.);
#7892=ORIENTED_EDGE('',*,*,#6018,.T.);
#7893=ORIENTED_EDGE('',*,*,#6003,.F.);
#7894=ORIENTED_EDGE('',*,*,#6019,.T.);
#7895=ORIENTED_EDGE('',*,*,#6005,.F.);
#7896=ORIENTED_EDGE('',*,*,#6020,.T.);
#7897=ORIENTED_EDGE('',*,*,#5539,.F.);
#7898=ORIENTED_EDGE('',*,*,#6021,.T.);
#7899=ORIENTED_EDGE('',*,*,#5538,.F.);
#7900=ORIENTED_EDGE('',*,*,#6022,.T.);
#7901=ORIENTED_EDGE('',*,*,#6010,.F.);
#7902=ORIENTED_EDGE('',*,*,#6023,.T.);
#7903=ORIENTED_EDGE('',*,*,#6024,.T.);
#7904=ORIENTED_EDGE('',*,*,#6025,.T.);
#7905=ORIENTED_EDGE('',*,*,#6026,.T.);
#7906=ORIENTED_EDGE('',*,*,#6027,.T.);
#7907=ORIENTED_EDGE('',*,*,#6028,.T.);
#7908=ORIENTED_EDGE('',*,*,#6029,.T.);
#7909=ORIENTED_EDGE('',*,*,#6030,.T.);
#7910=ORIENTED_EDGE('',*,*,#6031,.T.);
#7911=ORIENTED_EDGE('',*,*,#6032,.T.);
#7912=ORIENTED_EDGE('',*,*,#6033,.T.);
#7913=ORIENTED_EDGE('',*,*,#6034,.F.);
#7914=ORIENTED_EDGE('',*,*,#6035,.T.);
#7915=ORIENTED_EDGE('',*,*,#6036,.T.);
#7916=ORIENTED_EDGE('',*,*,#6037,.T.);
#7917=ORIENTED_EDGE('',*,*,#5471,.T.);
#7918=ORIENTED_EDGE('',*,*,#6038,.T.);
#7919=ORIENTED_EDGE('',*,*,#6039,.T.);
#7920=ORIENTED_EDGE('',*,*,#6040,.T.);
#7921=ORIENTED_EDGE('',*,*,#6041,.T.);
#7922=ORIENTED_EDGE('',*,*,#6042,.T.);
#7923=ORIENTED_EDGE('',*,*,#6043,.F.);
#7924=ORIENTED_EDGE('',*,*,#6044,.T.);
#7925=ORIENTED_EDGE('',*,*,#6045,.T.);
#7926=ORIENTED_EDGE('',*,*,#6046,.F.);
#7927=ORIENTED_EDGE('',*,*,#6047,.T.);
#7928=ORIENTED_EDGE('',*,*,#6048,.T.);
#7929=ORIENTED_EDGE('',*,*,#6049,.T.);
#7930=ORIENTED_EDGE('',*,*,#6050,.T.);
#7931=ORIENTED_EDGE('',*,*,#6051,.T.);
#7932=ORIENTED_EDGE('',*,*,#6052,.T.);
#7933=ORIENTED_EDGE('',*,*,#6053,.T.);
#7934=ORIENTED_EDGE('',*,*,#6054,.T.);
#7935=ORIENTED_EDGE('',*,*,#6055,.T.);
#7936=ORIENTED_EDGE('',*,*,#6056,.T.);
#7937=ORIENTED_EDGE('',*,*,#6057,.T.);
#7938=ORIENTED_EDGE('',*,*,#6058,.T.);
#7939=ORIENTED_EDGE('',*,*,#6059,.T.);
#7940=ORIENTED_EDGE('',*,*,#6060,.T.);
#7941=ORIENTED_EDGE('',*,*,#6061,.T.);
#7942=ORIENTED_EDGE('',*,*,#6062,.T.);
#7943=ORIENTED_EDGE('',*,*,#6063,.T.);
#7944=ORIENTED_EDGE('',*,*,#6064,.T.);
#7945=ORIENTED_EDGE('',*,*,#6065,.T.);
#7946=ORIENTED_EDGE('',*,*,#5439,.T.);
#7947=ORIENTED_EDGE('',*,*,#6066,.T.);
#7948=ORIENTED_EDGE('',*,*,#6067,.T.);
#7949=ORIENTED_EDGE('',*,*,#5358,.T.);
#7950=ORIENTED_EDGE('',*,*,#6068,.T.);
#7951=ORIENTED_EDGE('',*,*,#6069,.T.);
#7952=ORIENTED_EDGE('',*,*,#6070,.T.);
#7953=ORIENTED_EDGE('',*,*,#6071,.T.);
#7954=ORIENTED_EDGE('',*,*,#6072,.T.);
#7955=ORIENTED_EDGE('',*,*,#6073,.T.);
#7956=ORIENTED_EDGE('',*,*,#6074,.T.);
#7957=ORIENTED_EDGE('',*,*,#6075,.T.);
#7958=ORIENTED_EDGE('',*,*,#5362,.T.);
#7959=ORIENTED_EDGE('',*,*,#6076,.T.);
#7960=ORIENTED_EDGE('',*,*,#6077,.T.);
#7961=ORIENTED_EDGE('',*,*,#6078,.T.);
#7962=ORIENTED_EDGE('',*,*,#6079,.F.);
#7963=ORIENTED_EDGE('',*,*,#6080,.T.);
#7964=ORIENTED_EDGE('',*,*,#6081,.F.);
#7965=ORIENTED_EDGE('',*,*,#6082,.T.);
#7966=ORIENTED_EDGE('',*,*,#6083,.F.);
#7967=ORIENTED_EDGE('',*,*,#5866,.F.);
#7968=ORIENTED_EDGE('',*,*,#6084,.T.);
#7969=ORIENTED_EDGE('',*,*,#6079,.T.);
#7970=ORIENTED_EDGE('',*,*,#6085,.T.);
#7971=ORIENTED_EDGE('',*,*,#6086,.T.);
#7972=ORIENTED_EDGE('',*,*,#6087,.T.);
#7973=ORIENTED_EDGE('',*,*,#6088,.T.);
#7974=ORIENTED_EDGE('',*,*,#6089,.F.);
#7975=ORIENTED_EDGE('',*,*,#6090,.T.);
#7976=ORIENTED_EDGE('',*,*,#6091,.F.);
#7977=ORIENTED_EDGE('',*,*,#6092,.T.);
#7978=ORIENTED_EDGE('',*,*,#6093,.F.);
#7979=ORIENTED_EDGE('',*,*,#6093,.T.);
#7980=ORIENTED_EDGE('',*,*,#6094,.T.);
#7981=ORIENTED_EDGE('',*,*,#5882,.F.);
#7982=ORIENTED_EDGE('',*,*,#6095,.T.);
#7983=ORIENTED_EDGE('',*,*,#6096,.T.);
#7984=ORIENTED_EDGE('',*,*,#6097,.T.);
#7985=ORIENTED_EDGE('',*,*,#6098,.T.);
#7986=ORIENTED_EDGE('',*,*,#6099,.T.);
#7987=ORIENTED_EDGE('',*,*,#6100,.F.);
#7988=ORIENTED_EDGE('',*,*,#6101,.T.);
#7989=ORIENTED_EDGE('',*,*,#6102,.T.);
#7990=ORIENTED_EDGE('',*,*,#6103,.T.);
#7991=ORIENTED_EDGE('',*,*,#6104,.F.);
#7992=ORIENTED_EDGE('',*,*,#6105,.T.);
#7993=ORIENTED_EDGE('',*,*,#6106,.T.);
#7994=ORIENTED_EDGE('',*,*,#5534,.T.);
#7995=ORIENTED_EDGE('',*,*,#6107,.T.);
#7996=ORIENTED_EDGE('',*,*,#6108,.T.);
#7997=ORIENTED_EDGE('',*,*,#6109,.T.);
#7998=ORIENTED_EDGE('',*,*,#5535,.T.);
#7999=ORIENTED_EDGE('',*,*,#6110,.T.);
#8000=ORIENTED_EDGE('',*,*,#6111,.T.);
#8001=ORIENTED_EDGE('',*,*,#5450,.T.);
#8002=ORIENTED_EDGE('',*,*,#6112,.T.);
#8003=ORIENTED_EDGE('',*,*,#6113,.T.);
#8004=ORIENTED_EDGE('',*,*,#6114,.T.);
#8005=ORIENTED_EDGE('',*,*,#6115,.T.);
#8006=ORIENTED_EDGE('',*,*,#5813,.F.);
#8007=ORIENTED_EDGE('',*,*,#6116,.T.);
#8008=ORIENTED_EDGE('',*,*,#6117,.T.);
#8009=ORIENTED_EDGE('',*,*,#6118,.T.);
#8010=ORIENTED_EDGE('',*,*,#6119,.T.);
#8011=ORIENTED_EDGE('',*,*,#6120,.T.);
#8012=ORIENTED_EDGE('',*,*,#6121,.T.);
#8013=ORIENTED_EDGE('',*,*,#6122,.T.);
#8014=ORIENTED_EDGE('',*,*,#6123,.T.);
#8015=ORIENTED_EDGE('',*,*,#6124,.T.);
#8016=ORIENTED_EDGE('',*,*,#6125,.T.);
#8017=ORIENTED_EDGE('',*,*,#6126,.T.);
#8018=ORIENTED_EDGE('',*,*,#6127,.T.);
#8019=ORIENTED_EDGE('',*,*,#6128,.T.);
#8020=ORIENTED_EDGE('',*,*,#6129,.T.);
#8021=ORIENTED_EDGE('',*,*,#6130,.T.);
#8022=ORIENTED_EDGE('',*,*,#5521,.T.);
#8023=ORIENTED_EDGE('',*,*,#6131,.T.);
#8024=ORIENTED_EDGE('',*,*,#6132,.T.);
#8025=ORIENTED_EDGE('',*,*,#6133,.T.);
#8026=ORIENTED_EDGE('',*,*,#6134,.T.);
#8027=ORIENTED_EDGE('',*,*,#6135,.T.);
#8028=ORIENTED_EDGE('',*,*,#5519,.T.);
#8029=ORIENTED_EDGE('',*,*,#6136,.T.);
#8030=ORIENTED_EDGE('',*,*,#6137,.T.);
#8031=ORIENTED_EDGE('',*,*,#6138,.T.);
#8032=ORIENTED_EDGE('',*,*,#6139,.T.);
#8033=ORIENTED_EDGE('',*,*,#6140,.T.);
#8034=ORIENTED_EDGE('',*,*,#5372,.T.);
#8035=ORIENTED_EDGE('',*,*,#6141,.T.);
#8036=ORIENTED_EDGE('',*,*,#6142,.T.);
#8037=ORIENTED_EDGE('',*,*,#6143,.T.);
#8038=ORIENTED_EDGE('',*,*,#6144,.T.);
#8039=ORIENTED_EDGE('',*,*,#5366,.T.);
#8040=ORIENTED_EDGE('',*,*,#6145,.T.);
#8041=ORIENTED_EDGE('',*,*,#6146,.T.);
#8042=ORIENTED_EDGE('',*,*,#6137,.F.);
#8043=ORIENTED_EDGE('',*,*,#5368,.T.);
#8044=ORIENTED_EDGE('',*,*,#6132,.F.);
#8045=ORIENTED_EDGE('',*,*,#5376,.T.);
#8046=ORIENTED_EDGE('',*,*,#6134,.F.);
#8047=ORIENTED_EDGE('',*,*,#6147,.T.);
#8048=ORIENTED_EDGE('',*,*,#5523,.F.);
#8049=ORIENTED_EDGE('',*,*,#6148,.T.);
#8050=ORIENTED_EDGE('',*,*,#5522,.F.);
#8051=ORIENTED_EDGE('',*,*,#6149,.T.);
#8052=ORIENTED_EDGE('',*,*,#6139,.F.);
#8053=ORIENTED_EDGE('',*,*,#6150,.T.);
#8054=ORIENTED_EDGE('',*,*,#6151,.T.);
#8055=ORIENTED_EDGE('',*,*,#6152,.T.);
#8056=ORIENTED_EDGE('',*,*,#6153,.T.);
#8057=ORIENTED_EDGE('',*,*,#6154,.T.);
#8058=ORIENTED_EDGE('',*,*,#6155,.T.);
#8059=ORIENTED_EDGE('',*,*,#6156,.T.);
#8060=ORIENTED_EDGE('',*,*,#6157,.T.);
#8061=ORIENTED_EDGE('',*,*,#6158,.T.);
#8062=ORIENTED_EDGE('',*,*,#6159,.T.);
#8063=ORIENTED_EDGE('',*,*,#6160,.T.);
#8064=ORIENTED_EDGE('',*,*,#6161,.T.);
#8065=ORIENTED_EDGE('',*,*,#6162,.F.);
#8066=ORIENTED_EDGE('',*,*,#6163,.T.);
#8067=ORIENTED_EDGE('',*,*,#6164,.T.);
#8068=ORIENTED_EDGE('',*,*,#6165,.T.);
#8069=ORIENTED_EDGE('',*,*,#6166,.T.);
#8070=ORIENTED_EDGE('',*,*,#6167,.T.);
#8071=ORIENTED_EDGE('',*,*,#6168,.T.);
#8072=ORIENTED_EDGE('',*,*,#6169,.T.);
#8073=ORIENTED_EDGE('',*,*,#6170,.T.);
#8074=ORIENTED_EDGE('',*,*,#6171,.F.);
#8075=ORIENTED_EDGE('',*,*,#6172,.T.);
#8076=ORIENTED_EDGE('',*,*,#6173,.T.);
#8077=ORIENTED_EDGE('',*,*,#6174,.F.);
#8078=ORIENTED_EDGE('',*,*,#6175,.T.);
#8079=ORIENTED_EDGE('',*,*,#6176,.T.);
#8080=ORIENTED_EDGE('',*,*,#6177,.T.);
#8081=ORIENTED_EDGE('',*,*,#6178,.T.);
#8082=ORIENTED_EDGE('',*,*,#6179,.T.);
#8083=ORIENTED_EDGE('',*,*,#5425,.T.);
#8084=ORIENTED_EDGE('',*,*,#6180,.T.);
#8085=ORIENTED_EDGE('',*,*,#5419,.T.);
#8086=ORIENTED_EDGE('',*,*,#6181,.T.);
#8087=ORIENTED_EDGE('',*,*,#5423,.T.);
#8088=ORIENTED_EDGE('',*,*,#6182,.T.);
#8089=ORIENTED_EDGE('',*,*,#6183,.T.);
#8090=ORIENTED_EDGE('',*,*,#6184,.T.);
#8091=ORIENTED_EDGE('',*,*,#6185,.T.);
#8092=ORIENTED_EDGE('',*,*,#6186,.F.);
#8093=ORIENTED_EDGE('',*,*,#6187,.T.);
#8094=ORIENTED_EDGE('',*,*,#6188,.T.);
#8095=ORIENTED_EDGE('',*,*,#6189,.T.);
#8096=ORIENTED_EDGE('',*,*,#6190,.F.);
#8097=ORIENTED_EDGE('',*,*,#6191,.T.);
#8098=ORIENTED_EDGE('',*,*,#6192,.F.);
#8099=ORIENTED_EDGE('',*,*,#6193,.T.);
#8100=ORIENTED_EDGE('',*,*,#5683,.F.);
#8101=ORIENTED_EDGE('',*,*,#6194,.T.);
#8102=ORIENTED_EDGE('',*,*,#6190,.T.);
#8103=ORIENTED_EDGE('',*,*,#6195,.T.);
#8104=ORIENTED_EDGE('',*,*,#6196,.T.);
#8105=ORIENTED_EDGE('',*,*,#6197,.T.);
#8106=ORIENTED_EDGE('',*,*,#6198,.F.);
#8107=ORIENTED_EDGE('',*,*,#6199,.T.);
#8108=ORIENTED_EDGE('',*,*,#6200,.F.);
#8109=ORIENTED_EDGE('',*,*,#6201,.T.);
#8110=ORIENTED_EDGE('',*,*,#6202,.F.);
#8111=ORIENTED_EDGE('',*,*,#6203,.T.);
#8112=ORIENTED_EDGE('',*,*,#6202,.T.);
#8113=ORIENTED_EDGE('',*,*,#6204,.T.);
#8114=ORIENTED_EDGE('',*,*,#5687,.F.);
#8115=ORIENTED_EDGE('',*,*,#6205,.T.);
#8116=ORIENTED_EDGE('',*,*,#6206,.T.);
#8117=ORIENTED_EDGE('',*,*,#6207,.T.);
#8118=ORIENTED_EDGE('',*,*,#6208,.T.);
#8119=ORIENTED_EDGE('',*,*,#6209,.T.);
#8120=ORIENTED_EDGE('',*,*,#6210,.F.);
#8121=ORIENTED_EDGE('',*,*,#6211,.T.);
#8122=ORIENTED_EDGE('',*,*,#6212,.T.);
#8123=ORIENTED_EDGE('',*,*,#6213,.T.);
#8124=ORIENTED_EDGE('',*,*,#6214,.F.);
#8125=ORIENTED_EDGE('',*,*,#6215,.T.);
#8126=ORIENTED_EDGE('',*,*,#6216,.T.);
#8127=ORIENTED_EDGE('',*,*,#5515,.T.);
#8128=ORIENTED_EDGE('',*,*,#6217,.T.);
#8129=ORIENTED_EDGE('',*,*,#6218,.T.);
#8130=ORIENTED_EDGE('',*,*,#6219,.T.);
#8131=ORIENTED_EDGE('',*,*,#5517,.T.);
#8132=ORIENTED_EDGE('',*,*,#6220,.T.);
#8133=ORIENTED_EDGE('',*,*,#6221,.T.);
#8134=ORIENTED_EDGE('',*,*,#6222,.T.);
#8135=ORIENTED_EDGE('',*,*,#6223,.T.);
#8136=ORIENTED_EDGE('',*,*,#6224,.T.);
#8137=ORIENTED_EDGE('',*,*,#6225,.T.);
#8138=ORIENTED_EDGE('',*,*,#6226,.T.);
#8139=ORIENTED_EDGE('',*,*,#6039,.F.);
#8140=ORIENTED_EDGE('',*,*,#6227,.T.);
#8141=ORIENTED_EDGE('',*,*,#6228,.T.);
#8142=ORIENTED_EDGE('',*,*,#6229,.T.);
#8143=ORIENTED_EDGE('',*,*,#6230,.T.);
#8144=ORIENTED_EDGE('',*,*,#6231,.T.);
#8145=ORIENTED_EDGE('',*,*,#6232,.T.);
#8146=ORIENTED_EDGE('',*,*,#6233,.T.);
#8147=ORIENTED_EDGE('',*,*,#6234,.T.);
#8148=ORIENTED_EDGE('',*,*,#6235,.T.);
#8149=ORIENTED_EDGE('',*,*,#6236,.T.);
#8150=ORIENTED_EDGE('',*,*,#6237,.T.);
#8151=ORIENTED_EDGE('',*,*,#6238,.T.);
#8152=ORIENTED_EDGE('',*,*,#5467,.T.);
#8153=ORIENTED_EDGE('',*,*,#6239,.T.);
#8154=ORIENTED_EDGE('',*,*,#6240,.T.);
#8155=ORIENTED_EDGE('',*,*,#5502,.T.);
#8156=ORIENTED_EDGE('',*,*,#6241,.T.);
#8157=ORIENTED_EDGE('',*,*,#6242,.T.);
#8158=ORIENTED_EDGE('',*,*,#6243,.T.);
#8159=ORIENTED_EDGE('',*,*,#6244,.T.);
#8160=ORIENTED_EDGE('',*,*,#6245,.T.);
#8161=ORIENTED_EDGE('',*,*,#6246,.T.);
#8162=ORIENTED_EDGE('',*,*,#5500,.T.);
#8163=ORIENTED_EDGE('',*,*,#6247,.T.);
#8164=ORIENTED_EDGE('',*,*,#6248,.T.);
#8165=ORIENTED_EDGE('',*,*,#6249,.T.);
#8166=ORIENTED_EDGE('',*,*,#6250,.T.);
#8167=ORIENTED_EDGE('',*,*,#6251,.F.);
#8168=ORIENTED_EDGE('',*,*,#6252,.T.);
#8169=ORIENTED_EDGE('',*,*,#6253,.T.);
#8170=ORIENTED_EDGE('',*,*,#6254,.T.);
#8171=ORIENTED_EDGE('',*,*,#6255,.T.);
#8172=ORIENTED_EDGE('',*,*,#6256,.T.);
#8173=ORIENTED_EDGE('',*,*,#6257,.T.);
#8174=ORIENTED_EDGE('',*,*,#6258,.T.);
#8175=ORIENTED_EDGE('',*,*,#5395,.T.);
#8176=ORIENTED_EDGE('',*,*,#5737,.T.);
#8177=ORIENTED_EDGE('',*,*,#6259,.T.);
#8178=ORIENTED_EDGE('',*,*,#6260,.F.);
#8179=ORIENTED_EDGE('',*,*,#6247,.F.);
#8180=ORIENTED_EDGE('',*,*,#6261,.T.);
#8181=ORIENTED_EDGE('',*,*,#6242,.F.);
#8182=ORIENTED_EDGE('',*,*,#6262,.T.);
#8183=ORIENTED_EDGE('',*,*,#5724,.F.);
#8184=ORIENTED_EDGE('',*,*,#5397,.T.);
#8185=ORIENTED_EDGE('',*,*,#5506,.F.);
#8186=ORIENTED_EDGE('',*,*,#5401,.T.);
#8187=ORIENTED_EDGE('',*,*,#5504,.F.);
#8188=ORIENTED_EDGE('',*,*,#6263,.T.);
#8189=ORIENTED_EDGE('',*,*,#6249,.F.);
#8190=ORIENTED_EDGE('',*,*,#6264,.T.);
#8191=ORIENTED_EDGE('',*,*,#6265,.T.);
#8192=ORIENTED_EDGE('',*,*,#6266,.T.);
#8193=ORIENTED_EDGE('',*,*,#6267,.T.);
#8194=ORIENTED_EDGE('',*,*,#6268,.T.);
#8195=ORIENTED_EDGE('',*,*,#6269,.T.);
#8196=ORIENTED_EDGE('',*,*,#6270,.T.);
#8197=ORIENTED_EDGE('',*,*,#6271,.T.);
#8198=ORIENTED_EDGE('',*,*,#5452,.T.);
#8199=ORIENTED_EDGE('',*,*,#6272,.T.);
#8200=ORIENTED_EDGE('',*,*,#6273,.T.);
#8201=ORIENTED_EDGE('',*,*,#6274,.F.);
#8202=ORIENTED_EDGE('',*,*,#6275,.T.);
#8203=ORIENTED_EDGE('',*,*,#6276,.T.);
#8204=ORIENTED_EDGE('',*,*,#6277,.T.);
#8205=ORIENTED_EDGE('',*,*,#6278,.T.);
#8206=ORIENTED_EDGE('',*,*,#6279,.T.);
#8207=ORIENTED_EDGE('',*,*,#5986,.T.);
#8208=ORIENTED_EDGE('',*,*,#6280,.T.);
#8209=ORIENTED_EDGE('',*,*,#6281,.T.);
#8210=ORIENTED_EDGE('',*,*,#6282,.T.);
#8211=ORIENTED_EDGE('',*,*,#6283,.F.);
#8212=ORIENTED_EDGE('',*,*,#6284,.T.);
#8213=ORIENTED_EDGE('',*,*,#6285,.T.);
#8214=ORIENTED_EDGE('',*,*,#6286,.F.);
#8215=ORIENTED_EDGE('',*,*,#6287,.T.);
#8216=ORIENTED_EDGE('',*,*,#6288,.T.);
#8217=ORIENTED_EDGE('',*,*,#6289,.T.);
#8218=ORIENTED_EDGE('',*,*,#6290,.T.);
#8219=ORIENTED_EDGE('',*,*,#6291,.T.);
#8220=ORIENTED_EDGE('',*,*,#6292,.T.);
#8221=ORIENTED_EDGE('',*,*,#6293,.T.);
#8222=ORIENTED_EDGE('',*,*,#6294,.T.);
#8223=ORIENTED_EDGE('',*,*,#6295,.T.);
#8224=ORIENTED_EDGE('',*,*,#6296,.T.);
#8225=ORIENTED_EDGE('',*,*,#6297,.T.);
#8226=ORIENTED_EDGE('',*,*,#6298,.T.);
#8227=ORIENTED_EDGE('',*,*,#5411,.T.);
#8228=ORIENTED_EDGE('',*,*,#6299,.T.);
#8229=ORIENTED_EDGE('',*,*,#6300,.T.);
#8230=ORIENTED_EDGE('',*,*,#6301,.T.);
#8231=ORIENTED_EDGE('',*,*,#6302,.T.);
#8232=ORIENTED_EDGE('',*,*,#6303,.T.);
#8233=ORIENTED_EDGE('',*,*,#5427,.T.);
#8234=ORIENTED_EDGE('',*,*,#6304,.T.);
#8235=ORIENTED_EDGE('',*,*,#6305,.T.);
#8236=ORIENTED_EDGE('',*,*,#5415,.T.);
#8237=ORIENTED_EDGE('',*,*,#6188,.F.);
#8238=ORIENTED_EDGE('',*,*,#6306,.T.);
#8239=ORIENTED_EDGE('',*,*,#5872,.T.);
#8240=ORIENTED_EDGE('',*,*,#6307,.T.);
#8241=ORIENTED_EDGE('',*,*,#5892,.T.);
#8242=ORIENTED_EDGE('',*,*,#6308,.T.);
#8243=ORIENTED_EDGE('',*,*,#6196,.F.);
#8244=ORIENTED_EDGE('',*,*,#6309,.T.);
#8245=ORIENTED_EDGE('',*,*,#6310,.T.);
#8246=ORIENTED_EDGE('',*,*,#6311,.T.);
#8247=ORIENTED_EDGE('',*,*,#6312,.T.);
#8248=ORIENTED_EDGE('',*,*,#6313,.T.);
#8249=ORIENTED_EDGE('',*,*,#6314,.T.);
#8250=ORIENTED_EDGE('',*,*,#6315,.T.);
#8251=ORIENTED_EDGE('',*,*,#5496,.T.);
#8252=ORIENTED_EDGE('',*,*,#6316,.T.);
#8253=ORIENTED_EDGE('',*,*,#6317,.T.);
#8254=ORIENTED_EDGE('',*,*,#6318,.T.);
#8255=ORIENTED_EDGE('',*,*,#5498,.T.);
#8256=ORIENTED_EDGE('',*,*,#6319,.T.);
#8257=ORIENTED_EDGE('',*,*,#6320,.T.);
#8258=ORIENTED_EDGE('',*,*,#6321,.T.);
#8259=ORIENTED_EDGE('',*,*,#6322,.T.);
#8260=ORIENTED_EDGE('',*,*,#6323,.T.);
#8261=ORIENTED_EDGE('',*,*,#5454,.T.);
#8262=ORIENTED_EDGE('',*,*,#6324,.T.);
#8263=ORIENTED_EDGE('',*,*,#6167,.F.);
#8264=ORIENTED_EDGE('',*,*,#6325,.T.);
#8265=ORIENTED_EDGE('',*,*,#6326,.T.);
#8266=ORIENTED_EDGE('',*,*,#6327,.T.);
#8267=ORIENTED_EDGE('',*,*,#6328,.T.);
#8268=ORIENTED_EDGE('',*,*,#6329,.T.);
#8269=ORIENTED_EDGE('',*,*,#6330,.T.);
#8270=ORIENTED_EDGE('',*,*,#6331,.T.);
#8271=ORIENTED_EDGE('',*,*,#5461,.T.);
#8272=ORIENTED_EDGE('',*,*,#6332,.T.);
#8273=ORIENTED_EDGE('',*,*,#6333,.T.);
#8274=ORIENTED_EDGE('',*,*,#6334,.T.);
#8275=ORIENTED_EDGE('',*,*,#6335,.T.);
#8276=ORIENTED_EDGE('',*,*,#6336,.T.);
#8277=ORIENTED_EDGE('',*,*,#6337,.T.);
#8278=ORIENTED_EDGE('',*,*,#6338,.T.);
#8279=ORIENTED_EDGE('',*,*,#5489,.T.);
#8280=ORIENTED_EDGE('',*,*,#6339,.T.);
#8281=ORIENTED_EDGE('',*,*,#6340,.T.);
#8282=ORIENTED_EDGE('',*,*,#6341,.T.);
#8283=ORIENTED_EDGE('',*,*,#6342,.T.);
#8284=ORIENTED_EDGE('',*,*,#6343,.T.);
#8285=ORIENTED_EDGE('',*,*,#5487,.T.);
#8286=ORIENTED_EDGE('',*,*,#6344,.T.);
#8287=ORIENTED_EDGE('',*,*,#6345,.T.);
#8288=ORIENTED_EDGE('',*,*,#6346,.T.);
#8289=ORIENTED_EDGE('',*,*,#6347,.T.);
#8290=ORIENTED_EDGE('',*,*,#6348,.T.);
#8291=ORIENTED_EDGE('',*,*,#6349,.T.);
#8292=ORIENTED_EDGE('',*,*,#6350,.T.);
#8293=ORIENTED_EDGE('',*,*,#6351,.T.);
#8294=ORIENTED_EDGE('',*,*,#6352,.T.);
#8295=ORIENTED_EDGE('',*,*,#6353,.T.);
#8296=ORIENTED_EDGE('',*,*,#6354,.T.);
#8297=ORIENTED_EDGE('',*,*,#6355,.T.);
#8298=ORIENTED_EDGE('',*,*,#5478,.T.);
#8299=ORIENTED_EDGE('',*,*,#6345,.F.);
#8300=ORIENTED_EDGE('',*,*,#6356,.T.);
#8301=ORIENTED_EDGE('',*,*,#6340,.F.);
#8302=ORIENTED_EDGE('',*,*,#6357,.T.);
#8303=ORIENTED_EDGE('',*,*,#6342,.F.);
#8304=ORIENTED_EDGE('',*,*,#6358,.T.);
#8305=ORIENTED_EDGE('',*,*,#5493,.F.);
#8306=ORIENTED_EDGE('',*,*,#6359,.T.);
#8307=ORIENTED_EDGE('',*,*,#5491,.F.);
#8308=ORIENTED_EDGE('',*,*,#5480,.T.);
#8309=ORIENTED_EDGE('',*,*,#6347,.F.);
#8310=ORIENTED_EDGE('',*,*,#5484,.T.);
#8311=ORIENTED_EDGE('',*,*,#5483,.F.);
#8312=ORIENTED_EDGE('',*,*,#5650,.F.);
#8313=ORIENTED_EDGE('',*,*,#6360,.F.);
#8314=ORIENTED_EDGE('',*,*,#5492,.F.);
#8315=ORIENTED_EDGE('',*,*,#6360,.T.);
#8316=ORIENTED_EDGE('',*,*,#5649,.F.);
#8317=ORIENTED_EDGE('',*,*,#6361,.F.);
#8318=ORIENTED_EDGE('',*,*,#6359,.F.);
#8319=ORIENTED_EDGE('',*,*,#6361,.T.);
#8320=ORIENTED_EDGE('',*,*,#5648,.F.);
#8321=ORIENTED_EDGE('',*,*,#6362,.F.);
#8322=ORIENTED_EDGE('',*,*,#6343,.F.);
#8323=ORIENTED_EDGE('',*,*,#5485,.T.);
#8324=ORIENTED_EDGE('',*,*,#6346,.F.);
#8325=ORIENTED_EDGE('',*,*,#6363,.F.);
#8326=ORIENTED_EDGE('',*,*,#5651,.F.);
#8327=ORIENTED_EDGE('',*,*,#6362,.T.);
#8328=ORIENTED_EDGE('',*,*,#5647,.F.);
#8329=ORIENTED_EDGE('',*,*,#6364,.F.);
#8330=ORIENTED_EDGE('',*,*,#5488,.F.);
#8331=ORIENTED_EDGE('',*,*,#6363,.T.);
#8332=ORIENTED_EDGE('',*,*,#6357,.F.);
#8333=ORIENTED_EDGE('',*,*,#6365,.F.);
#8334=ORIENTED_EDGE('',*,*,#5652,.F.);
#8335=ORIENTED_EDGE('',*,*,#6364,.T.);
#8336=ORIENTED_EDGE('',*,*,#5646,.F.);
#8337=ORIENTED_EDGE('',*,*,#6365,.T.);
#8338=ORIENTED_EDGE('',*,*,#6339,.F.);
#8339=ORIENTED_EDGE('',*,*,#5481,.F.);
#8340=ORIENTED_EDGE('',*,*,#5490,.F.);
#8341=ORIENTED_EDGE('',*,*,#6366,.F.);
#8342=ORIENTED_EDGE('',*,*,#6349,.F.);
#8343=ORIENTED_EDGE('',*,*,#6366,.T.);
#8344=ORIENTED_EDGE('',*,*,#6358,.F.);
#8345=ORIENTED_EDGE('',*,*,#6367,.F.);
#8346=ORIENTED_EDGE('',*,*,#6350,.F.);
#8347=ORIENTED_EDGE('',*,*,#6367,.T.);
#8348=ORIENTED_EDGE('',*,*,#6344,.F.);
#8349=ORIENTED_EDGE('',*,*,#6368,.F.);
#8350=ORIENTED_EDGE('',*,*,#6351,.F.);
#8351=ORIENTED_EDGE('',*,*,#5479,.T.);
#8352=ORIENTED_EDGE('',*,*,#6355,.F.);
#8353=ORIENTED_EDGE('',*,*,#6369,.F.);
#8354=ORIENTED_EDGE('',*,*,#6348,.F.);
#8355=ORIENTED_EDGE('',*,*,#6368,.T.);
#8356=ORIENTED_EDGE('',*,*,#5486,.F.);
#8357=ORIENTED_EDGE('',*,*,#6370,.F.);
#8358=ORIENTED_EDGE('',*,*,#6352,.F.);
#8359=ORIENTED_EDGE('',*,*,#6369,.T.);
#8360=ORIENTED_EDGE('',*,*,#6354,.F.);
#8361=ORIENTED_EDGE('',*,*,#6371,.F.);
#8362=ORIENTED_EDGE('',*,*,#6356,.F.);
#8363=ORIENTED_EDGE('',*,*,#6370,.T.);
#8364=ORIENTED_EDGE('',*,*,#6341,.F.);
#8365=ORIENTED_EDGE('',*,*,#6371,.T.);
#8366=ORIENTED_EDGE('',*,*,#6353,.F.);
#8367=ORIENTED_EDGE('',*,*,#6372,.F.);
#8368=ORIENTED_EDGE('',*,*,#5602,.T.);
#8369=ORIENTED_EDGE('',*,*,#6373,.T.);
#8370=ORIENTED_EDGE('',*,*,#6374,.T.);
#8371=ORIENTED_EDGE('',*,*,#6374,.F.);
#8372=ORIENTED_EDGE('',*,*,#6375,.T.);
#8373=ORIENTED_EDGE('',*,*,#6376,.T.);
#8374=ORIENTED_EDGE('',*,*,#6377,.T.);
#8375=ORIENTED_EDGE('',*,*,#6377,.F.);
#8376=ORIENTED_EDGE('',*,*,#6378,.T.);
#8377=ORIENTED_EDGE('',*,*,#5769,.T.);
#8378=ORIENTED_EDGE('',*,*,#6379,.T.);
#8379=ORIENTED_EDGE('',*,*,#6379,.F.);
#8380=ORIENTED_EDGE('',*,*,#5768,.T.);
#8381=ORIENTED_EDGE('',*,*,#6380,.T.);
#8382=ORIENTED_EDGE('',*,*,#6381,.T.);
#8383=ORIENTED_EDGE('',*,*,#6381,.F.);
#8384=ORIENTED_EDGE('',*,*,#6382,.T.);
#8385=ORIENTED_EDGE('',*,*,#6383,.F.);
#8386=ORIENTED_EDGE('',*,*,#6384,.T.);
#8387=ORIENTED_EDGE('',*,*,#6385,.F.);
#8388=ORIENTED_EDGE('',*,*,#6386,.T.);
#8389=ORIENTED_EDGE('',*,*,#5970,.T.);
#8390=ORIENTED_EDGE('',*,*,#6387,.T.);
#8391=ORIENTED_EDGE('',*,*,#6387,.F.);
#8392=ORIENTED_EDGE('',*,*,#5974,.T.);
#8393=ORIENTED_EDGE('',*,*,#6388,.T.);
#8394=ORIENTED_EDGE('',*,*,#6389,.T.);
#8395=ORIENTED_EDGE('',*,*,#6389,.F.);
#8396=ORIENTED_EDGE('',*,*,#6390,.T.);
#8397=ORIENTED_EDGE('',*,*,#6391,.T.);
#8398=ORIENTED_EDGE('',*,*,#6392,.T.);
#8399=ORIENTED_EDGE('',*,*,#6392,.F.);
#8400=ORIENTED_EDGE('',*,*,#6393,.T.);
#8401=ORIENTED_EDGE('',*,*,#5561,.T.);
#8402=ORIENTED_EDGE('',*,*,#6394,.T.);
#8403=ORIENTED_EDGE('',*,*,#6394,.F.);
#8404=ORIENTED_EDGE('',*,*,#5560,.T.);
#8405=ORIENTED_EDGE('',*,*,#6395,.F.);
#8406=ORIENTED_EDGE('',*,*,#6396,.T.);
#8407=ORIENTED_EDGE('',*,*,#6397,.F.);
#8408=ORIENTED_EDGE('',*,*,#5588,.T.);
#8409=ORIENTED_EDGE('',*,*,#6398,.T.);
#8410=ORIENTED_EDGE('',*,*,#6399,.T.);
#8411=ORIENTED_EDGE('',*,*,#6399,.F.);
#8412=ORIENTED_EDGE('',*,*,#6400,.T.);
#8413=ORIENTED_EDGE('',*,*,#6401,.T.);
#8414=ORIENTED_EDGE('',*,*,#6402,.T.);
#8415=ORIENTED_EDGE('',*,*,#6402,.F.);
#8416=ORIENTED_EDGE('',*,*,#6403,.T.);
#8417=ORIENTED_EDGE('',*,*,#5759,.T.);
#8418=ORIENTED_EDGE('',*,*,#6404,.T.);
#8419=ORIENTED_EDGE('',*,*,#6404,.F.);
#8420=ORIENTED_EDGE('',*,*,#5758,.T.);
#8421=ORIENTED_EDGE('',*,*,#6405,.T.);
#8422=ORIENTED_EDGE('',*,*,#6406,.T.);
#8423=ORIENTED_EDGE('',*,*,#6406,.F.);
#8424=ORIENTED_EDGE('',*,*,#6407,.T.);
#8425=ORIENTED_EDGE('',*,*,#6408,.F.);
#8426=ORIENTED_EDGE('',*,*,#6409,.T.);
#8427=ORIENTED_EDGE('',*,*,#6410,.F.);
#8428=ORIENTED_EDGE('',*,*,#6411,.T.);
#8429=ORIENTED_EDGE('',*,*,#5754,.T.);
#8430=ORIENTED_EDGE('',*,*,#6412,.T.);
#8431=ORIENTED_EDGE('',*,*,#6412,.F.);
#8432=ORIENTED_EDGE('',*,*,#5753,.T.);
#8433=ORIENTED_EDGE('',*,*,#6413,.T.);
#8434=ORIENTED_EDGE('',*,*,#6414,.T.);
#8435=ORIENTED_EDGE('',*,*,#6414,.F.);
#8436=ORIENTED_EDGE('',*,*,#6415,.T.);
#8437=ORIENTED_EDGE('',*,*,#6416,.T.);
#8438=ORIENTED_EDGE('',*,*,#6417,.T.);
#8439=ORIENTED_EDGE('',*,*,#6417,.F.);
#8440=ORIENTED_EDGE('',*,*,#6418,.T.);
#8441=ORIENTED_EDGE('',*,*,#5575,.T.);
#8442=ORIENTED_EDGE('',*,*,#6419,.T.);
#8443=ORIENTED_EDGE('',*,*,#6419,.F.);
#8444=ORIENTED_EDGE('',*,*,#5574,.T.);
#8445=ORIENTED_EDGE('',*,*,#6420,.F.);
#8446=ORIENTED_EDGE('',*,*,#6421,.T.);
#8447=ORIENTED_EDGE('',*,*,#6422,.F.);
#8448=ORIENTED_EDGE('',*,*,#6026,.F.);
#8449=ORIENTED_EDGE('',*,*,#6423,.F.);
#8450=ORIENTED_EDGE('',*,*,#6129,.F.);
#8451=ORIENTED_EDGE('',*,*,#6423,.T.);
#8452=ORIENTED_EDGE('',*,*,#6025,.F.);
#8453=ORIENTED_EDGE('',*,*,#6424,.F.);
#8454=ORIENTED_EDGE('',*,*,#6425,.F.);
#8455=ORIENTED_EDGE('',*,*,#6426,.F.);
#8456=ORIENTED_EDGE('',*,*,#6422,.T.);
#8457=ORIENTED_EDGE('',*,*,#6427,.F.);
#8458=ORIENTED_EDGE('',*,*,#5577,.T.);
#8459=ORIENTED_EDGE('',*,*,#6424,.T.);
#8460=ORIENTED_EDGE('',*,*,#6024,.F.);
#8461=ORIENTED_EDGE('',*,*,#6428,.F.);
#8462=ORIENTED_EDGE('',*,*,#6125,.F.);
#8463=ORIENTED_EDGE('',*,*,#6425,.T.);
#8464=ORIENTED_EDGE('',*,*,#6124,.F.);
#8465=ORIENTED_EDGE('',*,*,#6429,.F.);
#8466=ORIENTED_EDGE('',*,*,#6130,.F.);
#8467=ORIENTED_EDGE('',*,*,#6427,.T.);
#8468=ORIENTED_EDGE('',*,*,#6128,.F.);
#8469=ORIENTED_EDGE('',*,*,#6430,.F.);
#8470=ORIENTED_EDGE('',*,*,#5578,.F.);
#8471=ORIENTED_EDGE('',*,*,#6426,.T.);
#8472=ORIENTED_EDGE('',*,*,#5576,.F.);
#8473=ORIENTED_EDGE('',*,*,#6418,.F.);
#8474=ORIENTED_EDGE('',*,*,#6416,.F.);
#8475=ORIENTED_EDGE('',*,*,#6027,.F.);
#8476=ORIENTED_EDGE('',*,*,#6413,.F.);
#8477=ORIENTED_EDGE('',*,*,#5757,.F.);
#8478=ORIENTED_EDGE('',*,*,#6431,.F.);
#8479=ORIENTED_EDGE('',*,*,#6028,.F.);
#8480=ORIENTED_EDGE('',*,*,#6415,.F.);
#8481=ORIENTED_EDGE('',*,*,#6432,.F.);
#8482=ORIENTED_EDGE('',*,*,#5755,.F.);
#8483=ORIENTED_EDGE('',*,*,#6411,.F.);
#8484=ORIENTED_EDGE('',*,*,#6433,.F.);
#8485=ORIENTED_EDGE('',*,*,#5824,.F.);
#8486=ORIENTED_EDGE('',*,*,#6434,.F.);
#8487=ORIENTED_EDGE('',*,*,#5946,.F.);
#8488=ORIENTED_EDGE('',*,*,#6435,.F.);
#8489=ORIENTED_EDGE('',*,*,#5756,.F.);
#8490=ORIENTED_EDGE('',*,*,#6435,.T.);
#8491=ORIENTED_EDGE('',*,*,#5945,.T.);
#8492=ORIENTED_EDGE('',*,*,#6436,.F.);
#8493=ORIENTED_EDGE('',*,*,#6431,.T.);
#8494=ORIENTED_EDGE('',*,*,#6437,.F.);
#8495=ORIENTED_EDGE('',*,*,#6428,.T.);
#8496=ORIENTED_EDGE('',*,*,#6438,.F.);
#8497=ORIENTED_EDGE('',*,*,#6439,.F.);
#8498=ORIENTED_EDGE('',*,*,#6046,.T.);
#8499=ORIENTED_EDGE('',*,*,#6440,.F.);
#8500=ORIENTED_EDGE('',*,*,#6441,.F.);
#8501=ORIENTED_EDGE('',*,*,#6430,.T.);
#8502=ORIENTED_EDGE('',*,*,#6429,.T.);
#8503=ORIENTED_EDGE('',*,*,#6442,.F.);
#8504=ORIENTED_EDGE('',*,*,#6433,.T.);
#8505=ORIENTED_EDGE('',*,*,#6410,.T.);
#8506=ORIENTED_EDGE('',*,*,#6421,.F.);
#8507=ORIENTED_EDGE('',*,*,#6443,.F.);
#8508=ORIENTED_EDGE('',*,*,#6434,.T.);
#8509=ORIENTED_EDGE('',*,*,#6432,.T.);
#8510=ORIENTED_EDGE('',*,*,#6444,.F.);
#8511=ORIENTED_EDGE('',*,*,#5947,.T.);
#8512=ORIENTED_EDGE('',*,*,#6436,.T.);
#8513=ORIENTED_EDGE('',*,*,#5944,.F.);
#8514=ORIENTED_EDGE('',*,*,#6445,.F.);
#8515=ORIENTED_EDGE('',*,*,#6029,.F.);
#8516=ORIENTED_EDGE('',*,*,#6438,.T.);
#8517=ORIENTED_EDGE('',*,*,#6030,.F.);
#8518=ORIENTED_EDGE('',*,*,#6446,.F.);
#8519=ORIENTED_EDGE('',*,*,#6036,.F.);
#8520=ORIENTED_EDGE('',*,*,#6437,.T.);
#8521=ORIENTED_EDGE('',*,*,#6035,.F.);
#8522=ORIENTED_EDGE('',*,*,#6447,.F.);
#8523=ORIENTED_EDGE('',*,*,#6126,.F.);
#8524=ORIENTED_EDGE('',*,*,#6442,.T.);
#8525=ORIENTED_EDGE('',*,*,#6127,.F.);
#8526=ORIENTED_EDGE('',*,*,#6448,.F.);
#8527=ORIENTED_EDGE('',*,*,#5579,.F.);
#8528=ORIENTED_EDGE('',*,*,#6440,.T.);
#8529=ORIENTED_EDGE('',*,*,#6045,.F.);
#8530=ORIENTED_EDGE('',*,*,#6449,.F.);
#8531=ORIENTED_EDGE('',*,*,#6122,.F.);
#8532=ORIENTED_EDGE('',*,*,#6450,.F.);
#8533=ORIENTED_EDGE('',*,*,#6123,.F.);
#8534=ORIENTED_EDGE('',*,*,#6451,.F.);
#8535=ORIENTED_EDGE('',*,*,#5585,.F.);
#8536=ORIENTED_EDGE('',*,*,#6441,.T.);
#8537=ORIENTED_EDGE('',*,*,#6121,.F.);
#8538=ORIENTED_EDGE('',*,*,#6452,.F.);
#8539=ORIENTED_EDGE('',*,*,#6119,.F.);
#8540=ORIENTED_EDGE('',*,*,#6439,.T.);
#8541=ORIENTED_EDGE('',*,*,#6118,.F.);
#8542=ORIENTED_EDGE('',*,*,#6453,.F.);
#8543=ORIENTED_EDGE('',*,*,#6047,.F.);
#8544=ORIENTED_EDGE('',*,*,#6451,.T.);
#8545=ORIENTED_EDGE('',*,*,#6449,.T.);
#8546=ORIENTED_EDGE('',*,*,#6454,.F.);
#8547=ORIENTED_EDGE('',*,*,#5586,.F.);
#8548=ORIENTED_EDGE('',*,*,#6420,.T.);
#8549=ORIENTED_EDGE('',*,*,#5573,.F.);
#8550=ORIENTED_EDGE('',*,*,#6455,.F.);
#8551=ORIENTED_EDGE('',*,*,#5818,.F.);
#8552=ORIENTED_EDGE('',*,*,#6443,.T.);
#8553=ORIENTED_EDGE('',*,*,#6456,.F.);
#8554=ORIENTED_EDGE('',*,*,#5819,.F.);
#8555=ORIENTED_EDGE('',*,*,#6457,.F.);
#8556=ORIENTED_EDGE('',*,*,#5993,.F.);
#8557=ORIENTED_EDGE('',*,*,#6444,.T.);
#8558=ORIENTED_EDGE('',*,*,#5823,.F.);
#8559=ORIENTED_EDGE('',*,*,#6458,.F.);
#8560=ORIENTED_EDGE('',*,*,#5938,.F.);
#8561=ORIENTED_EDGE('',*,*,#6459,.F.);
#8562=ORIENTED_EDGE('',*,*,#5940,.F.);
#8563=ORIENTED_EDGE('',*,*,#6460,.F.);
#8564=ORIENTED_EDGE('',*,*,#5814,.F.);
#8565=ORIENTED_EDGE('',*,*,#6445,.T.);
#8566=ORIENTED_EDGE('',*,*,#5943,.T.);
#8567=ORIENTED_EDGE('',*,*,#6461,.F.);
#8568=ORIENTED_EDGE('',*,*,#6446,.T.);
#8569=ORIENTED_EDGE('',*,*,#6447,.T.);
#8570=ORIENTED_EDGE('',*,*,#6034,.T.);
#8571=ORIENTED_EDGE('',*,*,#6462,.F.);
#8572=ORIENTED_EDGE('',*,*,#6448,.T.);
#8573=ORIENTED_EDGE('',*,*,#6452,.T.);
#8574=ORIENTED_EDGE('',*,*,#6450,.T.);
#8575=ORIENTED_EDGE('',*,*,#6463,.F.);
#8576=ORIENTED_EDGE('',*,*,#6464,.F.);
#8577=ORIENTED_EDGE('',*,*,#6453,.T.);
#8578=ORIENTED_EDGE('',*,*,#6465,.F.);
#8579=ORIENTED_EDGE('',*,*,#6466,.F.);
#8580=ORIENTED_EDGE('',*,*,#5908,.T.);
#8581=ORIENTED_EDGE('',*,*,#6467,.F.);
#8582=ORIENTED_EDGE('',*,*,#6468,.F.);
#8583=ORIENTED_EDGE('',*,*,#6467,.T.);
#8584=ORIENTED_EDGE('',*,*,#5907,.F.);
#8585=ORIENTED_EDGE('',*,*,#6469,.F.);
#8586=ORIENTED_EDGE('',*,*,#5761,.F.);
#8587=ORIENTED_EDGE('',*,*,#6405,.F.);
#8588=ORIENTED_EDGE('',*,*,#5762,.F.);
#8589=ORIENTED_EDGE('',*,*,#6470,.F.);
#8590=ORIENTED_EDGE('',*,*,#6155,.F.);
#8591=ORIENTED_EDGE('',*,*,#6407,.F.);
#8592=ORIENTED_EDGE('',*,*,#6468,.T.);
#8593=ORIENTED_EDGE('',*,*,#5760,.F.);
#8594=ORIENTED_EDGE('',*,*,#6403,.F.);
#8595=ORIENTED_EDGE('',*,*,#6401,.F.);
#8596=ORIENTED_EDGE('',*,*,#6050,.F.);
#8597=ORIENTED_EDGE('',*,*,#6454,.T.);
#8598=ORIENTED_EDGE('',*,*,#6044,.F.);
#8599=ORIENTED_EDGE('',*,*,#6400,.F.);
#8600=ORIENTED_EDGE('',*,*,#6398,.F.);
#8601=ORIENTED_EDGE('',*,*,#5587,.F.);
#8602=ORIENTED_EDGE('',*,*,#6455,.T.);
#8603=ORIENTED_EDGE('',*,*,#5572,.F.);
#8604=ORIENTED_EDGE('',*,*,#6471,.F.);
#8605=ORIENTED_EDGE('',*,*,#6457,.T.);
#8606=ORIENTED_EDGE('',*,*,#5820,.T.);
#8607=ORIENTED_EDGE('',*,*,#6456,.T.);
#8608=ORIENTED_EDGE('',*,*,#6472,.F.);
#8609=ORIENTED_EDGE('',*,*,#6473,.F.);
#8610=ORIENTED_EDGE('',*,*,#5939,.F.);
#8611=ORIENTED_EDGE('',*,*,#6458,.T.);
#8612=ORIENTED_EDGE('',*,*,#6474,.F.);
#8613=ORIENTED_EDGE('',*,*,#6460,.T.);
#8614=ORIENTED_EDGE('',*,*,#6459,.T.);
#8615=ORIENTED_EDGE('',*,*,#6115,.F.);
#8616=ORIENTED_EDGE('',*,*,#5477,.F.);
#8617=ORIENTED_EDGE('',*,*,#5941,.F.);
#8618=ORIENTED_EDGE('',*,*,#6461,.T.);
#8619=ORIENTED_EDGE('',*,*,#5942,.F.);
#8620=ORIENTED_EDGE('',*,*,#5475,.F.);
#8621=ORIENTED_EDGE('',*,*,#6037,.F.);
#8622=ORIENTED_EDGE('',*,*,#6462,.T.);
#8623=ORIENTED_EDGE('',*,*,#6033,.F.);
#8624=ORIENTED_EDGE('',*,*,#6475,.F.);
#8625=ORIENTED_EDGE('',*,*,#5580,.F.);
#8626=ORIENTED_EDGE('',*,*,#6463,.T.);
#8627=ORIENTED_EDGE('',*,*,#5584,.F.);
#8628=ORIENTED_EDGE('',*,*,#6476,.F.);
#8629=ORIENTED_EDGE('',*,*,#6120,.F.);
#8630=ORIENTED_EDGE('',*,*,#6465,.T.);
#8631=ORIENTED_EDGE('',*,*,#6117,.F.);
#8632=ORIENTED_EDGE('',*,*,#6477,.F.);
#8633=ORIENTED_EDGE('',*,*,#6042,.F.);
#8634=ORIENTED_EDGE('',*,*,#6464,.T.);
#8635=ORIENTED_EDGE('',*,*,#6041,.F.);
#8636=ORIENTED_EDGE('',*,*,#6478,.F.);
#8637=ORIENTED_EDGE('',*,*,#6048,.F.);
#8638=ORIENTED_EDGE('',*,*,#6466,.T.);
#8639=ORIENTED_EDGE('',*,*,#6049,.F.);
#8640=ORIENTED_EDGE('',*,*,#6479,.F.);
#8641=ORIENTED_EDGE('',*,*,#5909,.F.);
#8642=ORIENTED_EDGE('',*,*,#6469,.T.);
#8643=ORIENTED_EDGE('',*,*,#5906,.T.);
#8644=ORIENTED_EDGE('',*,*,#6480,.F.);
#8645=ORIENTED_EDGE('',*,*,#6470,.T.);
#8646=ORIENTED_EDGE('',*,*,#5589,.T.);
#8647=ORIENTED_EDGE('',*,*,#6397,.T.);
#8648=ORIENTED_EDGE('',*,*,#6409,.F.);
#8649=ORIENTED_EDGE('',*,*,#6481,.F.);
#8650=ORIENTED_EDGE('',*,*,#6471,.T.);
#8651=ORIENTED_EDGE('',*,*,#5571,.F.);
#8652=ORIENTED_EDGE('',*,*,#6482,.F.);
#8653=ORIENTED_EDGE('',*,*,#5994,.F.);
#8654=ORIENTED_EDGE('',*,*,#6472,.T.);
#8655=ORIENTED_EDGE('',*,*,#5992,.F.);
#8656=ORIENTED_EDGE('',*,*,#6483,.F.);
#8657=ORIENTED_EDGE('',*,*,#5990,.F.);
#8658=ORIENTED_EDGE('',*,*,#6473,.T.);
#8659=ORIENTED_EDGE('',*,*,#5989,.F.);
#8660=ORIENTED_EDGE('',*,*,#6484,.F.);
#8661=ORIENTED_EDGE('',*,*,#5821,.F.);
#8662=ORIENTED_EDGE('',*,*,#6474,.T.);
#8663=ORIENTED_EDGE('',*,*,#5822,.F.);
#8664=ORIENTED_EDGE('',*,*,#6485,.F.);
#8665=ORIENTED_EDGE('',*,*,#5815,.F.);
#8666=ORIENTED_EDGE('',*,*,#5581,.T.);
#8667=ORIENTED_EDGE('',*,*,#6475,.T.);
#8668=ORIENTED_EDGE('',*,*,#6486,.F.);
#8669=ORIENTED_EDGE('',*,*,#6487,.F.);
#8670=ORIENTED_EDGE('',*,*,#6477,.T.);
#8671=ORIENTED_EDGE('',*,*,#6476,.T.);
#8672=ORIENTED_EDGE('',*,*,#5472,.F.);
#8673=ORIENTED_EDGE('',*,*,#6043,.T.);
#8674=ORIENTED_EDGE('',*,*,#6479,.T.);
#8675=ORIENTED_EDGE('',*,*,#6478,.T.);
#8676=ORIENTED_EDGE('',*,*,#6488,.F.);
#8677=ORIENTED_EDGE('',*,*,#5910,.F.);
#8678=ORIENTED_EDGE('',*,*,#6480,.T.);
#8679=ORIENTED_EDGE('',*,*,#5905,.F.);
#8680=ORIENTED_EDGE('',*,*,#6489,.F.);
#8681=ORIENTED_EDGE('',*,*,#6156,.F.);
#8682=ORIENTED_EDGE('',*,*,#6490,.F.);
#8683=ORIENTED_EDGE('',*,*,#6153,.F.);
#8684=ORIENTED_EDGE('',*,*,#6491,.F.);
#8685=ORIENTED_EDGE('',*,*,#6239,.F.);
#8686=ORIENTED_EDGE('',*,*,#6492,.F.);
#8687=ORIENTED_EDGE('',*,*,#5775,.F.);
#8688=ORIENTED_EDGE('',*,*,#6493,.F.);
#8689=ORIENTED_EDGE('',*,*,#6000,.F.);
#8690=ORIENTED_EDGE('',*,*,#6408,.T.);
#8691=ORIENTED_EDGE('',*,*,#6154,.F.);
#8692=ORIENTED_EDGE('',*,*,#6494,.F.);
#8693=ORIENTED_EDGE('',*,*,#5590,.F.);
#8694=ORIENTED_EDGE('',*,*,#6481,.T.);
#8695=ORIENTED_EDGE('',*,*,#6483,.T.);
#8696=ORIENTED_EDGE('',*,*,#6482,.T.);
#8697=ORIENTED_EDGE('',*,*,#6495,.F.);
#8698=ORIENTED_EDGE('',*,*,#6485,.T.);
#8699=ORIENTED_EDGE('',*,*,#6484,.T.);
#8700=ORIENTED_EDGE('',*,*,#6496,.F.);
#8701=ORIENTED_EDGE('',*,*,#5474,.T.);
#8702=ORIENTED_EDGE('',*,*,#6114,.F.);
#8703=ORIENTED_EDGE('',*,*,#6497,.F.);
#8704=ORIENTED_EDGE('',*,*,#6031,.F.);
#8705=ORIENTED_EDGE('',*,*,#6486,.T.);
#8706=ORIENTED_EDGE('',*,*,#6032,.F.);
#8707=ORIENTED_EDGE('',*,*,#6498,.F.);
#8708=ORIENTED_EDGE('',*,*,#5786,.F.);
#8709=ORIENTED_EDGE('',*,*,#6487,.T.);
#8710=ORIENTED_EDGE('',*,*,#5785,.F.);
#8711=ORIENTED_EDGE('',*,*,#6499,.F.);
#8712=ORIENTED_EDGE('',*,*,#5582,.F.);
#8713=ORIENTED_EDGE('',*,*,#6488,.T.);
#8714=ORIENTED_EDGE('',*,*,#6040,.F.);
#8715=ORIENTED_EDGE('',*,*,#6500,.F.);
#8716=ORIENTED_EDGE('',*,*,#5911,.F.);
#8717=ORIENTED_EDGE('',*,*,#6489,.T.);
#8718=ORIENTED_EDGE('',*,*,#5904,.T.);
#8719=ORIENTED_EDGE('',*,*,#6501,.F.);
#8720=ORIENTED_EDGE('',*,*,#6502,.F.);
#8721=ORIENTED_EDGE('',*,*,#6491,.T.);
#8722=ORIENTED_EDGE('',*,*,#6152,.F.);
#8723=ORIENTED_EDGE('',*,*,#6503,.F.);
#8724=ORIENTED_EDGE('',*,*,#6504,.F.);
#8725=ORIENTED_EDGE('',*,*,#6494,.T.);
#8726=ORIENTED_EDGE('',*,*,#6490,.T.);
#8727=ORIENTED_EDGE('',*,*,#5466,.F.);
#8728=ORIENTED_EDGE('',*,*,#5591,.T.);
#8729=ORIENTED_EDGE('',*,*,#6493,.T.);
#8730=ORIENTED_EDGE('',*,*,#5774,.F.);
#8731=ORIENTED_EDGE('',*,*,#6505,.F.);
#8732=ORIENTED_EDGE('',*,*,#6506,.F.);
#8733=ORIENTED_EDGE('',*,*,#6507,.F.);
#8734=ORIENTED_EDGE('',*,*,#6492,.T.);
#8735=ORIENTED_EDGE('',*,*,#6508,.F.);
#8736=ORIENTED_EDGE('',*,*,#5563,.T.);
#8737=ORIENTED_EDGE('',*,*,#6505,.T.);
#8738=ORIENTED_EDGE('',*,*,#5773,.F.);
#8739=ORIENTED_EDGE('',*,*,#6509,.F.);
#8740=ORIENTED_EDGE('',*,*,#5996,.F.);
#8741=ORIENTED_EDGE('',*,*,#6506,.T.);
#8742=ORIENTED_EDGE('',*,*,#5995,.F.);
#8743=ORIENTED_EDGE('',*,*,#6510,.F.);
#8744=ORIENTED_EDGE('',*,*,#6001,.F.);
#8745=ORIENTED_EDGE('',*,*,#6508,.T.);
#8746=ORIENTED_EDGE('',*,*,#5999,.F.);
#8747=ORIENTED_EDGE('',*,*,#6511,.F.);
#8748=ORIENTED_EDGE('',*,*,#5564,.F.);
#8749=ORIENTED_EDGE('',*,*,#6495,.T.);
#8750=ORIENTED_EDGE('',*,*,#5570,.F.);
#8751=ORIENTED_EDGE('',*,*,#6512,.F.);
#8752=ORIENTED_EDGE('',*,*,#5991,.F.);
#8753=ORIENTED_EDGE('',*,*,#6496,.T.);
#8754=ORIENTED_EDGE('',*,*,#5988,.F.);
#8755=ORIENTED_EDGE('',*,*,#6513,.F.);
#8756=ORIENTED_EDGE('',*,*,#5816,.F.);
#8757=ORIENTED_EDGE('',*,*,#6498,.T.);
#8758=ORIENTED_EDGE('',*,*,#6497,.T.);
#8759=ORIENTED_EDGE('',*,*,#6514,.F.);
#8760=ORIENTED_EDGE('',*,*,#5787,.F.);
#8761=ORIENTED_EDGE('',*,*,#5583,.T.);
#8762=ORIENTED_EDGE('',*,*,#6499,.T.);
#8763=ORIENTED_EDGE('',*,*,#6515,.F.);
#8764=ORIENTED_EDGE('',*,*,#5470,.T.);
#8765=ORIENTED_EDGE('',*,*,#6500,.T.);
#8766=ORIENTED_EDGE('',*,*,#6226,.F.);
#8767=ORIENTED_EDGE('',*,*,#6516,.F.);
#8768=ORIENTED_EDGE('',*,*,#5912,.F.);
#8769=ORIENTED_EDGE('',*,*,#6517,.F.);
#8770=ORIENTED_EDGE('',*,*,#6158,.F.);
#8771=ORIENTED_EDGE('',*,*,#6501,.T.);
#8772=ORIENTED_EDGE('',*,*,#5903,.F.);
#8773=ORIENTED_EDGE('',*,*,#6502,.T.);
#8774=ORIENTED_EDGE('',*,*,#6164,.F.);
#8775=ORIENTED_EDGE('',*,*,#6518,.F.);
#8776=ORIENTED_EDGE('',*,*,#6157,.F.);
#8777=ORIENTED_EDGE('',*,*,#6503,.T.);
#8778=ORIENTED_EDGE('',*,*,#6151,.F.);
#8779=ORIENTED_EDGE('',*,*,#6519,.F.);
#8780=ORIENTED_EDGE('',*,*,#6236,.F.);
#8781=ORIENTED_EDGE('',*,*,#6504,.T.);
#8782=ORIENTED_EDGE('',*,*,#6235,.F.);
#8783=ORIENTED_EDGE('',*,*,#6520,.F.);
#8784=ORIENTED_EDGE('',*,*,#6240,.F.);
#8785=ORIENTED_EDGE('',*,*,#6507,.T.);
#8786=ORIENTED_EDGE('',*,*,#5562,.F.);
#8787=ORIENTED_EDGE('',*,*,#6393,.F.);
#8788=ORIENTED_EDGE('',*,*,#6391,.F.);
#8789=ORIENTED_EDGE('',*,*,#5776,.F.);
#8790=ORIENTED_EDGE('',*,*,#6388,.F.);
#8791=ORIENTED_EDGE('',*,*,#5973,.F.);
#8792=ORIENTED_EDGE('',*,*,#6521,.F.);
#8793=ORIENTED_EDGE('',*,*,#5777,.F.);
#8794=ORIENTED_EDGE('',*,*,#6390,.F.);
#8795=ORIENTED_EDGE('',*,*,#6522,.F.);
#8796=ORIENTED_EDGE('',*,*,#5971,.F.);
#8797=ORIENTED_EDGE('',*,*,#6386,.F.);
#8798=ORIENTED_EDGE('',*,*,#6523,.F.);
#8799=ORIENTED_EDGE('',*,*,#6290,.F.);
#8800=ORIENTED_EDGE('',*,*,#6524,.F.);
#8801=ORIENTED_EDGE('',*,*,#5954,.F.);
#8802=ORIENTED_EDGE('',*,*,#6525,.F.);
#8803=ORIENTED_EDGE('',*,*,#5972,.F.);
#8804=ORIENTED_EDGE('',*,*,#6525,.T.);
#8805=ORIENTED_EDGE('',*,*,#5953,.T.);
#8806=ORIENTED_EDGE('',*,*,#6526,.F.);
#8807=ORIENTED_EDGE('',*,*,#6521,.T.);
#8808=ORIENTED_EDGE('',*,*,#6527,.F.);
#8809=ORIENTED_EDGE('',*,*,#6509,.T.);
#8810=ORIENTED_EDGE('',*,*,#6528,.F.);
#8811=ORIENTED_EDGE('',*,*,#6511,.T.);
#8812=ORIENTED_EDGE('',*,*,#6510,.T.);
#8813=ORIENTED_EDGE('',*,*,#6529,.F.);
#8814=ORIENTED_EDGE('',*,*,#6513,.T.);
#8815=ORIENTED_EDGE('',*,*,#6512,.T.);
#8816=ORIENTED_EDGE('',*,*,#6530,.F.);
#8817=ORIENTED_EDGE('',*,*,#5817,.T.);
#8818=ORIENTED_EDGE('',*,*,#6514,.T.);
#8819=ORIENTED_EDGE('',*,*,#6116,.F.);
#8820=ORIENTED_EDGE('',*,*,#6531,.F.);
#8821=ORIENTED_EDGE('',*,*,#5788,.F.);
#8822=ORIENTED_EDGE('',*,*,#6515,.T.);
#8823=ORIENTED_EDGE('',*,*,#5784,.F.);
#8824=ORIENTED_EDGE('',*,*,#6532,.F.);
#8825=ORIENTED_EDGE('',*,*,#6038,.F.);
#8826=ORIENTED_EDGE('',*,*,#5913,.F.);
#8827=ORIENTED_EDGE('',*,*,#6516,.T.);
#8828=ORIENTED_EDGE('',*,*,#6533,.F.);
#8829=ORIENTED_EDGE('',*,*,#5744,.T.);
#8830=ORIENTED_EDGE('',*,*,#6519,.T.);
#8831=ORIENTED_EDGE('',*,*,#6518,.T.);
#8832=ORIENTED_EDGE('',*,*,#6534,.F.);
#8833=ORIENTED_EDGE('',*,*,#5468,.T.);
#8834=ORIENTED_EDGE('',*,*,#6520,.T.);
#8835=ORIENTED_EDGE('',*,*,#6535,.F.);
#8836=ORIENTED_EDGE('',*,*,#6523,.T.);
#8837=ORIENTED_EDGE('',*,*,#6385,.T.);
#8838=ORIENTED_EDGE('',*,*,#6396,.F.);
#8839=ORIENTED_EDGE('',*,*,#6536,.F.);
#8840=ORIENTED_EDGE('',*,*,#6524,.T.);
#8841=ORIENTED_EDGE('',*,*,#6522,.T.);
#8842=ORIENTED_EDGE('',*,*,#6537,.F.);
#8843=ORIENTED_EDGE('',*,*,#5955,.T.);
#8844=ORIENTED_EDGE('',*,*,#6526,.T.);
#8845=ORIENTED_EDGE('',*,*,#5952,.F.);
#8846=ORIENTED_EDGE('',*,*,#6538,.F.);
#8847=ORIENTED_EDGE('',*,*,#5778,.F.);
#8848=ORIENTED_EDGE('',*,*,#6528,.T.);
#8849=ORIENTED_EDGE('',*,*,#5779,.F.);
#8850=ORIENTED_EDGE('',*,*,#6539,.F.);
#8851=ORIENTED_EDGE('',*,*,#5809,.F.);
#8852=ORIENTED_EDGE('',*,*,#6527,.T.);
#8853=ORIENTED_EDGE('',*,*,#5808,.F.);
#8854=ORIENTED_EDGE('',*,*,#6540,.F.);
#8855=ORIENTED_EDGE('',*,*,#5997,.F.);
#8856=ORIENTED_EDGE('',*,*,#6529,.T.);
#8857=ORIENTED_EDGE('',*,*,#5998,.F.);
#8858=ORIENTED_EDGE('',*,*,#6541,.F.);
#8859=ORIENTED_EDGE('',*,*,#5565,.F.);
#8860=ORIENTED_EDGE('',*,*,#6530,.T.);
#8861=ORIENTED_EDGE('',*,*,#5569,.F.);
#8862=ORIENTED_EDGE('',*,*,#6542,.F.);
#8863=ORIENTED_EDGE('',*,*,#5811,.F.);
#8864=ORIENTED_EDGE('',*,*,#6531,.T.);
#8865=ORIENTED_EDGE('',*,*,#5812,.F.);
#8866=ORIENTED_EDGE('',*,*,#6543,.F.);
#8867=ORIENTED_EDGE('',*,*,#5789,.F.);
#8868=ORIENTED_EDGE('',*,*,#6532,.T.);
#8869=ORIENTED_EDGE('',*,*,#5783,.F.);
#8870=ORIENTED_EDGE('',*,*,#6544,.F.);
#8871=ORIENTED_EDGE('',*,*,#6227,.F.);
#8872=ORIENTED_EDGE('',*,*,#6533,.T.);
#8873=ORIENTED_EDGE('',*,*,#6225,.F.);
#8874=ORIENTED_EDGE('',*,*,#6545,.F.);
#8875=ORIENTED_EDGE('',*,*,#5741,.F.);
#8876=ORIENTED_EDGE('',*,*,#6534,.T.);
#8877=ORIENTED_EDGE('',*,*,#6163,.F.);
#8878=ORIENTED_EDGE('',*,*,#6546,.F.);
#8879=ORIENTED_EDGE('',*,*,#6237,.F.);
#8880=ORIENTED_EDGE('',*,*,#6535,.T.);
#8881=ORIENTED_EDGE('',*,*,#6238,.F.);
#8882=ORIENTED_EDGE('',*,*,#6547,.F.);
#8883=ORIENTED_EDGE('',*,*,#5592,.F.);
#8884=ORIENTED_EDGE('',*,*,#6395,.T.);
#8885=ORIENTED_EDGE('',*,*,#5559,.F.);
#8886=ORIENTED_EDGE('',*,*,#6548,.F.);
#8887=ORIENTED_EDGE('',*,*,#6284,.F.);
#8888=ORIENTED_EDGE('',*,*,#6536,.T.);
#8889=ORIENTED_EDGE('',*,*,#6549,.F.);
#8890=ORIENTED_EDGE('',*,*,#6285,.F.);
#8891=ORIENTED_EDGE('',*,*,#6550,.F.);
#8892=ORIENTED_EDGE('',*,*,#6331,.F.);
#8893=ORIENTED_EDGE('',*,*,#6537,.T.);
#8894=ORIENTED_EDGE('',*,*,#6289,.F.);
#8895=ORIENTED_EDGE('',*,*,#6551,.F.);
#8896=ORIENTED_EDGE('',*,*,#5956,.F.);
#8897=ORIENTED_EDGE('',*,*,#6552,.F.);
#8898=ORIENTED_EDGE('',*,*,#5958,.F.);
#8899=ORIENTED_EDGE('',*,*,#6553,.F.);
#8900=ORIENTED_EDGE('',*,*,#6280,.F.);
#8901=ORIENTED_EDGE('',*,*,#6538,.T.);
#8902=ORIENTED_EDGE('',*,*,#5951,.T.);
#8903=ORIENTED_EDGE('',*,*,#6554,.F.);
#8904=ORIENTED_EDGE('',*,*,#6539,.T.);
#8905=ORIENTED_EDGE('',*,*,#6540,.T.);
#8906=ORIENTED_EDGE('',*,*,#5807,.T.);
#8907=ORIENTED_EDGE('',*,*,#5464,.F.);
#8908=ORIENTED_EDGE('',*,*,#6541,.T.);
#8909=ORIENTED_EDGE('',*,*,#6542,.T.);
#8910=ORIENTED_EDGE('',*,*,#5568,.T.);
#8911=ORIENTED_EDGE('',*,*,#6555,.F.);
#8912=ORIENTED_EDGE('',*,*,#6543,.T.);
#8913=ORIENTED_EDGE('',*,*,#6544,.T.);
#8914=ORIENTED_EDGE('',*,*,#5782,.F.);
#8915=ORIENTED_EDGE('',*,*,#5746,.F.);
#8916=ORIENTED_EDGE('',*,*,#6545,.T.);
#8917=ORIENTED_EDGE('',*,*,#6546,.T.);
#8918=ORIENTED_EDGE('',*,*,#6162,.T.);
#8919=ORIENTED_EDGE('',*,*,#6556,.F.);
#8920=ORIENTED_EDGE('',*,*,#6547,.T.);
#8921=ORIENTED_EDGE('',*,*,#6548,.T.);
#8922=ORIENTED_EDGE('',*,*,#5558,.F.);
#8923=ORIENTED_EDGE('',*,*,#5458,.F.);
#8924=ORIENTED_EDGE('',*,*,#6550,.T.);
#8925=ORIENTED_EDGE('',*,*,#6286,.T.);
#8926=ORIENTED_EDGE('',*,*,#6549,.T.);
#8927=ORIENTED_EDGE('',*,*,#6557,.F.);
#8928=ORIENTED_EDGE('',*,*,#6558,.F.);
#8929=ORIENTED_EDGE('',*,*,#5957,.F.);
#8930=ORIENTED_EDGE('',*,*,#6551,.T.);
#8931=ORIENTED_EDGE('',*,*,#6559,.F.);
#8932=ORIENTED_EDGE('',*,*,#6553,.T.);
#8933=ORIENTED_EDGE('',*,*,#6552,.T.);
#8934=ORIENTED_EDGE('',*,*,#5985,.F.);
#8935=ORIENTED_EDGE('',*,*,#6560,.F.);
#8936=ORIENTED_EDGE('',*,*,#5948,.F.);
#8937=ORIENTED_EDGE('',*,*,#6554,.T.);
#8938=ORIENTED_EDGE('',*,*,#5950,.F.);
#8939=ORIENTED_EDGE('',*,*,#6561,.F.);
#8940=ORIENTED_EDGE('',*,*,#5810,.F.);
#8941=ORIENTED_EDGE('',*,*,#6555,.T.);
#8942=ORIENTED_EDGE('',*,*,#5567,.F.);
#8943=ORIENTED_EDGE('',*,*,#6562,.F.);
#8944=ORIENTED_EDGE('',*,*,#5790,.F.);
#8945=ORIENTED_EDGE('',*,*,#6563,.F.);
#8946=ORIENTED_EDGE('',*,*,#5800,.F.);
#8947=ORIENTED_EDGE('',*,*,#6564,.F.);
#8948=ORIENTED_EDGE('',*,*,#6160,.F.);
#8949=ORIENTED_EDGE('',*,*,#6556,.T.);
#8950=ORIENTED_EDGE('',*,*,#6161,.F.);
#8951=ORIENTED_EDGE('',*,*,#6565,.F.);
#8952=ORIENTED_EDGE('',*,*,#5593,.F.);
#8953=ORIENTED_EDGE('',*,*,#6557,.T.);
#8954=ORIENTED_EDGE('',*,*,#6330,.F.);
#8955=ORIENTED_EDGE('',*,*,#6566,.F.);
#8956=ORIENTED_EDGE('',*,*,#6328,.F.);
#8957=ORIENTED_EDGE('',*,*,#6558,.T.);
#8958=ORIENTED_EDGE('',*,*,#6327,.F.);
#8959=ORIENTED_EDGE('',*,*,#6567,.F.);
#8960=ORIENTED_EDGE('',*,*,#6287,.F.);
#8961=ORIENTED_EDGE('',*,*,#6559,.T.);
#8962=ORIENTED_EDGE('',*,*,#6288,.F.);
#8963=ORIENTED_EDGE('',*,*,#6568,.F.);
#8964=ORIENTED_EDGE('',*,*,#6281,.F.);
#8965=ORIENTED_EDGE('',*,*,#5949,.F.);
#8966=ORIENTED_EDGE('',*,*,#6560,.T.);
#8967=ORIENTED_EDGE('',*,*,#6569,.F.);
#8968=ORIENTED_EDGE('',*,*,#6561,.T.);
#8969=ORIENTED_EDGE('',*,*,#5566,.T.);
#8970=ORIENTED_EDGE('',*,*,#5462,.T.);
#8971=ORIENTED_EDGE('',*,*,#6570,.F.);
#8972=ORIENTED_EDGE('',*,*,#6562,.T.);
#8973=ORIENTED_EDGE('',*,*,#6565,.T.);
#8974=ORIENTED_EDGE('',*,*,#6564,.T.);
#8975=ORIENTED_EDGE('',*,*,#6571,.F.);
#8976=ORIENTED_EDGE('',*,*,#5594,.T.);
#8977=ORIENTED_EDGE('',*,*,#6566,.T.);
#8978=ORIENTED_EDGE('',*,*,#5460,.T.);
#8979=ORIENTED_EDGE('',*,*,#6572,.F.);
#8980=ORIENTED_EDGE('',*,*,#6568,.T.);
#8981=ORIENTED_EDGE('',*,*,#6567,.T.);
#8982=ORIENTED_EDGE('',*,*,#6573,.F.);
#8983=ORIENTED_EDGE('',*,*,#6569,.T.);
#8984=ORIENTED_EDGE('',*,*,#5984,.F.);
#8985=ORIENTED_EDGE('',*,*,#6574,.F.);
#8986=ORIENTED_EDGE('',*,*,#5805,.F.);
#8987=ORIENTED_EDGE('',*,*,#6570,.T.);
#8988=ORIENTED_EDGE('',*,*,#5806,.F.);
#8989=ORIENTED_EDGE('',*,*,#6575,.F.);
#8990=ORIENTED_EDGE('',*,*,#5791,.F.);
#8991=ORIENTED_EDGE('',*,*,#6571,.T.);
#8992=ORIENTED_EDGE('',*,*,#5799,.F.);
#8993=ORIENTED_EDGE('',*,*,#6576,.F.);
#8994=ORIENTED_EDGE('',*,*,#5595,.F.);
#8995=ORIENTED_EDGE('',*,*,#6577,.F.);
#8996=ORIENTED_EDGE('',*,*,#6165,.F.);
#8997=ORIENTED_EDGE('',*,*,#6578,.F.);
#8998=ORIENTED_EDGE('',*,*,#5597,.F.);
#8999=ORIENTED_EDGE('',*,*,#6579,.F.);
#9000=ORIENTED_EDGE('',*,*,#6170,.F.);
#9001=ORIENTED_EDGE('',*,*,#6580,.F.);
#9002=ORIENTED_EDGE('',*,*,#6228,.F.);
#9003=ORIENTED_EDGE('',*,*,#6171,.T.);
#9004=ORIENTED_EDGE('',*,*,#6579,.T.);
#9005=ORIENTED_EDGE('',*,*,#6581,.F.);
#9006=ORIENTED_EDGE('',*,*,#6578,.T.);
#9007=ORIENTED_EDGE('',*,*,#6572,.T.);
#9008=ORIENTED_EDGE('',*,*,#5557,.F.);
#9009=ORIENTED_EDGE('',*,*,#6582,.F.);
#9010=ORIENTED_EDGE('',*,*,#6329,.F.);
#9011=ORIENTED_EDGE('',*,*,#6573,.T.);
#9012=ORIENTED_EDGE('',*,*,#6326,.F.);
#9013=ORIENTED_EDGE('',*,*,#6583,.F.);
#9014=ORIENTED_EDGE('',*,*,#6282,.F.);
#9015=ORIENTED_EDGE('',*,*,#6575,.T.);
#9016=ORIENTED_EDGE('',*,*,#6574,.T.);
#9017=ORIENTED_EDGE('',*,*,#6584,.F.);
#9018=ORIENTED_EDGE('',*,*,#5792,.F.);
#9019=ORIENTED_EDGE('',*,*,#5596,.T.);
#9020=ORIENTED_EDGE('',*,*,#6576,.T.);
#9021=ORIENTED_EDGE('',*,*,#6585,.F.);
#9022=ORIENTED_EDGE('',*,*,#6577,.T.);
#9023=ORIENTED_EDGE('',*,*,#6586,.F.);
#9024=ORIENTED_EDGE('',*,*,#6587,.F.);
#9025=ORIENTED_EDGE('',*,*,#6580,.T.);
#9026=ORIENTED_EDGE('',*,*,#6587,.T.);
#9027=ORIENTED_EDGE('',*,*,#6175,.F.);
#9028=ORIENTED_EDGE('',*,*,#6588,.F.);
#9029=ORIENTED_EDGE('',*,*,#6229,.F.);
#9030=ORIENTED_EDGE('',*,*,#6589,.F.);
#9031=ORIENTED_EDGE('',*,*,#6230,.F.);
#9032=ORIENTED_EDGE('',*,*,#6590,.F.);
#9033=ORIENTED_EDGE('',*,*,#6232,.F.);
#9034=ORIENTED_EDGE('',*,*,#6581,.T.);
#9035=ORIENTED_EDGE('',*,*,#6231,.F.);
#9036=ORIENTED_EDGE('',*,*,#6591,.F.);
#9037=ORIENTED_EDGE('',*,*,#5598,.F.);
#9038=ORIENTED_EDGE('',*,*,#6583,.T.);
#9039=ORIENTED_EDGE('',*,*,#6582,.T.);
#9040=ORIENTED_EDGE('',*,*,#6592,.F.);
#9041=ORIENTED_EDGE('',*,*,#6283,.T.);
#9042=ORIENTED_EDGE('',*,*,#6584,.T.);
#9043=ORIENTED_EDGE('',*,*,#5987,.F.);
#9044=ORIENTED_EDGE('',*,*,#6593,.F.);
#9045=ORIENTED_EDGE('',*,*,#5793,.F.);
#9046=ORIENTED_EDGE('',*,*,#6585,.T.);
#9047=ORIENTED_EDGE('',*,*,#5798,.F.);
#9048=ORIENTED_EDGE('',*,*,#6594,.F.);
#9049=ORIENTED_EDGE('',*,*,#6166,.F.);
#9050=ORIENTED_EDGE('',*,*,#6586,.T.);
#9051=ORIENTED_EDGE('',*,*,#6169,.F.);
#9052=ORIENTED_EDGE('',*,*,#6595,.F.);
#9053=ORIENTED_EDGE('',*,*,#6176,.F.);
#9054=ORIENTED_EDGE('',*,*,#6588,.T.);
#9055=ORIENTED_EDGE('',*,*,#6174,.T.);
#9056=ORIENTED_EDGE('',*,*,#6596,.F.);
#9057=ORIENTED_EDGE('',*,*,#6590,.T.);
#9058=ORIENTED_EDGE('',*,*,#6591,.T.);
#9059=ORIENTED_EDGE('',*,*,#6589,.T.);
#9060=ORIENTED_EDGE('',*,*,#6597,.F.);
#9061=ORIENTED_EDGE('',*,*,#6592,.T.);
#9062=ORIENTED_EDGE('',*,*,#5556,.F.);
#9063=ORIENTED_EDGE('',*,*,#6598,.F.);
#9064=ORIENTED_EDGE('',*,*,#6278,.F.);
#9065=ORIENTED_EDGE('',*,*,#6593,.T.);
#9066=ORIENTED_EDGE('',*,*,#6279,.F.);
#9067=ORIENTED_EDGE('',*,*,#6599,.F.);
#9068=ORIENTED_EDGE('',*,*,#5794,.F.);
#9069=ORIENTED_EDGE('',*,*,#6594,.T.);
#9070=ORIENTED_EDGE('',*,*,#5797,.F.);
#9071=ORIENTED_EDGE('',*,*,#5455,.F.);
#9072=ORIENTED_EDGE('',*,*,#6325,.F.);
#9073=ORIENTED_EDGE('',*,*,#6600,.F.);
#9074=ORIENTED_EDGE('',*,*,#5928,.F.);
#9075=ORIENTED_EDGE('',*,*,#6601,.F.);
#9076=ORIENTED_EDGE('',*,*,#6595,.T.);
#9077=ORIENTED_EDGE('',*,*,#6601,.T.);
#9078=ORIENTED_EDGE('',*,*,#5927,.F.);
#9079=ORIENTED_EDGE('',*,*,#6602,.F.);
#9080=ORIENTED_EDGE('',*,*,#6177,.F.);
#9081=ORIENTED_EDGE('',*,*,#6596,.T.);
#9082=ORIENTED_EDGE('',*,*,#6173,.F.);
#9083=ORIENTED_EDGE('',*,*,#6603,.F.);
#9084=ORIENTED_EDGE('',*,*,#6233,.F.);
#9085=ORIENTED_EDGE('',*,*,#6597,.T.);
#9086=ORIENTED_EDGE('',*,*,#6234,.F.);
#9087=ORIENTED_EDGE('',*,*,#6604,.F.);
#9088=ORIENTED_EDGE('',*,*,#5599,.F.);
#9089=ORIENTED_EDGE('',*,*,#6598,.T.);
#9090=ORIENTED_EDGE('',*,*,#5555,.T.);
#9091=ORIENTED_EDGE('',*,*,#6605,.F.);
#9092=ORIENTED_EDGE('',*,*,#6599,.T.);
#9093=ORIENTED_EDGE('',*,*,#6600,.T.);
#9094=ORIENTED_EDGE('',*,*,#6168,.F.);
#9095=ORIENTED_EDGE('',*,*,#6606,.F.);
#9096=ORIENTED_EDGE('',*,*,#5929,.F.);
#9097=ORIENTED_EDGE('',*,*,#6602,.T.);
#9098=ORIENTED_EDGE('',*,*,#5937,.T.);
#9099=ORIENTED_EDGE('',*,*,#6607,.F.);
#9100=ORIENTED_EDGE('',*,*,#6608,.F.);
#9101=ORIENTED_EDGE('',*,*,#6604,.T.);
#9102=ORIENTED_EDGE('',*,*,#6603,.T.);
#9103=ORIENTED_EDGE('',*,*,#6609,.F.);
#9104=ORIENTED_EDGE('',*,*,#5600,.F.);
#9105=ORIENTED_EDGE('',*,*,#6605,.T.);
#9106=ORIENTED_EDGE('',*,*,#5554,.F.);
#9107=ORIENTED_EDGE('',*,*,#6610,.F.);
#9108=ORIENTED_EDGE('',*,*,#5795,.F.);
#9109=ORIENTED_EDGE('',*,*,#5457,.T.);
#9110=ORIENTED_EDGE('',*,*,#5796,.F.);
#9111=ORIENTED_EDGE('',*,*,#6611,.F.);
#9112=ORIENTED_EDGE('',*,*,#6272,.F.);
#9113=ORIENTED_EDGE('',*,*,#6606,.T.);
#9114=ORIENTED_EDGE('',*,*,#6324,.F.);
#9115=ORIENTED_EDGE('',*,*,#6612,.F.);
#9116=ORIENTED_EDGE('',*,*,#5930,.F.);
#9117=ORIENTED_EDGE('',*,*,#6607,.T.);
#9118=ORIENTED_EDGE('',*,*,#5936,.F.);
#9119=ORIENTED_EDGE('',*,*,#6613,.F.);
#9120=ORIENTED_EDGE('',*,*,#5771,.F.);
#9121=ORIENTED_EDGE('',*,*,#6380,.F.);
#9122=ORIENTED_EDGE('',*,*,#5772,.F.);
#9123=ORIENTED_EDGE('',*,*,#6614,.F.);
#9124=ORIENTED_EDGE('',*,*,#6269,.F.);
#9125=ORIENTED_EDGE('',*,*,#6382,.F.);
#9126=ORIENTED_EDGE('',*,*,#6608,.T.);
#9127=ORIENTED_EDGE('',*,*,#5770,.F.);
#9128=ORIENTED_EDGE('',*,*,#6378,.F.);
#9129=ORIENTED_EDGE('',*,*,#6376,.F.);
#9130=ORIENTED_EDGE('',*,*,#6178,.F.);
#9131=ORIENTED_EDGE('',*,*,#6609,.T.);
#9132=ORIENTED_EDGE('',*,*,#6172,.F.);
#9133=ORIENTED_EDGE('',*,*,#6375,.F.);
#9134=ORIENTED_EDGE('',*,*,#6373,.F.);
#9135=ORIENTED_EDGE('',*,*,#5601,.F.);
#9136=ORIENTED_EDGE('',*,*,#6610,.T.);
#9137=ORIENTED_EDGE('',*,*,#5553,.T.);
#9138=ORIENTED_EDGE('',*,*,#6615,.F.);
#9139=ORIENTED_EDGE('',*,*,#6611,.T.);
#9140=ORIENTED_EDGE('',*,*,#6612,.T.);
#9141=ORIENTED_EDGE('',*,*,#5453,.T.);
#9142=ORIENTED_EDGE('',*,*,#6616,.F.);
#9143=ORIENTED_EDGE('',*,*,#5931,.F.);
#9144=ORIENTED_EDGE('',*,*,#6613,.T.);
#9145=ORIENTED_EDGE('',*,*,#5935,.T.);
#9146=ORIENTED_EDGE('',*,*,#6617,.F.);
#9147=ORIENTED_EDGE('',*,*,#6614,.T.);
#9148=ORIENTED_EDGE('',*,*,#5547,.T.);
#9149=ORIENTED_EDGE('',*,*,#6372,.T.);
#9150=ORIENTED_EDGE('',*,*,#6384,.F.);
#9151=ORIENTED_EDGE('',*,*,#6618,.F.);
#9152=ORIENTED_EDGE('',*,*,#6615,.T.);
#9153=ORIENTED_EDGE('',*,*,#5552,.F.);
#9154=ORIENTED_EDGE('',*,*,#6619,.F.);
#9155=ORIENTED_EDGE('',*,*,#6273,.F.);
#9156=ORIENTED_EDGE('',*,*,#6616,.T.);
#9157=ORIENTED_EDGE('',*,*,#6277,.F.);
#9158=ORIENTED_EDGE('',*,*,#6620,.F.);
#9159=ORIENTED_EDGE('',*,*,#5932,.F.);
#9160=ORIENTED_EDGE('',*,*,#6617,.T.);
#9161=ORIENTED_EDGE('',*,*,#5934,.F.);
#9162=ORIENTED_EDGE('',*,*,#6621,.F.);
#9163=ORIENTED_EDGE('',*,*,#6270,.F.);
#9164=ORIENTED_EDGE('',*,*,#6383,.T.);
#9165=ORIENTED_EDGE('',*,*,#6268,.F.);
#9166=ORIENTED_EDGE('',*,*,#6622,.F.);
#9167=ORIENTED_EDGE('',*,*,#5548,.F.);
#9168=ORIENTED_EDGE('',*,*,#6618,.T.);
#9169=ORIENTED_EDGE('',*,*,#6623,.F.);
#9170=ORIENTED_EDGE('',*,*,#5550,.F.);
#9171=ORIENTED_EDGE('',*,*,#6624,.F.);
#9172=ORIENTED_EDGE('',*,*,#6336,.F.);
#9173=ORIENTED_EDGE('',*,*,#6625,.F.);
#9174=ORIENTED_EDGE('',*,*,#5551,.F.);
#9175=ORIENTED_EDGE('',*,*,#6626,.F.);
#9176=ORIENTED_EDGE('',*,*,#6335,.F.);
#9177=ORIENTED_EDGE('',*,*,#6619,.T.);
#9178=ORIENTED_EDGE('',*,*,#6625,.T.);
#9179=ORIENTED_EDGE('',*,*,#6627,.F.);
#9180=ORIENTED_EDGE('',*,*,#6274,.T.);
#9181=ORIENTED_EDGE('',*,*,#5933,.T.);
#9182=ORIENTED_EDGE('',*,*,#6620,.T.);
#9183=ORIENTED_EDGE('',*,*,#6628,.F.);
#9184=ORIENTED_EDGE('',*,*,#6621,.T.);
#9185=ORIENTED_EDGE('',*,*,#5549,.T.);
#9186=ORIENTED_EDGE('',*,*,#6622,.T.);
#9187=ORIENTED_EDGE('',*,*,#6629,.F.);
#9188=ORIENTED_EDGE('',*,*,#6624,.T.);
#9189=ORIENTED_EDGE('',*,*,#6626,.T.);
#9190=ORIENTED_EDGE('',*,*,#6623,.T.);
#9191=ORIENTED_EDGE('',*,*,#6630,.F.);
#9192=ORIENTED_EDGE('',*,*,#6627,.T.);
#9193=ORIENTED_EDGE('',*,*,#6334,.F.);
#9194=ORIENTED_EDGE('',*,*,#6631,.F.);
#9195=ORIENTED_EDGE('',*,*,#6275,.F.);
#9196=ORIENTED_EDGE('',*,*,#6628,.T.);
#9197=ORIENTED_EDGE('',*,*,#6276,.F.);
#9198=ORIENTED_EDGE('',*,*,#6632,.F.);
#9199=ORIENTED_EDGE('',*,*,#6271,.F.);
#9200=ORIENTED_EDGE('',*,*,#6629,.T.);
#9201=ORIENTED_EDGE('',*,*,#6267,.F.);
#9202=ORIENTED_EDGE('',*,*,#6633,.F.);
#9203=ORIENTED_EDGE('',*,*,#6337,.F.);
#9204=ORIENTED_EDGE('',*,*,#6630,.T.);
#9205=ORIENTED_EDGE('',*,*,#6338,.F.);
#9206=ORIENTED_EDGE('',*,*,#6634,.F.);
#9207=ORIENTED_EDGE('',*,*,#6332,.F.);
#9208=ORIENTED_EDGE('',*,*,#6632,.T.);
#9209=ORIENTED_EDGE('',*,*,#6631,.T.);
#9210=ORIENTED_EDGE('',*,*,#6635,.F.);
#9211=ORIENTED_EDGE('',*,*,#6633,.T.);
#9212=ORIENTED_EDGE('',*,*,#6266,.F.);
#9213=ORIENTED_EDGE('',*,*,#6636,.F.);
#9214=ORIENTED_EDGE('',*,*,#6634,.T.);
#9215=ORIENTED_EDGE('',*,*,#6635,.T.);
#9216=ORIENTED_EDGE('',*,*,#6333,.F.);
#9217=ORIENTED_EDGE('',*,*,#6636,.T.);
#9218=ORIENTED_EDGE('',*,*,#6265,.F.);
#9219=ORIENTED_EDGE('',*,*,#6637,.F.);
#9220=ORIENTED_EDGE('',*,*,#5843,.F.);
#9221=ORIENTED_EDGE('',*,*,#6638,.F.);
#9222=ORIENTED_EDGE('',*,*,#6112,.F.);
#9223=ORIENTED_EDGE('',*,*,#6639,.F.);
#9224=ORIENTED_EDGE('',*,*,#6637,.T.);
#9225=ORIENTED_EDGE('',*,*,#5449,.F.);
#9226=ORIENTED_EDGE('',*,*,#6640,.F.);
#9227=ORIENTED_EDGE('',*,*,#6638,.T.);
#9228=ORIENTED_EDGE('',*,*,#6641,.F.);
#9229=ORIENTED_EDGE('',*,*,#6639,.T.);
#9230=ORIENTED_EDGE('',*,*,#5835,.F.);
#9231=ORIENTED_EDGE('',*,*,#6642,.F.);
#9232=ORIENTED_EDGE('',*,*,#5844,.F.);
#9233=ORIENTED_EDGE('',*,*,#6641,.T.);
#9234=ORIENTED_EDGE('',*,*,#5848,.F.);
#9235=ORIENTED_EDGE('',*,*,#6643,.F.);
#9236=ORIENTED_EDGE('',*,*,#6075,.F.);
#9237=ORIENTED_EDGE('',*,*,#6640,.T.);
#9238=ORIENTED_EDGE('',*,*,#6074,.F.);
#9239=ORIENTED_EDGE('',*,*,#6644,.F.);
#9240=ORIENTED_EDGE('',*,*,#6113,.F.);
#9241=ORIENTED_EDGE('',*,*,#6645,.F.);
#9242=ORIENTED_EDGE('',*,*,#5447,.T.);
#9243=ORIENTED_EDGE('',*,*,#6646,.F.);
#9244=ORIENTED_EDGE('',*,*,#6647,.F.);
#9245=ORIENTED_EDGE('',*,*,#6642,.T.);
#9246=ORIENTED_EDGE('',*,*,#5445,.F.);
#9247=ORIENTED_EDGE('',*,*,#6648,.F.);
#9248=ORIENTED_EDGE('',*,*,#6643,.T.);
#9249=ORIENTED_EDGE('',*,*,#6649,.F.);
#9250=ORIENTED_EDGE('',*,*,#5884,.T.);
#9251=ORIENTED_EDGE('',*,*,#6644,.T.);
#9252=ORIENTED_EDGE('',*,*,#6073,.F.);
#9253=ORIENTED_EDGE('',*,*,#6650,.F.);
#9254=ORIENTED_EDGE('',*,*,#5533,.F.);
#9255=ORIENTED_EDGE('',*,*,#6646,.T.);
#9256=ORIENTED_EDGE('',*,*,#6111,.F.);
#9257=ORIENTED_EDGE('',*,*,#6651,.F.);
#9258=ORIENTED_EDGE('',*,*,#5612,.F.);
#9259=ORIENTED_EDGE('',*,*,#6645,.T.);
#9260=ORIENTED_EDGE('',*,*,#5611,.F.);
#9261=ORIENTED_EDGE('',*,*,#6652,.F.);
#9262=ORIENTED_EDGE('',*,*,#5836,.F.);
#9263=ORIENTED_EDGE('',*,*,#6647,.T.);
#9264=ORIENTED_EDGE('',*,*,#5978,.F.);
#9265=ORIENTED_EDGE('',*,*,#6653,.F.);
#9266=ORIENTED_EDGE('',*,*,#5845,.F.);
#9267=ORIENTED_EDGE('',*,*,#6654,.F.);
#9268=ORIENTED_EDGE('',*,*,#5846,.F.);
#9269=ORIENTED_EDGE('',*,*,#6655,.F.);
#9270=ORIENTED_EDGE('',*,*,#5859,.F.);
#9271=ORIENTED_EDGE('',*,*,#6649,.T.);
#9272=ORIENTED_EDGE('',*,*,#5847,.F.);
#9273=ORIENTED_EDGE('',*,*,#6656,.F.);
#9274=ORIENTED_EDGE('',*,*,#5885,.F.);
#9275=ORIENTED_EDGE('',*,*,#6648,.T.);
#9276=ORIENTED_EDGE('',*,*,#5883,.F.);
#9277=ORIENTED_EDGE('',*,*,#6657,.F.);
#9278=ORIENTED_EDGE('',*,*,#6068,.F.);
#9279=ORIENTED_EDGE('',*,*,#6650,.T.);
#9280=ORIENTED_EDGE('',*,*,#6072,.F.);
#9281=ORIENTED_EDGE('',*,*,#6658,.F.);
#9282=ORIENTED_EDGE('',*,*,#6107,.F.);
#9283=ORIENTED_EDGE('',*,*,#6659,.F.);
#9284=ORIENTED_EDGE('',*,*,#6651,.T.);
#9285=ORIENTED_EDGE('',*,*,#6660,.F.);
#9286=ORIENTED_EDGE('',*,*,#5443,.T.);
#9287=ORIENTED_EDGE('',*,*,#6652,.T.);
#9288=ORIENTED_EDGE('',*,*,#6661,.F.);
#9289=ORIENTED_EDGE('',*,*,#6655,.T.);
#9290=ORIENTED_EDGE('',*,*,#6653,.T.);
#9291=ORIENTED_EDGE('',*,*,#6662,.F.);
#9292=ORIENTED_EDGE('',*,*,#6656,.T.);
#9293=ORIENTED_EDGE('',*,*,#6654,.T.);
#9294=ORIENTED_EDGE('',*,*,#6663,.F.);
#9295=ORIENTED_EDGE('',*,*,#5886,.T.);
#9296=ORIENTED_EDGE('',*,*,#6657,.T.);
#9297=ORIENTED_EDGE('',*,*,#6094,.F.);
#9298=ORIENTED_EDGE('',*,*,#6664,.F.);
#9299=ORIENTED_EDGE('',*,*,#6069,.F.);
#9300=ORIENTED_EDGE('',*,*,#6665,.F.);
#9301=ORIENTED_EDGE('',*,*,#6658,.T.);
#9302=ORIENTED_EDGE('',*,*,#6666,.F.);
#9303=ORIENTED_EDGE('',*,*,#6660,.T.);
#9304=ORIENTED_EDGE('',*,*,#6110,.F.);
#9305=ORIENTED_EDGE('',*,*,#5440,.F.);
#9306=ORIENTED_EDGE('',*,*,#6065,.F.);
#9307=ORIENTED_EDGE('',*,*,#6659,.T.);
#9308=ORIENTED_EDGE('',*,*,#6064,.F.);
#9309=ORIENTED_EDGE('',*,*,#6667,.F.);
#9310=ORIENTED_EDGE('',*,*,#5613,.F.);
#9311=ORIENTED_EDGE('',*,*,#6661,.T.);
#9312=ORIENTED_EDGE('',*,*,#5617,.F.);
#9313=ORIENTED_EDGE('',*,*,#6668,.F.);
#9314=ORIENTED_EDGE('',*,*,#5975,.F.);
#9315=ORIENTED_EDGE('',*,*,#6662,.T.);
#9316=ORIENTED_EDGE('',*,*,#5977,.F.);
#9317=ORIENTED_EDGE('',*,*,#6669,.F.);
#9318=ORIENTED_EDGE('',*,*,#5860,.F.);
#9319=ORIENTED_EDGE('',*,*,#6663,.T.);
#9320=ORIENTED_EDGE('',*,*,#5858,.F.);
#9321=ORIENTED_EDGE('',*,*,#6670,.F.);
#9322=ORIENTED_EDGE('',*,*,#5887,.F.);
#9323=ORIENTED_EDGE('',*,*,#6664,.T.);
#9324=ORIENTED_EDGE('',*,*,#6092,.F.);
#9325=ORIENTED_EDGE('',*,*,#6671,.F.);
#9326=ORIENTED_EDGE('',*,*,#6070,.F.);
#9327=ORIENTED_EDGE('',*,*,#6666,.T.);
#9328=ORIENTED_EDGE('',*,*,#6071,.F.);
#9329=ORIENTED_EDGE('',*,*,#6672,.F.);
#9330=ORIENTED_EDGE('',*,*,#6058,.F.);
#9331=ORIENTED_EDGE('',*,*,#6665,.T.);
#9332=ORIENTED_EDGE('',*,*,#6057,.F.);
#9333=ORIENTED_EDGE('',*,*,#6673,.F.);
#9334=ORIENTED_EDGE('',*,*,#6108,.F.);
#9335=ORIENTED_EDGE('',*,*,#6674,.F.);
#9336=ORIENTED_EDGE('',*,*,#6667,.T.);
#9337=ORIENTED_EDGE('',*,*,#6675,.F.);
#9338=ORIENTED_EDGE('',*,*,#5864,.T.);
#9339=ORIENTED_EDGE('',*,*,#6676,.F.);
#9340=ORIENTED_EDGE('',*,*,#6668,.T.);
#9341=ORIENTED_EDGE('',*,*,#6677,.F.);
#9342=ORIENTED_EDGE('',*,*,#6669,.T.);
#9343=ORIENTED_EDGE('',*,*,#5618,.F.);
#9344=ORIENTED_EDGE('',*,*,#6678,.F.);
#9345=ORIENTED_EDGE('',*,*,#5861,.F.);
#9346=ORIENTED_EDGE('',*,*,#6670,.T.);
#9347=ORIENTED_EDGE('',*,*,#5857,.F.);
#9348=ORIENTED_EDGE('',*,*,#6679,.F.);
#9349=ORIENTED_EDGE('',*,*,#5959,.F.);
#9350=ORIENTED_EDGE('',*,*,#6671,.T.);
#9351=ORIENTED_EDGE('',*,*,#6091,.T.);
#9352=ORIENTED_EDGE('',*,*,#6680,.F.);
#9353=ORIENTED_EDGE('',*,*,#6672,.T.);
#9354=ORIENTED_EDGE('',*,*,#6681,.F.);
#9355=ORIENTED_EDGE('',*,*,#6673,.T.);
#9356=ORIENTED_EDGE('',*,*,#6682,.F.);
#9357=ORIENTED_EDGE('',*,*,#5442,.T.);
#9358=ORIENTED_EDGE('',*,*,#6106,.F.);
#9359=ORIENTED_EDGE('',*,*,#6683,.F.);
#9360=ORIENTED_EDGE('',*,*,#6066,.F.);
#9361=ORIENTED_EDGE('',*,*,#6675,.T.);
#9362=ORIENTED_EDGE('',*,*,#6063,.F.);
#9363=ORIENTED_EDGE('',*,*,#6684,.F.);
#9364=ORIENTED_EDGE('',*,*,#5865,.F.);
#9365=ORIENTED_EDGE('',*,*,#6674,.T.);
#9366=ORIENTED_EDGE('',*,*,#5871,.F.);
#9367=ORIENTED_EDGE('',*,*,#6685,.F.);
#9368=ORIENTED_EDGE('',*,*,#5615,.F.);
#9369=ORIENTED_EDGE('',*,*,#5614,.F.);
#9370=ORIENTED_EDGE('',*,*,#6677,.T.);
#9371=ORIENTED_EDGE('',*,*,#5616,.F.);
#9372=ORIENTED_EDGE('',*,*,#6686,.F.);
#9373=ORIENTED_EDGE('',*,*,#5855,.F.);
#9374=ORIENTED_EDGE('',*,*,#6676,.T.);
#9375=ORIENTED_EDGE('',*,*,#5854,.F.);
#9376=ORIENTED_EDGE('',*,*,#5438,.F.);
#9377=ORIENTED_EDGE('',*,*,#5976,.F.);
#9378=ORIENTED_EDGE('',*,*,#6678,.T.);
#9379=ORIENTED_EDGE('',*,*,#5983,.F.);
#9380=ORIENTED_EDGE('',*,*,#6687,.F.);
#9381=ORIENTED_EDGE('',*,*,#5862,.F.);
#9382=ORIENTED_EDGE('',*,*,#6688,.F.);
#9383=ORIENTED_EDGE('',*,*,#5863,.F.);
#9384=ORIENTED_EDGE('',*,*,#6689,.F.);
#9385=ORIENTED_EDGE('',*,*,#5842,.F.);
#9386=ORIENTED_EDGE('',*,*,#6679,.T.);
#9387=ORIENTED_EDGE('',*,*,#5856,.F.);
#9388=ORIENTED_EDGE('',*,*,#6690,.F.);
#9389=ORIENTED_EDGE('',*,*,#5895,.F.);
#9390=ORIENTED_EDGE('',*,*,#6680,.T.);
#9391=ORIENTED_EDGE('',*,*,#6090,.F.);
#9392=ORIENTED_EDGE('',*,*,#6691,.F.);
#9393=ORIENTED_EDGE('',*,*,#6059,.F.);
#9394=ORIENTED_EDGE('',*,*,#6682,.T.);
#9395=ORIENTED_EDGE('',*,*,#6056,.F.);
#9396=ORIENTED_EDGE('',*,*,#6692,.F.);
#9397=ORIENTED_EDGE('',*,*,#6052,.F.);
#9398=ORIENTED_EDGE('',*,*,#6681,.T.);
#9399=ORIENTED_EDGE('',*,*,#6051,.F.);
#9400=ORIENTED_EDGE('',*,*,#6693,.F.);
#9401=ORIENTED_EDGE('',*,*,#6109,.F.);
#9402=ORIENTED_EDGE('',*,*,#6694,.F.);
#9403=ORIENTED_EDGE('',*,*,#6105,.F.);
#9404=ORIENTED_EDGE('',*,*,#6695,.F.);
#9405=ORIENTED_EDGE('',*,*,#5532,.F.);
#9406=ORIENTED_EDGE('',*,*,#6683,.T.);
#9407=ORIENTED_EDGE('',*,*,#6694,.T.);
#9408=ORIENTED_EDGE('',*,*,#6696,.F.);
#9409=ORIENTED_EDGE('',*,*,#6684,.T.);
#9410=ORIENTED_EDGE('',*,*,#6062,.F.);
#9411=ORIENTED_EDGE('',*,*,#6697,.F.);
#9412=ORIENTED_EDGE('',*,*,#6084,.F.);
#9413=ORIENTED_EDGE('',*,*,#6685,.T.);
#9414=ORIENTED_EDGE('',*,*,#5870,.T.);
#9415=ORIENTED_EDGE('',*,*,#6698,.F.);
#9416=ORIENTED_EDGE('',*,*,#6686,.T.);
#9417=ORIENTED_EDGE('',*,*,#6689,.T.);
#9418=ORIENTED_EDGE('',*,*,#6687,.T.);
#9419=ORIENTED_EDGE('',*,*,#6699,.F.);
#9420=ORIENTED_EDGE('',*,*,#6690,.T.);
#9421=ORIENTED_EDGE('',*,*,#6688,.T.);
#9422=ORIENTED_EDGE('',*,*,#6700,.F.);
#9423=ORIENTED_EDGE('',*,*,#5896,.T.);
#9424=ORIENTED_EDGE('',*,*,#6691,.T.);
#9425=ORIENTED_EDGE('',*,*,#6089,.T.);
#9426=ORIENTED_EDGE('',*,*,#6701,.F.);
#9427=ORIENTED_EDGE('',*,*,#6702,.F.);
#9428=ORIENTED_EDGE('',*,*,#6703,.F.);
#9429=ORIENTED_EDGE('',*,*,#6692,.T.);
#9430=ORIENTED_EDGE('',*,*,#6704,.F.);
#9431=ORIENTED_EDGE('',*,*,#6695,.T.);
#9432=ORIENTED_EDGE('',*,*,#6693,.T.);
#9433=ORIENTED_EDGE('',*,*,#6705,.F.);
#9434=ORIENTED_EDGE('',*,*,#6696,.T.);
#9435=ORIENTED_EDGE('',*,*,#5531,.F.);
#9436=ORIENTED_EDGE('',*,*,#6706,.F.);
#9437=ORIENTED_EDGE('',*,*,#6067,.F.);
#9438=ORIENTED_EDGE('',*,*,#6697,.T.);
#9439=ORIENTED_EDGE('',*,*,#6061,.F.);
#9440=ORIENTED_EDGE('',*,*,#6707,.F.);
#9441=ORIENTED_EDGE('',*,*,#6080,.F.);
#9442=ORIENTED_EDGE('',*,*,#6698,.T.);
#9443=ORIENTED_EDGE('',*,*,#5869,.F.);
#9444=ORIENTED_EDGE('',*,*,#6708,.F.);
#9445=ORIENTED_EDGE('',*,*,#5849,.F.);
#9446=ORIENTED_EDGE('',*,*,#5436,.T.);
#9447=ORIENTED_EDGE('',*,*,#5853,.F.);
#9448=ORIENTED_EDGE('',*,*,#6709,.F.);
#9449=ORIENTED_EDGE('',*,*,#5979,.F.);
#9450=ORIENTED_EDGE('',*,*,#6699,.T.);
#9451=ORIENTED_EDGE('',*,*,#5982,.F.);
#9452=ORIENTED_EDGE('',*,*,#6710,.F.);
#9453=ORIENTED_EDGE('',*,*,#5837,.F.);
#9454=ORIENTED_EDGE('',*,*,#6700,.T.);
#9455=ORIENTED_EDGE('',*,*,#5841,.F.);
#9456=ORIENTED_EDGE('',*,*,#6711,.F.);
#9457=ORIENTED_EDGE('',*,*,#5897,.F.);
#9458=ORIENTED_EDGE('',*,*,#6712,.F.);
#9459=ORIENTED_EDGE('',*,*,#5715,.F.);
#9460=ORIENTED_EDGE('',*,*,#6701,.T.);
#9461=ORIENTED_EDGE('',*,*,#6088,.F.);
#9462=ORIENTED_EDGE('',*,*,#6702,.T.);
#9463=ORIENTED_EDGE('',*,*,#5714,.F.);
#9464=ORIENTED_EDGE('',*,*,#6713,.F.);
#9465=ORIENTED_EDGE('',*,*,#6060,.F.);
#9466=ORIENTED_EDGE('',*,*,#6704,.T.);
#9467=ORIENTED_EDGE('',*,*,#6055,.F.);
#9468=ORIENTED_EDGE('',*,*,#6714,.F.);
#9469=ORIENTED_EDGE('',*,*,#6223,.F.);
#9470=ORIENTED_EDGE('',*,*,#6703,.T.);
#9471=ORIENTED_EDGE('',*,*,#6222,.F.);
#9472=ORIENTED_EDGE('',*,*,#6715,.F.);
#9473=ORIENTED_EDGE('',*,*,#6053,.F.);
#9474=ORIENTED_EDGE('',*,*,#6705,.T.);
#9475=ORIENTED_EDGE('',*,*,#6054,.F.);
#9476=ORIENTED_EDGE('',*,*,#6716,.F.);
#9477=ORIENTED_EDGE('',*,*,#5526,.F.);
#9478=ORIENTED_EDGE('',*,*,#6707,.T.);
#9479=ORIENTED_EDGE('',*,*,#6706,.T.);
#9480=ORIENTED_EDGE('',*,*,#6717,.F.);
#9481=ORIENTED_EDGE('',*,*,#6081,.T.);
#9482=ORIENTED_EDGE('',*,*,#6708,.T.);
#9483=ORIENTED_EDGE('',*,*,#5880,.F.);
#9484=ORIENTED_EDGE('',*,*,#6718,.F.);
#9485=ORIENTED_EDGE('',*,*,#5850,.F.);
#9486=ORIENTED_EDGE('',*,*,#6719,.F.);
#9487=ORIENTED_EDGE('',*,*,#6709,.T.);
#9488=ORIENTED_EDGE('',*,*,#6720,.F.);
#9489=ORIENTED_EDGE('',*,*,#6721,.F.);
#9490=ORIENTED_EDGE('',*,*,#6710,.T.);
#9491=ORIENTED_EDGE('',*,*,#6722,.F.);
#9492=ORIENTED_EDGE('',*,*,#5890,.T.);
#9493=ORIENTED_EDGE('',*,*,#6711,.T.);
#9494=ORIENTED_EDGE('',*,*,#6723,.F.);
#9495=ORIENTED_EDGE('',*,*,#6724,.F.);
#9496=ORIENTED_EDGE('',*,*,#5727,.T.);
#9497=ORIENTED_EDGE('',*,*,#6204,.F.);
#9498=ORIENTED_EDGE('',*,*,#6725,.F.);
#9499=ORIENTED_EDGE('',*,*,#5709,.F.);
#9500=ORIENTED_EDGE('',*,*,#6714,.T.);
#9501=ORIENTED_EDGE('',*,*,#6713,.T.);
#9502=ORIENTED_EDGE('',*,*,#6726,.F.);
#9503=ORIENTED_EDGE('',*,*,#6716,.T.);
#9504=ORIENTED_EDGE('',*,*,#6715,.T.);
#9505=ORIENTED_EDGE('',*,*,#6727,.F.);
#9506=ORIENTED_EDGE('',*,*,#6717,.T.);
#9507=ORIENTED_EDGE('',*,*,#5530,.F.);
#9508=ORIENTED_EDGE('',*,*,#5529,.F.);
#9509=ORIENTED_EDGE('',*,*,#6728,.F.);
#9510=ORIENTED_EDGE('',*,*,#6082,.F.);
#9511=ORIENTED_EDGE('',*,*,#6718,.T.);
#9512=ORIENTED_EDGE('',*,*,#5877,.F.);
#9513=ORIENTED_EDGE('',*,*,#6729,.F.);
#9514=ORIENTED_EDGE('',*,*,#5851,.F.);
#9515=ORIENTED_EDGE('',*,*,#6720,.T.);
#9516=ORIENTED_EDGE('',*,*,#5852,.F.);
#9517=ORIENTED_EDGE('',*,*,#6730,.F.);
#9518=ORIENTED_EDGE('',*,*,#5828,.F.);
#9519=ORIENTED_EDGE('',*,*,#6719,.T.);
#9520=ORIENTED_EDGE('',*,*,#5827,.F.);
#9521=ORIENTED_EDGE('',*,*,#6731,.F.);
#9522=ORIENTED_EDGE('',*,*,#5980,.F.);
#9523=ORIENTED_EDGE('',*,*,#6722,.T.);
#9524=ORIENTED_EDGE('',*,*,#5981,.F.);
#9525=ORIENTED_EDGE('',*,*,#6732,.F.);
#9526=ORIENTED_EDGE('',*,*,#5833,.F.);
#9527=ORIENTED_EDGE('',*,*,#6721,.T.);
#9528=ORIENTED_EDGE('',*,*,#5832,.F.);
#9529=ORIENTED_EDGE('',*,*,#6733,.F.);
#9530=ORIENTED_EDGE('',*,*,#5838,.F.);
#9531=ORIENTED_EDGE('',*,*,#6734,.F.);
#9532=ORIENTED_EDGE('',*,*,#5839,.F.);
#9533=ORIENTED_EDGE('',*,*,#6735,.F.);
#9534=ORIENTED_EDGE('',*,*,#6317,.F.);
#9535=ORIENTED_EDGE('',*,*,#6723,.T.);
#9536=ORIENTED_EDGE('',*,*,#5840,.F.);
#9537=ORIENTED_EDGE('',*,*,#6736,.F.);
#9538=ORIENTED_EDGE('',*,*,#6302,.F.);
#9539=ORIENTED_EDGE('',*,*,#6724,.T.);
#9540=ORIENTED_EDGE('',*,*,#6301,.F.);
#9541=ORIENTED_EDGE('',*,*,#6737,.F.);
#9542=ORIENTED_EDGE('',*,*,#5891,.F.);
#9543=ORIENTED_EDGE('',*,*,#6725,.T.);
#9544=ORIENTED_EDGE('',*,*,#6201,.F.);
#9545=ORIENTED_EDGE('',*,*,#6738,.F.);
#9546=ORIENTED_EDGE('',*,*,#5710,.F.);
#9547=ORIENTED_EDGE('',*,*,#6726,.T.);
#9548=ORIENTED_EDGE('',*,*,#5713,.F.);
#9549=ORIENTED_EDGE('',*,*,#5434,.F.);
#9550=ORIENTED_EDGE('',*,*,#6224,.F.);
#9551=ORIENTED_EDGE('',*,*,#6727,.T.);
#9552=ORIENTED_EDGE('',*,*,#6221,.F.);
#9553=ORIENTED_EDGE('',*,*,#6739,.F.);
#9554=ORIENTED_EDGE('',*,*,#5527,.F.);
#9555=ORIENTED_EDGE('',*,*,#6740,.F.);
#9556=ORIENTED_EDGE('',*,*,#5528,.F.);
#9557=ORIENTED_EDGE('',*,*,#6741,.F.);
#9558=ORIENTED_EDGE('',*,*,#5696,.F.);
#9559=ORIENTED_EDGE('',*,*,#6728,.T.);
#9560=ORIENTED_EDGE('',*,*,#6740,.T.);
#9561=ORIENTED_EDGE('',*,*,#6742,.F.);
#9562=ORIENTED_EDGE('',*,*,#6083,.T.);
#9563=ORIENTED_EDGE('',*,*,#6729,.T.);
#9564=ORIENTED_EDGE('',*,*,#5876,.T.);
#9565=ORIENTED_EDGE('',*,*,#6743,.F.);
#9566=ORIENTED_EDGE('',*,*,#6730,.T.);
#9567=ORIENTED_EDGE('',*,*,#6732,.T.);
#9568=ORIENTED_EDGE('',*,*,#6731,.T.);
#9569=ORIENTED_EDGE('',*,*,#6744,.F.);
#9570=ORIENTED_EDGE('',*,*,#6735,.T.);
#9571=ORIENTED_EDGE('',*,*,#6733,.T.);
#9572=ORIENTED_EDGE('',*,*,#6745,.F.);
#9573=ORIENTED_EDGE('',*,*,#6736,.T.);
#9574=ORIENTED_EDGE('',*,*,#6734,.T.);
#9575=ORIENTED_EDGE('',*,*,#6746,.F.);
#9576=ORIENTED_EDGE('',*,*,#6737,.T.);
#9577=ORIENTED_EDGE('',*,*,#6300,.F.);
#9578=ORIENTED_EDGE('',*,*,#6747,.F.);
#9579=ORIENTED_EDGE('',*,*,#6308,.F.);
#9580=ORIENTED_EDGE('',*,*,#6738,.T.);
#9581=ORIENTED_EDGE('',*,*,#6200,.T.);
#9582=ORIENTED_EDGE('',*,*,#6748,.F.);
#9583=ORIENTED_EDGE('',*,*,#6749,.F.);
#9584=ORIENTED_EDGE('',*,*,#6741,.T.);
#9585=ORIENTED_EDGE('',*,*,#6739,.T.);
#9586=ORIENTED_EDGE('',*,*,#6750,.F.);
#9587=ORIENTED_EDGE('',*,*,#6751,.F.);
#9588=ORIENTED_EDGE('',*,*,#6076,.F.);
#9589=ORIENTED_EDGE('',*,*,#6742,.T.);
#9590=ORIENTED_EDGE('',*,*,#5695,.F.);
#9591=ORIENTED_EDGE('',*,*,#6743,.T.);
#9592=ORIENTED_EDGE('',*,*,#5875,.F.);
#9593=ORIENTED_EDGE('',*,*,#6752,.F.);
#9594=ORIENTED_EDGE('',*,*,#5829,.F.);
#9595=ORIENTED_EDGE('',*,*,#6744,.T.);
#9596=ORIENTED_EDGE('',*,*,#5826,.F.);
#9597=ORIENTED_EDGE('',*,*,#6753,.F.);
#9598=ORIENTED_EDGE('',*,*,#5834,.F.);
#9599=ORIENTED_EDGE('',*,*,#6745,.T.);
#9600=ORIENTED_EDGE('',*,*,#5831,.F.);
#9601=ORIENTED_EDGE('',*,*,#6754,.F.);
#9602=ORIENTED_EDGE('',*,*,#6318,.F.);
#9603=ORIENTED_EDGE('',*,*,#6746,.T.);
#9604=ORIENTED_EDGE('',*,*,#6316,.F.);
#9605=ORIENTED_EDGE('',*,*,#5428,.F.);
#9606=ORIENTED_EDGE('',*,*,#6303,.F.);
#9607=ORIENTED_EDGE('',*,*,#6747,.T.);
#9608=ORIENTED_EDGE('',*,*,#6299,.F.);
#9609=ORIENTED_EDGE('',*,*,#6755,.F.);
#9610=ORIENTED_EDGE('',*,*,#6197,.F.);
#9611=ORIENTED_EDGE('',*,*,#6748,.T.);
#9612=ORIENTED_EDGE('',*,*,#6199,.F.);
#9613=ORIENTED_EDGE('',*,*,#6756,.F.);
#9614=ORIENTED_EDGE('',*,*,#6184,.F.);
#9615=ORIENTED_EDGE('',*,*,#6749,.T.);
#9616=ORIENTED_EDGE('',*,*,#6183,.F.);
#9617=ORIENTED_EDGE('',*,*,#6757,.F.);
#9618=ORIENTED_EDGE('',*,*,#5711,.F.);
#9619=ORIENTED_EDGE('',*,*,#5432,.T.);
#9620=ORIENTED_EDGE('',*,*,#5712,.F.);
#9621=ORIENTED_EDGE('',*,*,#6758,.F.);
#9622=ORIENTED_EDGE('',*,*,#6217,.F.);
#9623=ORIENTED_EDGE('',*,*,#6750,.T.);
#9624=ORIENTED_EDGE('',*,*,#6220,.F.);
#9625=ORIENTED_EDGE('',*,*,#6759,.F.);
#9626=ORIENTED_EDGE('',*,*,#5697,.F.);
#9627=ORIENTED_EDGE('',*,*,#5729,.T.);
#9628=ORIENTED_EDGE('',*,*,#5702,.F.);
#9629=ORIENTED_EDGE('',*,*,#6760,.F.);
#9630=ORIENTED_EDGE('',*,*,#6194,.F.);
#9631=ORIENTED_EDGE('',*,*,#6752,.T.);
#9632=ORIENTED_EDGE('',*,*,#5874,.T.);
#9633=ORIENTED_EDGE('',*,*,#6761,.F.);
#9634=ORIENTED_EDGE('',*,*,#6762,.F.);
#9635=ORIENTED_EDGE('',*,*,#6754,.T.);
#9636=ORIENTED_EDGE('',*,*,#6753,.T.);
#9637=ORIENTED_EDGE('',*,*,#6763,.F.);
#9638=ORIENTED_EDGE('',*,*,#6198,.T.);
#9639=ORIENTED_EDGE('',*,*,#6755,.T.);
#9640=ORIENTED_EDGE('',*,*,#6764,.F.);
#9641=ORIENTED_EDGE('',*,*,#6756,.T.);
#9642=ORIENTED_EDGE('',*,*,#6758,.T.);
#9643=ORIENTED_EDGE('',*,*,#6757,.T.);
#9644=ORIENTED_EDGE('',*,*,#6765,.F.);
#9645=ORIENTED_EDGE('',*,*,#6759,.T.);
#9646=ORIENTED_EDGE('',*,*,#5516,.F.);
#9647=ORIENTED_EDGE('',*,*,#6766,.F.);
#9648=ORIENTED_EDGE('',*,*,#5698,.F.);
#9649=ORIENTED_EDGE('',*,*,#6760,.T.);
#9650=ORIENTED_EDGE('',*,*,#5701,.F.);
#9651=ORIENTED_EDGE('',*,*,#6767,.F.);
#9652=ORIENTED_EDGE('',*,*,#6191,.F.);
#9653=ORIENTED_EDGE('',*,*,#6761,.T.);
#9654=ORIENTED_EDGE('',*,*,#5873,.F.);
#9655=ORIENTED_EDGE('',*,*,#6768,.F.);
#9656=ORIENTED_EDGE('',*,*,#6291,.F.);
#9657=ORIENTED_EDGE('',*,*,#6762,.T.);
#9658=ORIENTED_EDGE('',*,*,#6298,.F.);
#9659=ORIENTED_EDGE('',*,*,#6769,.F.);
#9660=ORIENTED_EDGE('',*,*,#5830,.F.);
#9661=ORIENTED_EDGE('',*,*,#6763,.T.);
#9662=ORIENTED_EDGE('',*,*,#5825,.F.);
#9663=ORIENTED_EDGE('',*,*,#6770,.F.);
#9664=ORIENTED_EDGE('',*,*,#6314,.F.);
#9665=ORIENTED_EDGE('',*,*,#5430,.T.);
#9666=ORIENTED_EDGE('',*,*,#6323,.F.);
#9667=ORIENTED_EDGE('',*,*,#6771,.F.);
#9668=ORIENTED_EDGE('',*,*,#6304,.F.);
#9669=ORIENTED_EDGE('',*,*,#6764,.T.);
#9670=ORIENTED_EDGE('',*,*,#6305,.F.);
#9671=ORIENTED_EDGE('',*,*,#6772,.F.);
#9672=ORIENTED_EDGE('',*,*,#6185,.F.);
#9673=ORIENTED_EDGE('',*,*,#6765,.T.);
#9674=ORIENTED_EDGE('',*,*,#6182,.F.);
#9675=ORIENTED_EDGE('',*,*,#6773,.F.);
#9676=ORIENTED_EDGE('',*,*,#6218,.F.);
#9677=ORIENTED_EDGE('',*,*,#6766,.T.);
#9678=ORIENTED_EDGE('',*,*,#6216,.F.);
#9679=ORIENTED_EDGE('',*,*,#6774,.F.);
#9680=ORIENTED_EDGE('',*,*,#5699,.F.);
#9681=ORIENTED_EDGE('',*,*,#6775,.F.);
#9682=ORIENTED_EDGE('',*,*,#5700,.F.);
#9683=ORIENTED_EDGE('',*,*,#6776,.F.);
#9684=ORIENTED_EDGE('',*,*,#5513,.F.);
#9685=ORIENTED_EDGE('',*,*,#6767,.T.);
#9686=ORIENTED_EDGE('',*,*,#6775,.T.);
#9687=ORIENTED_EDGE('',*,*,#6777,.F.);
#9688=ORIENTED_EDGE('',*,*,#6192,.T.);
#9689=ORIENTED_EDGE('',*,*,#6768,.T.);
#9690=ORIENTED_EDGE('',*,*,#6306,.F.);
#9691=ORIENTED_EDGE('',*,*,#6778,.F.);
#9692=ORIENTED_EDGE('',*,*,#6292,.F.);
#9693=ORIENTED_EDGE('',*,*,#6770,.T.);
#9694=ORIENTED_EDGE('',*,*,#6769,.T.);
#9695=ORIENTED_EDGE('',*,*,#6779,.F.);
#9696=ORIENTED_EDGE('',*,*,#6772,.T.);
#9697=ORIENTED_EDGE('',*,*,#6771,.T.);
#9698=ORIENTED_EDGE('',*,*,#6780,.F.);
#9699=ORIENTED_EDGE('',*,*,#6781,.F.);
#9700=ORIENTED_EDGE('',*,*,#6773,.T.);
#9701=ORIENTED_EDGE('',*,*,#5426,.F.);
#9702=ORIENTED_EDGE('',*,*,#6776,.T.);
#9703=ORIENTED_EDGE('',*,*,#6774,.T.);
#9704=ORIENTED_EDGE('',*,*,#6782,.F.);
#9705=ORIENTED_EDGE('',*,*,#6777,.T.);
#9706=ORIENTED_EDGE('',*,*,#5512,.F.);
#9707=ORIENTED_EDGE('',*,*,#5511,.F.);
#9708=ORIENTED_EDGE('',*,*,#6783,.F.);
#9709=ORIENTED_EDGE('',*,*,#6193,.F.);
#9710=ORIENTED_EDGE('',*,*,#6778,.T.);
#9711=ORIENTED_EDGE('',*,*,#6187,.F.);
#9712=ORIENTED_EDGE('',*,*,#6784,.F.);
#9713=ORIENTED_EDGE('',*,*,#6293,.F.);
#9714=ORIENTED_EDGE('',*,*,#6779,.T.);
#9715=ORIENTED_EDGE('',*,*,#6297,.F.);
#9716=ORIENTED_EDGE('',*,*,#6785,.F.);
#9717=ORIENTED_EDGE('',*,*,#6315,.F.);
#9718=ORIENTED_EDGE('',*,*,#6780,.T.);
#9719=ORIENTED_EDGE('',*,*,#6322,.F.);
#9720=ORIENTED_EDGE('',*,*,#6786,.F.);
#9721=ORIENTED_EDGE('',*,*,#6181,.F.);
#9722=ORIENTED_EDGE('',*,*,#6781,.T.);
#9723=ORIENTED_EDGE('',*,*,#6179,.F.);
#9724=ORIENTED_EDGE('',*,*,#6787,.F.);
#9725=ORIENTED_EDGE('',*,*,#6219,.F.);
#9726=ORIENTED_EDGE('',*,*,#6782,.T.);
#9727=ORIENTED_EDGE('',*,*,#6215,.F.);
#9728=ORIENTED_EDGE('',*,*,#6788,.F.);
#9729=ORIENTED_EDGE('',*,*,#5514,.F.);
#9730=ORIENTED_EDGE('',*,*,#6186,.T.);
#9731=ORIENTED_EDGE('',*,*,#6783,.T.);
#9732=ORIENTED_EDGE('',*,*,#6789,.F.);
#9733=ORIENTED_EDGE('',*,*,#6784,.T.);
#9734=ORIENTED_EDGE('',*,*,#6785,.T.);
#9735=ORIENTED_EDGE('',*,*,#6296,.F.);
#9736=ORIENTED_EDGE('',*,*,#6790,.F.);
#9737=ORIENTED_EDGE('',*,*,#5497,.F.);
#9738=ORIENTED_EDGE('',*,*,#5424,.T.);
#9739=ORIENTED_EDGE('',*,*,#6786,.T.);
#9740=ORIENTED_EDGE('',*,*,#6791,.F.);
#9741=ORIENTED_EDGE('',*,*,#6788,.T.);
#9742=ORIENTED_EDGE('',*,*,#6787,.T.);
#9743=ORIENTED_EDGE('',*,*,#5422,.F.);
#9744=ORIENTED_EDGE('',*,*,#6789,.T.);
#9745=ORIENTED_EDGE('',*,*,#5510,.F.);
#9746=ORIENTED_EDGE('',*,*,#6792,.F.);
#9747=ORIENTED_EDGE('',*,*,#6294,.F.);
#9748=ORIENTED_EDGE('',*,*,#6790,.T.);
#9749=ORIENTED_EDGE('',*,*,#6295,.F.);
#9750=ORIENTED_EDGE('',*,*,#6793,.F.);
#9751=ORIENTED_EDGE('',*,*,#6319,.F.);
#9752=ORIENTED_EDGE('',*,*,#6791,.T.);
#9753=ORIENTED_EDGE('',*,*,#6321,.F.);
#9754=ORIENTED_EDGE('',*,*,#6794,.F.);
#9755=ORIENTED_EDGE('',*,*,#6180,.F.);
#9756=ORIENTED_EDGE('',*,*,#6793,.T.);
#9757=ORIENTED_EDGE('',*,*,#6792,.T.);
#9758=ORIENTED_EDGE('',*,*,#6795,.F.);
#9759=ORIENTED_EDGE('',*,*,#5420,.T.);
#9760=ORIENTED_EDGE('',*,*,#6794,.T.);
#9761=ORIENTED_EDGE('',*,*,#6796,.F.);
#9762=ORIENTED_EDGE('',*,*,#6795,.T.);
#9763=ORIENTED_EDGE('',*,*,#5509,.F.);
#9764=ORIENTED_EDGE('',*,*,#6796,.T.);
#9765=ORIENTED_EDGE('',*,*,#6320,.F.);
#9766=ORIENTED_EDGE('',*,*,#6797,.F.);
#9767=ORIENTED_EDGE('',*,*,#6214,.T.);
#9768=ORIENTED_EDGE('',*,*,#6798,.T.);
#9769=ORIENTED_EDGE('',*,*,#6799,.T.);
#9770=ORIENTED_EDGE('',*,*,#6799,.F.);
#9771=ORIENTED_EDGE('',*,*,#6800,.T.);
#9772=ORIENTED_EDGE('',*,*,#6801,.T.);
#9773=ORIENTED_EDGE('',*,*,#6802,.T.);
#9774=ORIENTED_EDGE('',*,*,#6802,.F.);
#9775=ORIENTED_EDGE('',*,*,#6803,.T.);
#9776=ORIENTED_EDGE('',*,*,#5603,.T.);
#9777=ORIENTED_EDGE('',*,*,#6804,.T.);
#9778=ORIENTED_EDGE('',*,*,#6804,.F.);
#9779=ORIENTED_EDGE('',*,*,#5545,.T.);
#9780=ORIENTED_EDGE('',*,*,#6805,.T.);
#9781=ORIENTED_EDGE('',*,*,#6806,.T.);
#9782=ORIENTED_EDGE('',*,*,#6806,.F.);
#9783=ORIENTED_EDGE('',*,*,#6807,.T.);
#9784=ORIENTED_EDGE('',*,*,#6808,.F.);
#9785=ORIENTED_EDGE('',*,*,#6809,.T.);
#9786=ORIENTED_EDGE('',*,*,#6810,.F.);
#9787=ORIENTED_EDGE('',*,*,#6811,.T.);
#9788=ORIENTED_EDGE('',*,*,#6100,.T.);
#9789=ORIENTED_EDGE('',*,*,#6812,.T.);
#9790=ORIENTED_EDGE('',*,*,#6812,.F.);
#9791=ORIENTED_EDGE('',*,*,#6104,.T.);
#9792=ORIENTED_EDGE('',*,*,#6813,.T.);
#9793=ORIENTED_EDGE('',*,*,#6814,.T.);
#9794=ORIENTED_EDGE('',*,*,#6814,.F.);
#9795=ORIENTED_EDGE('',*,*,#6815,.T.);
#9796=ORIENTED_EDGE('',*,*,#6816,.T.);
#9797=ORIENTED_EDGE('',*,*,#6817,.T.);
#9798=ORIENTED_EDGE('',*,*,#6817,.F.);
#9799=ORIENTED_EDGE('',*,*,#6818,.T.);
#9800=ORIENTED_EDGE('',*,*,#5606,.T.);
#9801=ORIENTED_EDGE('',*,*,#6819,.T.);
#9802=ORIENTED_EDGE('',*,*,#6819,.F.);
#9803=ORIENTED_EDGE('',*,*,#5605,.T.);
#9804=ORIENTED_EDGE('',*,*,#6820,.F.);
#9805=ORIENTED_EDGE('',*,*,#6821,.T.);
#9806=ORIENTED_EDGE('',*,*,#6822,.F.);
#9807=ORIENTED_EDGE('',*,*,#5542,.T.);
#9808=ORIENTED_EDGE('',*,*,#6823,.T.);
#9809=ORIENTED_EDGE('',*,*,#6824,.T.);
#9810=ORIENTED_EDGE('',*,*,#6824,.F.);
#9811=ORIENTED_EDGE('',*,*,#6825,.T.);
#9812=ORIENTED_EDGE('',*,*,#6826,.T.);
#9813=ORIENTED_EDGE('',*,*,#6827,.T.);
#9814=ORIENTED_EDGE('',*,*,#6827,.F.);
#9815=ORIENTED_EDGE('',*,*,#6828,.T.);
#9816=ORIENTED_EDGE('',*,*,#5764,.T.);
#9817=ORIENTED_EDGE('',*,*,#6829,.T.);
#9818=ORIENTED_EDGE('',*,*,#6829,.F.);
#9819=ORIENTED_EDGE('',*,*,#5763,.T.);
#9820=ORIENTED_EDGE('',*,*,#6830,.T.);
#9821=ORIENTED_EDGE('',*,*,#6831,.T.);
#9822=ORIENTED_EDGE('',*,*,#6831,.F.);
#9823=ORIENTED_EDGE('',*,*,#6832,.T.);
#9824=ORIENTED_EDGE('',*,*,#6833,.F.);
#9825=ORIENTED_EDGE('',*,*,#6834,.T.);
#9826=ORIENTED_EDGE('',*,*,#6835,.F.);
#9827=ORIENTED_EDGE('',*,*,#6836,.T.);
#9828=ORIENTED_EDGE('',*,*,#5965,.T.);
#9829=ORIENTED_EDGE('',*,*,#6837,.T.);
#9830=ORIENTED_EDGE('',*,*,#6837,.F.);
#9831=ORIENTED_EDGE('',*,*,#5969,.T.);
#9832=ORIENTED_EDGE('',*,*,#6838,.T.);
#9833=ORIENTED_EDGE('',*,*,#6839,.T.);
#9834=ORIENTED_EDGE('',*,*,#6839,.F.);
#9835=ORIENTED_EDGE('',*,*,#6840,.T.);
#9836=ORIENTED_EDGE('',*,*,#6841,.F.);
#9837=ORIENTED_EDGE('',*,*,#6842,.T.);
#9838=ORIENTED_EDGE('',*,*,#6842,.F.);
#9839=ORIENTED_EDGE('',*,*,#6843,.F.);
#9840=ORIENTED_EDGE('',*,*,#5540,.T.);
#9841=ORIENTED_EDGE('',*,*,#6844,.T.);
#9842=ORIENTED_EDGE('',*,*,#6844,.F.);
#9843=ORIENTED_EDGE('',*,*,#5608,.T.);
#9844=ORIENTED_EDGE('',*,*,#6845,.F.);
#9845=ORIENTED_EDGE('',*,*,#6846,.T.);
#9846=ORIENTED_EDGE('',*,*,#6847,.F.);
#9847=ORIENTED_EDGE('',*,*,#5676,.F.);
#9848=ORIENTED_EDGE('',*,*,#6848,.F.);
#9849=ORIENTED_EDGE('',*,*,#5967,.F.);
#9850=ORIENTED_EDGE('',*,*,#5677,.T.);
#9851=ORIENTED_EDGE('',*,*,#6847,.T.);
#9852=ORIENTED_EDGE('',*,*,#6849,.F.);
#9853=ORIENTED_EDGE('',*,*,#6850,.F.);
#9854=ORIENTED_EDGE('',*,*,#6851,.F.);
#9855=ORIENTED_EDGE('',*,*,#6852,.F.);
#9856=ORIENTED_EDGE('',*,*,#6848,.T.);
#9857=ORIENTED_EDGE('',*,*,#5675,.T.);
#9858=ORIENTED_EDGE('',*,*,#6852,.T.);
#9859=ORIENTED_EDGE('',*,*,#5963,.F.);
#9860=ORIENTED_EDGE('',*,*,#6840,.F.);
#9861=ORIENTED_EDGE('',*,*,#6838,.F.);
#9862=ORIENTED_EDGE('',*,*,#5968,.F.);
#9863=ORIENTED_EDGE('',*,*,#6849,.T.);
#9864=ORIENTED_EDGE('',*,*,#5966,.F.);
#9865=ORIENTED_EDGE('',*,*,#6836,.F.);
#9866=ORIENTED_EDGE('',*,*,#6853,.F.);
#9867=ORIENTED_EDGE('',*,*,#6096,.F.);
#9868=ORIENTED_EDGE('',*,*,#6850,.T.);
#9869=ORIENTED_EDGE('',*,*,#6099,.F.);
#9870=ORIENTED_EDGE('',*,*,#6854,.F.);
#9871=ORIENTED_EDGE('',*,*,#5678,.F.);
#9872=ORIENTED_EDGE('',*,*,#6855,.F.);
#9873=ORIENTED_EDGE('',*,*,#5680,.F.);
#9874=ORIENTED_EDGE('',*,*,#6856,.F.);
#9875=ORIENTED_EDGE('',*,*,#6102,.F.);
#9876=ORIENTED_EDGE('',*,*,#6851,.T.);
#9877=ORIENTED_EDGE('',*,*,#5674,.F.);
#9878=ORIENTED_EDGE('',*,*,#6857,.F.);
#9879=ORIENTED_EDGE('',*,*,#5964,.F.);
#9880=ORIENTED_EDGE('',*,*,#6853,.T.);
#9881=ORIENTED_EDGE('',*,*,#6835,.T.);
#9882=ORIENTED_EDGE('',*,*,#6846,.F.);
#9883=ORIENTED_EDGE('',*,*,#6858,.F.);
#9884=ORIENTED_EDGE('',*,*,#5679,.T.);
#9885=ORIENTED_EDGE('',*,*,#6854,.T.);
#9886=ORIENTED_EDGE('',*,*,#6859,.F.);
#9887=ORIENTED_EDGE('',*,*,#6856,.T.);
#9888=ORIENTED_EDGE('',*,*,#5665,.T.);
#9889=ORIENTED_EDGE('',*,*,#6855,.T.);
#9890=ORIENTED_EDGE('',*,*,#6860,.F.);
#9891=ORIENTED_EDGE('',*,*,#6861,.F.);
#9892=ORIENTED_EDGE('',*,*,#6862,.F.);
#9893=ORIENTED_EDGE('',*,*,#6863,.F.);
#9894=ORIENTED_EDGE('',*,*,#6857,.T.);
#9895=ORIENTED_EDGE('',*,*,#5673,.T.);
#9896=ORIENTED_EDGE('',*,*,#6863,.T.);
#9897=ORIENTED_EDGE('',*,*,#5765,.F.);
#9898=ORIENTED_EDGE('',*,*,#6828,.F.);
#9899=ORIENTED_EDGE('',*,*,#6826,.F.);
#9900=ORIENTED_EDGE('',*,*,#5961,.F.);
#9901=ORIENTED_EDGE('',*,*,#6841,.T.);
#9902=ORIENTED_EDGE('',*,*,#5962,.F.);
#9903=ORIENTED_EDGE('',*,*,#6825,.F.);
#9904=ORIENTED_EDGE('',*,*,#6823,.F.);
#9905=ORIENTED_EDGE('',*,*,#5541,.F.);
#9906=ORIENTED_EDGE('',*,*,#6843,.T.);
#9907=ORIENTED_EDGE('',*,*,#6845,.T.);
#9908=ORIENTED_EDGE('',*,*,#5607,.F.);
#9909=ORIENTED_EDGE('',*,*,#6818,.F.);
#9910=ORIENTED_EDGE('',*,*,#6816,.F.);
#9911=ORIENTED_EDGE('',*,*,#6097,.F.);
#9912=ORIENTED_EDGE('',*,*,#6858,.T.);
#9913=ORIENTED_EDGE('',*,*,#6859,.T.);
#9914=ORIENTED_EDGE('',*,*,#6098,.F.);
#9915=ORIENTED_EDGE('',*,*,#6815,.F.);
#9916=ORIENTED_EDGE('',*,*,#6813,.F.);
#9917=ORIENTED_EDGE('',*,*,#6103,.F.);
#9918=ORIENTED_EDGE('',*,*,#6860,.T.);
#9919=ORIENTED_EDGE('',*,*,#6101,.F.);
#9920=ORIENTED_EDGE('',*,*,#6811,.F.);
#9921=ORIENTED_EDGE('',*,*,#6864,.F.);
#9922=ORIENTED_EDGE('',*,*,#6206,.F.);
#9923=ORIENTED_EDGE('',*,*,#6861,.T.);
#9924=ORIENTED_EDGE('',*,*,#6209,.F.);
#9925=ORIENTED_EDGE('',*,*,#6865,.F.);
#9926=ORIENTED_EDGE('',*,*,#5666,.F.);
#9927=ORIENTED_EDGE('',*,*,#6862,.T.);
#9928=ORIENTED_EDGE('',*,*,#5672,.F.);
#9929=ORIENTED_EDGE('',*,*,#6866,.F.);
#9930=ORIENTED_EDGE('',*,*,#5766,.F.);
#9931=ORIENTED_EDGE('',*,*,#6832,.F.);
#9932=ORIENTED_EDGE('',*,*,#6830,.F.);
#9933=ORIENTED_EDGE('',*,*,#5767,.F.);
#9934=ORIENTED_EDGE('',*,*,#6867,.F.);
#9935=ORIENTED_EDGE('',*,*,#6312,.F.);
#9936=ORIENTED_EDGE('',*,*,#5543,.T.);
#9937=ORIENTED_EDGE('',*,*,#6822,.T.);
#9938=ORIENTED_EDGE('',*,*,#6834,.F.);
#9939=ORIENTED_EDGE('',*,*,#6868,.F.);
#9940=ORIENTED_EDGE('',*,*,#6864,.T.);
#9941=ORIENTED_EDGE('',*,*,#6810,.T.);
#9942=ORIENTED_EDGE('',*,*,#6821,.F.);
#9943=ORIENTED_EDGE('',*,*,#6869,.F.);
#9944=ORIENTED_EDGE('',*,*,#5667,.T.);
#9945=ORIENTED_EDGE('',*,*,#6865,.T.);
#9946=ORIENTED_EDGE('',*,*,#6870,.F.);
#9947=ORIENTED_EDGE('',*,*,#6871,.F.);
#9948=ORIENTED_EDGE('',*,*,#6866,.T.);
#9949=ORIENTED_EDGE('',*,*,#5671,.T.);
#9950=ORIENTED_EDGE('',*,*,#6872,.F.);
#9951=ORIENTED_EDGE('',*,*,#6867,.T.);
#9952=ORIENTED_EDGE('',*,*,#6833,.T.);
#9953=ORIENTED_EDGE('',*,*,#6311,.F.);
#9954=ORIENTED_EDGE('',*,*,#6807,.F.);
#9955=ORIENTED_EDGE('',*,*,#6805,.F.);
#9956=ORIENTED_EDGE('',*,*,#5544,.F.);
#9957=ORIENTED_EDGE('',*,*,#6868,.T.);
#9958=ORIENTED_EDGE('',*,*,#6820,.T.);
#9959=ORIENTED_EDGE('',*,*,#5604,.F.);
#9960=ORIENTED_EDGE('',*,*,#6803,.F.);
#9961=ORIENTED_EDGE('',*,*,#6801,.F.);
#9962=ORIENTED_EDGE('',*,*,#6207,.F.);
#9963=ORIENTED_EDGE('',*,*,#6869,.T.);
#9964=ORIENTED_EDGE('',*,*,#6870,.T.);
#9965=ORIENTED_EDGE('',*,*,#6208,.F.);
#9966=ORIENTED_EDGE('',*,*,#6800,.F.);
#9967=ORIENTED_EDGE('',*,*,#6798,.F.);
#9968=ORIENTED_EDGE('',*,*,#6213,.F.);
#9969=ORIENTED_EDGE('',*,*,#6871,.T.);
#9970=ORIENTED_EDGE('',*,*,#6212,.F.);
#9971=ORIENTED_EDGE('',*,*,#6873,.F.);
#9972=ORIENTED_EDGE('',*,*,#5668,.F.);
#9973=ORIENTED_EDGE('',*,*,#6872,.T.);
#9974=ORIENTED_EDGE('',*,*,#5670,.F.);
#9975=ORIENTED_EDGE('',*,*,#6874,.F.);
#9976=ORIENTED_EDGE('',*,*,#6313,.F.);
#9977=ORIENTED_EDGE('',*,*,#6210,.T.);
#9978=ORIENTED_EDGE('',*,*,#6797,.T.);
#9979=ORIENTED_EDGE('',*,*,#6809,.F.);
#9980=ORIENTED_EDGE('',*,*,#6875,.F.);
#9981=ORIENTED_EDGE('',*,*,#5669,.T.);
#9982=ORIENTED_EDGE('',*,*,#6873,.T.);
#9983=ORIENTED_EDGE('',*,*,#6876,.F.);
#9984=ORIENTED_EDGE('',*,*,#6874,.T.);
#9985=ORIENTED_EDGE('',*,*,#6808,.T.);
#9986=ORIENTED_EDGE('',*,*,#6310,.F.);
#9987=ORIENTED_EDGE('',*,*,#6876,.T.);
#9988=ORIENTED_EDGE('',*,*,#6211,.F.);
#9989=ORIENTED_EDGE('',*,*,#6875,.T.);
#9990=ORIENTED_EDGE('',*,*,#6877,.F.);
#9991=ORIENTED_EDGE('',*,*,#5926,.F.);
#9992=ORIENTED_EDGE('',*,*,#6878,.F.);
#9993=ORIENTED_EDGE('',*,*,#6085,.F.);
#9994=ORIENTED_EDGE('',*,*,#6878,.T.);
#9995=ORIENTED_EDGE('',*,*,#5925,.F.);
#9996=ORIENTED_EDGE('',*,*,#6879,.F.);
#9997=ORIENTED_EDGE('',*,*,#5867,.F.);
#9998=ORIENTED_EDGE('',*,*,#6880,.F.);
#9999=ORIENTED_EDGE('',*,*,#5898,.F.);
#10000=ORIENTED_EDGE('',*,*,#6877,.T.);
#10001=ORIENTED_EDGE('',*,*,#6078,.F.);
#10002=ORIENTED_EDGE('',*,*,#6879,.T.);
#10003=ORIENTED_EDGE('',*,*,#5924,.F.);
#10004=ORIENTED_EDGE('',*,*,#6881,.F.);
#10005=ORIENTED_EDGE('',*,*,#5881,.F.);
#10006=ORIENTED_EDGE('',*,*,#5732,.T.);
#10007=ORIENTED_EDGE('',*,*,#6195,.F.);
#10008=ORIENTED_EDGE('',*,*,#6882,.F.);
#10009=ORIENTED_EDGE('',*,*,#5920,.F.);
#10010=ORIENTED_EDGE('',*,*,#6881,.T.);
#10011=ORIENTED_EDGE('',*,*,#5923,.F.);
#10012=ORIENTED_EDGE('',*,*,#6883,.F.);
#10013=ORIENTED_EDGE('',*,*,#5879,.F.);
#10014=ORIENTED_EDGE('',*,*,#6882,.T.);
#10015=ORIENTED_EDGE('',*,*,#6189,.F.);
#10016=ORIENTED_EDGE('',*,*,#6884,.F.);
#10017=ORIENTED_EDGE('',*,*,#5921,.F.);
#10018=ORIENTED_EDGE('',*,*,#6883,.T.);
#10019=ORIENTED_EDGE('',*,*,#5922,.F.);
#10020=ORIENTED_EDGE('',*,*,#6884,.T.);
#10021=ORIENTED_EDGE('',*,*,#6307,.F.);
#10022=ORIENTED_EDGE('',*,*,#6885,.F.);
#10023=ORIENTED_EDGE('',*,*,#6095,.F.);
#10024=ORIENTED_EDGE('',*,*,#6886,.F.);
#10025=ORIENTED_EDGE('',*,*,#5639,.F.);
#10026=ORIENTED_EDGE('',*,*,#6886,.T.);
#10027=ORIENTED_EDGE('',*,*,#5889,.F.);
#10028=ORIENTED_EDGE('',*,*,#6887,.F.);
#10029=ORIENTED_EDGE('',*,*,#5640,.F.);
#10030=ORIENTED_EDGE('',*,*,#6888,.F.);
#10031=ORIENTED_EDGE('',*,*,#6086,.F.);
#10032=ORIENTED_EDGE('',*,*,#6885,.T.);
#10033=ORIENTED_EDGE('',*,*,#5638,.F.);
#10034=ORIENTED_EDGE('',*,*,#6887,.T.);
#10035=ORIENTED_EDGE('',*,*,#5960,.F.);
#10036=ORIENTED_EDGE('',*,*,#6889,.F.);
#10037=ORIENTED_EDGE('',*,*,#5641,.F.);
#10038=ORIENTED_EDGE('',*,*,#5734,.T.);
#10039=ORIENTED_EDGE('',*,*,#5645,.F.);
#10040=ORIENTED_EDGE('',*,*,#6890,.F.);
#10041=ORIENTED_EDGE('',*,*,#6205,.F.);
#10042=ORIENTED_EDGE('',*,*,#6889,.T.);
#10043=ORIENTED_EDGE('',*,*,#5893,.F.);
#10044=ORIENTED_EDGE('',*,*,#6891,.F.);
#10045=ORIENTED_EDGE('',*,*,#5642,.F.);
#10046=ORIENTED_EDGE('',*,*,#6890,.T.);
#10047=ORIENTED_EDGE('',*,*,#5644,.F.);
#10048=ORIENTED_EDGE('',*,*,#6892,.F.);
#10049=ORIENTED_EDGE('',*,*,#6203,.F.);
#10050=ORIENTED_EDGE('',*,*,#6891,.T.);
#10051=ORIENTED_EDGE('',*,*,#6309,.F.);
#10052=ORIENTED_EDGE('',*,*,#6892,.T.);
#10053=ORIENTED_EDGE('',*,*,#5643,.F.);
#10054=ORIENTED_EDGE('',*,*,#6893,.F.);
#10055=ORIENTED_EDGE('',*,*,#5629,.F.);
#10056=ORIENTED_EDGE('',*,*,#5402,.F.);
#10057=ORIENTED_EDGE('',*,*,#5505,.F.);
#10058=ORIENTED_EDGE('',*,*,#6893,.T.);
#10059=ORIENTED_EDGE('',*,*,#6264,.F.);
#10060=ORIENTED_EDGE('',*,*,#6894,.F.);
#10061=ORIENTED_EDGE('',*,*,#5630,.F.);
#10062=ORIENTED_EDGE('',*,*,#6895,.F.);
#10063=ORIENTED_EDGE('',*,*,#5635,.F.);
#10064=ORIENTED_EDGE('',*,*,#6896,.F.);
#10065=ORIENTED_EDGE('',*,*,#6246,.F.);
#10066=ORIENTED_EDGE('',*,*,#6894,.T.);
#10067=ORIENTED_EDGE('',*,*,#6248,.F.);
#10068=ORIENTED_EDGE('',*,*,#6897,.F.);
#10069=ORIENTED_EDGE('',*,*,#5631,.F.);
#10070=ORIENTED_EDGE('',*,*,#6896,.T.);
#10071=ORIENTED_EDGE('',*,*,#5634,.F.);
#10072=ORIENTED_EDGE('',*,*,#6898,.F.);
#10073=ORIENTED_EDGE('',*,*,#5501,.F.);
#10074=ORIENTED_EDGE('',*,*,#6897,.T.);
#10075=ORIENTED_EDGE('',*,*,#6262,.F.);
#10076=ORIENTED_EDGE('',*,*,#6899,.F.);
#10077=ORIENTED_EDGE('',*,*,#5632,.F.);
#10078=ORIENTED_EDGE('',*,*,#6898,.T.);
#10079=ORIENTED_EDGE('',*,*,#5633,.F.);
#10080=ORIENTED_EDGE('',*,*,#6899,.T.);
#10081=ORIENTED_EDGE('',*,*,#6241,.F.);
#10082=ORIENTED_EDGE('',*,*,#6900,.F.);
#10083=ORIENTED_EDGE('',*,*,#5503,.F.);
#10084=ORIENTED_EDGE('',*,*,#5396,.F.);
#10085=ORIENTED_EDGE('',*,*,#6258,.F.);
#10086=ORIENTED_EDGE('',*,*,#6900,.T.);
#10087=ORIENTED_EDGE('',*,*,#6257,.F.);
#10088=ORIENTED_EDGE('',*,*,#6901,.F.);
#10089=ORIENTED_EDGE('',*,*,#6263,.F.);
#10090=ORIENTED_EDGE('',*,*,#6252,.F.);
#10091=ORIENTED_EDGE('',*,*,#6902,.T.);
#10092=ORIENTED_EDGE('',*,*,#6244,.F.);
#10093=ORIENTED_EDGE('',*,*,#6903,.F.);
#10094=ORIENTED_EDGE('',*,*,#6901,.T.);
#10095=ORIENTED_EDGE('',*,*,#6256,.F.);
#10096=ORIENTED_EDGE('',*,*,#6904,.F.);
#10097=ORIENTED_EDGE('',*,*,#6250,.F.);
#10098=ORIENTED_EDGE('',*,*,#6903,.T.);
#10099=ORIENTED_EDGE('',*,*,#5499,.F.);
#10100=ORIENTED_EDGE('',*,*,#6905,.F.);
#10101=ORIENTED_EDGE('',*,*,#6253,.F.);
#10102=ORIENTED_EDGE('',*,*,#6904,.T.);
#10103=ORIENTED_EDGE('',*,*,#6255,.F.);
#10104=ORIENTED_EDGE('',*,*,#6906,.F.);
#10105=ORIENTED_EDGE('',*,*,#6261,.F.);
#10106=ORIENTED_EDGE('',*,*,#6905,.T.);
#10107=ORIENTED_EDGE('',*,*,#6243,.F.);
#10108=ORIENTED_EDGE('',*,*,#6906,.T.);
#10109=ORIENTED_EDGE('',*,*,#6254,.F.);
#10110=ORIENTED_EDGE('',*,*,#5381,.T.);
#10111=ORIENTED_EDGE('',*,*,#5656,.F.);
#10112=ORIENTED_EDGE('',*,*,#6907,.F.);
#10113=ORIENTED_EDGE('',*,*,#6148,.F.);
#10114=ORIENTED_EDGE('',*,*,#5379,.T.);
#10115=ORIENTED_EDGE('',*,*,#6150,.F.);
#10116=ORIENTED_EDGE('',*,*,#6908,.F.);
#10117=ORIENTED_EDGE('',*,*,#5657,.F.);
#10118=ORIENTED_EDGE('',*,*,#6907,.T.);
#10119=ORIENTED_EDGE('',*,*,#5655,.F.);
#10120=ORIENTED_EDGE('',*,*,#6909,.F.);
#10121=ORIENTED_EDGE('',*,*,#6135,.F.);
#10122=ORIENTED_EDGE('',*,*,#6908,.T.);
#10123=ORIENTED_EDGE('',*,*,#6138,.F.);
#10124=ORIENTED_EDGE('',*,*,#5375,.F.);
#10125=ORIENTED_EDGE('',*,*,#5658,.F.);
#10126=ORIENTED_EDGE('',*,*,#6909,.T.);
#10127=ORIENTED_EDGE('',*,*,#5654,.F.);
#10128=ORIENTED_EDGE('',*,*,#6910,.F.);
#10129=ORIENTED_EDGE('',*,*,#5520,.F.);
#10130=ORIENTED_EDGE('',*,*,#6910,.T.);
#10131=ORIENTED_EDGE('',*,*,#5653,.F.);
#10132=ORIENTED_EDGE('',*,*,#5377,.T.);
#10133=ORIENTED_EDGE('',*,*,#6131,.F.);
#10134=ORIENTED_EDGE('',*,*,#5371,.T.);
#10135=ORIENTED_EDGE('',*,*,#6147,.F.);
#10136=ORIENTED_EDGE('',*,*,#6911,.F.);
#10137=ORIENTED_EDGE('',*,*,#6141,.F.);
#10138=ORIENTED_EDGE('',*,*,#5373,.T.);
#10139=ORIENTED_EDGE('',*,*,#6146,.F.);
#10140=ORIENTED_EDGE('',*,*,#6912,.F.);
#10141=ORIENTED_EDGE('',*,*,#6149,.F.);
#10142=ORIENTED_EDGE('',*,*,#6911,.T.);
#10143=ORIENTED_EDGE('',*,*,#6136,.F.);
#10144=ORIENTED_EDGE('',*,*,#6913,.F.);
#10145=ORIENTED_EDGE('',*,*,#6142,.F.);
#10146=ORIENTED_EDGE('',*,*,#6912,.T.);
#10147=ORIENTED_EDGE('',*,*,#6145,.F.);
#10148=ORIENTED_EDGE('',*,*,#5369,.F.);
#10149=ORIENTED_EDGE('',*,*,#6140,.F.);
#10150=ORIENTED_EDGE('',*,*,#6913,.T.);
#10151=ORIENTED_EDGE('',*,*,#5518,.F.);
#10152=ORIENTED_EDGE('',*,*,#6914,.F.);
#10153=ORIENTED_EDGE('',*,*,#6143,.F.);
#10154=ORIENTED_EDGE('',*,*,#6914,.T.);
#10155=ORIENTED_EDGE('',*,*,#6133,.F.);
#10156=ORIENTED_EDGE('',*,*,#5367,.T.);
#10157=ORIENTED_EDGE('',*,*,#6144,.F.);
#10158=ORIENTED_EDGE('',*,*,#5349,.T.);
#10159=ORIENTED_EDGE('',*,*,#5661,.F.);
#10160=ORIENTED_EDGE('',*,*,#6915,.F.);
#10161=ORIENTED_EDGE('',*,*,#6021,.F.);
#10162=ORIENTED_EDGE('',*,*,#5347,.T.);
#10163=ORIENTED_EDGE('',*,*,#6023,.F.);
#10164=ORIENTED_EDGE('',*,*,#6916,.F.);
#10165=ORIENTED_EDGE('',*,*,#5662,.F.);
#10166=ORIENTED_EDGE('',*,*,#6915,.T.);
#10167=ORIENTED_EDGE('',*,*,#5660,.F.);
#10168=ORIENTED_EDGE('',*,*,#5345,.F.);
#10169=ORIENTED_EDGE('',*,*,#6006,.F.);
#10170=ORIENTED_EDGE('',*,*,#6916,.T.);
#10171=ORIENTED_EDGE('',*,*,#6009,.F.);
#10172=ORIENTED_EDGE('',*,*,#6917,.F.);
#10173=ORIENTED_EDGE('',*,*,#5663,.F.);
#10174=ORIENTED_EDGE('',*,*,#6917,.T.);
#10175=ORIENTED_EDGE('',*,*,#6019,.F.);
#10176=ORIENTED_EDGE('',*,*,#6918,.F.);
#10177=ORIENTED_EDGE('',*,*,#5664,.F.);
#10178=ORIENTED_EDGE('',*,*,#5343,.T.);
#10179=ORIENTED_EDGE('',*,*,#5659,.F.);
#10180=ORIENTED_EDGE('',*,*,#6918,.T.);
#10181=ORIENTED_EDGE('',*,*,#6002,.F.);
#10182=ORIENTED_EDGE('',*,*,#5339,.T.);
#10183=ORIENTED_EDGE('',*,*,#6020,.F.);
#10184=ORIENTED_EDGE('',*,*,#6919,.F.);
#10185=ORIENTED_EDGE('',*,*,#6012,.F.);
#10186=ORIENTED_EDGE('',*,*,#5341,.T.);
#10187=ORIENTED_EDGE('',*,*,#6017,.F.);
#10188=ORIENTED_EDGE('',*,*,#6920,.F.);
#10189=ORIENTED_EDGE('',*,*,#6022,.F.);
#10190=ORIENTED_EDGE('',*,*,#6919,.T.);
#10191=ORIENTED_EDGE('',*,*,#6007,.F.);
#10192=ORIENTED_EDGE('',*,*,#5335,.F.);
#10193=ORIENTED_EDGE('',*,*,#6013,.F.);
#10194=ORIENTED_EDGE('',*,*,#6920,.T.);
#10195=ORIENTED_EDGE('',*,*,#6016,.F.);
#10196=ORIENTED_EDGE('',*,*,#6921,.F.);
#10197=ORIENTED_EDGE('',*,*,#6011,.F.);
#10198=ORIENTED_EDGE('',*,*,#6921,.T.);
#10199=ORIENTED_EDGE('',*,*,#6015,.F.);
#10200=ORIENTED_EDGE('',*,*,#6922,.F.);
#10201=ORIENTED_EDGE('',*,*,#6018,.F.);
#10202=ORIENTED_EDGE('',*,*,#5337,.T.);
#10203=ORIENTED_EDGE('',*,*,#6004,.F.);
#10204=ORIENTED_EDGE('',*,*,#6922,.T.);
#10205=ORIENTED_EDGE('',*,*,#6014,.F.);
#10206=ORIENTED_EDGE('',*,*,#5750,.F.);
#10207=ORIENTED_EDGE('',*,*,#6923,.T.);
#10208=ORIENTED_EDGE('',*,*,#5803,.T.);
#10209=ORIENTED_EDGE('',*,*,#6924,.F.);
#10210=ORIENTED_EDGE('',*,*,#5780,.T.);
#10211=ORIENTED_EDGE('',*,*,#6925,.T.);
#10212=ORIENTED_EDGE('',*,*,#5748,.F.);
#10213=ORIENTED_EDGE('',*,*,#6926,.T.);
#10214=ORIENTED_EDGE('',*,*,#6927,.F.);
#10215=ORIENTED_EDGE('',*,*,#5915,.F.);
#10216=ORIENTED_EDGE('',*,*,#6928,.T.);
#10217=ORIENTED_EDGE('',*,*,#5751,.T.);
#10218=ORIENTED_EDGE('',*,*,#6924,.T.);
#10219=ORIENTED_EDGE('',*,*,#5802,.F.);
#10220=ORIENTED_EDGE('',*,*,#5622,.F.);
#10221=ORIENTED_EDGE('',*,*,#6929,.F.);
#10222=ORIENTED_EDGE('',*,*,#6930,.F.);
#10223=ORIENTED_EDGE('',*,*,#5690,.T.);
#10224=ORIENTED_EDGE('',*,*,#5749,.F.);
#10225=ORIENTED_EDGE('',*,*,#6925,.F.);
#10226=ORIENTED_EDGE('',*,*,#5804,.F.);
#10227=ORIENTED_EDGE('',*,*,#6923,.F.);
#10228=ORIENTED_EDGE('',*,*,#5310,.T.);
#10229=ORIENTED_EDGE('',*,*,#5318,.F.);
#10230=ORIENTED_EDGE('',*,*,#5313,.T.);
#10231=ORIENTED_EDGE('',*,*,#5312,.F.);
#10232=ORIENTED_EDGE('',*,*,#5309,.F.);
#10233=ORIENTED_EDGE('',*,*,#5316,.T.);
#10234=ORIENTED_EDGE('',*,*,#5902,.F.);
#10235=ORIENTED_EDGE('',*,*,#6931,.F.);
#10236=ORIENTED_EDGE('',*,*,#6932,.F.);
#10237=ORIENTED_EDGE('',*,*,#5624,.T.);
#10238=ORIENTED_EDGE('',*,*,#5801,.T.);
#10239=ORIENTED_EDGE('',*,*,#6563,.T.);
#10240=ORIENTED_EDGE('',*,*,#6159,.F.);
#10241=ORIENTED_EDGE('',*,*,#6517,.T.);
#10242=ORIENTED_EDGE('',*,*,#5742,.T.);
#10243=ORIENTED_EDGE('',*,*,#5739,.F.);
#10244=ORIENTED_EDGE('',*,*,#5745,.T.);
#10245=ORIENTED_EDGE('',*,*,#5781,.T.);
#10246=ORIENTED_EDGE('',*,*,#6926,.F.);
#10247=ORIENTED_EDGE('',*,*,#5752,.T.);
#10248=ORIENTED_EDGE('',*,*,#6928,.F.);
#10249=ORIENTED_EDGE('',*,*,#5914,.F.);
#10250=ORIENTED_EDGE('',*,*,#5900,.T.);
#10251=ORIENTED_EDGE('',*,*,#6933,.F.);
#10252=ORIENTED_EDGE('',*,*,#5693,.T.);
#10253=ORIENTED_EDGE('',*,*,#6934,.T.);
#10254=ORIENTED_EDGE('',*,*,#5901,.T.);
#10255=ORIENTED_EDGE('',*,*,#6934,.F.);
#10256=ORIENTED_EDGE('',*,*,#5692,.T.);
#10257=ORIENTED_EDGE('',*,*,#6935,.T.);
#10258=ORIENTED_EDGE('',*,*,#6936,.F.);
#10259=ORIENTED_EDGE('',*,*,#6931,.T.);
#10260=ORIENTED_EDGE('',*,*,#6937,.F.);
#10261=ORIENTED_EDGE('',*,*,#6929,.T.);
#10262=ORIENTED_EDGE('',*,*,#5621,.T.);
#10263=ORIENTED_EDGE('',*,*,#6932,.T.);
#10264=ORIENTED_EDGE('',*,*,#6936,.T.);
#10265=ORIENTED_EDGE('',*,*,#5704,.T.);
#10266=ORIENTED_EDGE('',*,*,#5728,.F.);
#10267=ORIENTED_EDGE('',*,*,#5681,.T.);
#10268=ORIENTED_EDGE('',*,*,#5731,.F.);
#10269=ORIENTED_EDGE('',*,*,#5919,.F.);
#10270=ORIENTED_EDGE('',*,*,#6938,.F.);
#10271=ORIENTED_EDGE('',*,*,#5705,.T.);
#10272=ORIENTED_EDGE('',*,*,#6938,.T.);
#10273=ORIENTED_EDGE('',*,*,#5918,.F.);
#10274=ORIENTED_EDGE('',*,*,#6939,.F.);
#10275=ORIENTED_EDGE('',*,*,#6927,.T.);
#10276=ORIENTED_EDGE('',*,*,#5689,.F.);
#10277=ORIENTED_EDGE('',*,*,#6940,.T.);
#10278=ORIENTED_EDGE('',*,*,#5916,.T.);
#10279=ORIENTED_EDGE('',*,*,#6933,.T.);
#10280=ORIENTED_EDGE('',*,*,#5899,.T.);
#10281=ORIENTED_EDGE('',*,*,#6880,.T.);
#10282=ORIENTED_EDGE('',*,*,#6077,.F.);
#10283=ORIENTED_EDGE('',*,*,#6751,.T.);
#10284=ORIENTED_EDGE('',*,*,#5694,.F.);
#10285=ORIENTED_EDGE('',*,*,#5706,.T.);
#10286=ORIENTED_EDGE('',*,*,#6939,.T.);
#10287=ORIENTED_EDGE('',*,*,#5917,.F.);
#10288=ORIENTED_EDGE('',*,*,#6940,.F.);
#10289=ORIENTED_EDGE('',*,*,#5707,.T.);
#10290=ORIENTED_EDGE('',*,*,#6941,.F.);
#10291=ORIENTED_EDGE('',*,*,#5626,.T.);
#10292=ORIENTED_EDGE('',*,*,#5733,.F.);
#10293=ORIENTED_EDGE('',*,*,#5685,.T.);
#10294=ORIENTED_EDGE('',*,*,#5726,.F.);
#10295=ORIENTED_EDGE('',*,*,#5721,.T.);
#10296=ORIENTED_EDGE('',*,*,#6942,.F.);
#10297=ORIENTED_EDGE('',*,*,#5627,.T.);
#10298=ORIENTED_EDGE('',*,*,#6941,.T.);
#10299=ORIENTED_EDGE('',*,*,#5720,.T.);
#10300=ORIENTED_EDGE('',*,*,#6943,.F.);
#10301=ORIENTED_EDGE('',*,*,#6259,.F.);
#10302=ORIENTED_EDGE('',*,*,#5736,.T.);
#10303=ORIENTED_EDGE('',*,*,#5722,.T.);
#10304=ORIENTED_EDGE('',*,*,#5735,.F.);
#10305=ORIENTED_EDGE('',*,*,#6942,.T.);
#10306=ORIENTED_EDGE('',*,*,#6712,.T.);
#10307=ORIENTED_EDGE('',*,*,#6087,.F.);
#10308=ORIENTED_EDGE('',*,*,#6888,.T.);
#10309=ORIENTED_EDGE('',*,*,#5637,.F.);
#10310=ORIENTED_EDGE('',*,*,#6944,.T.);
#10311=ORIENTED_EDGE('',*,*,#5716,.F.);
#10312=ORIENTED_EDGE('',*,*,#5717,.T.);
#10313=ORIENTED_EDGE('',*,*,#6944,.F.);
#10314=ORIENTED_EDGE('',*,*,#5636,.T.);
#10315=ORIENTED_EDGE('',*,*,#6945,.T.);
#10316=ORIENTED_EDGE('',*,*,#6945,.F.);
#10317=ORIENTED_EDGE('',*,*,#6895,.T.);
#10318=ORIENTED_EDGE('',*,*,#6245,.F.);
#10319=ORIENTED_EDGE('',*,*,#6902,.F.);
#10320=ORIENTED_EDGE('',*,*,#6251,.T.);
#10321=ORIENTED_EDGE('',*,*,#6946,.T.);
#10322=ORIENTED_EDGE('',*,*,#5718,.F.);
#10323=ORIENTED_EDGE('',*,*,#6946,.F.);
#10324=ORIENTED_EDGE('',*,*,#6260,.T.);
#10325=ORIENTED_EDGE('',*,*,#6943,.T.);
#10326=ORIENTED_EDGE('',*,*,#5719,.F.);
#10327=ORIENTED_EDGE('',*,*,#5691,.T.);
#10328=ORIENTED_EDGE('',*,*,#6930,.T.);
#10329=ORIENTED_EDGE('',*,*,#6937,.T.);
#10330=ORIENTED_EDGE('',*,*,#6935,.F.);
#10539=CYLINDRICAL_SURFACE('',#11524,2.1875);
#10540=CYLINDRICAL_SURFACE('',#11527,2.5625);
#10541=CYLINDRICAL_SURFACE('',#11530,3.4375);
#10542=CYLINDRICAL_SURFACE('',#11533,1.3125);
#10543=CYLINDRICAL_SURFACE('',#11692,0.3125);
#10544=CYLINDRICAL_SURFACE('',#11695,0.3125);
#10545=CYLINDRICAL_SURFACE('',#11698,0.3125);
#10546=CYLINDRICAL_SURFACE('',#11705,0.3125);
#10547=CYLINDRICAL_SURFACE('',#11708,0.3125);
#10548=CYLINDRICAL_SURFACE('',#11711,0.3125);
#10549=CYLINDRICAL_SURFACE('',#11714,0.3125);
#10550=CYLINDRICAL_SURFACE('',#11732,0.937500000000001);
#10551=CYLINDRICAL_SURFACE('',#11735,4.375);
#10552=CYLINDRICAL_SURFACE('',#11738,2.8125);
#10553=CYLINDRICAL_SURFACE('',#11739,2.8125);
#10554=CYLINDRICAL_SURFACE('',#11740,0.937500000000001);
#10555=CYLINDRICAL_SURFACE('',#11742,0.937500000000001);
#10556=CYLINDRICAL_SURFACE('',#11745,4.375);
#10557=CYLINDRICAL_SURFACE('',#11748,2.8125);
#10558=CYLINDRICAL_SURFACE('',#11749,2.8125);
#10559=CYLINDRICAL_SURFACE('',#11753,0.937500000000001);
#10560=CYLINDRICAL_SURFACE('',#11755,0.937500000000001);
#10561=CYLINDRICAL_SURFACE('',#11758,4.375);
#10562=CYLINDRICAL_SURFACE('',#11759,2.8125);
#10563=CYLINDRICAL_SURFACE('',#11760,2.8125);
#10564=CYLINDRICAL_SURFACE('',#11765,0.937500000000001);
#10565=CYLINDRICAL_SURFACE('',#11767,0.937500000000001);
#10566=CYLINDRICAL_SURFACE('',#11768,4.375);
#10567=CYLINDRICAL_SURFACE('',#11769,48.4375);
#10568=CYLINDRICAL_SURFACE('',#11810,2.8125);
#10569=CYLINDRICAL_SURFACE('',#11811,2.8125);
#10570=CYLINDRICAL_SURFACE('',#11816,0.937500000000001);
#10571=CYLINDRICAL_SURFACE('',#11818,1.25);
#10572=CYLINDRICAL_SURFACE('',#11860,0.3125);
#10573=CYLINDRICAL_SURFACE('',#11863,0.3125);
#10574=CYLINDRICAL_SURFACE('',#11866,0.3125);
#10575=CYLINDRICAL_SURFACE('',#11869,0.3125);
#10576=CYLINDRICAL_SURFACE('',#11872,0.3125);
#10577=CYLINDRICAL_SURFACE('',#11874,0.3125);
#10578=CYLINDRICAL_SURFACE('',#11877,0.3125);
#10579=CYLINDRICAL_SURFACE('',#11880,0.312499999999999);
#10580=CYLINDRICAL_SURFACE('',#11931,49.6875);
#10581=CYLINDRICAL_SURFACE('',#11934,49.6875);
#10582=CYLINDRICAL_SURFACE('',#11956,5.625);
#10583=CYLINDRICAL_SURFACE('',#11981,5.625);
#10584=CYLINDRICAL_SURFACE('',#11995,21.875);
#10585=CYLINDRICAL_SURFACE('',#12006,55.);
#10586=CYLINDRICAL_SURFACE('',#12016,0.937500000000001);
#10587=CYLINDRICAL_SURFACE('',#12019,0.937500000000001);
#10588=CYLINDRICAL_SURFACE('',#12022,0.937500000000001);
#10589=CYLINDRICAL_SURFACE('',#12040,49.6875);
#10590=CYLINDRICAL_SURFACE('',#12057,5.625);
#10591=CYLINDRICAL_SURFACE('',#12061,5.625);
#10592=CYLINDRICAL_SURFACE('',#12072,21.875);
#10593=CYLINDRICAL_SURFACE('',#12083,55.);
#10594=CYLINDRICAL_SURFACE('',#12093,0.937500000000001);
#10595=CYLINDRICAL_SURFACE('',#12094,0.937500000000001);
#10596=CYLINDRICAL_SURFACE('',#12097,0.937500000000001);
#10597=CYLINDRICAL_SURFACE('',#12115,49.6875);
#10598=CYLINDRICAL_SURFACE('',#12120,5.625);
#10599=CYLINDRICAL_SURFACE('',#12124,5.625);
#10600=CYLINDRICAL_SURFACE('',#12135,21.875);
#10601=CYLINDRICAL_SURFACE('',#12146,55.);
#10602=CYLINDRICAL_SURFACE('',#12157,0.937500000000001);
#10603=CYLINDRICAL_SURFACE('',#12160,0.937500000000001);
#10604=CYLINDRICAL_SURFACE('',#12161,0.937500000000001);
#10605=CYLINDRICAL_SURFACE('',#12188,5.625);
#10606=CYLINDRICAL_SURFACE('',#12191,5.625);
#10607=CYLINDRICAL_SURFACE('',#12199,21.875);
#10608=CYLINDRICAL_SURFACE('',#12210,55.);
#10609=CYLINDRICAL_SURFACE('',#12221,0.937500000000001);
#10610=CYLINDRICAL_SURFACE('',#12224,0.937500000000001);
#10611=CYLINDRICAL_SURFACE('',#12227,0.937500000000001);
#10612=CYLINDRICAL_SURFACE('',#12232,0.3125);
#10613=CYLINDRICAL_SURFACE('',#12234,0.3125);
#10614=CYLINDRICAL_SURFACE('',#12245,0.3125);
#10615=CYLINDRICAL_SURFACE('',#12247,0.3125);
#10616=CYLINDRICAL_SURFACE('',#12262,0.312500000000001);
#10617=CYLINDRICAL_SURFACE('',#12264,0.3125);
#10618=CYLINDRICAL_SURFACE('',#12267,0.3125);
#10619=CYLINDRICAL_SURFACE('',#12281,0.312500000000001);
#10620=CYLINDRICAL_SURFACE('',#12284,0.3125);
#10621=CYLINDRICAL_SURFACE('',#12287,0.312499999999999);
#10622=CYLINDRICAL_SURFACE('',#12297,0.312500000000002);
#10623=CYLINDRICAL_SURFACE('',#12309,0.3125);
#10624=CYLINDRICAL_SURFACE('',#12315,0.312500000000001);
#10625=CYLINDRICAL_SURFACE('',#12316,0.3125);
#10626=CYLINDRICAL_SURFACE('',#12319,0.312499999999999);
#10627=CYLINDRICAL_SURFACE('',#12325,0.3125);
#10628=CYLINDRICAL_SURFACE('',#12327,0.312499999999999);
#10629=CYLINDRICAL_SURFACE('',#12344,0.3125);
#10630=CYLINDRICAL_SURFACE('',#12346,0.312500000000001);
#10631=CYLINDRICAL_SURFACE('',#12350,0.3125);
#10632=CYLINDRICAL_SURFACE('',#12359,0.3125);
#10633=CYLINDRICAL_SURFACE('',#12361,0.3125);
#10634=CYLINDRICAL_SURFACE('',#12364,0.312499999999999);
#10635=CYLINDRICAL_SURFACE('',#12370,0.3125);
#10636=CYLINDRICAL_SURFACE('',#12375,0.3125);
#10637=CYLINDRICAL_SURFACE('',#12378,0.3125);
#10638=CYLINDRICAL_SURFACE('',#12390,0.312499999999999);
#10639=CYLINDRICAL_SURFACE('',#12401,0.3125);
#10640=CYLINDRICAL_SURFACE('',#12404,0.3125);
#10641=CYLINDRICAL_SURFACE('',#12406,0.312499999999999);
#10642=CYLINDRICAL_SURFACE('',#12409,0.3125);
#10643=CYLINDRICAL_SURFACE('',#12411,0.3125);
#10644=CYLINDRICAL_SURFACE('',#12419,0.312500000000001);
#10645=CYLINDRICAL_SURFACE('',#12429,0.3125);
#10646=CYLINDRICAL_SURFACE('',#12433,0.312499999999999);
#10647=CYLINDRICAL_SURFACE('',#12435,0.3125);
#10648=CYLINDRICAL_SURFACE('',#12437,0.3125);
#10649=CYLINDRICAL_SURFACE('',#12449,0.3125);
#10650=CYLINDRICAL_SURFACE('',#12451,0.3125);
#10651=CYLINDRICAL_SURFACE('',#12455,0.3125);
#10652=CYLINDRICAL_SURFACE('',#12458,0.312499999999999);
#10653=CYLINDRICAL_SURFACE('',#12462,0.3125);
#10654=CYLINDRICAL_SURFACE('',#12471,0.312499999999999);
#10655=CYLINDRICAL_SURFACE('',#12478,0.312499999999999);
#10656=CYLINDRICAL_SURFACE('',#12483,0.3125);
#10657=CYLINDRICAL_SURFACE('',#12485,0.3125);
#10658=CYLINDRICAL_SURFACE('',#12491,0.3125);
#10659=CYLINDRICAL_SURFACE('',#12494,0.3125);
#10660=CYLINDRICAL_SURFACE('',#12500,0.3125);
#10661=CYLINDRICAL_SURFACE('',#12503,0.3125);
#10662=CYLINDRICAL_SURFACE('',#12511,0.3125);
#10663=CYLINDRICAL_SURFACE('',#12513,0.3125);
#10664=CYLINDRICAL_SURFACE('',#12519,0.3125);
#10665=CYLINDRICAL_SURFACE('',#12527,0.3125);
#10666=CYLINDRICAL_SURFACE('',#12531,0.3125);
#10667=CYLINDRICAL_SURFACE('',#12536,0.312499169784042);
#10668=CYLINDRICAL_SURFACE('',#12547,0.312499999999999);
#10669=CYLINDRICAL_SURFACE('',#12561,0.312499805812968);
#10670=CYLINDRICAL_SURFACE('',#12566,0.3125);
#10671=CYLINDRICAL_SURFACE('',#12568,0.312500000000001);
#10672=CYLINDRICAL_SURFACE('',#12583,0.312500000000001);
#10673=CYLINDRICAL_SURFACE('',#12586,0.312500000000001);
#10674=CYLINDRICAL_SURFACE('',#12588,0.3125);
#10675=CYLINDRICAL_SURFACE('',#12590,0.3125);
#10676=CYLINDRICAL_SURFACE('',#12593,0.312499805814757);
#10677=CYLINDRICAL_SURFACE('',#12608,0.312500000000001);
#10678=CYLINDRICAL_SURFACE('',#12610,0.3125);
#10679=CYLINDRICAL_SURFACE('',#12614,0.312500000000001);
#10680=CYLINDRICAL_SURFACE('',#12615,0.312500000000001);
#10681=CYLINDRICAL_SURFACE('',#12619,0.3125);
#10682=CYLINDRICAL_SURFACE('',#12624,0.3125);
#10683=CYLINDRICAL_SURFACE('',#12643,0.3125);
#10684=CYLINDRICAL_SURFACE('',#12645,0.3125);
#10685=CYLINDRICAL_SURFACE('',#12647,0.312500000000001);
#10686=CYLINDRICAL_SURFACE('',#12649,0.31249916978701);
#10687=CYLINDRICAL_SURFACE('',#12652,0.3125);
#10688=CYLINDRICAL_SURFACE('',#12656,0.312499169785485);
#10689=CYLINDRICAL_SURFACE('',#12658,0.3125);
#10690=CYLINDRICAL_SURFACE('',#12679,0.3125);
#10691=CYLINDRICAL_SURFACE('',#12683,0.3125);
#10692=CYLINDRICAL_SURFACE('',#12687,0.312499805816233);
#10693=CYLINDRICAL_SURFACE('',#12692,0.3125);
#10694=CYLINDRICAL_SURFACE('',#12694,0.3125);
#10695=CYLINDRICAL_SURFACE('',#12696,0.312500000000001);
#10696=CYLINDRICAL_SURFACE('',#12713,0.3125);
#10697=CYLINDRICAL_SURFACE('',#12718,0.3125);
#10698=CYLINDRICAL_SURFACE('',#12720,0.312499999999999);
#10699=CYLINDRICAL_SURFACE('',#12721,0.3125);
#10700=CYLINDRICAL_SURFACE('',#12726,0.312500000000001);
#10701=CYLINDRICAL_SURFACE('',#12728,0.312500000000001);
#10702=CYLINDRICAL_SURFACE('',#12739,0.3125);
#10703=CYLINDRICAL_SURFACE('',#12741,0.3125);
#10704=CYLINDRICAL_SURFACE('',#12746,0.312499999999999);
#10705=CYLINDRICAL_SURFACE('',#12750,0.312499805811005);
#10706=CYLINDRICAL_SURFACE('',#12752,0.312500000000001);
#10707=CYLINDRICAL_SURFACE('',#12768,0.3125);
#10708=CYLINDRICAL_SURFACE('',#12770,0.312500000000001);
#10709=CYLINDRICAL_SURFACE('',#12772,0.312499169782492);
#10710=CYLINDRICAL_SURFACE('',#12774,0.3125);
#10711=CYLINDRICAL_SURFACE('',#12784,0.312499999999996);
#10712=CYLINDRICAL_SURFACE('',#12786,0.3125);
#10713=CYLINDRICAL_SURFACE('',#12795,0.3125);
#10714=CYLINDRICAL_SURFACE('',#12802,0.3125);
#10715=CYLINDRICAL_SURFACE('',#12813,0.3125);
#10716=CYLINDRICAL_SURFACE('',#12820,0.3125);
#10717=CYLINDRICAL_SURFACE('',#12828,0.3125);
#10718=CYLINDRICAL_SURFACE('',#12830,0.3125);
#10719=CYLINDRICAL_SURFACE('',#12836,0.3125);
#10720=CYLINDRICAL_SURFACE('',#12838,0.3125);
#10721=CYLINDRICAL_SURFACE('',#12844,0.3125);
#10722=CYLINDRICAL_SURFACE('',#12846,0.3125);
#10723=CYLINDRICAL_SURFACE('',#12852,0.3125);
#10724=CYLINDRICAL_SURFACE('',#12854,0.3125);
#10725=CYLINDRICAL_SURFACE('',#12861,0.3125);
#10726=CYLINDRICAL_SURFACE('',#12864,0.3125);
#10727=CYLINDRICAL_SURFACE('',#12875,0.3125);
#10728=CYLINDRICAL_SURFACE('',#12878,0.3125);
#10729=CYLINDRICAL_SURFACE('',#12889,0.3125);
#10730=CYLINDRICAL_SURFACE('',#12891,0.3125);
#10731=CYLINDRICAL_SURFACE('',#12899,0.3125);
#10732=CYLINDRICAL_SURFACE('',#12901,0.3125);
#10733=CYLINDRICAL_SURFACE('',#12909,0.3125);
#10734=CYLINDRICAL_SURFACE('',#12910,0.3125);
#10735=CYLINDRICAL_SURFACE('',#12919,0.3125);
#10736=CYLINDRICAL_SURFACE('',#12920,0.3125);
#10737=CYLINDRICAL_SURFACE('',#12925,20.);
#10738=CYLINDRICAL_SURFACE('',#12928,1.25);
#10750=ADVANCED_FACE('',(#1012),#10539,.F.);
#10751=ADVANCED_FACE('',(#1013),#10540,.F.);
#10752=ADVANCED_FACE('',(#1014),#10541,.T.);
#10753=ADVANCED_FACE('',(#1015),#10542,.F.);
#10754=ADVANCED_FACE('',(#1016),#837,.T.);
#10755=ADVANCED_FACE('',(#1017),#838,.T.);
#10756=ADVANCED_FACE('',(#1018),#839,.T.);
#10757=ADVANCED_FACE('',(#1019),#840,.T.);
#10758=ADVANCED_FACE('',(#1020),#841,.F.);
#10759=ADVANCED_FACE('',(#1021),#842,.F.);
#10760=ADVANCED_FACE('',(#1022),#843,.T.);
#10761=ADVANCED_FACE('',(#1023),#844,.T.);
#10762=ADVANCED_FACE('',(#1024),#845,.T.);
#10763=ADVANCED_FACE('',(#1025),#846,.T.);
#10764=ADVANCED_FACE('',(#1026),#847,.T.);
#10765=ADVANCED_FACE('',(#1027),#848,.T.);
#10766=ADVANCED_FACE('',(#1028),#849,.F.);
#10767=ADVANCED_FACE('',(#1029),#850,.F.);
#10768=ADVANCED_FACE('',(#1030),#851,.T.);
#10769=ADVANCED_FACE('',(#1031),#852,.T.);
#10770=ADVANCED_FACE('',(#1032),#853,.T.);
#10771=ADVANCED_FACE('',(#1033),#854,.T.);
#10772=ADVANCED_FACE('',(#1034),#855,.T.);
#10773=ADVANCED_FACE('',(#1035),#856,.T.);
#10774=ADVANCED_FACE('',(#1036),#857,.F.);
#10775=ADVANCED_FACE('',(#1037),#858,.T.);
#10776=ADVANCED_FACE('',(#1038),#859,.T.);
#10777=ADVANCED_FACE('',(#1039),#860,.T.);
#10778=ADVANCED_FACE('',(#1040),#861,.T.);
#10779=ADVANCED_FACE('',(#1041),#862,.T.);
#10780=ADVANCED_FACE('',(#1042),#863,.F.);
#10781=ADVANCED_FACE('',(#1043),#864,.F.);
#10782=ADVANCED_FACE('',(#1044),#865,.F.);
#10783=ADVANCED_FACE('',(#1045),#866,.F.);
#10784=ADVANCED_FACE('',(#1046),#867,.F.);
#10785=ADVANCED_FACE('',(#1047),#868,.F.);
#10786=ADVANCED_FACE('',(#1048),#10543,.F.);
#10787=ADVANCED_FACE('',(#1049),#10544,.F.);
#10788=ADVANCED_FACE('',(#1050),#10545,.F.);
#10789=ADVANCED_FACE('',(#1051),#869,.T.);
#10790=ADVANCED_FACE('',(#1052),#10546,.T.);
#10791=ADVANCED_FACE('',(#1053),#10547,.F.);
#10792=ADVANCED_FACE('',(#1054),#10548,.T.);
#10793=ADVANCED_FACE('',(#1055),#10549,.F.);
#10794=ADVANCED_FACE('',(#1056),#870,.T.);
#10795=ADVANCED_FACE('',(#1057),#871,.F.);
#10796=ADVANCED_FACE('',(#1058),#872,.T.);
#10797=ADVANCED_FACE('',(#1059),#10550,.F.);
#10798=ADVANCED_FACE('',(#1060),#10551,.T.);
#10799=ADVANCED_FACE('',(#1061),#10552,.F.);
#10800=ADVANCED_FACE('',(#1062),#10553,.F.);
#10801=ADVANCED_FACE('',(#1063),#10554,.T.);
#10802=ADVANCED_FACE('',(#1064),#10555,.F.);
#10803=ADVANCED_FACE('',(#1065),#10556,.T.);
#10804=ADVANCED_FACE('',(#1066),#10557,.F.);
#10805=ADVANCED_FACE('',(#1067),#10558,.F.);
#10806=ADVANCED_FACE('',(#1068),#817,.T.);
#10807=ADVANCED_FACE('',(#1069),#10559,.T.);
#10808=ADVANCED_FACE('',(#1070),#10560,.F.);
#10809=ADVANCED_FACE('',(#1071),#10561,.T.);
#10810=ADVANCED_FACE('',(#1072),#10562,.F.);
#10811=ADVANCED_FACE('',(#1073),#10563,.F.);
#10812=ADVANCED_FACE('',(#1074),#818,.T.);
#10813=ADVANCED_FACE('',(#1075),#10564,.T.);
#10814=ADVANCED_FACE('',(#1076),#10565,.F.);
#10815=ADVANCED_FACE('',(#1077),#10566,.T.);
#10816=ADVANCED_FACE('',(#1078),#10567,.F.);
#10817=ADVANCED_FACE('',(#1079),#10568,.F.);
#10818=ADVANCED_FACE('',(#1080),#10569,.F.);
#10819=ADVANCED_FACE('',(#1081),#819,.T.);
#10820=ADVANCED_FACE('',(#1082),#10570,.T.);
#10821=ADVANCED_FACE('',(#1083),#10571,.F.);
#10822=ADVANCED_FACE('',(#1084,#284,#285,#286,#287,#288,#289,#290,#291),
#315,.T.);
#10823=ADVANCED_FACE('',(#1085),#316,.F.);
#10824=ADVANCED_FACE('',(#1086),#317,.F.);
#10825=ADVANCED_FACE('',(#1087,#292),#318,.F.);
#10826=ADVANCED_FACE('',(#1088,#293),#319,.F.);
#10827=ADVANCED_FACE('',(#1089),#320,.F.);
#10828=ADVANCED_FACE('',(#1090),#10572,.T.);
#10829=ADVANCED_FACE('',(#1091),#10573,.T.);
#10830=ADVANCED_FACE('',(#1092),#10574,.T.);
#10831=ADVANCED_FACE('',(#1093),#10575,.T.);
#10832=ADVANCED_FACE('',(#1094),#10576,.T.);
#10833=ADVANCED_FACE('',(#1095),#10577,.F.);
#10834=ADVANCED_FACE('',(#1096),#321,.F.);
#10835=ADVANCED_FACE('',(#1097),#10578,.T.);
#10836=ADVANCED_FACE('',(#1098),#10579,.T.);
#10837=ADVANCED_FACE('',(#1099,#294),#322,.T.);
#10838=ADVANCED_FACE('',(#1100),#323,.T.);
#10839=ADVANCED_FACE('',(#1101),#324,.T.);
#10840=ADVANCED_FACE('',(#1102),#325,.T.);
#10841=ADVANCED_FACE('',(#1103),#326,.T.);
#10842=ADVANCED_FACE('',(#1104),#820,.F.);
#10843=ADVANCED_FACE('',(#1105),#327,.F.);
#10844=ADVANCED_FACE('',(#1106),#328,.F.);
#10845=ADVANCED_FACE('',(#1107),#329,.T.);
#10846=ADVANCED_FACE('',(#1108),#821,.F.);
#10847=ADVANCED_FACE('',(#1109),#822,.T.);
#10848=ADVANCED_FACE('',(#1110),#10580,.T.);
#10849=ADVANCED_FACE('',(#1111),#10581,.T.);
#10850=ADVANCED_FACE('',(#1112),#823,.T.);
#10851=ADVANCED_FACE('',(#1113),#824,.T.);
#10852=ADVANCED_FACE('',(#1114,#295),#330,.F.);
#10853=ADVANCED_FACE('',(#1115,#296),#331,.F.);
#10854=ADVANCED_FACE('',(#1116),#332,.F.);
#10855=ADVANCED_FACE('',(#1117),#333,.F.);
#10856=ADVANCED_FACE('',(#1118),#10582,.T.);
#10857=ADVANCED_FACE('',(#1119),#334,.F.);
#10858=ADVANCED_FACE('',(#1120),#335,.F.);
#10859=ADVANCED_FACE('',(#1121,#297,#298,#299,#300,#301,#302,#303,#304),
#336,.F.);
#10860=ADVANCED_FACE('',(#1122),#10583,.T.);
#10861=ADVANCED_FACE('',(#1123),#825,.F.);
#10862=ADVANCED_FACE('',(#1124),#337,.T.);
#10863=ADVANCED_FACE('',(#1125),#338,.T.);
#10864=ADVANCED_FACE('',(#1126),#339,.F.);
#10865=ADVANCED_FACE('',(#1127),#340,.F.);
#10866=ADVANCED_FACE('',(#1128),#10584,.T.);
#10867=ADVANCED_FACE('',(#1129),#341,.T.);
#10868=ADVANCED_FACE('',(#1130),#342,.T.);
#10869=ADVANCED_FACE('',(#1131),#343,.T.);
#10870=ADVANCED_FACE('',(#1132),#344,.F.);
#10871=ADVANCED_FACE('',(#1133),#10585,.T.);
#10872=ADVANCED_FACE('',(#1134),#345,.F.);
#10873=ADVANCED_FACE('',(#1135),#346,.F.);
#10874=ADVANCED_FACE('',(#1136),#347,.T.);
#10875=ADVANCED_FACE('',(#1137),#10586,.F.);
#10876=ADVANCED_FACE('',(#1138),#10587,.F.);
#10877=ADVANCED_FACE('',(#1139),#10588,.F.);
#10878=ADVANCED_FACE('',(#1140),#826,.F.);
#10879=ADVANCED_FACE('',(#1141),#348,.F.);
#10880=ADVANCED_FACE('',(#1142),#349,.T.);
#10881=ADVANCED_FACE('',(#1143),#827,.F.);
#10882=ADVANCED_FACE('',(#1144),#10589,.T.);
#10883=ADVANCED_FACE('',(#1145),#828,.T.);
#10884=ADVANCED_FACE('',(#1146,#305),#350,.F.);
#10885=ADVANCED_FACE('',(#1147,#306),#351,.F.);
#10886=ADVANCED_FACE('',(#1148),#352,.F.);
#10887=ADVANCED_FACE('',(#1149),#10590,.T.);
#10888=ADVANCED_FACE('',(#1150),#353,.F.);
#10889=ADVANCED_FACE('',(#1151),#10591,.T.);
#10890=ADVANCED_FACE('',(#1152),#829,.F.);
#10891=ADVANCED_FACE('',(#1153),#354,.T.);
#10892=ADVANCED_FACE('',(#1154),#355,.F.);
#10893=ADVANCED_FACE('',(#1155),#356,.F.);
#10894=ADVANCED_FACE('',(#1156),#10592,.T.);
#10895=ADVANCED_FACE('',(#1157),#357,.T.);
#10896=ADVANCED_FACE('',(#1158),#358,.T.);
#10897=ADVANCED_FACE('',(#1159),#359,.T.);
#10898=ADVANCED_FACE('',(#1160),#360,.F.);
#10899=ADVANCED_FACE('',(#1161),#10593,.T.);
#10900=ADVANCED_FACE('',(#1162),#361,.F.);
#10901=ADVANCED_FACE('',(#1163),#362,.F.);
#10902=ADVANCED_FACE('',(#1164),#363,.T.);
#10903=ADVANCED_FACE('',(#1165),#10594,.F.);
#10904=ADVANCED_FACE('',(#1166),#10595,.F.);
#10905=ADVANCED_FACE('',(#1167),#10596,.F.);
#10906=ADVANCED_FACE('',(#1168),#830,.F.);
#10907=ADVANCED_FACE('',(#1169),#364,.F.);
#10908=ADVANCED_FACE('',(#1170),#365,.T.);
#10909=ADVANCED_FACE('',(#1171),#831,.F.);
#10910=ADVANCED_FACE('',(#1172),#10597,.T.);
#10911=ADVANCED_FACE('',(#1173),#832,.T.);
#10912=ADVANCED_FACE('',(#1174),#366,.F.);
#10913=ADVANCED_FACE('',(#1175),#10598,.T.);
#10914=ADVANCED_FACE('',(#1176),#367,.F.);
#10915=ADVANCED_FACE('',(#1177),#10599,.T.);
#10916=ADVANCED_FACE('',(#1178),#833,.F.);
#10917=ADVANCED_FACE('',(#1179),#368,.T.);
#10918=ADVANCED_FACE('',(#1180),#369,.F.);
#10919=ADVANCED_FACE('',(#1181),#370,.F.);
#10920=ADVANCED_FACE('',(#1182),#10600,.T.);
#10921=ADVANCED_FACE('',(#1183),#371,.T.);
#10922=ADVANCED_FACE('',(#1184),#372,.T.);
#10923=ADVANCED_FACE('',(#1185),#373,.T.);
#10924=ADVANCED_FACE('',(#1186),#374,.F.);
#10925=ADVANCED_FACE('',(#1187),#10601,.T.);
#10926=ADVANCED_FACE('',(#1188),#375,.F.);
#10927=ADVANCED_FACE('',(#1189),#376,.F.);
#10928=ADVANCED_FACE('',(#1190),#377,.T.);
#10929=ADVANCED_FACE('',(#1191),#10602,.F.);
#10930=ADVANCED_FACE('',(#1192),#10603,.F.);
#10931=ADVANCED_FACE('',(#1193),#10604,.F.);
#10932=ADVANCED_FACE('',(#1194),#834,.F.);
#10933=ADVANCED_FACE('',(#1195),#378,.F.);
#10934=ADVANCED_FACE('',(#1196),#379,.T.);
#10935=ADVANCED_FACE('',(#1197),#835,.F.);
#10936=ADVANCED_FACE('',(#1198,#307),#380,.F.);
#10937=ADVANCED_FACE('',(#1199,#308),#381,.F.);
#10938=ADVANCED_FACE('',(#1200),#10605,.T.);
#10939=ADVANCED_FACE('',(#1201),#10606,.T.);
#10940=ADVANCED_FACE('',(#1202),#836,.F.);
#10941=ADVANCED_FACE('',(#1203),#382,.F.);
#10942=ADVANCED_FACE('',(#1204),#383,.F.);
#10943=ADVANCED_FACE('',(#1205),#10607,.T.);
#10944=ADVANCED_FACE('',(#1206),#384,.T.);
#10945=ADVANCED_FACE('',(#1207),#385,.T.);
#10946=ADVANCED_FACE('',(#1208),#386,.T.);
#10947=ADVANCED_FACE('',(#1209),#387,.F.);
#10948=ADVANCED_FACE('',(#1210),#10608,.T.);
#10949=ADVANCED_FACE('',(#1211),#388,.F.);
#10950=ADVANCED_FACE('',(#1212),#389,.F.);
#10951=ADVANCED_FACE('',(#1213),#390,.T.);
#10952=ADVANCED_FACE('',(#1214),#10609,.F.);
#10953=ADVANCED_FACE('',(#1215),#10610,.F.);
#10954=ADVANCED_FACE('',(#1216),#10611,.F.);
#10955=ADVANCED_FACE('',(#1217),#873,.T.);
#10956=ADVANCED_FACE('',(#1218),#874,.T.);
#10957=ADVANCED_FACE('',(#1219),#10612,.T.);
#10958=ADVANCED_FACE('',(#1220),#10613,.T.);
#10959=ADVANCED_FACE('',(#1221),#875,.T.);
#10960=ADVANCED_FACE('',(#1222),#876,.T.);
#10961=ADVANCED_FACE('',(#1223),#877,.T.);
#10962=ADVANCED_FACE('',(#1224),#878,.F.);
#10963=ADVANCED_FACE('',(#1225),#879,.F.);
#10964=ADVANCED_FACE('',(#1226),#10614,.F.);
#10965=ADVANCED_FACE('',(#1227),#10615,.F.);
#10966=ADVANCED_FACE('',(#1228),#880,.F.);
#10967=ADVANCED_FACE('',(#1229),#881,.F.);
#10968=ADVANCED_FACE('',(#1230),#882,.F.);
#10969=ADVANCED_FACE('',(#1231),#195,.T.);
#10970=ADVANCED_FACE('',(#1232),#196,.T.);
#10971=ADVANCED_FACE('',(#1233),#197,.T.);
#10972=ADVANCED_FACE('',(#1234),#198,.T.);
#10973=ADVANCED_FACE('',(#1235),#199,.T.);
#10974=ADVANCED_FACE('',(#1236),#200,.T.);
#10975=ADVANCED_FACE('',(#1237),#201,.T.);
#10976=ADVANCED_FACE('',(#1238),#202,.T.);
#10977=ADVANCED_FACE('',(#1239),#203,.T.);
#10978=ADVANCED_FACE('',(#1240),#204,.T.);
#10979=ADVANCED_FACE('',(#1241),#205,.T.);
#10980=ADVANCED_FACE('',(#1242),#206,.T.);
#10981=ADVANCED_FACE('',(#1243),#207,.T.);
#10982=ADVANCED_FACE('',(#1244),#208,.T.);
#10983=ADVANCED_FACE('',(#1245),#209,.T.);
#10984=ADVANCED_FACE('',(#1246),#210,.T.);
#10985=ADVANCED_FACE('',(#1247),#211,.T.);
#10986=ADVANCED_FACE('',(#1248),#212,.T.);
#10987=ADVANCED_FACE('',(#1249),#213,.T.);
#10988=ADVANCED_FACE('',(#1250),#214,.T.);
#10989=ADVANCED_FACE('',(#1251),#75,.F.);
#10990=ADVANCED_FACE('',(#1252),#76,.F.);
#10991=ADVANCED_FACE('',(#1253),#77,.T.);
#10992=ADVANCED_FACE('',(#1254),#883,.F.);
#10993=ADVANCED_FACE('',(#1255),#10616,.T.);
#10994=ADVANCED_FACE('',(#1256),#10617,.T.);
#10995=ADVANCED_FACE('',(#1257),#884,.T.);
#10996=ADVANCED_FACE('',(#1258),#78,.F.);
#10997=ADVANCED_FACE('',(#1259),#79,.F.);
#10998=ADVANCED_FACE('',(#1260),#10618,.T.);
#10999=ADVANCED_FACE('',(#1261),#80,.T.);
#11000=ADVANCED_FACE('',(#1262),#27,.F.);
#11001=ADVANCED_FACE('',(#1263),#81,.F.);
#11002=ADVANCED_FACE('',(#1264),#28,.T.);
#11003=ADVANCED_FACE('',(#1265),#215,.T.);
#11004=ADVANCED_FACE('',(#1266),#82,.T.);
#11005=ADVANCED_FACE('',(#1267),#885,.T.);
#11006=ADVANCED_FACE('',(#1268),#83,.F.);
#11007=ADVANCED_FACE('',(#1269),#10619,.F.);
#11008=ADVANCED_FACE('',(#1270),#886,.T.);
#11009=ADVANCED_FACE('',(#1271),#84,.F.);
#11010=ADVANCED_FACE('',(#1272),#10620,.T.);
#11011=ADVANCED_FACE('',(#1273),#10621,.T.);
#11012=ADVANCED_FACE('',(#1274),#887,.F.);
#11013=ADVANCED_FACE('',(#1275),#85,.T.);
#11014=ADVANCED_FACE('',(#1276),#888,.T.);
#11015=ADVANCED_FACE('',(#1277),#86,.F.);
#11016=ADVANCED_FACE('',(#1278),#889,.T.);
#11017=ADVANCED_FACE('',(#1279),#10622,.T.);
#11018=ADVANCED_FACE('',(#1280),#87,.T.);
#11019=ADVANCED_FACE('',(#1281),#88,.F.);
#11020=ADVANCED_FACE('',(#1282),#29,.T.);
#11021=ADVANCED_FACE('',(#1283),#30,.F.);
#11022=ADVANCED_FACE('',(#1284),#89,.T.);
#11023=ADVANCED_FACE('',(#1285),#10623,.T.);
#11024=ADVANCED_FACE('',(#1286),#90,.F.);
#11025=ADVANCED_FACE('',(#1287),#91,.F.);
#11026=ADVANCED_FACE('',(#1288),#890,.T.);
#11027=ADVANCED_FACE('',(#1289),#92,.T.);
#11028=ADVANCED_FACE('',(#1290),#93,.F.);
#11029=ADVANCED_FACE('',(#1291),#94,.T.);
#11030=ADVANCED_FACE('',(#1292),#891,.T.);
#11031=ADVANCED_FACE('',(#1293),#10624,.T.);
#11032=ADVANCED_FACE('',(#1294),#10625,.F.);
#11033=ADVANCED_FACE('',(#1295),#892,.T.);
#11034=ADVANCED_FACE('',(#1296),#10626,.F.);
#11035=ADVANCED_FACE('',(#1297),#95,.F.);
#11036=ADVANCED_FACE('',(#1298),#893,.T.);
#11037=ADVANCED_FACE('',(#1299),#96,.T.);
#11038=ADVANCED_FACE('',(#1300),#216,.T.);
#11039=ADVANCED_FACE('',(#1301),#10627,.T.);
#11040=ADVANCED_FACE('',(#1302),#10628,.T.);
#11041=ADVANCED_FACE('',(#1303),#894,.F.);
#11042=ADVANCED_FACE('',(#1304),#97,.F.);
#11043=ADVANCED_FACE('',(#1305),#98,.F.);
#11044=ADVANCED_FACE('',(#1306),#99,.F.);
#11045=ADVANCED_FACE('',(#1307),#100,.T.);
#11046=ADVANCED_FACE('',(#1308),#895,.T.);
#11047=ADVANCED_FACE('',(#1309),#101,.F.);
#11048=ADVANCED_FACE('',(#1310),#102,.F.);
#11049=ADVANCED_FACE('',(#1311),#896,.T.);
#11050=ADVANCED_FACE('',(#1312),#31,.T.);
#11051=ADVANCED_FACE('',(#1313),#32,.F.);
#11052=ADVANCED_FACE('',(#1314),#10629,.F.);
#11053=ADVANCED_FACE('',(#1315),#10630,.T.);
#11054=ADVANCED_FACE('',(#1316),#897,.F.);
#11055=ADVANCED_FACE('',(#1317),#10631,.T.);
#11056=ADVANCED_FACE('',(#1318),#103,.T.);
#11057=ADVANCED_FACE('',(#1319),#104,.F.);
#11058=ADVANCED_FACE('',(#1320),#105,.T.);
#11059=ADVANCED_FACE('',(#1321),#106,.F.);
#11060=ADVANCED_FACE('',(#1322),#107,.T.);
#11061=ADVANCED_FACE('',(#1323),#898,.F.);
#11062=ADVANCED_FACE('',(#1324),#10632,.T.);
#11063=ADVANCED_FACE('',(#1325),#10633,.T.);
#11064=ADVANCED_FACE('',(#1326),#899,.T.);
#11065=ADVANCED_FACE('',(#1327),#10634,.F.);
#11066=ADVANCED_FACE('',(#1328),#900,.T.);
#11067=ADVANCED_FACE('',(#1329),#108,.F.);
#11068=ADVANCED_FACE('',(#1330),#901,.T.);
#11069=ADVANCED_FACE('',(#1331),#10635,.T.);
#11070=ADVANCED_FACE('',(#1332),#109,.F.);
#11071=ADVANCED_FACE('',(#1333),#902,.F.);
#11072=ADVANCED_FACE('',(#1334),#10636,.T.);
#11073=ADVANCED_FACE('',(#1335),#903,.T.);
#11074=ADVANCED_FACE('',(#1336),#110,.F.);
#11075=ADVANCED_FACE('',(#1337),#111,.F.);
#11076=ADVANCED_FACE('',(#1338),#10637,.T.);
#11077=ADVANCED_FACE('',(#1339),#112,.T.);
#11078=ADVANCED_FACE('',(#1340),#33,.F.);
#11079=ADVANCED_FACE('',(#1341),#34,.T.);
#11080=ADVANCED_FACE('',(#1342),#113,.F.);
#11081=ADVANCED_FACE('',(#1343),#904,.T.);
#11082=ADVANCED_FACE('',(#1344),#10638,.T.);
#11083=ADVANCED_FACE('',(#1345),#905,.T.);
#11084=ADVANCED_FACE('',(#1346),#35,.F.);
#11085=ADVANCED_FACE('',(#1347),#36,.T.);
#11086=ADVANCED_FACE('',(#1348),#217,.T.);
#11087=ADVANCED_FACE('',(#1349),#114,.T.);
#11088=ADVANCED_FACE('',(#1350),#906,.T.);
#11089=ADVANCED_FACE('',(#1351),#115,.F.);
#11090=ADVANCED_FACE('',(#1352),#10639,.F.);
#11091=ADVANCED_FACE('',(#1353),#907,.T.);
#11092=ADVANCED_FACE('',(#1354),#10640,.F.);
#11093=ADVANCED_FACE('',(#1355),#10641,.T.);
#11094=ADVANCED_FACE('',(#1356),#908,.T.);
#11095=ADVANCED_FACE('',(#1357),#10642,.F.);
#11096=ADVANCED_FACE('',(#1358),#10643,.F.);
#11097=ADVANCED_FACE('',(#1359),#909,.T.);
#11098=ADVANCED_FACE('',(#1360),#910,.T.);
#11099=ADVANCED_FACE('',(#1361),#116,.F.);
#11100=ADVANCED_FACE('',(#1362),#911,.T.);
#11101=ADVANCED_FACE('',(#1363),#10644,.T.);
#11102=ADVANCED_FACE('',(#1364),#117,.T.);
#11103=ADVANCED_FACE('',(#1365),#118,.F.);
#11104=ADVANCED_FACE('',(#1366),#119,.F.);
#11105=ADVANCED_FACE('',(#1367),#912,.T.);
#11106=ADVANCED_FACE('',(#1368),#120,.F.);
#11107=ADVANCED_FACE('',(#1369),#121,.T.);
#11108=ADVANCED_FACE('',(#1370),#122,.F.);
#11109=ADVANCED_FACE('',(#1371),#123,.T.);
#11110=ADVANCED_FACE('',(#1372),#913,.T.);
#11111=ADVANCED_FACE('',(#1373),#10645,.T.);
#11112=ADVANCED_FACE('',(#1374),#914,.F.);
#11113=ADVANCED_FACE('',(#1375),#10646,.T.);
#11114=ADVANCED_FACE('',(#1376),#10647,.F.);
#11115=ADVANCED_FACE('',(#1377),#10648,.T.);
#11116=ADVANCED_FACE('',(#1378),#915,.F.);
#11117=ADVANCED_FACE('',(#1379),#124,.F.);
#11118=ADVANCED_FACE('',(#1380),#916,.T.);
#11119=ADVANCED_FACE('',(#1381),#125,.F.);
#11120=ADVANCED_FACE('',(#1382),#126,.F.);
#11121=ADVANCED_FACE('',(#1383),#37,.T.);
#11122=ADVANCED_FACE('',(#1384),#38,.F.);
#11123=ADVANCED_FACE('',(#1385),#10649,.F.);
#11124=ADVANCED_FACE('',(#1386),#10650,.T.);
#11125=ADVANCED_FACE('',(#1387),#917,.F.);
#11126=ADVANCED_FACE('',(#1388),#10651,.F.);
#11127=ADVANCED_FACE('',(#1389),#10652,.F.);
#11128=ADVANCED_FACE('',(#1390),#127,.F.);
#11129=ADVANCED_FACE('',(#1391),#918,.T.);
#11130=ADVANCED_FACE('',(#1392),#10653,.F.);
#11131=ADVANCED_FACE('',(#1393),#919,.T.);
#11132=ADVANCED_FACE('',(#1394),#128,.F.);
#11133=ADVANCED_FACE('',(#1395),#39,.F.);
#11134=ADVANCED_FACE('',(#1396),#920,.F.);
#11135=ADVANCED_FACE('',(#1397),#10654,.T.);
#11136=ADVANCED_FACE('',(#1398),#921,.T.);
#11137=ADVANCED_FACE('',(#1399),#129,.F.);
#11138=ADVANCED_FACE('',(#1400),#922,.T.);
#11139=ADVANCED_FACE('',(#1401),#10655,.T.);
#11140=ADVANCED_FACE('',(#1402),#130,.F.);
#11141=ADVANCED_FACE('',(#1403),#131,.F.);
#11142=ADVANCED_FACE('',(#1404),#40,.T.);
#11143=ADVANCED_FACE('',(#1405),#10656,.F.);
#11144=ADVANCED_FACE('',(#1406),#10657,.T.);
#11145=ADVANCED_FACE('',(#1407),#923,.T.);
#11146=ADVANCED_FACE('',(#1408),#132,.T.);
#11147=ADVANCED_FACE('',(#1409),#924,.T.);
#11148=ADVANCED_FACE('',(#1410),#133,.F.);
#11149=ADVANCED_FACE('',(#1411),#10658,.T.);
#11150=ADVANCED_FACE('',(#1412),#134,.F.);
#11151=ADVANCED_FACE('',(#1413),#10659,.T.);
#11152=ADVANCED_FACE('',(#1414),#135,.T.);
#11153=ADVANCED_FACE('',(#1415),#136,.T.);
#11154=ADVANCED_FACE('',(#1416),#925,.F.);
#11155=ADVANCED_FACE('',(#1417),#10660,.T.);
#11156=ADVANCED_FACE('',(#1418),#926,.T.);
#11157=ADVANCED_FACE('',(#1419),#10661,.T.);
#11158=ADVANCED_FACE('',(#1420),#137,.F.);
#11159=ADVANCED_FACE('',(#1421),#138,.F.);
#11160=ADVANCED_FACE('',(#1422),#927,.T.);
#11161=ADVANCED_FACE('',(#1423),#139,.F.);
#11162=ADVANCED_FACE('',(#1424),#928,.T.);
#11163=ADVANCED_FACE('',(#1425),#140,.T.);
#11164=ADVANCED_FACE('',(#1426),#218,.T.);
#11165=ADVANCED_FACE('',(#1427),#10662,.F.);
#11166=ADVANCED_FACE('',(#1428),#10663,.T.);
#11167=ADVANCED_FACE('',(#1429),#929,.T.);
#11168=ADVANCED_FACE('',(#1430),#930,.T.);
#11169=ADVANCED_FACE('',(#1431),#10664,.T.);
#11170=ADVANCED_FACE('',(#1432),#931,.T.);
#11171=ADVANCED_FACE('',(#1433),#141,.F.);
#11172=ADVANCED_FACE('',(#1434),#142,.T.);
#11173=ADVANCED_FACE('',(#1435),#143,.T.);
#11174=ADVANCED_FACE('',(#1436),#41,.T.);
#11175=ADVANCED_FACE('',(#1437),#10665,.F.);
#11176=ADVANCED_FACE('',(#1438),#144,.F.);
#11177=ADVANCED_FACE('',(#1439),#145,.F.);
#11178=ADVANCED_FACE('',(#1440),#10666,.T.);
#11179=ADVANCED_FACE('',(#1441),#42,.F.);
#11180=ADVANCED_FACE('',(#1442),#146,.F.);
#11181=ADVANCED_FACE('',(#1443),#932,.F.);
#11182=ADVANCED_FACE('',(#1444),#10667,.F.);
#11183=ADVANCED_FACE('',(#1445),#43,.F.);
#11184=ADVANCED_FACE('',(#1446),#44,.F.);
#11185=ADVANCED_FACE('',(#1447),#933,.F.);
#11186=ADVANCED_FACE('',(#1448),#934,.F.);
#11187=ADVANCED_FACE('',(#1449),#10668,.F.);
#11188=ADVANCED_FACE('',(#1450),#45,.F.);
#11189=ADVANCED_FACE('',(#1451),#46,.F.);
#11190=ADVANCED_FACE('',(#1452),#147,.T.);
#11191=ADVANCED_FACE('',(#1453),#935,.F.);
#11192=ADVANCED_FACE('',(#1454),#148,.F.);
#11193=ADVANCED_FACE('',(#1455),#936,.F.);
#11194=ADVANCED_FACE('',(#1456),#10669,.F.);
#11195=ADVANCED_FACE('',(#1457),#937,.F.);
#11196=ADVANCED_FACE('',(#1458),#149,.T.);
#11197=ADVANCED_FACE('',(#1459),#10670,.T.);
#11198=ADVANCED_FACE('',(#1460),#10671,.F.);
#11199=ADVANCED_FACE('',(#1461),#47,.F.);
#11200=ADVANCED_FACE('',(#1462),#48,.F.);
#11201=ADVANCED_FACE('',(#1463),#49,.F.);
#11202=ADVANCED_FACE('',(#1464),#150,.T.);
#11203=ADVANCED_FACE('',(#1465),#938,.T.);
#11204=ADVANCED_FACE('',(#1466),#50,.F.);
#11205=ADVANCED_FACE('',(#1467),#10672,.F.);
#11206=ADVANCED_FACE('',(#1468),#939,.F.);
#11207=ADVANCED_FACE('',(#1469),#151,.F.);
#11208=ADVANCED_FACE('',(#1470),#10673,.F.);
#11209=ADVANCED_FACE('',(#1471),#10674,.T.);
#11210=ADVANCED_FACE('',(#1472),#10675,.T.);
#11211=ADVANCED_FACE('',(#1473),#940,.F.);
#11212=ADVANCED_FACE('',(#1474),#10676,.F.);
#11213=ADVANCED_FACE('',(#1475),#152,.T.);
#11214=ADVANCED_FACE('',(#1476),#51,.F.);
#11215=ADVANCED_FACE('',(#1477),#941,.F.);
#11216=ADVANCED_FACE('',(#1478),#942,.T.);
#11217=ADVANCED_FACE('',(#1479),#153,.T.);
#11218=ADVANCED_FACE('',(#1480),#52,.F.);
#11219=ADVANCED_FACE('',(#1481),#10677,.F.);
#11220=ADVANCED_FACE('',(#1482),#10678,.T.);
#11221=ADVANCED_FACE('',(#1483),#154,.T.);
#11222=ADVANCED_FACE('',(#1484),#943,.F.);
#11223=ADVANCED_FACE('',(#1485),#10679,.F.);
#11224=ADVANCED_FACE('',(#1486),#10680,.F.);
#11225=ADVANCED_FACE('',(#1487),#944,.F.);
#11226=ADVANCED_FACE('',(#1488),#10681,.T.);
#11227=ADVANCED_FACE('',(#1489),#155,.T.);
#11228=ADVANCED_FACE('',(#1490),#945,.F.);
#11229=ADVANCED_FACE('',(#1491),#10682,.F.);
#11230=ADVANCED_FACE('',(#1492),#156,.F.);
#11231=ADVANCED_FACE('',(#1493),#53,.F.);
#11232=ADVANCED_FACE('',(#1494),#946,.T.);
#11233=ADVANCED_FACE('',(#1495),#157,.T.);
#11234=ADVANCED_FACE('',(#1496),#54,.F.);
#11235=ADVANCED_FACE('',(#1497),#158,.T.);
#11236=ADVANCED_FACE('',(#1498),#159,.T.);
#11237=ADVANCED_FACE('',(#1499),#55,.F.);
#11238=ADVANCED_FACE('',(#1500),#56,.F.);
#11239=ADVANCED_FACE('',(#1501),#947,.F.);
#11240=ADVANCED_FACE('',(#1502),#10683,.T.);
#11241=ADVANCED_FACE('',(#1503),#10684,.T.);
#11242=ADVANCED_FACE('',(#1504),#10685,.F.);
#11243=ADVANCED_FACE('',(#1505),#10686,.F.);
#11244=ADVANCED_FACE('',(#1506),#160,.T.);
#11245=ADVANCED_FACE('',(#1507),#10687,.T.);
#11246=ADVANCED_FACE('',(#1508),#948,.F.);
#11247=ADVANCED_FACE('',(#1509),#10688,.F.);
#11248=ADVANCED_FACE('',(#1510),#10689,.F.);
#11249=ADVANCED_FACE('',(#1511),#949,.F.);
#11250=ADVANCED_FACE('',(#1512),#161,.T.);
#11251=ADVANCED_FACE('',(#1513),#950,.T.);
#11252=ADVANCED_FACE('',(#1514),#57,.F.);
#11253=ADVANCED_FACE('',(#1515),#58,.F.);
#11254=ADVANCED_FACE('',(#1516),#162,.T.);
#11255=ADVANCED_FACE('',(#1517),#951,.T.);
#11256=ADVANCED_FACE('',(#1518),#59,.F.);
#11257=ADVANCED_FACE('',(#1519),#60,.F.);
#11258=ADVANCED_FACE('',(#1520),#163,.T.);
#11259=ADVANCED_FACE('',(#1521),#10690,.T.);
#11260=ADVANCED_FACE('',(#1522),#952,.F.);
#11261=ADVANCED_FACE('',(#1523),#164,.F.);
#11262=ADVANCED_FACE('',(#1524),#10691,.F.);
#11263=ADVANCED_FACE('',(#1525),#953,.F.);
#11264=ADVANCED_FACE('',(#1526),#10692,.F.);
#11265=ADVANCED_FACE('',(#1527),#954,.F.);
#11266=ADVANCED_FACE('',(#1528),#10693,.T.);
#11267=ADVANCED_FACE('',(#1529),#10694,.T.);
#11268=ADVANCED_FACE('',(#1530),#10695,.F.);
#11269=ADVANCED_FACE('',(#1531),#165,.F.);
#11270=ADVANCED_FACE('',(#1532),#955,.F.);
#11271=ADVANCED_FACE('',(#1533),#166,.T.);
#11272=ADVANCED_FACE('',(#1534),#167,.T.);
#11273=ADVANCED_FACE('',(#1535),#61,.F.);
#11274=ADVANCED_FACE('',(#1536),#62,.F.);
#11275=ADVANCED_FACE('',(#1537),#63,.F.);
#11276=ADVANCED_FACE('',(#1538),#956,.T.);
#11277=ADVANCED_FACE('',(#1539),#168,.T.);
#11278=ADVANCED_FACE('',(#1540),#64,.F.);
#11279=ADVANCED_FACE('',(#1541),#10696,.T.);
#11280=ADVANCED_FACE('',(#1542),#169,.T.);
#11281=ADVANCED_FACE('',(#1543),#957,.F.);
#11282=ADVANCED_FACE('',(#1544),#10697,.F.);
#11283=ADVANCED_FACE('',(#1545),#10698,.F.);
#11284=ADVANCED_FACE('',(#1546),#10699,.T.);
#11285=ADVANCED_FACE('',(#1547),#170,.T.);
#11286=ADVANCED_FACE('',(#1548),#958,.F.);
#11287=ADVANCED_FACE('',(#1549),#10700,.F.);
#11288=ADVANCED_FACE('',(#1550),#10701,.F.);
#11289=ADVANCED_FACE('',(#1551),#959,.T.);
#11290=ADVANCED_FACE('',(#1552),#171,.T.);
#11291=ADVANCED_FACE('',(#1553),#65,.F.);
#11292=ADVANCED_FACE('',(#1554),#172,.T.);
#11293=ADVANCED_FACE('',(#1555),#66,.F.);
#11294=ADVANCED_FACE('',(#1556),#960,.F.);
#11295=ADVANCED_FACE('',(#1557),#10702,.T.);
#11296=ADVANCED_FACE('',(#1558),#10703,.T.);
#11297=ADVANCED_FACE('',(#1559),#961,.F.);
#11298=ADVANCED_FACE('',(#1560),#173,.F.);
#11299=ADVANCED_FACE('',(#1561),#10704,.F.);
#11300=ADVANCED_FACE('',(#1562),#962,.F.);
#11301=ADVANCED_FACE('',(#1563),#10705,.F.);
#11302=ADVANCED_FACE('',(#1564),#10706,.F.);
#11303=ADVANCED_FACE('',(#1565),#963,.F.);
#11304=ADVANCED_FACE('',(#1566),#174,.T.);
#11305=ADVANCED_FACE('',(#1567),#964,.T.);
#11306=ADVANCED_FACE('',(#1568),#67,.F.);
#11307=ADVANCED_FACE('',(#1569),#68,.F.);
#11308=ADVANCED_FACE('',(#1570),#69,.F.);
#11309=ADVANCED_FACE('',(#1571),#70,.F.);
#11310=ADVANCED_FACE('',(#1572),#175,.T.);
#11311=ADVANCED_FACE('',(#1573),#10707,.T.);
#11312=ADVANCED_FACE('',(#1574),#10708,.F.);
#11313=ADVANCED_FACE('',(#1575),#10709,.F.);
#11314=ADVANCED_FACE('',(#1576),#10710,.F.);
#11315=ADVANCED_FACE('',(#1577),#176,.F.);
#11316=ADVANCED_FACE('',(#1578),#177,.T.);
#11317=ADVANCED_FACE('',(#1579),#965,.F.);
#11318=ADVANCED_FACE('',(#1580),#71,.F.);
#11319=ADVANCED_FACE('',(#1581),#72,.F.);
#11320=ADVANCED_FACE('',(#1582),#966,.F.);
#11321=ADVANCED_FACE('',(#1583),#10711,.F.);
#11322=ADVANCED_FACE('',(#1584),#10712,.F.);
#11323=ADVANCED_FACE('',(#1585),#73,.F.);
#11324=ADVANCED_FACE('',(#1586),#74,.F.);
#11325=ADVANCED_FACE('',(#1587),#178,.F.);
#11326=ADVANCED_FACE('',(#1588),#219,.T.);
#11327=ADVANCED_FACE('',(#1589),#220,.T.);
#11328=ADVANCED_FACE('',(#1590),#221,.T.);
#11329=ADVANCED_FACE('',(#1591),#222,.T.);
#11330=ADVANCED_FACE('',(#1592),#223,.T.);
#11331=ADVANCED_FACE('',(#1593),#224,.T.);
#11332=ADVANCED_FACE('',(#1594),#225,.T.);
#11333=ADVANCED_FACE('',(#1595),#226,.T.);
#11334=ADVANCED_FACE('',(#1596),#227,.T.);
#11335=ADVANCED_FACE('',(#1597),#228,.T.);
#11336=ADVANCED_FACE('',(#1598),#229,.T.);
#11337=ADVANCED_FACE('',(#1599),#230,.T.);
#11338=ADVANCED_FACE('',(#1600),#231,.T.);
#11339=ADVANCED_FACE('',(#1601),#232,.T.);
#11340=ADVANCED_FACE('',(#1602),#233,.T.);
#11341=ADVANCED_FACE('',(#1603),#234,.T.);
#11342=ADVANCED_FACE('',(#1604),#235,.T.);
#11343=ADVANCED_FACE('',(#1605),#236,.T.);
#11344=ADVANCED_FACE('',(#1606),#237,.T.);
#11345=ADVANCED_FACE('',(#1607),#238,.T.);
#11346=ADVANCED_FACE('',(#1608),#10713,.T.);
#11347=ADVANCED_FACE('',(#1609),#179,.T.);
#11348=ADVANCED_FACE('',(#1610),#180,.T.);
#11349=ADVANCED_FACE('',(#1611),#181,.F.);
#11350=ADVANCED_FACE('',(#1612),#182,.F.);
#11351=ADVANCED_FACE('',(#1613),#967,.T.);
#11352=ADVANCED_FACE('',(#1614),#10714,.T.);
#11353=ADVANCED_FACE('',(#1615),#968,.T.);
#11354=ADVANCED_FACE('',(#1616),#239,.T.);
#11355=ADVANCED_FACE('',(#1617),#183,.T.);
#11356=ADVANCED_FACE('',(#1618),#184,.T.);
#11357=ADVANCED_FACE('',(#1619),#185,.T.);
#11358=ADVANCED_FACE('',(#1620),#186,.F.);
#11359=ADVANCED_FACE('',(#1621),#969,.T.);
#11360=ADVANCED_FACE('',(#1622),#970,.T.);
#11361=ADVANCED_FACE('',(#1623),#187,.F.);
#11362=ADVANCED_FACE('',(#1624),#188,.F.);
#11363=ADVANCED_FACE('',(#1625),#971,.T.);
#11364=ADVANCED_FACE('',(#1626),#10715,.T.);
#11365=ADVANCED_FACE('',(#1627),#189,.F.);
#11366=ADVANCED_FACE('',(#1628),#240,.T.);
#11367=ADVANCED_FACE('',(#1629),#241,.T.);
#11368=ADVANCED_FACE('',(#1630),#190,.T.);
#11369=ADVANCED_FACE('',(#1631),#191,.T.);
#11370=ADVANCED_FACE('',(#1632),#972,.T.);
#11371=ADVANCED_FACE('',(#1633),#973,.T.);
#11372=ADVANCED_FACE('',(#1634),#192,.F.);
#11373=ADVANCED_FACE('',(#1635),#10716,.T.);
#11374=ADVANCED_FACE('',(#1636),#974,.T.);
#11375=ADVANCED_FACE('',(#1637),#242,.T.);
#11376=ADVANCED_FACE('',(#1638),#193,.T.);
#11377=ADVANCED_FACE('',(#1639),#194,.F.);
#11378=ADVANCED_FACE('',(#1640),#975,.T.);
#11379=ADVANCED_FACE('',(#1641),#10717,.T.);
#11380=ADVANCED_FACE('',(#1642),#10718,.T.);
#11381=ADVANCED_FACE('',(#1643),#976,.T.);
#11382=ADVANCED_FACE('',(#1644),#977,.T.);
#11383=ADVANCED_FACE('',(#1645),#10719,.T.);
#11384=ADVANCED_FACE('',(#1646),#10720,.T.);
#11385=ADVANCED_FACE('',(#1647),#978,.T.);
#11386=ADVANCED_FACE('',(#1648),#979,.T.);
#11387=ADVANCED_FACE('',(#1649),#10721,.T.);
#11388=ADVANCED_FACE('',(#1650),#10722,.T.);
#11389=ADVANCED_FACE('',(#1651),#980,.T.);
#11390=ADVANCED_FACE('',(#1652),#981,.T.);
#11391=ADVANCED_FACE('',(#1653),#10723,.T.);
#11392=ADVANCED_FACE('',(#1654),#10724,.T.);
#11393=ADVANCED_FACE('',(#1655),#982,.T.);
#11394=ADVANCED_FACE('',(#1656),#983,.T.);
#11395=ADVANCED_FACE('',(#1657),#984,.T.);
#11396=ADVANCED_FACE('',(#1658),#10725,.T.);
#11397=ADVANCED_FACE('',(#1659),#10726,.T.);
#11398=ADVANCED_FACE('',(#1660),#985,.T.);
#11399=ADVANCED_FACE('',(#1661),#986,.T.);
#11400=ADVANCED_FACE('',(#1662),#987,.T.);
#11401=ADVANCED_FACE('',(#1663),#988,.F.);
#11402=ADVANCED_FACE('',(#1664),#989,.F.);
#11403=ADVANCED_FACE('',(#1665),#10727,.F.);
#11404=ADVANCED_FACE('',(#1666),#10728,.F.);
#11405=ADVANCED_FACE('',(#1667),#990,.F.);
#11406=ADVANCED_FACE('',(#1668),#991,.F.);
#11407=ADVANCED_FACE('',(#1669),#992,.F.);
#11408=ADVANCED_FACE('',(#1670),#993,.T.);
#11409=ADVANCED_FACE('',(#1671),#994,.T.);
#11410=ADVANCED_FACE('',(#1672),#10729,.T.);
#11411=ADVANCED_FACE('',(#1673),#10730,.T.);
#11412=ADVANCED_FACE('',(#1674),#995,.T.);
#11413=ADVANCED_FACE('',(#1675),#996,.T.);
#11414=ADVANCED_FACE('',(#1676),#997,.F.);
#11415=ADVANCED_FACE('',(#1677),#998,.F.);
#11416=ADVANCED_FACE('',(#1678),#10731,.F.);
#11417=ADVANCED_FACE('',(#1679),#10732,.F.);
#11418=ADVANCED_FACE('',(#1680),#999,.F.);
#11419=ADVANCED_FACE('',(#1681),#1000,.F.);
#11420=ADVANCED_FACE('',(#1682),#1001,.T.);
#11421=ADVANCED_FACE('',(#1683),#1002,.T.);
#11422=ADVANCED_FACE('',(#1684),#10733,.T.);
#11423=ADVANCED_FACE('',(#1685),#10734,.T.);
#11424=ADVANCED_FACE('',(#1686),#1003,.T.);
#11425=ADVANCED_FACE('',(#1687),#1004,.T.);
#11426=ADVANCED_FACE('',(#1688),#1005,.F.);
#11427=ADVANCED_FACE('',(#1689),#1006,.F.);
#11428=ADVANCED_FACE('',(#1690),#10735,.F.);
#11429=ADVANCED_FACE('',(#1691),#10736,.F.);
#11430=ADVANCED_FACE('',(#1692),#1007,.F.);
#11431=ADVANCED_FACE('',(#1693),#1008,.F.);
#11432=ADVANCED_FACE('',(#1694),#10737,.F.);
#11433=ADVANCED_FACE('',(#1695),#391,.F.);
#11434=ADVANCED_FACE('',(#1696),#392,.T.);
#11435=ADVANCED_FACE('',(#1697),#10738,.T.);
#11436=ADVANCED_FACE('',(#1698,#309),#393,.T.);
#11437=ADVANCED_FACE('',(#1699,#310),#394,.T.);
#11438=ADVANCED_FACE('',(#1700,#311),#395,.F.);
#11439=ADVANCED_FACE('',(#1701),#396,.F.);
#11440=ADVANCED_FACE('',(#1702),#397,.F.);
#11441=ADVANCED_FACE('',(#1703),#398,.F.);
#11442=ADVANCED_FACE('',(#1704),#399,.F.);
#11443=ADVANCED_FACE('',(#1705),#400,.T.);
#11444=ADVANCED_FACE('',(#1706),#401,.T.);
#11445=ADVANCED_FACE('',(#1707),#402,.T.);
#11446=ADVANCED_FACE('',(#1708),#403,.F.);
#11447=ADVANCED_FACE('',(#1709),#404,.F.);
#11448=ADVANCED_FACE('',(#1710),#405,.T.);
#11449=ADVANCED_FACE('',(#1711),#406,.T.);
#11450=ADVANCED_FACE('',(#1712),#407,.T.);
#11451=ADVANCED_FACE('',(#1713),#408,.T.);
#11452=ADVANCED_FACE('',(#1714),#409,.F.);
#11453=ADVANCED_FACE('',(#1715),#410,.T.);
#11454=ADVANCED_FACE('',(#1716),#411,.F.);
#11455=ADVANCED_FACE('',(#1717),#412,.F.);
#11456=ADVANCED_FACE('',(#1718),#413,.F.);
#11497=CLOSED_SHELL('',(#10750,#10751,#10752,#10753,#10754,#10755,#10756,
#10757,#10758,#10759,#10760,#10761,#10762,#10763,#10764,#10765,#10766,#10767,
#10768,#10769,#10770,#10771,#10772,#10773,#10774,#10775,#10776,#10777,#10778,
#10779,#10780,#10781,#10782,#10783,#10784,#10785,#10786,#10787,#10788,#10789,
#10790,#10791,#10792,#10793,#10794,#10795,#10796,#10797,#10798,#10799,#10800,
#10801,#10802,#10803,#10804,#10805,#10806,#10807,#10808,#10809,#10810,#10811,
#10812,#10813,#10814,#10815,#10816,#10817,#10818,#10819,#10820,#10821,#10822,
#10823,#10824,#10825,#10826,#10827,#10828,#10829,#10830,#10831,#10832,#10833,
#10834,#10835,#10836,#10837,#10838,#10839,#10840,#10841,#10842,#10843,#10844,
#10845,#10846,#10847,#10848,#10849,#10850,#10851,#10852,#10853,#10854,#10855,
#10856,#10857,#10858,#10859,#10860,#10861,#10862,#10863,#10864,#10865,#10866,
#10867,#10868,#10869,#10870,#10871,#10872,#10873,#10874,#10875,#10876,#10877,
#10878,#10879,#10880,#10881,#10882,#10883,#10884,#10885,#10886,#10887,#10888,
#10889,#10890,#10891,#10892,#10893,#10894,#10895,#10896,#10897,#10898,#10899,
#10900,#10901,#10902,#10903,#10904,#10905,#10906,#10907,#10908,#10909,#10910,
#10911,#10912,#10913,#10914,#10915,#10916,#10917,#10918,#10919,#10920,#10921,
#10922,#10923,#10924,#10925,#10926,#10927,#10928,#10929,#10930,#10931,#10932,
#10933,#10934,#10935,#10936,#10937,#10938,#10939,#10940,#10941,#10942,#10943,
#10944,#10945,#10946,#10947,#10948,#10949,#10950,#10951,#10952,#10953,#10954,
#10955,#10956,#10957,#10958,#10959,#10960,#10961,#10962,#10963,#10964,#10965,
#10966,#10967,#10968,#10969,#10970,#10971,#10972,#10973,#10974,#10975,#10976,
#10977,#10978,#10979,#10980,#10981,#10982,#10983,#10984,#10985,#10986,#10987,
#10988,#10989,#10990,#10991,#10992,#10993,#10994,#10995,#10996,#10997,#10998,
#10999,#11000,#11001,#11002,#11003,#11004,#11005,#11006,#11007,#11008,#11009,
#11010,#11011,#11012,#11013,#11014,#11015,#11016,#11017,#11018,#11019,#11020,
#11021,#11022,#11023,#11024,#11025,#11026,#11027,#11028,#11029,#11030,#11031,
#11032,#11033,#11034,#11035,#11036,#11037,#11038,#11039,#11040,#11041,#11042,
#11043,#11044,#11045,#11046,#11047,#11048,#11049,#11050,#11051,#11052,#11053,
#11054,#11055,#11056,#11057,#11058,#11059,#11060,#11061,#11062,#11063,#11064,
#11065,#11066,#11067,#11068,#11069,#11070,#11071,#11072,#11073,#11074,#11075,
#11076,#11077,#11078,#11079,#11080,#11081,#11082,#11083,#11084,#11085,#11086,
#11087,#11088,#11089,#11090,#11091,#11092,#11093,#11094,#11095,#11096,#11097,
#11098,#11099,#11100,#11101,#11102,#11103,#11104,#11105,#11106,#11107,#11108,
#11109,#11110,#11111,#11112,#11113,#11114,#11115,#11116,#11117,#11118,#11119,
#11120,#11121,#11122,#11123,#11124,#11125,#11126,#11127,#11128,#11129,#11130,
#11131,#11132,#11133,#11134,#11135,#11136,#11137,#11138,#11139,#11140,#11141,
#11142,#11143,#11144,#11145,#11146,#11147,#11148,#11149,#11150,#11151,#11152,
#11153,#11154,#11155,#11156,#11157,#11158,#11159,#11160,#11161,#11162,#11163,
#11164,#11165,#11166,#11167,#11168,#11169,#11170,#11171,#11172,#11173,#11174,
#11175,#11176,#11177,#11178,#11179,#11180,#11181,#11182,#11183,#11184,#11185,
#11186,#11187,#11188,#11189,#11190,#11191,#11192,#11193,#11194,#11195,#11196,
#11197,#11198,#11199,#11200,#11201,#11202,#11203,#11204,#11205,#11206,#11207,
#11208,#11209,#11210,#11211,#11212,#11213,#11214,#11215,#11216,#11217,#11218,
#11219,#11220,#11221,#11222,#11223,#11224,#11225,#11226,#11227,#11228,#11229,
#11230,#11231,#11232,#11233,#11234,#11235,#11236,#11237,#11238,#11239,#11240,
#11241,#11242,#11243,#11244,#11245,#11246,#11247,#11248,#11249,#11250,#11251,
#11252,#11253,#11254,#11255,#11256,#11257,#11258,#11259,#11260,#11261,#11262,
#11263,#11264,#11265,#11266,#11267,#11268,#11269,#11270,#11271,#11272,#11273,
#11274,#11275,#11276,#11277,#11278,#11279,#11280,#11281,#11282,#11283,#11284,
#11285,#11286,#11287,#11288,#11289,#11290,#11291,#11292,#11293,#11294,#11295,
#11296,#11297,#11298,#11299,#11300,#11301,#11302,#11303,#11304,#11305,#11306,
#11307,#11308,#11309,#11310,#11311,#11312,#11313,#11314,#11315,#11316,#11317,
#11318,#11319,#11320,#11321,#11322,#11323,#11324,#11325,#11326,#11327,#11328,
#11329,#11330,#11331,#11332,#11333,#11334,#11335,#11336,#11337,#11338,#11339,
#11340,#11341,#11342,#11343,#11344,#11345,#11346,#11347,#11348,#11349,#11350,
#11351,#11352,#11353,#11354,#11355,#11356,#11357,#11358,#11359,#11360,#11361,
#11362,#11363,#11364,#11365,#11366,#11367,#11368,#11369,#11370,#11371,#11372,
#11373,#11374,#11375,#11376,#11377,#11378,#11379,#11380,#11381,#11382,#11383,
#11384,#11385,#11386,#11387,#11388,#11389,#11390,#11391,#11392,#11393,#11394,
#11395,#11396,#11397,#11398,#11399,#11400,#11401,#11402,#11403,#11404,#11405,
#11406,#11407,#11408,#11409,#11410,#11411,#11412,#11413,#11414,#11415,#11416,
#11417,#11418,#11419,#11420,#11421,#11422,#11423,#11424,#11425,#11426,#11427,
#11428,#11429,#11430,#11431,#11432,#11433,#11434,#11435,#11436,#11437,#11438,
#11439,#11440,#11441,#11442,#11443,#11444,#11445,#11446,#11447,#11448,#11449,
#11450,#11451,#11452,#11453,#11454,#11455,#11456));
#11523=AXIS2_PLACEMENT_3D('',#16374,#12995,#12996);
#11524=AXIS2_PLACEMENT_3D('',#16375,#12997,#12998);
#11525=AXIS2_PLACEMENT_3D('',#16377,#12999,#13000);
#11526=AXIS2_PLACEMENT_3D('',#16380,#13002,#13003);
#11527=AXIS2_PLACEMENT_3D('',#16381,#13004,#13005);
#11528=AXIS2_PLACEMENT_3D('',#16383,#13006,#13007);
#11529=AXIS2_PLACEMENT_3D('',#16386,#13009,#13010);
#11530=AXIS2_PLACEMENT_3D('',#16387,#13011,#13012);
#11531=AXIS2_PLACEMENT_3D('',#16389,#13013,#13014);
#11532=AXIS2_PLACEMENT_3D('',#16392,#13016,#13017);
#11533=AXIS2_PLACEMENT_3D('',#16393,#13018,#13019);
#11534=AXIS2_PLACEMENT_3D('',#16395,#13020,#13021);
#11535=AXIS2_PLACEMENT_3D('',#16398,#13023,#13024);
#11536=AXIS2_PLACEMENT_3D('',#16399,#13025,#13026);
#11537=AXIS2_PLACEMENT_3D('',#16402,#13027,#13028);
#11538=AXIS2_PLACEMENT_3D('',#16403,#13029,#13030);
#11539=AXIS2_PLACEMENT_3D('',#16405,#13031,#13032);
#11540=AXIS2_PLACEMENT_3D('',#16406,#13033,#13034);
#11541=AXIS2_PLACEMENT_3D('',#16407,#13035,#13036);
#11542=AXIS2_PLACEMENT_3D('',#16409,#13037,#13038);
#11543=AXIS2_PLACEMENT_3D('',#16411,#13039,#13040);
#11544=AXIS2_PLACEMENT_3D('',#16413,#13041,#13042);
#11545=AXIS2_PLACEMENT_3D('',#16414,#13043,#13044);
#11546=AXIS2_PLACEMENT_3D('',#16415,#13045,#13046);
#11547=AXIS2_PLACEMENT_3D('',#16417,#13047,#13048);
#11548=AXIS2_PLACEMENT_3D('',#16419,#13049,#13050);
#11549=AXIS2_PLACEMENT_3D('',#16420,#13051,#13052);
#11550=AXIS2_PLACEMENT_3D('',#16421,#13053,#13054);
#11551=AXIS2_PLACEMENT_3D('',#16423,#13055,#13056);
#11552=AXIS2_PLACEMENT_3D('',#16425,#13057,#13058);
#11553=AXIS2_PLACEMENT_3D('',#16427,#13059,#13060);
#11554=AXIS2_PLACEMENT_3D('',#16428,#13061,#13062);
#11555=AXIS2_PLACEMENT_3D('',#16429,#13063,#13064);
#11556=AXIS2_PLACEMENT_3D('',#16432,#13065,#13066);
#11557=AXIS2_PLACEMENT_3D('',#16434,#13067,#13068);
#11558=AXIS2_PLACEMENT_3D('',#16436,#13069,#13070);
#11559=AXIS2_PLACEMENT_3D('',#16437,#13071,#13072);
#11560=AXIS2_PLACEMENT_3D('',#16438,#13073,#13074);
#11561=AXIS2_PLACEMENT_3D('',#16441,#13075,#13076);
#11562=AXIS2_PLACEMENT_3D('',#16443,#13077,#13078);
#11563=AXIS2_PLACEMENT_3D('',#16445,#13079,#13080);
#11564=AXIS2_PLACEMENT_3D('',#16446,#13081,#13082);
#11565=AXIS2_PLACEMENT_3D('',#16447,#13083,#13084);
#11566=AXIS2_PLACEMENT_3D('',#16450,#13085,#13086);
#11567=AXIS2_PLACEMENT_3D('',#16452,#13087,#13088);
#11568=AXIS2_PLACEMENT_3D('',#16454,#13089,#13090);
#11569=AXIS2_PLACEMENT_3D('',#16455,#13091,#13092);
#11570=AXIS2_PLACEMENT_3D('',#16456,#13093,#13094);
#11571=AXIS2_PLACEMENT_3D('',#16459,#13095,#13096);
#11572=AXIS2_PLACEMENT_3D('',#16461,#13097,#13098);
#11573=AXIS2_PLACEMENT_3D('',#16463,#13099,#13100);
#11574=AXIS2_PLACEMENT_3D('',#16464,#13101,#13102);
#11575=AXIS2_PLACEMENT_3D('',#16465,#13103,#13104);
#11576=AXIS2_PLACEMENT_3D('',#16468,#13105,#13106);
#11577=AXIS2_PLACEMENT_3D('',#16469,#13107,#13108);
#11578=AXIS2_PLACEMENT_3D('',#16471,#13109,#13110);
#11579=AXIS2_PLACEMENT_3D('',#16472,#13111,#13112);
#11580=AXIS2_PLACEMENT_3D('',#16473,#13113,#13114);
#11581=AXIS2_PLACEMENT_3D('',#16475,#13115,#13116);
#11582=AXIS2_PLACEMENT_3D('',#16477,#13117,#13118);
#11583=AXIS2_PLACEMENT_3D('',#16479,#13119,#13120);
#11584=AXIS2_PLACEMENT_3D('',#16480,#13121,#13122);
#11585=AXIS2_PLACEMENT_3D('',#16481,#13123,#13124);
#11586=AXIS2_PLACEMENT_3D('',#16483,#13125,#13126);
#11587=AXIS2_PLACEMENT_3D('',#16485,#13127,#13128);
#11588=AXIS2_PLACEMENT_3D('',#16487,#13129,#13130);
#11589=AXIS2_PLACEMENT_3D('',#16488,#13131,#13132);
#11590=AXIS2_PLACEMENT_3D('',#16489,#13133,#13134);
#11591=AXIS2_PLACEMENT_3D('',#16491,#13135,#13136);
#11592=AXIS2_PLACEMENT_3D('',#16493,#13137,#13138);
#11593=AXIS2_PLACEMENT_3D('',#16495,#13139,#13140);
#11594=AXIS2_PLACEMENT_3D('',#16496,#13141,#13142);
#11595=AXIS2_PLACEMENT_3D('',#16497,#13143,#13144);
#11596=AXIS2_PLACEMENT_3D('',#16500,#13145,#13146);
#11597=AXIS2_PLACEMENT_3D('',#16502,#13147,#13148);
#11598=AXIS2_PLACEMENT_3D('',#16504,#13149,#13150);
#11599=AXIS2_PLACEMENT_3D('',#16505,#13151,#13152);
#11600=AXIS2_PLACEMENT_3D('',#16506,#13153,#13154);
#11601=AXIS2_PLACEMENT_3D('',#16509,#13155,#13156);
#11602=AXIS2_PLACEMENT_3D('',#16511,#13157,#13158);
#11603=AXIS2_PLACEMENT_3D('',#16513,#13159,#13160);
#11604=AXIS2_PLACEMENT_3D('',#16514,#13161,#13162);
#11605=AXIS2_PLACEMENT_3D('',#16515,#13163,#13164);
#11606=AXIS2_PLACEMENT_3D('',#16518,#13165,#13166);
#11607=AXIS2_PLACEMENT_3D('',#16520,#13167,#13168);
#11608=AXIS2_PLACEMENT_3D('',#16522,#13169,#13170);
#11609=AXIS2_PLACEMENT_3D('',#16523,#13171,#13172);
#11610=AXIS2_PLACEMENT_3D('',#16524,#13173,#13174);
#11611=AXIS2_PLACEMENT_3D('',#16527,#13175,#13176);
#11612=AXIS2_PLACEMENT_3D('',#16529,#13177,#13178);
#11613=AXIS2_PLACEMENT_3D('',#16531,#13179,#13180);
#11614=AXIS2_PLACEMENT_3D('',#16532,#13181,#13182);
#11615=AXIS2_PLACEMENT_3D('',#16533,#13183,#13184);
#11616=AXIS2_PLACEMENT_3D('',#16535,#13185,#13186);
#11617=AXIS2_PLACEMENT_3D('',#16537,#13187,#13188);
#11618=AXIS2_PLACEMENT_3D('',#16538,#13189,#13190);
#11619=AXIS2_PLACEMENT_3D('',#16539,#13191,#13192);
#11620=AXIS2_PLACEMENT_3D('',#16541,#13193,#13194);
#11621=AXIS2_PLACEMENT_3D('',#16543,#13195,#13196);
#11622=AXIS2_PLACEMENT_3D('',#16544,#13197,#13198);
#11623=AXIS2_PLACEMENT_3D('',#16545,#13199,#13200);
#11624=AXIS2_PLACEMENT_3D('',#16547,#13201,#13202);
#11625=AXIS2_PLACEMENT_3D('',#16549,#13203,#13204);
#11626=AXIS2_PLACEMENT_3D('',#16551,#13205,#13206);
#11627=AXIS2_PLACEMENT_3D('',#16552,#13207,#13208);
#11628=AXIS2_PLACEMENT_3D('',#16553,#13209,#13210);
#11629=AXIS2_PLACEMENT_3D('',#16555,#13211,#13212);
#11630=AXIS2_PLACEMENT_3D('',#16557,#13213,#13214);
#11631=AXIS2_PLACEMENT_3D('',#16558,#13215,#13216);
#11632=AXIS2_PLACEMENT_3D('',#16559,#13217,#13218);
#11633=AXIS2_PLACEMENT_3D('',#16562,#13219,#13220);
#11634=AXIS2_PLACEMENT_3D('',#16564,#13221,#13222);
#11635=AXIS2_PLACEMENT_3D('',#16566,#13223,#13224);
#11636=AXIS2_PLACEMENT_3D('',#16567,#13225,#13226);
#11637=AXIS2_PLACEMENT_3D('',#16568,#13227,#13228);
#11638=AXIS2_PLACEMENT_3D('',#16571,#13229,#13230);
#11639=AXIS2_PLACEMENT_3D('',#16573,#13231,#13232);
#11640=AXIS2_PLACEMENT_3D('',#16575,#13233,#13234);
#11641=AXIS2_PLACEMENT_3D('',#16576,#13235,#13236);
#11642=AXIS2_PLACEMENT_3D('',#16577,#13237,#13238);
#11643=AXIS2_PLACEMENT_3D('',#16580,#13239,#13240);
#11644=AXIS2_PLACEMENT_3D('',#16582,#13241,#13242);
#11645=AXIS2_PLACEMENT_3D('',#16583,#13243,#13244);
#11646=AXIS2_PLACEMENT_3D('',#16584,#13245,#13246);
#11647=AXIS2_PLACEMENT_3D('',#16585,#13247,#13248);
#11648=AXIS2_PLACEMENT_3D('',#16587,#13249,#13250);
#11649=AXIS2_PLACEMENT_3D('',#16589,#13251,#13252);
#11650=AXIS2_PLACEMENT_3D('',#16591,#13253,#13254);
#11651=AXIS2_PLACEMENT_3D('',#16592,#13255,#13256);
#11652=AXIS2_PLACEMENT_3D('',#16593,#13257,#13258);
#11653=AXIS2_PLACEMENT_3D('',#16595,#13259,#13260);
#11654=AXIS2_PLACEMENT_3D('',#16597,#13261,#13262);
#11655=AXIS2_PLACEMENT_3D('',#16599,#13263,#13264);
#11656=AXIS2_PLACEMENT_3D('',#16600,#13265,#13266);
#11657=AXIS2_PLACEMENT_3D('',#16601,#13267,#13268);
#11658=AXIS2_PLACEMENT_3D('',#16603,#13269,#13270);
#11659=AXIS2_PLACEMENT_3D('',#16605,#13271,#13272);
#11660=AXIS2_PLACEMENT_3D('',#16607,#13273,#13274);
#11661=AXIS2_PLACEMENT_3D('',#16608,#13275,#13276);
#11662=AXIS2_PLACEMENT_3D('',#16609,#13277,#13278);
#11663=AXIS2_PLACEMENT_3D('',#16612,#13279,#13280);
#11664=AXIS2_PLACEMENT_3D('',#16614,#13281,#13282);
#11665=AXIS2_PLACEMENT_3D('',#16616,#13283,#13284);
#11666=AXIS2_PLACEMENT_3D('',#16617,#13285,#13286);
#11667=AXIS2_PLACEMENT_3D('',#16618,#13287,#13288);
#11668=AXIS2_PLACEMENT_3D('',#16621,#13289,#13290);
#11669=AXIS2_PLACEMENT_3D('',#16623,#13291,#13292);
#11670=AXIS2_PLACEMENT_3D('',#16625,#13293,#13294);
#11671=AXIS2_PLACEMENT_3D('',#16626,#13295,#13296);
#11672=AXIS2_PLACEMENT_3D('',#16627,#13297,#13298);
#11673=AXIS2_PLACEMENT_3D('',#16630,#13299,#13300);
#11674=AXIS2_PLACEMENT_3D('',#16632,#13301,#13302);
#11675=AXIS2_PLACEMENT_3D('',#16634,#13303,#13304);
#11676=AXIS2_PLACEMENT_3D('',#16635,#13305,#13306);
#11677=AXIS2_PLACEMENT_3D('',#16636,#13307,#13308);
#11678=AXIS2_PLACEMENT_3D('',#16639,#13309,#13310);
#11679=AXIS2_PLACEMENT_3D('',#16641,#13311,#13312);
#11680=AXIS2_PLACEMENT_3D('',#16643,#13313,#13314);
#11681=AXIS2_PLACEMENT_3D('',#16644,#13315,#13316);
#11682=AXIS2_PLACEMENT_3D('',#16645,#13317,#13318);
#11683=AXIS2_PLACEMENT_3D('',#16648,#13319,#13320);
#11684=AXIS2_PLACEMENT_3D('',#16650,#13321,#13322);
#11685=AXIS2_PLACEMENT_3D('',#16652,#13323,#13324);
#11686=AXIS2_PLACEMENT_3D('',#16653,#13325,#13326);
#11687=AXIS2_PLACEMENT_3D('',#16654,#13327,#13328);
#11688=AXIS2_PLACEMENT_3D('',#16657,#13329,#13330);
#11689=AXIS2_PLACEMENT_3D('',#16659,#13331,#13332);
#11690=AXIS2_PLACEMENT_3D('',#16661,#13333,#13334);
#11691=AXIS2_PLACEMENT_3D('',#16662,#13335,#13336);
#11692=AXIS2_PLACEMENT_3D('',#16663,#13337,#13338);
#11693=AXIS2_PLACEMENT_3D('',#16666,#13339,#13340);
#11694=AXIS2_PLACEMENT_3D('',#16670,#13342,#13343);
#11695=AXIS2_PLACEMENT_3D('',#16672,#13345,#13346);
#11696=AXIS2_PLACEMENT_3D('',#16675,#13347,#13348);
#11697=AXIS2_PLACEMENT_3D('',#16679,#13350,#13351);
#11698=AXIS2_PLACEMENT_3D('',#16681,#13353,#13354);
#11699=AXIS2_PLACEMENT_3D('',#16684,#13355,#13356);
#11700=AXIS2_PLACEMENT_3D('',#16688,#13358,#13359);
#11701=AXIS2_PLACEMENT_3D('',#16690,#13361,#13362);
#11702=AXIS2_PLACEMENT_3D('',#16692,#13363,#13364);
#11703=AXIS2_PLACEMENT_3D('',#16694,#13365,#13366);
#11704=AXIS2_PLACEMENT_3D('',#16695,#13367,#13368);
#11705=AXIS2_PLACEMENT_3D('',#16696,#13369,#13370);
#11706=AXIS2_PLACEMENT_3D('',#16699,#13371,#13372);
#11707=AXIS2_PLACEMENT_3D('',#16703,#13374,#13375);
#11708=AXIS2_PLACEMENT_3D('',#16705,#13377,#13378);
#11709=AXIS2_PLACEMENT_3D('',#16708,#13379,#13380);
#11710=AXIS2_PLACEMENT_3D('',#16712,#13382,#13383);
#11711=AXIS2_PLACEMENT_3D('',#16714,#13385,#13386);
#11712=AXIS2_PLACEMENT_3D('',#16717,#13387,#13388);
#11713=AXIS2_PLACEMENT_3D('',#16721,#13390,#13391);
#11714=AXIS2_PLACEMENT_3D('',#16723,#13393,#13394);
#11715=AXIS2_PLACEMENT_3D('',#16726,#13395,#13396);
#11716=AXIS2_PLACEMENT_3D('',#16730,#13398,#13399);
#11717=AXIS2_PLACEMENT_3D('',#16732,#13401,#13402);
#11718=AXIS2_PLACEMENT_3D('',#16735,#13403,#13404);
#11719=AXIS2_PLACEMENT_3D('',#16737,#13405,#13406);
#11720=AXIS2_PLACEMENT_3D('',#16739,#13407,#13408);
#11721=AXIS2_PLACEMENT_3D('',#16740,#13409,#13410);
#11722=AXIS2_PLACEMENT_3D('',#16741,#13411,#13412);
#11723=AXIS2_PLACEMENT_3D('',#16744,#13413,#13414);
#11724=AXIS2_PLACEMENT_3D('',#16746,#13415,#13416);
#11725=AXIS2_PLACEMENT_3D('',#16748,#13417,#13418);
#11726=AXIS2_PLACEMENT_3D('',#16749,#13419,#13420);
#11727=AXIS2_PLACEMENT_3D('',#16750,#13421,#13422);
#11728=AXIS2_PLACEMENT_3D('',#16753,#13423,#13424);
#11729=AXIS2_PLACEMENT_3D('',#16755,#13425,#13426);
#11730=AXIS2_PLACEMENT_3D('',#16757,#13427,#13428);
#11731=AXIS2_PLACEMENT_3D('',#16758,#13429,#13430);
#11732=AXIS2_PLACEMENT_3D('',#16759,#13431,#13432);
#11733=AXIS2_PLACEMENT_3D('',#16762,#13433,#13434);
#11734=AXIS2_PLACEMENT_3D('',#16766,#13436,#13437);
#11735=AXIS2_PLACEMENT_3D('',#16768,#13439,#13440);
#11736=AXIS2_PLACEMENT_3D('',#16770,#13441,#13442);
#11737=AXIS2_PLACEMENT_3D('',#16773,#13444,#13445);
#11738=AXIS2_PLACEMENT_3D('',#16775,#13447,#13448);
#11739=AXIS2_PLACEMENT_3D('',#16777,#13450,#13451);
#11740=AXIS2_PLACEMENT_3D('',#16779,#13453,#13454);
#11741=AXIS2_PLACEMENT_3D('',#16783,#13456,#13457);
#11742=AXIS2_PLACEMENT_3D('',#16785,#13459,#13460);
#11743=AXIS2_PLACEMENT_3D('',#16788,#13461,#13462);
#11744=AXIS2_PLACEMENT_3D('',#16792,#13464,#13465);
#11745=AXIS2_PLACEMENT_3D('',#16794,#13467,#13468);
#11746=AXIS2_PLACEMENT_3D('',#16796,#13469,#13470);
#11747=AXIS2_PLACEMENT_3D('',#16799,#13472,#13473);
#11748=AXIS2_PLACEMENT_3D('',#16801,#13475,#13476);
#11749=AXIS2_PLACEMENT_3D('',#16803,#13478,#13479);
#11750=AXIS2_PLACEMENT_3D('',#16805,#13481,#13482);
#11751=AXIS2_PLACEMENT_3D('',#16816,#13483,#13484);
#11752=AXIS2_PLACEMENT_3D('',#16840,#13485,#13486);
#11753=AXIS2_PLACEMENT_3D('',#16849,#13487,#13488);
#11754=AXIS2_PLACEMENT_3D('',#16853,#13490,#13491);
#11755=AXIS2_PLACEMENT_3D('',#16855,#13493,#13494);
#11756=AXIS2_PLACEMENT_3D('',#16858,#13495,#13496);
#11757=AXIS2_PLACEMENT_3D('',#16862,#13498,#13499);
#11758=AXIS2_PLACEMENT_3D('',#16864,#13501,#13502);
#11759=AXIS2_PLACEMENT_3D('',#16867,#13505,#13506);
#11760=AXIS2_PLACEMENT_3D('',#16869,#13508,#13509);
#11761=AXIS2_PLACEMENT_3D('',#16871,#13511,#13512);
#11762=AXIS2_PLACEMENT_3D('',#16874,#13513,#13514);
#11763=AXIS2_PLACEMENT_3D('',#16885,#13515,#13516);
#11764=AXIS2_PLACEMENT_3D('',#16909,#13517,#13518);
#11765=AXIS2_PLACEMENT_3D('',#16918,#13519,#13520);
#11766=AXIS2_PLACEMENT_3D('',#16921,#13521,#13522);
#11767=AXIS2_PLACEMENT_3D('',#16924,#13525,#13526);
#11768=AXIS2_PLACEMENT_3D('',#16927,#13529,#13530);
#11769=AXIS2_PLACEMENT_3D('',#16930,#13533,#13534);
#11770=AXIS2_PLACEMENT_3D('',#16933,#13535,#13536);
#11771=AXIS2_PLACEMENT_3D('',#16935,#13537,#13538);
#11772=AXIS2_PLACEMENT_3D('',#16937,#13539,#13540);
#11773=AXIS2_PLACEMENT_3D('',#16939,#13541,#13542);
#11774=AXIS2_PLACEMENT_3D('',#16941,#13543,#13544);
#11775=AXIS2_PLACEMENT_3D('',#16943,#13545,#13546);
#11776=AXIS2_PLACEMENT_3D('',#16947,#13548,#13549);
#11777=AXIS2_PLACEMENT_3D('',#16949,#13550,#13551);
#11778=AXIS2_PLACEMENT_3D('',#17000,#13553,#13554);
#11779=AXIS2_PLACEMENT_3D('',#17036,#13556,#13557);
#11780=AXIS2_PLACEMENT_3D('',#17074,#13559,#13560);
#11781=AXIS2_PLACEMENT_3D('',#17120,#13561,#13562);
#11782=AXIS2_PLACEMENT_3D('',#17122,#13563,#13564);
#11783=AXIS2_PLACEMENT_3D('',#17124,#13565,#13566);
#11784=AXIS2_PLACEMENT_3D('',#17126,#13567,#13568);
#11785=AXIS2_PLACEMENT_3D('',#17176,#13570,#13571);
#11786=AXIS2_PLACEMENT_3D('',#17210,#13572,#13573);
#11787=AXIS2_PLACEMENT_3D('',#17249,#13575,#13576);
#11788=AXIS2_PLACEMENT_3D('',#17297,#13578,#13579);
#11789=AXIS2_PLACEMENT_3D('',#17299,#13580,#13581);
#11790=AXIS2_PLACEMENT_3D('',#17301,#13582,#13583);
#11791=AXIS2_PLACEMENT_3D('',#17303,#13584,#13585);
#11792=AXIS2_PLACEMENT_3D('',#17354,#13587,#13588);
#11793=AXIS2_PLACEMENT_3D('',#17390,#13590,#13591);
#11794=AXIS2_PLACEMENT_3D('',#17426,#13592,#13593);
#11795=AXIS2_PLACEMENT_3D('',#17474,#13595,#13596);
#11796=AXIS2_PLACEMENT_3D('',#17476,#13597,#13598);
#11797=AXIS2_PLACEMENT_3D('',#17478,#13599,#13600);
#11798=AXIS2_PLACEMENT_3D('',#17480,#13601,#13602);
#11799=AXIS2_PLACEMENT_3D('',#17528,#13603,#13604);
#11800=AXIS2_PLACEMENT_3D('',#17564,#13606,#13607);
#11801=AXIS2_PLACEMENT_3D('',#17603,#13609,#13610);
#11802=AXIS2_PLACEMENT_3D('',#17651,#13612,#13613);
#11803=AXIS2_PLACEMENT_3D('',#17652,#13614,#13615);
#11804=AXIS2_PLACEMENT_3D('',#17654,#13616,#13617);
#11805=AXIS2_PLACEMENT_3D('',#17656,#13618,#13619);
#11806=AXIS2_PLACEMENT_3D('',#17658,#13620,#13621);
#11807=AXIS2_PLACEMENT_3D('',#17660,#13622,#13623);
#11808=AXIS2_PLACEMENT_3D('',#17662,#13624,#13625);
#11809=AXIS2_PLACEMENT_3D('',#17663,#13626,#13627);
#11810=AXIS2_PLACEMENT_3D('',#17664,#13628,#13629);
#11811=AXIS2_PLACEMENT_3D('',#17666,#13631,#13632);
#11812=AXIS2_PLACEMENT_3D('',#17668,#13634,#13635);
#11813=AXIS2_PLACEMENT_3D('',#17671,#13636,#13637);
#11814=AXIS2_PLACEMENT_3D('',#17682,#13638,#13639);
#11815=AXIS2_PLACEMENT_3D('',#17706,#13640,#13641);
#11816=AXIS2_PLACEMENT_3D('',#17715,#13642,#13643);
#11817=AXIS2_PLACEMENT_3D('',#17718,#13644,#13645);
#11818=AXIS2_PLACEMENT_3D('',#17721,#13648,#13649);
#11819=AXIS2_PLACEMENT_3D('',#17724,#13650,#13651);
#11820=AXIS2_PLACEMENT_3D('',#17728,#13653,#13654);
#11821=AXIS2_PLACEMENT_3D('',#17730,#13656,#13657);
#11822=AXIS2_PLACEMENT_3D('',#17740,#13662,#13663);
#11823=AXIS2_PLACEMENT_3D('',#17742,#13664,#13665);
#11824=AXIS2_PLACEMENT_3D('',#17746,#13667,#13668);
#11825=AXIS2_PLACEMENT_3D('',#17748,#13669,#13670);
#11826=AXIS2_PLACEMENT_3D('',#17750,#13671,#13672);
#11827=AXIS2_PLACEMENT_3D('',#17760,#13677,#13678);
#11828=AXIS2_PLACEMENT_3D('',#17764,#13680,#13681);
#11829=AXIS2_PLACEMENT_3D('',#17768,#13683,#13684);
#11830=AXIS2_PLACEMENT_3D('',#17771,#13686,#13687);
#11831=AXIS2_PLACEMENT_3D('',#17774,#13688,#13689);
#11832=AXIS2_PLACEMENT_3D('',#17776,#13690,#13691);
#11833=AXIS2_PLACEMENT_3D('',#17780,#13693,#13694);
#11834=AXIS2_PLACEMENT_3D('',#17781,#13695,#13696);
#11835=AXIS2_PLACEMENT_3D('',#17784,#13698,#13699);
#11836=AXIS2_PLACEMENT_3D('',#17786,#13700,#13701);
#11837=AXIS2_PLACEMENT_3D('',#17788,#13702,#13703);
#11838=AXIS2_PLACEMENT_3D('',#17791,#13705,#13706);
#11839=AXIS2_PLACEMENT_3D('',#17793,#13707,#13708);
#11840=AXIS2_PLACEMENT_3D('',#17796,#13710,#13711);
#11841=AXIS2_PLACEMENT_3D('',#17799,#13713,#13714);
#11842=AXIS2_PLACEMENT_3D('',#17801,#13715,#13716);
#11843=AXIS2_PLACEMENT_3D('',#17804,#13718,#13719);
#11844=AXIS2_PLACEMENT_3D('',#17816,#13720,#13721);
#11845=AXIS2_PLACEMENT_3D('',#17849,#13723,#13724);
#11846=AXIS2_PLACEMENT_3D('',#17893,#13726,#13727);
#11847=AXIS2_PLACEMENT_3D('',#17926,#13729,#13730);
#11848=AXIS2_PLACEMENT_3D('',#17948,#13732,#13733);
#11849=AXIS2_PLACEMENT_3D('',#17957,#13738,#13739);
#11850=AXIS2_PLACEMENT_3D('',#17966,#13744,#13745);
#11851=AXIS2_PLACEMENT_3D('',#17983,#13753,#13754);
#11852=AXIS2_PLACEMENT_3D('',#17987,#13756,#13757);
#11853=AXIS2_PLACEMENT_3D('',#17991,#13759,#13760);
#11854=AXIS2_PLACEMENT_3D('',#17995,#13762,#13763);
#11855=AXIS2_PLACEMENT_3D('',#18003,#13768,#13769);
#11856=AXIS2_PLACEMENT_3D('',#18010,#13772,#13773);
#11857=AXIS2_PLACEMENT_3D('',#18014,#13775,#13776);
#11858=AXIS2_PLACEMENT_3D('',#18019,#13779,#13780);
#11859=AXIS2_PLACEMENT_3D('',#18033,#13788,#13789);
#11860=AXIS2_PLACEMENT_3D('',#18040,#13794,#13795);
#11861=AXIS2_PLACEMENT_3D('',#18041,#13796,#13797);
#11862=AXIS2_PLACEMENT_3D('',#18042,#13798,#13799);
#11863=AXIS2_PLACEMENT_3D('',#18043,#13800,#13801);
#11864=AXIS2_PLACEMENT_3D('',#18044,#13802,#13803);
#11865=AXIS2_PLACEMENT_3D('',#18045,#13804,#13805);
#11866=AXIS2_PLACEMENT_3D('',#18046,#13806,#13807);
#11867=AXIS2_PLACEMENT_3D('',#18050,#13809,#13810);
#11868=AXIS2_PLACEMENT_3D('',#18051,#13811,#13812);
#11869=AXIS2_PLACEMENT_3D('',#18052,#13813,#13814);
#11870=AXIS2_PLACEMENT_3D('',#18053,#13815,#13816);
#11871=AXIS2_PLACEMENT_3D('',#18054,#13817,#13818);
#11872=AXIS2_PLACEMENT_3D('',#18055,#13819,#13820);
#11873=AXIS2_PLACEMENT_3D('',#18056,#13821,#13822);
#11874=AXIS2_PLACEMENT_3D('',#18057,#13823,#13824);
#11875=AXIS2_PLACEMENT_3D('',#18059,#13825,#13826);
#11876=AXIS2_PLACEMENT_3D('',#18061,#13828,#13829);
#11877=AXIS2_PLACEMENT_3D('',#18070,#13834,#13835);
#11878=AXIS2_PLACEMENT_3D('',#18072,#13836,#13837);
#11879=AXIS2_PLACEMENT_3D('',#18075,#13839,#13840);
#11880=AXIS2_PLACEMENT_3D('',#18076,#13841,#13842);
#11881=AXIS2_PLACEMENT_3D('',#18078,#13843,#13844);
#11882=AXIS2_PLACEMENT_3D('',#18080,#13845,#13846);
#11883=AXIS2_PLACEMENT_3D('',#18082,#13848,#13849);
#11884=AXIS2_PLACEMENT_3D('',#18087,#13851,#13852);
#11885=AXIS2_PLACEMENT_3D('',#18089,#13853,#13854);
#11886=AXIS2_PLACEMENT_3D('',#18093,#13857,#13858);
#11887=AXIS2_PLACEMENT_3D('',#18096,#13859,#13860);
#11888=AXIS2_PLACEMENT_3D('',#18098,#13861,#13862);
#11889=AXIS2_PLACEMENT_3D('',#18170,#13864,#13865);
#11890=AXIS2_PLACEMENT_3D('',#18173,#13866,#13867);
#11891=AXIS2_PLACEMENT_3D('',#18175,#13868,#13869);
#11892=AXIS2_PLACEMENT_3D('',#18247,#13871,#13872);
#11893=AXIS2_PLACEMENT_3D('',#18250,#13873,#13874);
#11894=AXIS2_PLACEMENT_3D('',#18252,#13875,#13876);
#11895=AXIS2_PLACEMENT_3D('',#18324,#13878,#13879);
#11896=AXIS2_PLACEMENT_3D('',#18327,#13880,#13881);
#11897=AXIS2_PLACEMENT_3D('',#18329,#13882,#13883);
#11898=AXIS2_PLACEMENT_3D('',#18401,#13885,#13886);
#11899=AXIS2_PLACEMENT_3D('',#18404,#13887,#13888);
#11900=AXIS2_PLACEMENT_3D('',#18456,#13889,#13890);
#11901=AXIS2_PLACEMENT_3D('',#18458,#13891,#13892);
#11902=AXIS2_PLACEMENT_3D('',#18469,#13893,#13894);
#11903=AXIS2_PLACEMENT_3D('',#18470,#13895,#13896);
#11904=AXIS2_PLACEMENT_3D('',#18471,#13897,#13898);
#11905=AXIS2_PLACEMENT_3D('',#18477,#13901,#13902);
#11906=AXIS2_PLACEMENT_3D('',#18479,#13903,#13904);
#11907=AXIS2_PLACEMENT_3D('',#18483,#13906,#13907);
#11908=AXIS2_PLACEMENT_3D('',#18487,#13909,#13910);
#11909=AXIS2_PLACEMENT_3D('',#18489,#13911,#13912);
#11910=AXIS2_PLACEMENT_3D('',#18493,#13914,#13915);
#11911=AXIS2_PLACEMENT_3D('',#18497,#13917,#13918);
#11912=AXIS2_PLACEMENT_3D('',#18499,#13919,#13920);
#11913=AXIS2_PLACEMENT_3D('',#18503,#13922,#13923);
#11914=AXIS2_PLACEMENT_3D('',#18506,#13925,#13926);
#11915=AXIS2_PLACEMENT_3D('',#18510,#13928,#13929);
#11916=AXIS2_PLACEMENT_3D('',#18517,#13933,#13934);
#11917=AXIS2_PLACEMENT_3D('',#18518,#13935,#13936);
#11918=AXIS2_PLACEMENT_3D('',#18519,#13937,#13938);
#11919=AXIS2_PLACEMENT_3D('',#18562,#13942,#13943);
#11920=AXIS2_PLACEMENT_3D('',#18564,#13945,#13946);
#11921=AXIS2_PLACEMENT_3D('',#18575,#13951,#13952);
#11922=AXIS2_PLACEMENT_3D('',#18606,#13954,#13955);
#11923=AXIS2_PLACEMENT_3D('',#18609,#13956,#13957);
#11924=AXIS2_PLACEMENT_3D('',#18672,#13958,#13959);
#11925=AXIS2_PLACEMENT_3D('',#18674,#13960,#13961);
#11926=AXIS2_PLACEMENT_3D('',#18676,#13962,#13963);
#11927=AXIS2_PLACEMENT_3D('',#18732,#13964,#13965);
#11928=AXIS2_PLACEMENT_3D('',#18744,#13966,#13967);
#11929=AXIS2_PLACEMENT_3D('',#18755,#13968,#13969);
#11930=AXIS2_PLACEMENT_3D('',#18777,#13970,#13971);
#11931=AXIS2_PLACEMENT_3D('',#18778,#13972,#13973);
#11932=AXIS2_PLACEMENT_3D('',#18783,#13975,#13976);
#11933=AXIS2_PLACEMENT_3D('',#18786,#13978,#13979);
#11934=AXIS2_PLACEMENT_3D('',#18787,#13980,#13981);
#11935=AXIS2_PLACEMENT_3D('',#18788,#13982,#13983);
#11936=AXIS2_PLACEMENT_3D('',#18789,#13984,#13985);
#11937=AXIS2_PLACEMENT_3D('',#18790,#13986,#13987);
#11938=AXIS2_PLACEMENT_3D('',#18795,#13989,#13990);
#11939=AXIS2_PLACEMENT_3D('',#18799,#13992,#13993);
#11940=AXIS2_PLACEMENT_3D('',#18829,#13994,#13995);
#11941=AXIS2_PLACEMENT_3D('',#18830,#13996,#13997);
#11942=AXIS2_PLACEMENT_3D('',#18835,#13999,#14000);
#11943=AXIS2_PLACEMENT_3D('',#18839,#14002,#14003);
#11944=AXIS2_PLACEMENT_3D('',#18881,#14004,#14005);
#11945=AXIS2_PLACEMENT_3D('',#18882,#14006,#14007);
#11946=AXIS2_PLACEMENT_3D('',#18887,#14009,#14010);
#11947=AXIS2_PLACEMENT_3D('',#18891,#14012,#14013);
#11948=AXIS2_PLACEMENT_3D('',#18895,#14016,#14017);
#11949=AXIS2_PLACEMENT_3D('',#18896,#14018,#14019);
#11950=AXIS2_PLACEMENT_3D('',#18901,#14021,#14022);
#11951=AXIS2_PLACEMENT_3D('',#18905,#14024,#14025);
#11952=AXIS2_PLACEMENT_3D('',#18909,#14027,#14028);
#11953=AXIS2_PLACEMENT_3D('',#18912,#14030,#14031);
#11954=AXIS2_PLACEMENT_3D('',#18913,#14032,#14033);
#11955=AXIS2_PLACEMENT_3D('',#19026,#14039,#14040);
#11956=AXIS2_PLACEMENT_3D('',#19154,#14046,#14047);
#11957=AXIS2_PLACEMENT_3D('',#19155,#14048,#14049);
#11958=AXIS2_PLACEMENT_3D('',#19156,#14050,#14051);
#11959=AXIS2_PLACEMENT_3D('',#19157,#14052,#14053);
#11960=AXIS2_PLACEMENT_3D('',#19231,#14059,#14060);
#11961=AXIS2_PLACEMENT_3D('',#19290,#14066,#14067);
#11962=AXIS2_PLACEMENT_3D('',#19361,#14074,#14075);
#11963=AXIS2_PLACEMENT_3D('',#19394,#14077,#14078);
#11964=AXIS2_PLACEMENT_3D('',#19454,#14080,#14081);
#11965=AXIS2_PLACEMENT_3D('',#19455,#14082,#14083);
#11966=AXIS2_PLACEMENT_3D('',#19468,#14090,#14091);
#11967=AXIS2_PLACEMENT_3D('',#19472,#14093,#14094);
#11968=AXIS2_PLACEMENT_3D('',#19476,#14096,#14097);
#11969=AXIS2_PLACEMENT_3D('',#19479,#14099,#14100);
#11970=AXIS2_PLACEMENT_3D('',#19482,#14101,#14102);
#11971=AXIS2_PLACEMENT_3D('',#19542,#14104,#14105);
#11972=AXIS2_PLACEMENT_3D('',#19544,#14106,#14107);
#11973=AXIS2_PLACEMENT_3D('',#19604,#14109,#14110);
#11974=AXIS2_PLACEMENT_3D('',#19640,#14112,#14113);
#11975=AXIS2_PLACEMENT_3D('',#19699,#14115,#14116);
#11976=AXIS2_PLACEMENT_3D('',#19759,#14118,#14119);
#11977=AXIS2_PLACEMENT_3D('',#19795,#14121,#14122);
#11978=AXIS2_PLACEMENT_3D('',#19797,#14123,#14124);
#11979=AXIS2_PLACEMENT_3D('',#19857,#14126,#14127);
#11980=AXIS2_PLACEMENT_3D('',#19893,#14129,#14130);
#11981=AXIS2_PLACEMENT_3D('',#19951,#14132,#14133);
#11982=AXIS2_PLACEMENT_3D('',#19952,#14134,#14135);
#11983=AXIS2_PLACEMENT_3D('',#19953,#14136,#14137);
#11984=AXIS2_PLACEMENT_3D('',#19954,#14138,#14139);
#11985=AXIS2_PLACEMENT_3D('',#19966,#14140,#14141);
#11986=AXIS2_PLACEMENT_3D('',#19976,#14142,#14143);
#11987=AXIS2_PLACEMENT_3D('',#19977,#14144,#14145);
#11988=AXIS2_PLACEMENT_3D('',#19980,#14146,#14147);
#11989=AXIS2_PLACEMENT_3D('',#20053,#14149,#14150);
#11990=AXIS2_PLACEMENT_3D('',#20054,#14151,#14152);
#11991=AXIS2_PLACEMENT_3D('',#20057,#14153,#14154);
#11992=AXIS2_PLACEMENT_3D('',#20130,#14156,#14157);
#11993=AXIS2_PLACEMENT_3D('',#20131,#14158,#14159);
#11994=AXIS2_PLACEMENT_3D('',#20143,#14163,#14164);
#11995=AXIS2_PLACEMENT_3D('',#20158,#14169,#14170);
#11996=AXIS2_PLACEMENT_3D('',#20163,#14172,#14173);
#11997=AXIS2_PLACEMENT_3D('',#20166,#14175,#14176);
#11998=AXIS2_PLACEMENT_3D('',#20167,#14177,#14178);
#11999=AXIS2_PLACEMENT_3D('',#20172,#14180,#14181);
#12000=AXIS2_PLACEMENT_3D('',#20175,#14183,#14184);
#12001=AXIS2_PLACEMENT_3D('',#20176,#14185,#14186);
#12002=AXIS2_PLACEMENT_3D('',#20189,#14189,#14190);
#12003=AXIS2_PLACEMENT_3D('',#20194,#14192,#14193);
#12004=AXIS2_PLACEMENT_3D('',#20197,#14195,#14196);
#12005=AXIS2_PLACEMENT_3D('',#20198,#14197,#14198);
#12006=AXIS2_PLACEMENT_3D('',#20208,#14201,#14202);
#12007=AXIS2_PLACEMENT_3D('',#20210,#14203,#14204);
#12008=AXIS2_PLACEMENT_3D('',#20213,#14206,#14207);
#12009=AXIS2_PLACEMENT_3D('',#20214,#14208,#14209);
#12010=AXIS2_PLACEMENT_3D('',#20220,#14213,#14214);
#12011=AXIS2_PLACEMENT_3D('',#20229,#14219,#14220);
#12012=AXIS2_PLACEMENT_3D('',#20231,#14221,#14222);
#12013=AXIS2_PLACEMENT_3D('',#20234,#14224,#14225);
#12014=AXIS2_PLACEMENT_3D('',#20236,#14226,#14227);
#12015=AXIS2_PLACEMENT_3D('',#20239,#14229,#14230);
#12016=AXIS2_PLACEMENT_3D('',#20240,#14231,#14232);
#12017=AXIS2_PLACEMENT_3D('',#20241,#14233,#14234);
#12018=AXIS2_PLACEMENT_3D('',#20242,#14235,#14236);
#12019=AXIS2_PLACEMENT_3D('',#20243,#14237,#14238);
#12020=AXIS2_PLACEMENT_3D('',#20244,#14239,#14240);
#12021=AXIS2_PLACEMENT_3D('',#20245,#14241,#14242);
#12022=AXIS2_PLACEMENT_3D('',#20246,#14243,#14244);
#12023=AXIS2_PLACEMENT_3D('',#20247,#14245,#14246);
#12024=AXIS2_PLACEMENT_3D('',#20248,#14247,#14248);
#12025=AXIS2_PLACEMENT_3D('',#20249,#14249,#14250);
#12026=AXIS2_PLACEMENT_3D('',#20252,#14251,#14252);
#12027=AXIS2_PLACEMENT_3D('',#20304,#14253,#14254);
#12028=AXIS2_PLACEMENT_3D('',#20306,#14255,#14256);
#12029=AXIS2_PLACEMENT_3D('',#20317,#14257,#14258);
#12030=AXIS2_PLACEMENT_3D('',#20318,#14259,#14260);
#12031=AXIS2_PLACEMENT_3D('',#20319,#14261,#14262);
#12032=AXIS2_PLACEMENT_3D('',#20364,#14267,#14268);
#12033=AXIS2_PLACEMENT_3D('',#20366,#14270,#14271);
#12034=AXIS2_PLACEMENT_3D('',#20374,#14275,#14276);
#12035=AXIS2_PLACEMENT_3D('',#20405,#14278,#14279);
#12036=AXIS2_PLACEMENT_3D('',#20408,#14280,#14281);
#12037=AXIS2_PLACEMENT_3D('',#20471,#14282,#14283);
#12038=AXIS2_PLACEMENT_3D('',#20473,#14284,#14285);
#12039=AXIS2_PLACEMENT_3D('',#20475,#14286,#14287);
#12040=AXIS2_PLACEMENT_3D('',#20531,#14288,#14289);
#12041=AXIS2_PLACEMENT_3D('',#20536,#14291,#14292);
#12042=AXIS2_PLACEMENT_3D('',#20539,#14294,#14295);
#12043=AXIS2_PLACEMENT_3D('',#20540,#14296,#14297);
#12044=AXIS2_PLACEMENT_3D('',#20545,#14299,#14300);
#12045=AXIS2_PLACEMENT_3D('',#20549,#14302,#14303);
#12046=AXIS2_PLACEMENT_3D('',#20591,#14304,#14305);
#12047=AXIS2_PLACEMENT_3D('',#20592,#14306,#14307);
#12048=AXIS2_PLACEMENT_3D('',#20597,#14309,#14310);
#12049=AXIS2_PLACEMENT_3D('',#20601,#14312,#14313);
#12050=AXIS2_PLACEMENT_3D('',#20605,#14316,#14317);
#12051=AXIS2_PLACEMENT_3D('',#20606,#14318,#14319);
#12052=AXIS2_PLACEMENT_3D('',#20611,#14321,#14322);
#12053=AXIS2_PLACEMENT_3D('',#20615,#14324,#14325);
#12054=AXIS2_PLACEMENT_3D('',#20619,#14327,#14328);
#12055=AXIS2_PLACEMENT_3D('',#20622,#14330,#14331);
#12056=AXIS2_PLACEMENT_3D('',#20623,#14332,#14333);
#12057=AXIS2_PLACEMENT_3D('',#20736,#14339,#14340);
#12058=AXIS2_PLACEMENT_3D('',#20737,#14341,#14342);
#12059=AXIS2_PLACEMENT_3D('',#20738,#14343,#14344);
#12060=AXIS2_PLACEMENT_3D('',#20739,#14345,#14346);
#12061=AXIS2_PLACEMENT_3D('',#20813,#14352,#14353);
#12062=AXIS2_PLACEMENT_3D('',#20814,#14354,#14355);
#12063=AXIS2_PLACEMENT_3D('',#20815,#14356,#14357);
#12064=AXIS2_PLACEMENT_3D('',#20816,#14358,#14359);
#12065=AXIS2_PLACEMENT_3D('',#20828,#14360,#14361);
#12066=AXIS2_PLACEMENT_3D('',#20838,#14362,#14363);
#12067=AXIS2_PLACEMENT_3D('',#20839,#14364,#14365);
#12068=AXIS2_PLACEMENT_3D('',#20842,#14366,#14367);
#12069=AXIS2_PLACEMENT_3D('',#20915,#14369,#14370);
#12070=AXIS2_PLACEMENT_3D('',#20916,#14371,#14372);
#12071=AXIS2_PLACEMENT_3D('',#20931,#14377,#14378);
#12072=AXIS2_PLACEMENT_3D('',#20943,#14382,#14383);
#12073=AXIS2_PLACEMENT_3D('',#20946,#14385,#14386);
#12074=AXIS2_PLACEMENT_3D('',#20947,#14387,#14388);
#12075=AXIS2_PLACEMENT_3D('',#20948,#14389,#14390);
#12076=AXIS2_PLACEMENT_3D('',#20953,#14392,#14393);
#12077=AXIS2_PLACEMENT_3D('',#20956,#14395,#14396);
#12078=AXIS2_PLACEMENT_3D('',#20957,#14397,#14398);
#12079=AXIS2_PLACEMENT_3D('',#20970,#14401,#14402);
#12080=AXIS2_PLACEMENT_3D('',#20975,#14404,#14405);
#12081=AXIS2_PLACEMENT_3D('',#20978,#14407,#14408);
#12082=AXIS2_PLACEMENT_3D('',#20979,#14409,#14410);
#12083=AXIS2_PLACEMENT_3D('',#20989,#14413,#14414);
#12084=AXIS2_PLACEMENT_3D('',#20990,#14415,#14416);
#12085=AXIS2_PLACEMENT_3D('',#20992,#14418,#14419);
#12086=AXIS2_PLACEMENT_3D('',#20993,#14420,#14421);
#12087=AXIS2_PLACEMENT_3D('',#20999,#14425,#14426);
#12088=AXIS2_PLACEMENT_3D('',#21006,#14431,#14432);
#12089=AXIS2_PLACEMENT_3D('',#21008,#14433,#14434);
#12090=AXIS2_PLACEMENT_3D('',#21012,#14436,#14437);
#12091=AXIS2_PLACEMENT_3D('',#21013,#14438,#14439);
#12092=AXIS2_PLACEMENT_3D('',#21016,#14441,#14442);
#12093=AXIS2_PLACEMENT_3D('',#21017,#14443,#14444);
#12094=AXIS2_PLACEMENT_3D('',#21018,#14445,#14446);
#12095=AXIS2_PLACEMENT_3D('',#21019,#14447,#14448);
#12096=AXIS2_PLACEMENT_3D('',#21020,#14449,#14450);
#12097=AXIS2_PLACEMENT_3D('',#21021,#14451,#14452);
#12098=AXIS2_PLACEMENT_3D('',#21022,#14453,#14454);
#12099=AXIS2_PLACEMENT_3D('',#21023,#14455,#14456);
#12100=AXIS2_PLACEMENT_3D('',#21024,#14457,#14458);
#12101=AXIS2_PLACEMENT_3D('',#21027,#14459,#14460);
#12102=AXIS2_PLACEMENT_3D('',#21079,#14461,#14462);
#12103=AXIS2_PLACEMENT_3D('',#21081,#14463,#14464);
#12104=AXIS2_PLACEMENT_3D('',#21092,#14465,#14466);
#12105=AXIS2_PLACEMENT_3D('',#21093,#14467,#14468);
#12106=AXIS2_PLACEMENT_3D('',#21094,#14469,#14470);
#12107=AXIS2_PLACEMENT_3D('',#21141,#14476,#14477);
#12108=AXIS2_PLACEMENT_3D('',#21142,#14478,#14479);
#12109=AXIS2_PLACEMENT_3D('',#21153,#14484,#14485);
#12110=AXIS2_PLACEMENT_3D('',#21184,#14487,#14488);
#12111=AXIS2_PLACEMENT_3D('',#21187,#14489,#14490);
#12112=AXIS2_PLACEMENT_3D('',#21250,#14491,#14492);
#12113=AXIS2_PLACEMENT_3D('',#21252,#14493,#14494);
#12114=AXIS2_PLACEMENT_3D('',#21254,#14495,#14496);
#12115=AXIS2_PLACEMENT_3D('',#21310,#14497,#14498);
#12116=AXIS2_PLACEMENT_3D('',#21313,#14501,#14502);
#12117=AXIS2_PLACEMENT_3D('',#21319,#14505,#14506);
#12118=AXIS2_PLACEMENT_3D('',#21361,#14507,#14508);
#12119=AXIS2_PLACEMENT_3D('',#21362,#14509,#14510);
#12120=AXIS2_PLACEMENT_3D('',#21475,#14516,#14517);
#12121=AXIS2_PLACEMENT_3D('',#21476,#14518,#14519);
#12122=AXIS2_PLACEMENT_3D('',#21477,#14520,#14521);
#12123=AXIS2_PLACEMENT_3D('',#21478,#14522,#14523);
#12124=AXIS2_PLACEMENT_3D('',#21552,#14529,#14530);
#12125=AXIS2_PLACEMENT_3D('',#21553,#14531,#14532);
#12126=AXIS2_PLACEMENT_3D('',#21554,#14533,#14534);
#12127=AXIS2_PLACEMENT_3D('',#21555,#14535,#14536);
#12128=AXIS2_PLACEMENT_3D('',#21567,#14537,#14538);
#12129=AXIS2_PLACEMENT_3D('',#21577,#14539,#14540);
#12130=AXIS2_PLACEMENT_3D('',#21578,#14541,#14542);
#12131=AXIS2_PLACEMENT_3D('',#21581,#14543,#14544);
#12132=AXIS2_PLACEMENT_3D('',#21654,#14546,#14547);
#12133=AXIS2_PLACEMENT_3D('',#21655,#14548,#14549);
#12134=AXIS2_PLACEMENT_3D('',#21670,#14554,#14555);
#12135=AXIS2_PLACEMENT_3D('',#21685,#14560,#14561);
#12136=AXIS2_PLACEMENT_3D('',#21689,#14563,#14564);
#12137=AXIS2_PLACEMENT_3D('',#21690,#14565,#14566);
#12138=AXIS2_PLACEMENT_3D('',#21691,#14567,#14568);
#12139=AXIS2_PLACEMENT_3D('',#21696,#14570,#14571);
#12140=AXIS2_PLACEMENT_3D('',#21699,#14573,#14574);
#12141=AXIS2_PLACEMENT_3D('',#21700,#14575,#14576);
#12142=AXIS2_PLACEMENT_3D('',#21713,#14579,#14580);
#12143=AXIS2_PLACEMENT_3D('',#21718,#14582,#14583);
#12144=AXIS2_PLACEMENT_3D('',#21721,#14585,#14586);
#12145=AXIS2_PLACEMENT_3D('',#21722,#14587,#14588);
#12146=AXIS2_PLACEMENT_3D('',#21729,#14590,#14591);
#12147=AXIS2_PLACEMENT_3D('',#21731,#14592,#14593);
#12148=AXIS2_PLACEMENT_3D('',#21734,#14595,#14596);
#12149=AXIS2_PLACEMENT_3D('',#21735,#14597,#14598);
#12150=AXIS2_PLACEMENT_3D('',#21741,#14602,#14603);
#12151=AXIS2_PLACEMENT_3D('',#21750,#14608,#14609);
#12152=AXIS2_PLACEMENT_3D('',#21757,#14612,#14613);
#12153=AXIS2_PLACEMENT_3D('',#21759,#14614,#14615);
#12154=AXIS2_PLACEMENT_3D('',#21761,#14616,#14617);
#12155=AXIS2_PLACEMENT_3D('',#21765,#14619,#14620);
#12156=AXIS2_PLACEMENT_3D('',#21766,#14621,#14622);
#12157=AXIS2_PLACEMENT_3D('',#21770,#14625,#14626);
#12158=AXIS2_PLACEMENT_3D('',#21771,#14627,#14628);
#12159=AXIS2_PLACEMENT_3D('',#21772,#14629,#14630);
#12160=AXIS2_PLACEMENT_3D('',#21773,#14631,#14632);
#12161=AXIS2_PLACEMENT_3D('',#21774,#14633,#14634);
#12162=AXIS2_PLACEMENT_3D('',#21775,#14635,#14636);
#12163=AXIS2_PLACEMENT_3D('',#21776,#14637,#14638);
#12164=AXIS2_PLACEMENT_3D('',#21777,#14639,#14640);
#12165=AXIS2_PLACEMENT_3D('',#21780,#14641,#14642);
#12166=AXIS2_PLACEMENT_3D('',#21832,#14643,#14644);
#12167=AXIS2_PLACEMENT_3D('',#21834,#14645,#14646);
#12168=AXIS2_PLACEMENT_3D('',#21845,#14647,#14648);
#12169=AXIS2_PLACEMENT_3D('',#21846,#14649,#14650);
#12170=AXIS2_PLACEMENT_3D('',#21847,#14651,#14652);
#12171=AXIS2_PLACEMENT_3D('',#21890,#14656,#14657);
#12172=AXIS2_PLACEMENT_3D('',#21892,#14659,#14660);
#12173=AXIS2_PLACEMENT_3D('',#21900,#14664,#14665);
#12174=AXIS2_PLACEMENT_3D('',#21931,#14667,#14668);
#12175=AXIS2_PLACEMENT_3D('',#21934,#14669,#14670);
#12176=AXIS2_PLACEMENT_3D('',#21997,#14671,#14672);
#12177=AXIS2_PLACEMENT_3D('',#21999,#14673,#14674);
#12178=AXIS2_PLACEMENT_3D('',#22001,#14675,#14676);
#12179=AXIS2_PLACEMENT_3D('',#22057,#14677,#14678);
#12180=AXIS2_PLACEMENT_3D('',#22062,#14680,#14681);
#12181=AXIS2_PLACEMENT_3D('',#22066,#14683,#14684);
#12182=AXIS2_PLACEMENT_3D('',#22070,#14686,#14687);
#12183=AXIS2_PLACEMENT_3D('',#22073,#14689,#14690);
#12184=AXIS2_PLACEMENT_3D('',#22074,#14691,#14692);
#12185=AXIS2_PLACEMENT_3D('',#22079,#14694,#14695);
#12186=AXIS2_PLACEMENT_3D('',#22083,#14697,#14698);
#12187=AXIS2_PLACEMENT_3D('',#22087,#14701,#14702);
#12188=AXIS2_PLACEMENT_3D('',#22088,#14703,#14704);
#12189=AXIS2_PLACEMENT_3D('',#22089,#14705,#14706);
#12190=AXIS2_PLACEMENT_3D('',#22090,#14707,#14708);
#12191=AXIS2_PLACEMENT_3D('',#22091,#14709,#14710);
#12192=AXIS2_PLACEMENT_3D('',#22092,#14711,#14712);
#12193=AXIS2_PLACEMENT_3D('',#22093,#14713,#14714);
#12194=AXIS2_PLACEMENT_3D('',#22094,#14715,#14716);
#12195=AXIS2_PLACEMENT_3D('',#22106,#14717,#14718);
#12196=AXIS2_PLACEMENT_3D('',#22116,#14719,#14720);
#12197=AXIS2_PLACEMENT_3D('',#22117,#14721,#14722);
#12198=AXIS2_PLACEMENT_3D('',#22132,#14727,#14728);
#12199=AXIS2_PLACEMENT_3D('',#22147,#14733,#14734);
#12200=AXIS2_PLACEMENT_3D('',#22148,#14735,#14736);
#12201=AXIS2_PLACEMENT_3D('',#22149,#14737,#14738);
#12202=AXIS2_PLACEMENT_3D('',#22150,#14739,#14740);
#12203=AXIS2_PLACEMENT_3D('',#22155,#14742,#14743);
#12204=AXIS2_PLACEMENT_3D('',#22158,#14745,#14746);
#12205=AXIS2_PLACEMENT_3D('',#22159,#14747,#14748);
#12206=AXIS2_PLACEMENT_3D('',#22169,#14750,#14751);
#12207=AXIS2_PLACEMENT_3D('',#22174,#14753,#14754);
#12208=AXIS2_PLACEMENT_3D('',#22177,#14756,#14757);
#12209=AXIS2_PLACEMENT_3D('',#22178,#14758,#14759);
#12210=AXIS2_PLACEMENT_3D('',#22188,#14762,#14763);
#12211=AXIS2_PLACEMENT_3D('',#22190,#14764,#14765);
#12212=AXIS2_PLACEMENT_3D('',#22193,#14767,#14768);
#12213=AXIS2_PLACEMENT_3D('',#22194,#14769,#14770);
#12214=AXIS2_PLACEMENT_3D('',#22200,#14774,#14775);
#12215=AXIS2_PLACEMENT_3D('',#22207,#14780,#14781);
#12216=AXIS2_PLACEMENT_3D('',#22209,#14782,#14783);
#12217=AXIS2_PLACEMENT_3D('',#22211,#14784,#14785);
#12218=AXIS2_PLACEMENT_3D('',#22215,#14787,#14788);
#12219=AXIS2_PLACEMENT_3D('',#22217,#14789,#14790);
#12220=AXIS2_PLACEMENT_3D('',#22219,#14791,#14792);
#12221=AXIS2_PLACEMENT_3D('',#22221,#14794,#14795);
#12222=AXIS2_PLACEMENT_3D('',#22222,#14796,#14797);
#12223=AXIS2_PLACEMENT_3D('',#22223,#14798,#14799);
#12224=AXIS2_PLACEMENT_3D('',#22224,#14800,#14801);
#12225=AXIS2_PLACEMENT_3D('',#22225,#14802,#14803);
#12226=AXIS2_PLACEMENT_3D('',#22226,#14804,#14805);
#12227=AXIS2_PLACEMENT_3D('',#22227,#14806,#14807);
#12228=AXIS2_PLACEMENT_3D('',#22228,#14808,#14809);
#12229=AXIS2_PLACEMENT_3D('',#22229,#14810,#14811);
#12230=AXIS2_PLACEMENT_3D('',#22230,#14812,#14813);
#12231=AXIS2_PLACEMENT_3D('',#22231,#14814,#14815);
#12232=AXIS2_PLACEMENT_3D('',#22232,#14816,#14817);
#12233=AXIS2_PLACEMENT_3D('',#22233,#14818,#14819);
#12234=AXIS2_PLACEMENT_3D('',#22234,#14820,#14821);
#12235=AXIS2_PLACEMENT_3D('',#22235,#14822,#14823);
#12236=AXIS2_PLACEMENT_3D('',#22236,#14824,#14825);
#12237=AXIS2_PLACEMENT_3D('',#22237,#14826,#14827);
#12238=AXIS2_PLACEMENT_3D('',#22238,#14828,#14829);
#12239=AXIS2_PLACEMENT_3D('',#22239,#14830,#14831);
#12240=AXIS2_PLACEMENT_3D('',#22240,#14832,#14833);
#12241=AXIS2_PLACEMENT_3D('',#22241,#14834,#14835);
#12242=AXIS2_PLACEMENT_3D('',#22242,#14836,#14837);
#12243=AXIS2_PLACEMENT_3D('',#22243,#14838,#14839);
#12244=AXIS2_PLACEMENT_3D('',#22244,#14840,#14841);
#12245=AXIS2_PLACEMENT_3D('',#22245,#14842,#14843);
#12246=AXIS2_PLACEMENT_3D('',#22246,#14844,#14845);
#12247=AXIS2_PLACEMENT_3D('',#22247,#14846,#14847);
#12248=AXIS2_PLACEMENT_3D('',#22248,#14848,#14849);
#12249=AXIS2_PLACEMENT_3D('',#22249,#14850,#14851);
#12250=AXIS2_PLACEMENT_3D('',#22250,#14852,#14853);
#12251=AXIS2_PLACEMENT_3D('',#22251,#14854,#14855);
#12252=AXIS2_PLACEMENT_3D('',#22252,#14856,#14857);
#12253=AXIS2_PLACEMENT_3D('',#22253,#14858,#14859);
#12254=AXIS2_PLACEMENT_3D('',#23068,#14860,#14861);
#12255=AXIS2_PLACEMENT_3D('',#23889,#14862,#14863);
#12256=AXIS2_PLACEMENT_3D('',#23984,#14864,#14865);
#12257=AXIS2_PLACEMENT_3D('',#24009,#14866,#14867);
#12258=AXIS2_PLACEMENT_3D('',#24092,#14868,#14869);
#12259=AXIS2_PLACEMENT_3D('',#24093,#14870,#14871);
#12260=AXIS2_PLACEMENT_3D('',#24094,#14872,#14873);
#12261=AXIS2_PLACEMENT_3D('',#24095,#14874,#14875);
#12262=AXIS2_PLACEMENT_3D('',#24096,#14876,#14877);
#12263=AXIS2_PLACEMENT_3D('',#24097,#14878,#14879);
#12264=AXIS2_PLACEMENT_3D('',#24098,#14880,#14881);
#12265=AXIS2_PLACEMENT_3D('',#24099,#14882,#14883);
#12266=AXIS2_PLACEMENT_3D('',#24100,#14884,#14885);
#12267=AXIS2_PLACEMENT_3D('',#24217,#14886,#14887);
#12268=AXIS2_PLACEMENT_3D('',#24218,#14888,#14889);
#12269=AXIS2_PLACEMENT_3D('',#24219,#14890,#14891);
#12270=AXIS2_PLACEMENT_3D('',#24238,#14892,#14893);
#12271=AXIS2_PLACEMENT_3D('',#24239,#14894,#14895);
#12272=AXIS2_PLACEMENT_3D('',#24240,#14896,#14897);
#12273=AXIS2_PLACEMENT_3D('',#24241,#14898,#14899);
#12274=AXIS2_PLACEMENT_3D('',#24266,#14900,#14901);
#12275=AXIS2_PLACEMENT_3D('',#24267,#14902,#14903);
#12276=AXIS2_PLACEMENT_3D('',#24320,#14904,#14905);
#12277=AXIS2_PLACEMENT_3D('',#24321,#14906,#14907);
#12278=AXIS2_PLACEMENT_3D('',#24459,#14908,#14909);
#12279=AXIS2_PLACEMENT_3D('',#24460,#14910,#14911);
#12280=AXIS2_PLACEMENT_3D('',#24461,#14912,#14913);
#12281=AXIS2_PLACEMENT_3D('',#24520,#14914,#14915);
#12282=AXIS2_PLACEMENT_3D('',#24521,#14916,#14917);
#12283=AXIS2_PLACEMENT_3D('',#24522,#14918,#14919);
#12284=AXIS2_PLACEMENT_3D('',#24581,#14920,#14921);
#12285=AXIS2_PLACEMENT_3D('',#24582,#14922,#14923);
#12286=AXIS2_PLACEMENT_3D('',#24583,#14924,#14925);
#12287=AXIS2_PLACEMENT_3D('',#24584,#14926,#14927);
#12288=AXIS2_PLACEMENT_3D('',#24585,#14928,#14929);
#12289=AXIS2_PLACEMENT_3D('',#24586,#14930,#14931);
#12290=AXIS2_PLACEMENT_3D('',#24587,#14932,#14933);
#12291=AXIS2_PLACEMENT_3D('',#24618,#14934,#14935);
#12292=AXIS2_PLACEMENT_3D('',#24619,#14936,#14937);
#12293=AXIS2_PLACEMENT_3D('',#24620,#14938,#14939);
#12294=AXIS2_PLACEMENT_3D('',#24633,#14940,#14941);
#12295=AXIS2_PLACEMENT_3D('',#24646,#14942,#14943);
#12296=AXIS2_PLACEMENT_3D('',#24647,#14944,#14945);
#12297=AXIS2_PLACEMENT_3D('',#24648,#14946,#14947);
#12298=AXIS2_PLACEMENT_3D('',#24649,#14948,#14949);
#12299=AXIS2_PLACEMENT_3D('',#24650,#14950,#14951);
#12300=AXIS2_PLACEMENT_3D('',#24669,#14952,#14953);
#12301=AXIS2_PLACEMENT_3D('',#24688,#14954,#14955);
#12302=AXIS2_PLACEMENT_3D('',#24689,#14956,#14957);
#12303=AXIS2_PLACEMENT_3D('',#24690,#14958,#14959);
#12304=AXIS2_PLACEMENT_3D('',#24691,#14960,#14961);
#12305=AXIS2_PLACEMENT_3D('',#24692,#14962,#14963);
#12306=AXIS2_PLACEMENT_3D('',#24693,#14964,#14965);
#12307=AXIS2_PLACEMENT_3D('',#24712,#14966,#14967);
#12308=AXIS2_PLACEMENT_3D('',#24713,#14968,#14969);
#12309=AXIS2_PLACEMENT_3D('',#24739,#14970,#14971);
#12310=AXIS2_PLACEMENT_3D('',#24740,#14972,#14973);
#12311=AXIS2_PLACEMENT_3D('',#24826,#14974,#14975);
#12312=AXIS2_PLACEMENT_3D('',#24857,#14976,#14977);
#12313=AXIS2_PLACEMENT_3D('',#24934,#14978,#14979);
#12314=AXIS2_PLACEMENT_3D('',#25029,#14980,#14981);
#12315=AXIS2_PLACEMENT_3D('',#25030,#14982,#14983);
#12316=AXIS2_PLACEMENT_3D('',#25031,#14984,#14985);
#12317=AXIS2_PLACEMENT_3D('',#25032,#14986,#14987);
#12318=AXIS2_PLACEMENT_3D('',#25033,#14988,#14989);
#12319=AXIS2_PLACEMENT_3D('',#25080,#14990,#14991);
#12320=AXIS2_PLACEMENT_3D('',#25081,#14992,#14993);
#12321=AXIS2_PLACEMENT_3D('',#25155,#14994,#14995);
#12322=AXIS2_PLACEMENT_3D('',#25156,#14996,#14997);
#12323=AXIS2_PLACEMENT_3D('',#25175,#14998,#14999);
#12324=AXIS2_PLACEMENT_3D('',#25236,#15000,#15001);
#12325=AXIS2_PLACEMENT_3D('',#25237,#15002,#15003);
#12326=AXIS2_PLACEMENT_3D('',#25238,#15004,#15005);
#12327=AXIS2_PLACEMENT_3D('',#25239,#15006,#15007);
#12328=AXIS2_PLACEMENT_3D('',#25240,#15008,#15009);
#12329=AXIS2_PLACEMENT_3D('',#25241,#15010,#15011);
#12330=AXIS2_PLACEMENT_3D('',#25242,#15012,#15013);
#12331=AXIS2_PLACEMENT_3D('',#25255,#15014,#15015);
#12332=AXIS2_PLACEMENT_3D('',#25311,#15016,#15017);
#12333=AXIS2_PLACEMENT_3D('',#25372,#15018,#15019);
#12334=AXIS2_PLACEMENT_3D('',#25373,#15020,#15021);
#12335=AXIS2_PLACEMENT_3D('',#25374,#15022,#15023);
#12336=AXIS2_PLACEMENT_3D('',#25463,#15024,#15025);
#12337=AXIS2_PLACEMENT_3D('',#25552,#15026,#15027);
#12338=AXIS2_PLACEMENT_3D('',#25553,#15028,#15029);
#12339=AXIS2_PLACEMENT_3D('',#25554,#15030,#15031);
#12340=AXIS2_PLACEMENT_3D('',#25555,#15032,#15033);
#12341=AXIS2_PLACEMENT_3D('',#25556,#15034,#15035);
#12342=AXIS2_PLACEMENT_3D('',#25557,#15036,#15037);
#12343=AXIS2_PLACEMENT_3D('',#25558,#15038,#15039);
#12344=AXIS2_PLACEMENT_3D('',#25559,#15040,#15041);
#12345=AXIS2_PLACEMENT_3D('',#25560,#15042,#15043);
#12346=AXIS2_PLACEMENT_3D('',#25561,#15044,#15045);
#12347=AXIS2_PLACEMENT_3D('',#25562,#15046,#15047);
#12348=AXIS2_PLACEMENT_3D('',#25563,#15048,#15049);
#12349=AXIS2_PLACEMENT_3D('',#25564,#15050,#15051);
#12350=AXIS2_PLACEMENT_3D('',#25565,#15052,#15053);
#12351=AXIS2_PLACEMENT_3D('',#25566,#15054,#15055);
#12352=AXIS2_PLACEMENT_3D('',#25585,#15056,#15057);
#12353=AXIS2_PLACEMENT_3D('',#25656,#15058,#15059);
#12354=AXIS2_PLACEMENT_3D('',#25763,#15060,#15061);
#12355=AXIS2_PLACEMENT_3D('',#25846,#15062,#15063);
#12356=AXIS2_PLACEMENT_3D('',#25847,#15064,#15065);
#12357=AXIS2_PLACEMENT_3D('',#25848,#15066,#15067);
#12358=AXIS2_PLACEMENT_3D('',#25849,#15068,#15069);
#12359=AXIS2_PLACEMENT_3D('',#25850,#15070,#15071);
#12360=AXIS2_PLACEMENT_3D('',#25851,#15072,#15073);
#12361=AXIS2_PLACEMENT_3D('',#25852,#15074,#15075);
#12362=AXIS2_PLACEMENT_3D('',#25853,#15076,#15077);
#12363=AXIS2_PLACEMENT_3D('',#25854,#15078,#15079);
#12364=AXIS2_PLACEMENT_3D('',#25901,#15080,#15081);
#12365=AXIS2_PLACEMENT_3D('',#25902,#15082,#15083);
#12366=AXIS2_PLACEMENT_3D('',#25903,#15084,#15085);
#12367=AXIS2_PLACEMENT_3D('',#25904,#15086,#15087);
#12368=AXIS2_PLACEMENT_3D('',#25981,#15088,#15089);
#12369=AXIS2_PLACEMENT_3D('',#25982,#15090,#15091);
#12370=AXIS2_PLACEMENT_3D('',#25983,#15092,#15093);
#12371=AXIS2_PLACEMENT_3D('',#25984,#15094,#15095);
#12372=AXIS2_PLACEMENT_3D('',#25997,#15096,#15097);
#12373=AXIS2_PLACEMENT_3D('',#25998,#15098,#15099);
#12374=AXIS2_PLACEMENT_3D('',#25999,#15100,#15101);
#12375=AXIS2_PLACEMENT_3D('',#26000,#15102,#15103);
#12376=AXIS2_PLACEMENT_3D('',#26001,#15104,#15105);
#12377=AXIS2_PLACEMENT_3D('',#26002,#15106,#15107);
#12378=AXIS2_PLACEMENT_3D('',#26119,#15108,#15109);
#12379=AXIS2_PLACEMENT_3D('',#26120,#15110,#15111);
#12380=AXIS2_PLACEMENT_3D('',#26121,#15112,#15113);
#12381=AXIS2_PLACEMENT_3D('',#26140,#15114,#15115);
#12382=AXIS2_PLACEMENT_3D('',#26141,#15116,#15117);
#12383=AXIS2_PLACEMENT_3D('',#26142,#15118,#15119);
#12384=AXIS2_PLACEMENT_3D('',#26143,#15120,#15121);
#12385=AXIS2_PLACEMENT_3D('',#26144,#15122,#15123);
#12386=AXIS2_PLACEMENT_3D('',#26145,#15124,#15125);
#12387=AXIS2_PLACEMENT_3D('',#26176,#15126,#15127);
#12388=AXIS2_PLACEMENT_3D('',#26177,#15128,#15129);
#12389=AXIS2_PLACEMENT_3D('',#26178,#15130,#15131);
#12390=AXIS2_PLACEMENT_3D('',#26179,#15132,#15133);
#12391=AXIS2_PLACEMENT_3D('',#26180,#15134,#15135);
#12392=AXIS2_PLACEMENT_3D('',#26181,#15136,#15137);
#12393=AXIS2_PLACEMENT_3D('',#26182,#15138,#15139);
#12394=AXIS2_PLACEMENT_3D('',#26183,#15140,#15141);
#12395=AXIS2_PLACEMENT_3D('',#26184,#15142,#15143);
#12396=AXIS2_PLACEMENT_3D('',#26185,#15144,#15145);
#12397=AXIS2_PLACEMENT_3D('',#26186,#15146,#15147);
#12398=AXIS2_PLACEMENT_3D('',#26324,#15148,#15149);
#12399=AXIS2_PLACEMENT_3D('',#26325,#15150,#15151);
#12400=AXIS2_PLACEMENT_3D('',#26326,#15152,#15153);
#12401=AXIS2_PLACEMENT_3D('',#26385,#15154,#15155);
#12402=AXIS2_PLACEMENT_3D('',#26386,#15156,#15157);
#12403=AXIS2_PLACEMENT_3D('',#26387,#15158,#15159);
#12404=AXIS2_PLACEMENT_3D('',#26422,#15160,#15161);
#12405=AXIS2_PLACEMENT_3D('',#26423,#15162,#15163);
#12406=AXIS2_PLACEMENT_3D('',#26424,#15164,#15165);
#12407=AXIS2_PLACEMENT_3D('',#26471,#15166,#15167);
#12408=AXIS2_PLACEMENT_3D('',#26472,#15168,#15169);
#12409=AXIS2_PLACEMENT_3D('',#26473,#15170,#15171);
#12410=AXIS2_PLACEMENT_3D('',#26474,#15172,#15173);
#12411=AXIS2_PLACEMENT_3D('',#26475,#15174,#15175);
#12412=AXIS2_PLACEMENT_3D('',#26476,#15176,#15177);
#12413=AXIS2_PLACEMENT_3D('',#26477,#15178,#15179);
#12414=AXIS2_PLACEMENT_3D('',#26512,#15180,#15181);
#12415=AXIS2_PLACEMENT_3D('',#26513,#15182,#15183);
#12416=AXIS2_PLACEMENT_3D('',#26526,#15184,#15185);
#12417=AXIS2_PLACEMENT_3D('',#26539,#15186,#15187);
#12418=AXIS2_PLACEMENT_3D('',#26540,#15188,#15189);
#12419=AXIS2_PLACEMENT_3D('',#26541,#15190,#15191);
#12420=AXIS2_PLACEMENT_3D('',#26542,#15192,#15193);
#12421=AXIS2_PLACEMENT_3D('',#26543,#15194,#15195);
#12422=AXIS2_PLACEMENT_3D('',#26562,#15196,#15197);
#12423=AXIS2_PLACEMENT_3D('',#26611,#15198,#15199);
#12424=AXIS2_PLACEMENT_3D('',#26612,#15200,#15201);
#12425=AXIS2_PLACEMENT_3D('',#26631,#15202,#15203);
#12426=AXIS2_PLACEMENT_3D('',#26738,#15204,#15205);
#12427=AXIS2_PLACEMENT_3D('',#26833,#15206,#15207);
#12428=AXIS2_PLACEMENT_3D('',#26834,#15208,#15209);
#12429=AXIS2_PLACEMENT_3D('',#26835,#15210,#15211);
#12430=AXIS2_PLACEMENT_3D('',#26836,#15212,#15213);
#12431=AXIS2_PLACEMENT_3D('',#26837,#15214,#15215);
#12432=AXIS2_PLACEMENT_3D('',#26838,#15216,#15217);
#12433=AXIS2_PLACEMENT_3D('',#26839,#15218,#15219);
#12434=AXIS2_PLACEMENT_3D('',#26840,#15220,#15221);
#12435=AXIS2_PLACEMENT_3D('',#26872,#15222,#15223);
#12436=AXIS2_PLACEMENT_3D('',#26873,#15224,#15225);
#12437=AXIS2_PLACEMENT_3D('',#26874,#15226,#15227);
#12438=AXIS2_PLACEMENT_3D('',#26875,#15228,#15229);
#12439=AXIS2_PLACEMENT_3D('',#26876,#15230,#15231);
#12440=AXIS2_PLACEMENT_3D('',#26877,#15232,#15233);
#12441=AXIS2_PLACEMENT_3D('',#26890,#15234,#15235);
#12442=AXIS2_PLACEMENT_3D('',#26891,#15236,#15237);
#12443=AXIS2_PLACEMENT_3D('',#26892,#15238,#15239);
#12444=AXIS2_PLACEMENT_3D('',#26966,#15240,#15241);
#12445=AXIS2_PLACEMENT_3D('',#26967,#15242,#15243);
#12446=AXIS2_PLACEMENT_3D('',#26968,#15244,#15245);
#12447=AXIS2_PLACEMENT_3D('',#26969,#15246,#15247);
#12448=AXIS2_PLACEMENT_3D('',#26970,#15248,#15249);
#12449=AXIS2_PLACEMENT_3D('',#26971,#15250,#15251);
#12450=AXIS2_PLACEMENT_3D('',#26972,#15252,#15253);
#12451=AXIS2_PLACEMENT_3D('',#26973,#15254,#15255);
#12452=AXIS2_PLACEMENT_3D('',#26974,#15256,#15257);
#12453=AXIS2_PLACEMENT_3D('',#26975,#15258,#15259);
#12454=AXIS2_PLACEMENT_3D('',#26976,#15260,#15261);
#12455=AXIS2_PLACEMENT_3D('',#26977,#15262,#15263);
#12456=AXIS2_PLACEMENT_3D('',#26978,#15264,#15265);
#12457=AXIS2_PLACEMENT_3D('',#26979,#15266,#15267);
#12458=AXIS2_PLACEMENT_3D('',#26980,#15268,#15269);
#12459=AXIS2_PLACEMENT_3D('',#26981,#15270,#15271);
#12460=AXIS2_PLACEMENT_3D('',#26982,#15272,#15273);
#12461=AXIS2_PLACEMENT_3D('',#27059,#15274,#15275);
#12462=AXIS2_PLACEMENT_3D('',#27106,#15276,#15277);
#12463=AXIS2_PLACEMENT_3D('',#27107,#15278,#15279);
#12464=AXIS2_PLACEMENT_3D('',#27108,#15280,#15281);
#12465=AXIS2_PLACEMENT_3D('',#27109,#15282,#15283);
#12466=AXIS2_PLACEMENT_3D('',#27186,#15284,#15285);
#12467=AXIS2_PLACEMENT_3D('',#27187,#15286,#15287);
#12468=AXIS2_PLACEMENT_3D('',#27188,#15288,#15289);
#12469=AXIS2_PLACEMENT_3D('',#27189,#15290,#15291);
#12470=AXIS2_PLACEMENT_3D('',#27190,#15292,#15293);
#12471=AXIS2_PLACEMENT_3D('',#27191,#15294,#15295);
#12472=AXIS2_PLACEMENT_3D('',#27192,#15296,#15297);
#12473=AXIS2_PLACEMENT_3D('',#27245,#15298,#15299);
#12474=AXIS2_PLACEMENT_3D('',#27246,#15300,#15301);
#12475=AXIS2_PLACEMENT_3D('',#27277,#15302,#15303);
#12476=AXIS2_PLACEMENT_3D('',#27278,#15304,#15305);
#12477=AXIS2_PLACEMENT_3D('',#27279,#15306,#15307);
#12478=AXIS2_PLACEMENT_3D('',#27280,#15308,#15309);
#12479=AXIS2_PLACEMENT_3D('',#27281,#15310,#15311);
#12480=AXIS2_PLACEMENT_3D('',#27379,#15312,#15313);
#12481=AXIS2_PLACEMENT_3D('',#27380,#15314,#15315);
#12482=AXIS2_PLACEMENT_3D('',#27381,#15316,#15317);
#12483=AXIS2_PLACEMENT_3D('',#27382,#15318,#15319);
#12484=AXIS2_PLACEMENT_3D('',#27383,#15320,#15321);
#12485=AXIS2_PLACEMENT_3D('',#27384,#15322,#15323);
#12486=AXIS2_PLACEMENT_3D('',#27431,#15324,#15325);
#12487=AXIS2_PLACEMENT_3D('',#27462,#15326,#15327);
#12488=AXIS2_PLACEMENT_3D('',#27463,#15328,#15329);
#12489=AXIS2_PLACEMENT_3D('',#27464,#15330,#15331);
#12490=AXIS2_PLACEMENT_3D('',#27465,#15332,#15333);
#12491=AXIS2_PLACEMENT_3D('',#27490,#15334,#15335);
#12492=AXIS2_PLACEMENT_3D('',#27491,#15336,#15337);
#12493=AXIS2_PLACEMENT_3D('',#27522,#15338,#15339);
#12494=AXIS2_PLACEMENT_3D('',#27523,#15340,#15341);
#12495=AXIS2_PLACEMENT_3D('',#27524,#15342,#15343);
#12496=AXIS2_PLACEMENT_3D('',#27543,#15344,#15345);
#12497=AXIS2_PLACEMENT_3D('',#27599,#15346,#15347);
#12498=AXIS2_PLACEMENT_3D('',#27600,#15348,#15349);
#12499=AXIS2_PLACEMENT_3D('',#27601,#15350,#15351);
#12500=AXIS2_PLACEMENT_3D('',#27602,#15352,#15353);
#12501=AXIS2_PLACEMENT_3D('',#27634,#15354,#15355);
#12502=AXIS2_PLACEMENT_3D('',#27635,#15356,#15357);
#12503=AXIS2_PLACEMENT_3D('',#27636,#15358,#15359);
#12504=AXIS2_PLACEMENT_3D('',#27637,#15360,#15361);
#12505=AXIS2_PLACEMENT_3D('',#27723,#15362,#15363);
#12506=AXIS2_PLACEMENT_3D('',#27742,#15364,#15365);
#12507=AXIS2_PLACEMENT_3D('',#27743,#15366,#15367);
#12508=AXIS2_PLACEMENT_3D('',#27744,#15368,#15369);
#12509=AXIS2_PLACEMENT_3D('',#27763,#15370,#15371);
#12510=AXIS2_PLACEMENT_3D('',#27824,#15372,#15373);
#12511=AXIS2_PLACEMENT_3D('',#27825,#15374,#15375);
#12512=AXIS2_PLACEMENT_3D('',#27826,#15376,#15377);
#12513=AXIS2_PLACEMENT_3D('',#27827,#15378,#15379);
#12514=AXIS2_PLACEMENT_3D('',#27828,#15380,#15381);
#12515=AXIS2_PLACEMENT_3D('',#27829,#15382,#15383);
#12516=AXIS2_PLACEMENT_3D('',#27830,#15384,#15385);
#12517=AXIS2_PLACEMENT_3D('',#27831,#15386,#15387);
#12518=AXIS2_PLACEMENT_3D('',#27832,#15388,#15389);
#12519=AXIS2_PLACEMENT_3D('',#27833,#15390,#15391);
#12520=AXIS2_PLACEMENT_3D('',#27834,#15392,#15393);
#12521=AXIS2_PLACEMENT_3D('',#27835,#15394,#15395);
#12522=AXIS2_PLACEMENT_3D('',#27836,#15396,#15397);
#12523=AXIS2_PLACEMENT_3D('',#27871,#15398,#15399);
#12524=AXIS2_PLACEMENT_3D('',#27890,#15400,#15401);
#12525=AXIS2_PLACEMENT_3D('',#28064,#15402,#15403);
#12526=AXIS2_PLACEMENT_3D('',#28065,#15404,#15405);
#12527=AXIS2_PLACEMENT_3D('',#28066,#15406,#15407);
#12528=AXIS2_PLACEMENT_3D('',#28067,#15408,#15409);
#12529=AXIS2_PLACEMENT_3D('',#28080,#15410,#15411);
#12530=AXIS2_PLACEMENT_3D('',#28093,#15412,#15413);
#12531=AXIS2_PLACEMENT_3D('',#28094,#15414,#15415);
#12532=AXIS2_PLACEMENT_3D('',#28183,#15416,#15417);
#12533=AXIS2_PLACEMENT_3D('',#28184,#15418,#15419);
#12534=AXIS2_PLACEMENT_3D('',#28209,#15420,#15421);
#12535=AXIS2_PLACEMENT_3D('',#28210,#15422,#15423);
#12536=AXIS2_PLACEMENT_3D('',#28211,#15424,#15425);
#12537=AXIS2_PLACEMENT_3D('',#28212,#15426,#15427);
#12538=AXIS2_PLACEMENT_3D('',#28213,#15428,#15429);
#12539=AXIS2_PLACEMENT_3D('',#28214,#15430,#15431);
#12540=AXIS2_PLACEMENT_3D('',#28215,#15432,#15433);
#12541=AXIS2_PLACEMENT_3D('',#28216,#15434,#15435);
#12542=AXIS2_PLACEMENT_3D('',#28217,#15436,#15437);
#12543=AXIS2_PLACEMENT_3D('',#28218,#15438,#15439);
#12544=AXIS2_PLACEMENT_3D('',#28219,#15440,#15441);
#12545=AXIS2_PLACEMENT_3D('',#28220,#15442,#15443);
#12546=AXIS2_PLACEMENT_3D('',#28221,#15444,#15445);
#12547=AXIS2_PLACEMENT_3D('',#28235,#15446,#15447);
#12548=AXIS2_PLACEMENT_3D('',#28236,#15448,#15449);
#12549=AXIS2_PLACEMENT_3D('',#28237,#15450,#15451);
#12550=AXIS2_PLACEMENT_3D('',#28238,#15452,#15453);
#12551=AXIS2_PLACEMENT_3D('',#28239,#15454,#15455);
#12552=AXIS2_PLACEMENT_3D('',#28240,#15456,#15457);
#12553=AXIS2_PLACEMENT_3D('',#28241,#15458,#15459);
#12554=AXIS2_PLACEMENT_3D('',#28260,#15460,#15461);
#12555=AXIS2_PLACEMENT_3D('',#28261,#15462,#15463);
#12556=AXIS2_PLACEMENT_3D('',#28262,#15464,#15465);
#12557=AXIS2_PLACEMENT_3D('',#28263,#15466,#15467);
#12558=AXIS2_PLACEMENT_3D('',#28276,#15468,#15469);
#12559=AXIS2_PLACEMENT_3D('',#28277,#15470,#15471);
#12560=AXIS2_PLACEMENT_3D('',#28278,#15472,#15473);
#12561=AXIS2_PLACEMENT_3D('',#28279,#15474,#15475);
#12562=AXIS2_PLACEMENT_3D('',#28280,#15476,#15477);
#12563=AXIS2_PLACEMENT_3D('',#28281,#15478,#15479);
#12564=AXIS2_PLACEMENT_3D('',#28298,#15480,#15481);
#12565=AXIS2_PLACEMENT_3D('',#28323,#15482,#15483);
#12566=AXIS2_PLACEMENT_3D('',#28324,#15484,#15485);
#12567=AXIS2_PLACEMENT_3D('',#28325,#15486,#15487);
#12568=AXIS2_PLACEMENT_3D('',#28326,#15488,#15489);
#12569=AXIS2_PLACEMENT_3D('',#28327,#15490,#15491);
#12570=AXIS2_PLACEMENT_3D('',#28328,#15492,#15493);
#12571=AXIS2_PLACEMENT_3D('',#28329,#15494,#15495);
#12572=AXIS2_PLACEMENT_3D('',#28330,#15496,#15497);
#12573=AXIS2_PLACEMENT_3D('',#28331,#15498,#15499);
#12574=AXIS2_PLACEMENT_3D('',#28332,#15500,#15501);
#12575=AXIS2_PLACEMENT_3D('',#28333,#15502,#15503);
#12576=AXIS2_PLACEMENT_3D('',#28334,#15504,#15505);
#12577=AXIS2_PLACEMENT_3D('',#28353,#15506,#15507);
#12578=AXIS2_PLACEMENT_3D('',#28354,#15508,#15509);
#12579=AXIS2_PLACEMENT_3D('',#28355,#15510,#15511);
#12580=AXIS2_PLACEMENT_3D('',#28356,#15512,#15513);
#12581=AXIS2_PLACEMENT_3D('',#28357,#15514,#15515);
#12582=AXIS2_PLACEMENT_3D('',#28358,#15516,#15517);
#12583=AXIS2_PLACEMENT_3D('',#28359,#15518,#15519);
#12584=AXIS2_PLACEMENT_3D('',#28360,#15520,#15521);
#12585=AXIS2_PLACEMENT_3D('',#28395,#15522,#15523);
#12586=AXIS2_PLACEMENT_3D('',#28396,#15524,#15525);
#12587=AXIS2_PLACEMENT_3D('',#28397,#15526,#15527);
#12588=AXIS2_PLACEMENT_3D('',#28398,#15528,#15529);
#12589=AXIS2_PLACEMENT_3D('',#28399,#15530,#15531);
#12590=AXIS2_PLACEMENT_3D('',#28400,#15532,#15533);
#12591=AXIS2_PLACEMENT_3D('',#28401,#15534,#15535);
#12592=AXIS2_PLACEMENT_3D('',#28402,#15536,#15537);
#12593=AXIS2_PLACEMENT_3D('',#28419,#15538,#15539);
#12594=AXIS2_PLACEMENT_3D('',#28420,#15540,#15541);
#12595=AXIS2_PLACEMENT_3D('',#28439,#15542,#15543);
#12596=AXIS2_PLACEMENT_3D('',#28440,#15544,#15545);
#12597=AXIS2_PLACEMENT_3D('',#28441,#15546,#15547);
#12598=AXIS2_PLACEMENT_3D('',#28442,#15548,#15549);
#12599=AXIS2_PLACEMENT_3D('',#28443,#15550,#15551);
#12600=AXIS2_PLACEMENT_3D('',#28444,#15552,#15553);
#12601=AXIS2_PLACEMENT_3D('',#28445,#15554,#15555);
#12602=AXIS2_PLACEMENT_3D('',#28446,#15556,#15557);
#12603=AXIS2_PLACEMENT_3D('',#28447,#15558,#15559);
#12604=AXIS2_PLACEMENT_3D('',#28466,#15560,#15561);
#12605=AXIS2_PLACEMENT_3D('',#28467,#15562,#15563);
#12606=AXIS2_PLACEMENT_3D('',#28468,#15564,#15565);
#12607=AXIS2_PLACEMENT_3D('',#28469,#15566,#15567);
#12608=AXIS2_PLACEMENT_3D('',#28470,#15568,#15569);
#12609=AXIS2_PLACEMENT_3D('',#28471,#15570,#15571);
#12610=AXIS2_PLACEMENT_3D('',#28472,#15572,#15573);
#12611=AXIS2_PLACEMENT_3D('',#28473,#15574,#15575);
#12612=AXIS2_PLACEMENT_3D('',#28528,#15576,#15577);
#12613=AXIS2_PLACEMENT_3D('',#28529,#15578,#15579);
#12614=AXIS2_PLACEMENT_3D('',#28549,#15580,#15581);
#12615=AXIS2_PLACEMENT_3D('',#28550,#15582,#15583);
#12616=AXIS2_PLACEMENT_3D('',#28551,#15584,#15585);
#12617=AXIS2_PLACEMENT_3D('',#28552,#15586,#15587);
#12618=AXIS2_PLACEMENT_3D('',#28566,#15588,#15589);
#12619=AXIS2_PLACEMENT_3D('',#28567,#15590,#15591);
#12620=AXIS2_PLACEMENT_3D('',#28568,#15592,#15593);
#12621=AXIS2_PLACEMENT_3D('',#28593,#15594,#15595);
#12622=AXIS2_PLACEMENT_3D('',#28594,#15596,#15597);
#12623=AXIS2_PLACEMENT_3D('',#28595,#15598,#15599);
#12624=AXIS2_PLACEMENT_3D('',#28596,#15600,#15601);
#12625=AXIS2_PLACEMENT_3D('',#28597,#15602,#15603);
#12626=AXIS2_PLACEMENT_3D('',#28610,#15604,#15605);
#12627=AXIS2_PLACEMENT_3D('',#28611,#15606,#15607);
#12628=AXIS2_PLACEMENT_3D('',#28612,#15608,#15609);
#12629=AXIS2_PLACEMENT_3D('',#28613,#15610,#15611);
#12630=AXIS2_PLACEMENT_3D('',#28614,#15612,#15613);
#12631=AXIS2_PLACEMENT_3D('',#28615,#15614,#15615);
#12632=AXIS2_PLACEMENT_3D('',#28634,#15616,#15617);
#12633=AXIS2_PLACEMENT_3D('',#28635,#15618,#15619);
#12634=AXIS2_PLACEMENT_3D('',#28636,#15620,#15621);
#12635=AXIS2_PLACEMENT_3D('',#28655,#15622,#15623);
#12636=AXIS2_PLACEMENT_3D('',#28674,#15624,#15625);
#12637=AXIS2_PLACEMENT_3D('',#28688,#15626,#15627);
#12638=AXIS2_PLACEMENT_3D('',#28689,#15628,#15629);
#12639=AXIS2_PLACEMENT_3D('',#28690,#15630,#15631);
#12640=AXIS2_PLACEMENT_3D('',#28691,#15632,#15633);
#12641=AXIS2_PLACEMENT_3D('',#28692,#15634,#15635);
#12642=AXIS2_PLACEMENT_3D('',#28693,#15636,#15637);
#12643=AXIS2_PLACEMENT_3D('',#28713,#15638,#15639);
#12644=AXIS2_PLACEMENT_3D('',#28714,#15640,#15641);
#12645=AXIS2_PLACEMENT_3D('',#28715,#15642,#15643);
#12646=AXIS2_PLACEMENT_3D('',#28716,#15644,#15645);
#12647=AXIS2_PLACEMENT_3D('',#28717,#15646,#15647);
#12648=AXIS2_PLACEMENT_3D('',#28718,#15648,#15649);
#12649=AXIS2_PLACEMENT_3D('',#28719,#15650,#15651);
#12650=AXIS2_PLACEMENT_3D('',#28720,#15652,#15653);
#12651=AXIS2_PLACEMENT_3D('',#28739,#15654,#15655);
#12652=AXIS2_PLACEMENT_3D('',#28740,#15656,#15657);
#12653=AXIS2_PLACEMENT_3D('',#28741,#15658,#15659);
#12654=AXIS2_PLACEMENT_3D('',#28742,#15660,#15661);
#12655=AXIS2_PLACEMENT_3D('',#28743,#15662,#15663);
#12656=AXIS2_PLACEMENT_3D('',#28744,#15664,#15665);
#12657=AXIS2_PLACEMENT_3D('',#28745,#15666,#15667);
#12658=AXIS2_PLACEMENT_3D('',#28746,#15668,#15669);
#12659=AXIS2_PLACEMENT_3D('',#28747,#15670,#15671);
#12660=AXIS2_PLACEMENT_3D('',#28748,#15672,#15673);
#12661=AXIS2_PLACEMENT_3D('',#28749,#15674,#15675);
#12662=AXIS2_PLACEMENT_3D('',#28768,#15676,#15677);
#12663=AXIS2_PLACEMENT_3D('',#28769,#15678,#15679);
#12664=AXIS2_PLACEMENT_3D('',#28770,#15680,#15681);
#12665=AXIS2_PLACEMENT_3D('',#28771,#15682,#15683);
#12666=AXIS2_PLACEMENT_3D('',#28772,#15684,#15685);
#12667=AXIS2_PLACEMENT_3D('',#28773,#15686,#15687);
#12668=AXIS2_PLACEMENT_3D('',#28774,#15688,#15689);
#12669=AXIS2_PLACEMENT_3D('',#28775,#15690,#15691);
#12670=AXIS2_PLACEMENT_3D('',#28776,#15692,#15693);
#12671=AXIS2_PLACEMENT_3D('',#28811,#15694,#15695);
#12672=AXIS2_PLACEMENT_3D('',#28812,#15696,#15697);
#12673=AXIS2_PLACEMENT_3D('',#28813,#15698,#15699);
#12674=AXIS2_PLACEMENT_3D('',#28814,#15700,#15701);
#12675=AXIS2_PLACEMENT_3D('',#28815,#15702,#15703);
#12676=AXIS2_PLACEMENT_3D('',#28816,#15704,#15705);
#12677=AXIS2_PLACEMENT_3D('',#28817,#15706,#15707);
#12678=AXIS2_PLACEMENT_3D('',#28872,#15708,#15709);
#12679=AXIS2_PLACEMENT_3D('',#28873,#15710,#15711);
#12680=AXIS2_PLACEMENT_3D('',#28874,#15712,#15713);
#12681=AXIS2_PLACEMENT_3D('',#28875,#15714,#15715);
#12682=AXIS2_PLACEMENT_3D('',#28910,#15716,#15717);
#12683=AXIS2_PLACEMENT_3D('',#28911,#15718,#15719);
#12684=AXIS2_PLACEMENT_3D('',#28912,#15720,#15721);
#12685=AXIS2_PLACEMENT_3D('',#28913,#15722,#15723);
#12686=AXIS2_PLACEMENT_3D('',#28914,#15724,#15725);
#12687=AXIS2_PLACEMENT_3D('',#28915,#15726,#15727);
#12688=AXIS2_PLACEMENT_3D('',#28916,#15728,#15729);
#12689=AXIS2_PLACEMENT_3D('',#28917,#15730,#15731);
#12690=AXIS2_PLACEMENT_3D('',#28918,#15732,#15733);
#12691=AXIS2_PLACEMENT_3D('',#28919,#15734,#15735);
#12692=AXIS2_PLACEMENT_3D('',#28920,#15736,#15737);
#12693=AXIS2_PLACEMENT_3D('',#28921,#15738,#15739);
#12694=AXIS2_PLACEMENT_3D('',#28922,#15740,#15741);
#12695=AXIS2_PLACEMENT_3D('',#28923,#15742,#15743);
#12696=AXIS2_PLACEMENT_3D('',#28924,#15744,#15745);
#12697=AXIS2_PLACEMENT_3D('',#28937,#15746,#15747);
#12698=AXIS2_PLACEMENT_3D('',#28938,#15748,#15749);
#12699=AXIS2_PLACEMENT_3D('',#28961,#15750,#15751);
#12700=AXIS2_PLACEMENT_3D('',#28980,#15752,#15753);
#12701=AXIS2_PLACEMENT_3D('',#28999,#15754,#15755);
#12702=AXIS2_PLACEMENT_3D('',#29000,#15756,#15757);
#12703=AXIS2_PLACEMENT_3D('',#29001,#15758,#15759);
#12704=AXIS2_PLACEMENT_3D('',#29002,#15760,#15761);
#12705=AXIS2_PLACEMENT_3D('',#29003,#15762,#15763);
#12706=AXIS2_PLACEMENT_3D('',#29004,#15764,#15765);
#12707=AXIS2_PLACEMENT_3D('',#29005,#15766,#15767);
#12708=AXIS2_PLACEMENT_3D('',#29006,#15768,#15769);
#12709=AXIS2_PLACEMENT_3D('',#29007,#15770,#15771);
#12710=AXIS2_PLACEMENT_3D('',#29026,#15772,#15773);
#12711=AXIS2_PLACEMENT_3D('',#29043,#15774,#15775);
#12712=AXIS2_PLACEMENT_3D('',#29044,#15776,#15777);
#12713=AXIS2_PLACEMENT_3D('',#29045,#15778,#15779);
#12714=AXIS2_PLACEMENT_3D('',#29046,#15780,#15781);
#12715=AXIS2_PLACEMENT_3D('',#29107,#15782,#15783);
#12716=AXIS2_PLACEMENT_3D('',#29108,#15784,#15785);
#12717=AXIS2_PLACEMENT_3D('',#29109,#15786,#15787);
#12718=AXIS2_PLACEMENT_3D('',#29110,#15788,#15789);
#12719=AXIS2_PLACEMENT_3D('',#29111,#15790,#15791);
#12720=AXIS2_PLACEMENT_3D('',#29112,#15792,#15793);
#12721=AXIS2_PLACEMENT_3D('',#29113,#15794,#15795);
#12722=AXIS2_PLACEMENT_3D('',#29114,#15796,#15797);
#12723=AXIS2_PLACEMENT_3D('',#29139,#15798,#15799);
#12724=AXIS2_PLACEMENT_3D('',#29140,#15800,#15801);
#12725=AXIS2_PLACEMENT_3D('',#29141,#15802,#15803);
#12726=AXIS2_PLACEMENT_3D('',#29142,#15804,#15805);
#12727=AXIS2_PLACEMENT_3D('',#29143,#15806,#15807);
#12728=AXIS2_PLACEMENT_3D('',#29144,#15808,#15809);
#12729=AXIS2_PLACEMENT_3D('',#29145,#15810,#15811);
#12730=AXIS2_PLACEMENT_3D('',#29146,#15812,#15813);
#12731=AXIS2_PLACEMENT_3D('',#29147,#15814,#15815);
#12732=AXIS2_PLACEMENT_3D('',#29166,#15816,#15817);
#12733=AXIS2_PLACEMENT_3D('',#29186,#15818,#15819);
#12734=AXIS2_PLACEMENT_3D('',#29187,#15820,#15821);
#12735=AXIS2_PLACEMENT_3D('',#29219,#15822,#15823);
#12736=AXIS2_PLACEMENT_3D('',#29220,#15824,#15825);
#12737=AXIS2_PLACEMENT_3D('',#29221,#15826,#15827);
#12738=AXIS2_PLACEMENT_3D('',#29222,#15828,#15829);
#12739=AXIS2_PLACEMENT_3D('',#29223,#15830,#15831);
#12740=AXIS2_PLACEMENT_3D('',#29224,#15832,#15833);
#12741=AXIS2_PLACEMENT_3D('',#29225,#15834,#15835);
#12742=AXIS2_PLACEMENT_3D('',#29226,#15836,#15837);
#12743=AXIS2_PLACEMENT_3D('',#29227,#15838,#15839);
#12744=AXIS2_PLACEMENT_3D('',#29228,#15840,#15841);
#12745=AXIS2_PLACEMENT_3D('',#29241,#15842,#15843);
#12746=AXIS2_PLACEMENT_3D('',#29242,#15844,#15845);
#12747=AXIS2_PLACEMENT_3D('',#29243,#15846,#15847);
#12748=AXIS2_PLACEMENT_3D('',#29244,#15848,#15849);
#12749=AXIS2_PLACEMENT_3D('',#29245,#15850,#15851);
#12750=AXIS2_PLACEMENT_3D('',#29246,#15852,#15853);
#12751=AXIS2_PLACEMENT_3D('',#29247,#15854,#15855);
#12752=AXIS2_PLACEMENT_3D('',#29248,#15856,#15857);
#12753=AXIS2_PLACEMENT_3D('',#29249,#15858,#15859);
#12754=AXIS2_PLACEMENT_3D('',#29250,#15860,#15861);
#12755=AXIS2_PLACEMENT_3D('',#29270,#15862,#15863);
#12756=AXIS2_PLACEMENT_3D('',#29289,#15864,#15865);
#12757=AXIS2_PLACEMENT_3D('',#29290,#15866,#15867);
#12758=AXIS2_PLACEMENT_3D('',#29291,#15868,#15869);
#12759=AXIS2_PLACEMENT_3D('',#29292,#15870,#15871);
#12760=AXIS2_PLACEMENT_3D('',#29293,#15872,#15873);
#12761=AXIS2_PLACEMENT_3D('',#29294,#15874,#15875);
#12762=AXIS2_PLACEMENT_3D('',#29295,#15876,#15877);
#12763=AXIS2_PLACEMENT_3D('',#29296,#15878,#15879);
#12764=AXIS2_PLACEMENT_3D('',#29297,#15880,#15881);
#12765=AXIS2_PLACEMENT_3D('',#29298,#15882,#15883);
#12766=AXIS2_PLACEMENT_3D('',#29299,#15884,#15885);
#12767=AXIS2_PLACEMENT_3D('',#29354,#15886,#15887);
#12768=AXIS2_PLACEMENT_3D('',#29355,#15888,#15889);
#12769=AXIS2_PLACEMENT_3D('',#29356,#15890,#15891);
#12770=AXIS2_PLACEMENT_3D('',#29357,#15892,#15893);
#12771=AXIS2_PLACEMENT_3D('',#29358,#15894,#15895);
#12772=AXIS2_PLACEMENT_3D('',#29359,#15896,#15897);
#12773=AXIS2_PLACEMENT_3D('',#29360,#15898,#15899);
#12774=AXIS2_PLACEMENT_3D('',#29361,#15900,#15901);
#12775=AXIS2_PLACEMENT_3D('',#29362,#15902,#15903);
#12776=AXIS2_PLACEMENT_3D('',#29375,#15904,#15905);
#12777=AXIS2_PLACEMENT_3D('',#29416,#15906,#15907);
#12778=AXIS2_PLACEMENT_3D('',#29417,#15908,#15909);
#12779=AXIS2_PLACEMENT_3D('',#29418,#15910,#15911);
#12780=AXIS2_PLACEMENT_3D('',#29419,#15912,#15913);
#12781=AXIS2_PLACEMENT_3D('',#29420,#15914,#15915);
#12782=AXIS2_PLACEMENT_3D('',#29421,#15916,#15917);
#12783=AXIS2_PLACEMENT_3D('',#29422,#15918,#15919);
#12784=AXIS2_PLACEMENT_3D('',#29423,#15920,#15921);
#12785=AXIS2_PLACEMENT_3D('',#29424,#15922,#15923);
#12786=AXIS2_PLACEMENT_3D('',#29425,#15924,#15925);
#12787=AXIS2_PLACEMENT_3D('',#29426,#15926,#15927);
#12788=AXIS2_PLACEMENT_3D('',#29427,#15928,#15929);
#12789=AXIS2_PLACEMENT_3D('',#29428,#15930,#15931);
#12790=AXIS2_PLACEMENT_3D('',#29429,#15932,#15933);
#12791=AXIS2_PLACEMENT_3D('',#29430,#15934,#15935);
#12792=AXIS2_PLACEMENT_3D('',#30273,#15936,#15937);
#12793=AXIS2_PLACEMENT_3D('',#31065,#15938,#15939);
#12794=AXIS2_PLACEMENT_3D('',#31133,#15940,#15941);
#12795=AXIS2_PLACEMENT_3D('',#31140,#15942,#15943);
#12796=AXIS2_PLACEMENT_3D('',#31141,#15944,#15945);
#12797=AXIS2_PLACEMENT_3D('',#31142,#15946,#15947);
#12798=AXIS2_PLACEMENT_3D('',#31183,#15948,#15949);
#12799=AXIS2_PLACEMENT_3D('',#31202,#15950,#15951);
#12800=AXIS2_PLACEMENT_3D('',#31279,#15952,#15953);
#12801=AXIS2_PLACEMENT_3D('',#31280,#15954,#15955);
#12802=AXIS2_PLACEMENT_3D('',#31281,#15956,#15957);
#12803=AXIS2_PLACEMENT_3D('',#31282,#15958,#15959);
#12804=AXIS2_PLACEMENT_3D('',#31283,#15960,#15961);
#12805=AXIS2_PLACEMENT_3D('',#31284,#15962,#15963);
#12806=AXIS2_PLACEMENT_3D('',#31285,#15964,#15965);
#12807=AXIS2_PLACEMENT_3D('',#31488,#15966,#15967);
#12808=AXIS2_PLACEMENT_3D('',#31507,#15968,#15969);
#12809=AXIS2_PLACEMENT_3D('',#31554,#15970,#15971);
#12810=AXIS2_PLACEMENT_3D('',#31555,#15972,#15973);
#12811=AXIS2_PLACEMENT_3D('',#31610,#15974,#15975);
#12812=AXIS2_PLACEMENT_3D('',#31611,#15976,#15977);
#12813=AXIS2_PLACEMENT_3D('',#31612,#15978,#15979);
#12814=AXIS2_PLACEMENT_3D('',#31613,#15980,#15981);
#12815=AXIS2_PLACEMENT_3D('',#31723,#15982,#15983);
#12816=AXIS2_PLACEMENT_3D('',#31880,#15984,#15985);
#12817=AXIS2_PLACEMENT_3D('',#31899,#15986,#15987);
#12818=AXIS2_PLACEMENT_3D('',#31900,#15988,#15989);
#12819=AXIS2_PLACEMENT_3D('',#31901,#15990,#15991);
#12820=AXIS2_PLACEMENT_3D('',#31926,#15992,#15993);
#12821=AXIS2_PLACEMENT_3D('',#31927,#15994,#15995);
#12822=AXIS2_PLACEMENT_3D('',#31928,#15996,#15997);
#12823=AXIS2_PLACEMENT_3D('',#31929,#15998,#15999);
#12824=AXIS2_PLACEMENT_3D('',#31978,#16000,#16001);
#12825=AXIS2_PLACEMENT_3D('',#32043,#16002,#16003);
#12826=AXIS2_PLACEMENT_3D('',#32044,#16004,#16005);
#12827=AXIS2_PLACEMENT_3D('',#32045,#16006,#16007);
#12828=AXIS2_PLACEMENT_3D('',#32046,#16008,#16009);
#12829=AXIS2_PLACEMENT_3D('',#32047,#16010,#16011);
#12830=AXIS2_PLACEMENT_3D('',#32048,#16012,#16013);
#12831=AXIS2_PLACEMENT_3D('',#32049,#16014,#16015);
#12832=AXIS2_PLACEMENT_3D('',#32050,#16016,#16017);
#12833=AXIS2_PLACEMENT_3D('',#32051,#16018,#16019);
#12834=AXIS2_PLACEMENT_3D('',#32052,#16020,#16021);
#12835=AXIS2_PLACEMENT_3D('',#32053,#16022,#16023);
#12836=AXIS2_PLACEMENT_3D('',#32054,#16024,#16025);
#12837=AXIS2_PLACEMENT_3D('',#32055,#16026,#16027);
#12838=AXIS2_PLACEMENT_3D('',#32056,#16028,#16029);
#12839=AXIS2_PLACEMENT_3D('',#32057,#16030,#16031);
#12840=AXIS2_PLACEMENT_3D('',#32058,#16032,#16033);
#12841=AXIS2_PLACEMENT_3D('',#32059,#16034,#16035);
#12842=AXIS2_PLACEMENT_3D('',#32060,#16036,#16037);
#12843=AXIS2_PLACEMENT_3D('',#32061,#16038,#16039);
#12844=AXIS2_PLACEMENT_3D('',#32062,#16040,#16041);
#12845=AXIS2_PLACEMENT_3D('',#32063,#16042,#16043);
#12846=AXIS2_PLACEMENT_3D('',#32064,#16044,#16045);
#12847=AXIS2_PLACEMENT_3D('',#32065,#16046,#16047);
#12848=AXIS2_PLACEMENT_3D('',#32066,#16048,#16049);
#12849=AXIS2_PLACEMENT_3D('',#32067,#16050,#16051);
#12850=AXIS2_PLACEMENT_3D('',#32068,#16052,#16053);
#12851=AXIS2_PLACEMENT_3D('',#32069,#16054,#16055);
#12852=AXIS2_PLACEMENT_3D('',#32070,#16056,#16057);
#12853=AXIS2_PLACEMENT_3D('',#32071,#16058,#16059);
#12854=AXIS2_PLACEMENT_3D('',#32072,#16060,#16061);
#12855=AXIS2_PLACEMENT_3D('',#32073,#16062,#16063);
#12856=AXIS2_PLACEMENT_3D('',#32074,#16064,#16065);
#12857=AXIS2_PLACEMENT_3D('',#32075,#16066,#16067);
#12858=AXIS2_PLACEMENT_3D('',#32076,#16068,#16069);
#12859=AXIS2_PLACEMENT_3D('',#32077,#16070,#16071);
#12860=AXIS2_PLACEMENT_3D('',#32078,#16072,#16073);
#12861=AXIS2_PLACEMENT_3D('',#32079,#16074,#16075);
#12862=AXIS2_PLACEMENT_3D('',#32080,#16076,#16077);
#12863=AXIS2_PLACEMENT_3D('',#32081,#16078,#16079);
#12864=AXIS2_PLACEMENT_3D('',#32082,#16080,#16081);
#12865=AXIS2_PLACEMENT_3D('',#32083,#16082,#16083);
#12866=AXIS2_PLACEMENT_3D('',#32084,#16084,#16085);
#12867=AXIS2_PLACEMENT_3D('',#32085,#16086,#16087);
#12868=AXIS2_PLACEMENT_3D('',#32086,#16088,#16089);
#12869=AXIS2_PLACEMENT_3D('',#32087,#16090,#16091);
#12870=AXIS2_PLACEMENT_3D('',#32088,#16092,#16093);
#12871=AXIS2_PLACEMENT_3D('',#32089,#16094,#16095);
#12872=AXIS2_PLACEMENT_3D('',#32090,#16096,#16097);
#12873=AXIS2_PLACEMENT_3D('',#32091,#16098,#16099);
#12874=AXIS2_PLACEMENT_3D('',#32092,#16100,#16101);
#12875=AXIS2_PLACEMENT_3D('',#32093,#16102,#16103);
#12876=AXIS2_PLACEMENT_3D('',#32094,#16104,#16105);
#12877=AXIS2_PLACEMENT_3D('',#32095,#16106,#16107);
#12878=AXIS2_PLACEMENT_3D('',#32096,#16108,#16109);
#12879=AXIS2_PLACEMENT_3D('',#32097,#16110,#16111);
#12880=AXIS2_PLACEMENT_3D('',#32098,#16112,#16113);
#12881=AXIS2_PLACEMENT_3D('',#32099,#16114,#16115);
#12882=AXIS2_PLACEMENT_3D('',#32100,#16116,#16117);
#12883=AXIS2_PLACEMENT_3D('',#32101,#16118,#16119);
#12884=AXIS2_PLACEMENT_3D('',#32102,#16120,#16121);
#12885=AXIS2_PLACEMENT_3D('',#32103,#16122,#16123);
#12886=AXIS2_PLACEMENT_3D('',#32104,#16124,#16125);
#12887=AXIS2_PLACEMENT_3D('',#32105,#16126,#16127);
#12888=AXIS2_PLACEMENT_3D('',#32106,#16128,#16129);
#12889=AXIS2_PLACEMENT_3D('',#32107,#16130,#16131);
#12890=AXIS2_PLACEMENT_3D('',#32108,#16132,#16133);
#12891=AXIS2_PLACEMENT_3D('',#32109,#16134,#16135);
#12892=AXIS2_PLACEMENT_3D('',#32110,#16136,#16137);
#12893=AXIS2_PLACEMENT_3D('',#32111,#16138,#16139);
#12894=AXIS2_PLACEMENT_3D('',#32112,#16140,#16141);
#12895=AXIS2_PLACEMENT_3D('',#32113,#16142,#16143);
#12896=AXIS2_PLACEMENT_3D('',#32114,#16144,#16145);
#12897=AXIS2_PLACEMENT_3D('',#32115,#16146,#16147);
#12898=AXIS2_PLACEMENT_3D('',#32116,#16148,#16149);
#12899=AXIS2_PLACEMENT_3D('',#32117,#16150,#16151);
#12900=AXIS2_PLACEMENT_3D('',#32118,#16152,#16153);
#12901=AXIS2_PLACEMENT_3D('',#32119,#16154,#16155);
#12902=AXIS2_PLACEMENT_3D('',#32120,#16156,#16157);
#12903=AXIS2_PLACEMENT_3D('',#32121,#16158,#16159);
#12904=AXIS2_PLACEMENT_3D('',#32122,#16160,#16161);
#12905=AXIS2_PLACEMENT_3D('',#32123,#16162,#16163);
#12906=AXIS2_PLACEMENT_3D('',#32124,#16164,#16165);
#12907=AXIS2_PLACEMENT_3D('',#32125,#16166,#16167);
#12908=AXIS2_PLACEMENT_3D('',#32126,#16168,#16169);
#12909=AXIS2_PLACEMENT_3D('',#32127,#16170,#16171);
#12910=AXIS2_PLACEMENT_3D('',#32128,#16172,#16173);
#12911=AXIS2_PLACEMENT_3D('',#32129,#16174,#16175);
#12912=AXIS2_PLACEMENT_3D('',#32130,#16176,#16177);
#12913=AXIS2_PLACEMENT_3D('',#32131,#16178,#16179);
#12914=AXIS2_PLACEMENT_3D('',#32132,#16180,#16181);
#12915=AXIS2_PLACEMENT_3D('',#32133,#16182,#16183);
#12916=AXIS2_PLACEMENT_3D('',#32134,#16184,#16185);
#12917=AXIS2_PLACEMENT_3D('',#32135,#16186,#16187);
#12918=AXIS2_PLACEMENT_3D('',#32136,#16188,#16189);
#12919=AXIS2_PLACEMENT_3D('',#32137,#16190,#16191);
#12920=AXIS2_PLACEMENT_3D('',#32138,#16192,#16193);
#12921=AXIS2_PLACEMENT_3D('',#32139,#16194,#16195);
#12922=AXIS2_PLACEMENT_3D('',#32140,#16196,#16197);
#12923=AXIS2_PLACEMENT_3D('',#32141,#16198,#16199);
#12924=AXIS2_PLACEMENT_3D('',#32142,#16200,#16201);
#12925=AXIS2_PLACEMENT_3D('',#32143,#16202,#16203);
#12926=AXIS2_PLACEMENT_3D('',#32146,#16206,#16207);
#12927=AXIS2_PLACEMENT_3D('',#32149,#16210,#16211);
#12928=AXIS2_PLACEMENT_3D('',#32155,#16216,#16217);
#12929=AXIS2_PLACEMENT_3D('',#32156,#16218,#16219);
#12930=AXIS2_PLACEMENT_3D('',#32157,#16220,#16221);
#12931=AXIS2_PLACEMENT_3D('',#32158,#16222,#16223);
#12932=AXIS2_PLACEMENT_3D('',#32159,#16224,#16225);
#12933=AXIS2_PLACEMENT_3D('',#32163,#16228,#16229);
#12934=AXIS2_PLACEMENT_3D('',#32164,#16230,#16231);
#12935=AXIS2_PLACEMENT_3D('',#32167,#16234,#16235);
#12936=AXIS2_PLACEMENT_3D('',#32171,#16238,#16239);
#12937=AXIS2_PLACEMENT_3D('',#32173,#16241,#16242);
#12938=AXIS2_PLACEMENT_3D('',#32175,#16244,#16245);
#12939=AXIS2_PLACEMENT_3D('',#32177,#16247,#16248);
#12940=AXIS2_PLACEMENT_3D('',#32179,#16250,#16251);
#12941=AXIS2_PLACEMENT_3D('',#32180,#16252,#16253);
#12942=AXIS2_PLACEMENT_3D('',#32181,#16254,#16255);
#12943=AXIS2_PLACEMENT_3D('',#32183,#16257,#16258);
#12944=AXIS2_PLACEMENT_3D('',#32185,#16260,#16261);
#12945=AXIS2_PLACEMENT_3D('',#32187,#16263,#16264);
#12946=AXIS2_PLACEMENT_3D('',#32189,#16266,#16267);
#12947=AXIS2_PLACEMENT_3D('',#32191,#16269,#16270);
#12948=AXIS2_PLACEMENT_3D('',#32193,#16272,#16273);
#12949=AXIS2_PLACEMENT_3D('',#32194,#16274,#16275);
#12995=DIRECTION('axis',(0.,0.,1.));
#12996=DIRECTION('refdir',(1.,0.,0.));
#12997=DIRECTION('center_axis',(0.,1.,0.));
#12998=DIRECTION('ref_axis',(0.,0.,1.));
#12999=DIRECTION('center_axis',(0.,1.,0.));
#13000=DIRECTION('ref_axis',(0.,0.,1.));
#13001=DIRECTION('',(0.,1.,0.));
#13002=DIRECTION('center_axis',(0.,1.,0.));
#13003=DIRECTION('ref_axis',(1.,0.,0.));
#13004=DIRECTION('center_axis',(0.,1.,0.));
#13005=DIRECTION('ref_axis',(0.,0.,1.));
#13006=DIRECTION('center_axis',(0.,1.,0.));
#13007=DIRECTION('ref_axis',(0.,0.,1.));
#13008=DIRECTION('',(0.,1.,0.));
#13009=DIRECTION('center_axis',(0.,1.,0.));
#13010=DIRECTION('ref_axis',(0.,0.,1.));
#13011=DIRECTION('center_axis',(0.,1.,0.));
#13012=DIRECTION('ref_axis',(0.,0.,1.));
#13013=DIRECTION('center_axis',(0.,1.,0.));
#13014=DIRECTION('ref_axis',(1.,0.,0.));
#13015=DIRECTION('',(0.,-1.,0.));
#13016=DIRECTION('center_axis',(0.,1.,0.));
#13017=DIRECTION('ref_axis',(0.,0.,1.));
#13018=DIRECTION('center_axis',(0.,1.,0.));
#13019=DIRECTION('ref_axis',(0.,0.,1.));
#13020=DIRECTION('center_axis',(0.,1.,0.));
#13021=DIRECTION('ref_axis',(0.,0.,1.));
#13022=DIRECTION('',(0.,1.,0.));
#13023=DIRECTION('center_axis',(0.,1.,0.));
#13024=DIRECTION('ref_axis',(0.,0.,1.));
#13025=DIRECTION('center_axis',(0.,1.,0.));
#13026=DIRECTION('ref_axis',(0.,0.,1.));
#13027=DIRECTION('center_axis',(0.,1.,0.));
#13028=DIRECTION('ref_axis',(0.,0.,1.));
#13029=DIRECTION('center_axis',(0.,1.,0.));
#13030=DIRECTION('ref_axis',(0.,0.,1.));
#13031=DIRECTION('center_axis',(-1.,0.,0.));
#13032=DIRECTION('ref_axis',(0.,0.,-1.));
#13033=DIRECTION('center_axis',(0.,-1.,0.));
#13034=DIRECTION('ref_axis',(0.,0.,1.));
#13035=DIRECTION('center_axis',(0.,1.,0.));
#13036=DIRECTION('ref_axis',(0.,0.,1.));
#13037=DIRECTION('center_axis',(0.,1.,0.));
#13038=DIRECTION('ref_axis',(0.,0.,1.));
#13039=DIRECTION('center_axis',(-1.,0.,0.));
#13040=DIRECTION('ref_axis',(0.,0.,-1.));
#13041=DIRECTION('center_axis',(0.,-1.,0.));
#13042=DIRECTION('ref_axis',(0.,0.,1.));
#13043=DIRECTION('center_axis',(0.,-1.,0.));
#13044=DIRECTION('ref_axis',(0.,0.,1.));
#13045=DIRECTION('center_axis',(0.,-1.,0.));
#13046=DIRECTION('ref_axis',(0.,0.,-1.));
#13047=DIRECTION('center_axis',(0.,-1.,0.));
#13048=DIRECTION('ref_axis',(0.,0.,-1.));
#13049=DIRECTION('center_axis',(-1.,0.,0.));
#13050=DIRECTION('ref_axis',(0.,0.,1.));
#13051=DIRECTION('center_axis',(0.,1.,0.));
#13052=DIRECTION('ref_axis',(0.,0.,-1.));
#13053=DIRECTION('center_axis',(0.,1.,0.));
#13054=DIRECTION('ref_axis',(0.,0.,1.));
#13055=DIRECTION('center_axis',(0.,1.,0.));
#13056=DIRECTION('ref_axis',(0.,0.,1.));
#13057=DIRECTION('center_axis',(-1.,0.,0.));
#13058=DIRECTION('ref_axis',(0.,0.,-1.));
#13059=DIRECTION('center_axis',(0.,-1.,0.));
#13060=DIRECTION('ref_axis',(0.,0.,1.));
#13061=DIRECTION('center_axis',(0.,-1.,0.));
#13062=DIRECTION('ref_axis',(0.,0.,1.));
#13063=DIRECTION('center_axis',(0.,1.,0.));
#13064=DIRECTION('ref_axis',(0.,0.,1.));
#13065=DIRECTION('center_axis',(0.,1.,0.));
#13066=DIRECTION('ref_axis',(0.,0.,1.));
#13067=DIRECTION('center_axis',(0.,0.,-1.));
#13068=DIRECTION('ref_axis',(-1.,0.,0.));
#13069=DIRECTION('center_axis',(0.,-1.,0.));
#13070=DIRECTION('ref_axis',(-7.40148683083437E-15,0.,1.));
#13071=DIRECTION('center_axis',(-0.528132444354927,0.,0.849162011173186));
#13072=DIRECTION('ref_axis',(0.849162011173186,0.,0.528132444354927));
#13073=DIRECTION('center_axis',(0.,1.,0.));
#13074=DIRECTION('ref_axis',(0.,0.,1.));
#13075=DIRECTION('center_axis',(0.,1.,0.));
#13076=DIRECTION('ref_axis',(0.,0.,1.));
#13077=DIRECTION('center_axis',(0.808689828521621,0.,0.588235294117645));
#13078=DIRECTION('ref_axis',(0.588235294117644,0.,-0.808689828521621));
#13079=DIRECTION('center_axis',(0.,-1.,0.));
#13080=DIRECTION('ref_axis',(0.,0.,1.));
#13081=DIRECTION('center_axis',(0.588235294117645,0.,0.808689828521621));
#13082=DIRECTION('ref_axis',(0.808689828521621,0.,-0.588235294117644));
#13083=DIRECTION('center_axis',(0.,1.,0.));
#13084=DIRECTION('ref_axis',(0.,0.,1.));
#13085=DIRECTION('center_axis',(0.,-1.,0.));
#13086=DIRECTION('ref_axis',(0.,0.,1.));
#13087=DIRECTION('center_axis',(0.528132444354927,1.46586199943601E-14,
-0.849162011173186));
#13088=DIRECTION('ref_axis',(-0.849162011173186,-1.56277058526093E-29,-0.528132444354927));
#13089=DIRECTION('center_axis',(0.,1.,0.));
#13090=DIRECTION('ref_axis',(0.,0.,1.));
#13091=DIRECTION('center_axis',(0.,0.,1.));
#13092=DIRECTION('ref_axis',(1.,0.,0.));
#13093=DIRECTION('center_axis',(0.,1.,0.));
#13094=DIRECTION('ref_axis',(0.,0.,1.));
#13095=DIRECTION('center_axis',(0.,-1.,0.));
#13096=DIRECTION('ref_axis',(0.,0.,1.));
#13097=DIRECTION('center_axis',(-0.588235294117631,0.,-0.80868982852163));
#13098=DIRECTION('ref_axis',(-0.80868982852163,0.,0.588235294117631));
#13099=DIRECTION('center_axis',(0.,1.,0.));
#13100=DIRECTION('ref_axis',(0.,0.,1.));
#13101=DIRECTION('center_axis',(-0.808689828521621,0.,-0.588235294117645));
#13102=DIRECTION('ref_axis',(-0.588235294117644,0.,0.808689828521621));
#13103=DIRECTION('center_axis',(0.,1.,0.));
#13104=DIRECTION('ref_axis',(0.,0.,1.));
#13105=DIRECTION('center_axis',(0.,1.,0.));
#13106=DIRECTION('ref_axis',(0.,0.,1.));
#13107=DIRECTION('center_axis',(0.,1.,0.));
#13108=DIRECTION('ref_axis',(0.,0.,1.));
#13109=DIRECTION('center_axis',(-1.,0.,0.));
#13110=DIRECTION('ref_axis',(0.,0.,-1.));
#13111=DIRECTION('center_axis',(0.,-1.,0.));
#13112=DIRECTION('ref_axis',(0.,0.,1.));
#13113=DIRECTION('center_axis',(0.,1.,0.));
#13114=DIRECTION('ref_axis',(0.,0.,1.));
#13115=DIRECTION('center_axis',(0.,1.,0.));
#13116=DIRECTION('ref_axis',(0.,0.,1.));
#13117=DIRECTION('center_axis',(-1.,0.,0.));
#13118=DIRECTION('ref_axis',(0.,0.,-1.));
#13119=DIRECTION('center_axis',(0.,-1.,0.));
#13120=DIRECTION('ref_axis',(0.,0.,1.));
#13121=DIRECTION('center_axis',(0.,-1.,0.));
#13122=DIRECTION('ref_axis',(0.,0.,1.));
#13123=DIRECTION('center_axis',(0.,-1.,0.));
#13124=DIRECTION('ref_axis',(0.,0.,-1.));
#13125=DIRECTION('center_axis',(0.,-1.,0.));
#13126=DIRECTION('ref_axis',(0.,0.,-1.));
#13127=DIRECTION('center_axis',(-1.,0.,0.));
#13128=DIRECTION('ref_axis',(0.,0.,1.));
#13129=DIRECTION('center_axis',(0.,1.,0.));
#13130=DIRECTION('ref_axis',(0.,0.,-1.));
#13131=DIRECTION('center_axis',(0.,1.,0.));
#13132=DIRECTION('ref_axis',(0.,0.,-1.));
#13133=DIRECTION('center_axis',(0.,1.,0.));
#13134=DIRECTION('ref_axis',(0.,0.,1.));
#13135=DIRECTION('center_axis',(0.,1.,0.));
#13136=DIRECTION('ref_axis',(0.,0.,1.));
#13137=DIRECTION('center_axis',(-1.,0.,0.));
#13138=DIRECTION('ref_axis',(0.,0.,-1.));
#13139=DIRECTION('center_axis',(0.,-1.,0.));
#13140=DIRECTION('ref_axis',(0.,0.,1.));
#13141=DIRECTION('center_axis',(0.,-1.,0.));
#13142=DIRECTION('ref_axis',(0.,0.,1.));
#13143=DIRECTION('center_axis',(0.,1.,0.));
#13144=DIRECTION('ref_axis',(0.,0.,1.));
#13145=DIRECTION('center_axis',(0.,1.,0.));
#13146=DIRECTION('ref_axis',(0.,0.,1.));
#13147=DIRECTION('center_axis',(0.528132444354927,0.,0.849162011173186));
#13148=DIRECTION('ref_axis',(0.849162011173186,0.,-0.528132444354927));
#13149=DIRECTION('center_axis',(0.,-1.,0.));
#13150=DIRECTION('ref_axis',(0.,0.,1.));
#13151=DIRECTION('center_axis',(0.,0.,-1.));
#13152=DIRECTION('ref_axis',(-1.,0.,0.));
#13153=DIRECTION('center_axis',(0.,1.,0.));
#13154=DIRECTION('ref_axis',(0.,0.,1.));
#13155=DIRECTION('center_axis',(0.,1.,0.));
#13156=DIRECTION('ref_axis',(0.,0.,1.));
#13157=DIRECTION('center_axis',(-0.588235294117645,0.,0.808689828521621));
#13158=DIRECTION('ref_axis',(0.808689828521621,0.,0.588235294117644));
#13159=DIRECTION('center_axis',(0.,-1.,0.));
#13160=DIRECTION('ref_axis',(-1.48029736616688E-15,0.,1.));
#13161=DIRECTION('center_axis',(-0.808689828521621,0.,0.588235294117645));
#13162=DIRECTION('ref_axis',(0.588235294117644,0.,0.808689828521621));
#13163=DIRECTION('center_axis',(0.,1.,0.));
#13164=DIRECTION('ref_axis',(0.,0.,1.));
#13165=DIRECTION('center_axis',(0.,-1.,0.));
#13166=DIRECTION('ref_axis',(0.,0.,1.));
#13167=DIRECTION('center_axis',(0.,0.,1.));
#13168=DIRECTION('ref_axis',(1.,0.,0.));
#13169=DIRECTION('center_axis',(0.,1.,0.));
#13170=DIRECTION('ref_axis',(0.,0.,1.));
#13171=DIRECTION('center_axis',(-0.528132444354927,0.,-0.849162011173186));
#13172=DIRECTION('ref_axis',(-0.849162011173186,0.,0.528132444354927));
#13173=DIRECTION('center_axis',(0.,1.,0.));
#13174=DIRECTION('ref_axis',(0.,0.,1.));
#13175=DIRECTION('center_axis',(0.,-1.,0.));
#13176=DIRECTION('ref_axis',(0.,0.,1.));
#13177=DIRECTION('center_axis',(0.808689828521621,0.,-0.588235294117645));
#13178=DIRECTION('ref_axis',(-0.588235294117644,0.,-0.808689828521621));
#13179=DIRECTION('center_axis',(0.,1.,0.));
#13180=DIRECTION('ref_axis',(0.,0.,1.));
#13181=DIRECTION('center_axis',(0.588235294117645,0.,-0.808689828521621));
#13182=DIRECTION('ref_axis',(-0.808689828521621,0.,-0.588235294117644));
#13183=DIRECTION('center_axis',(0.,1.,0.));
#13184=DIRECTION('ref_axis',(0.,0.,1.));
#13185=DIRECTION('center_axis',(0.,1.,0.));
#13186=DIRECTION('ref_axis',(0.,0.,1.));
#13187=DIRECTION('center_axis',(-1.,0.,0.));
#13188=DIRECTION('ref_axis',(0.,0.,-1.));
#13189=DIRECTION('center_axis',(0.,-1.,0.));
#13190=DIRECTION('ref_axis',(0.,0.,1.));
#13191=DIRECTION('center_axis',(0.,1.,0.));
#13192=DIRECTION('ref_axis',(0.,0.,1.));
#13193=DIRECTION('center_axis',(0.,1.,0.));
#13194=DIRECTION('ref_axis',(0.,0.,1.));
#13195=DIRECTION('center_axis',(-1.,0.,0.));
#13196=DIRECTION('ref_axis',(0.,0.,-1.));
#13197=DIRECTION('center_axis',(0.,-1.,0.));
#13198=DIRECTION('ref_axis',(0.,0.,1.));
#13199=DIRECTION('center_axis',(0.,-1.,0.));
#13200=DIRECTION('ref_axis',(0.,0.,-1.));
#13201=DIRECTION('center_axis',(0.,-1.,0.));
#13202=DIRECTION('ref_axis',(0.,0.,-1.));
#13203=DIRECTION('center_axis',(-1.,0.,0.));
#13204=DIRECTION('ref_axis',(0.,0.,1.));
#13205=DIRECTION('center_axis',(0.,1.,0.));
#13206=DIRECTION('ref_axis',(0.,0.,-1.));
#13207=DIRECTION('center_axis',(0.,1.,0.));
#13208=DIRECTION('ref_axis',(0.,0.,-1.));
#13209=DIRECTION('center_axis',(0.,1.,0.));
#13210=DIRECTION('ref_axis',(0.,0.,1.));
#13211=DIRECTION('center_axis',(0.,1.,0.));
#13212=DIRECTION('ref_axis',(0.,0.,1.));
#13213=DIRECTION('center_axis',(-1.,0.,0.));
#13214=DIRECTION('ref_axis',(0.,0.,-1.));
#13215=DIRECTION('center_axis',(0.,-1.,0.));
#13216=DIRECTION('ref_axis',(0.,0.,1.));
#13217=DIRECTION('center_axis',(0.,1.,0.));
#13218=DIRECTION('ref_axis',(0.,0.,1.));
#13219=DIRECTION('center_axis',(0.,1.,0.));
#13220=DIRECTION('ref_axis',(0.,0.,1.));
#13221=DIRECTION('center_axis',(-0.808689828521621,0.,-0.588235294117645));
#13222=DIRECTION('ref_axis',(-0.588235294117644,0.,0.808689828521621));
#13223=DIRECTION('center_axis',(0.,-1.,0.));
#13224=DIRECTION('ref_axis',(0.,0.,1.));
#13225=DIRECTION('center_axis',(0.,0.,1.));
#13226=DIRECTION('ref_axis',(1.,0.,0.));
#13227=DIRECTION('center_axis',(0.,1.,0.));
#13228=DIRECTION('ref_axis',(0.,0.,1.));
#13229=DIRECTION('center_axis',(0.,-1.,0.));
#13230=DIRECTION('ref_axis',(0.,0.,1.));
#13231=DIRECTION('center_axis',(0.,0.,-1.));
#13232=DIRECTION('ref_axis',(-1.,0.,0.));
#13233=DIRECTION('center_axis',(0.,1.,0.));
#13234=DIRECTION('ref_axis',(0.,0.,1.));
#13235=DIRECTION('center_axis',(0.808689828521621,0.,0.588235294117645));
#13236=DIRECTION('ref_axis',(0.588235294117644,0.,-0.808689828521621));
#13237=DIRECTION('center_axis',(0.,1.,0.));
#13238=DIRECTION('ref_axis',(0.,0.,1.));
#13239=DIRECTION('center_axis',(0.,1.,0.));
#13240=DIRECTION('ref_axis',(0.,0.,1.));
#13241=DIRECTION('center_axis',(-1.,0.,0.));
#13242=DIRECTION('ref_axis',(0.,0.,-1.));
#13243=DIRECTION('center_axis',(0.,-1.,0.));
#13244=DIRECTION('ref_axis',(0.,0.,1.));
#13245=DIRECTION('center_axis',(0.,1.,0.));
#13246=DIRECTION('ref_axis',(0.,0.,1.));
#13247=DIRECTION('center_axis',(0.,1.,0.));
#13248=DIRECTION('ref_axis',(0.,0.,1.));
#13249=DIRECTION('center_axis',(0.,1.,0.));
#13250=DIRECTION('ref_axis',(0.,0.,1.));
#13251=DIRECTION('center_axis',(-1.,0.,0.));
#13252=DIRECTION('ref_axis',(0.,0.,-1.));
#13253=DIRECTION('center_axis',(0.,-1.,0.));
#13254=DIRECTION('ref_axis',(0.,0.,1.));
#13255=DIRECTION('center_axis',(0.,-1.,0.));
#13256=DIRECTION('ref_axis',(0.,0.,1.));
#13257=DIRECTION('center_axis',(0.,-1.,0.));
#13258=DIRECTION('ref_axis',(0.,0.,-1.));
#13259=DIRECTION('center_axis',(0.,-1.,0.));
#13260=DIRECTION('ref_axis',(0.,0.,-1.));
#13261=DIRECTION('center_axis',(-1.,0.,0.));
#13262=DIRECTION('ref_axis',(0.,0.,1.));
#13263=DIRECTION('center_axis',(0.,1.,0.));
#13264=DIRECTION('ref_axis',(0.,0.,-1.));
#13265=DIRECTION('center_axis',(0.,1.,0.));
#13266=DIRECTION('ref_axis',(0.,0.,-1.));
#13267=DIRECTION('center_axis',(0.,1.,0.));
#13268=DIRECTION('ref_axis',(0.,0.,1.));
#13269=DIRECTION('center_axis',(0.,1.,0.));
#13270=DIRECTION('ref_axis',(0.,0.,1.));
#13271=DIRECTION('center_axis',(-1.,0.,0.));
#13272=DIRECTION('ref_axis',(0.,0.,-1.));
#13273=DIRECTION('center_axis',(0.,-1.,0.));
#13274=DIRECTION('ref_axis',(0.,0.,1.));
#13275=DIRECTION('center_axis',(0.,-1.,0.));
#13276=DIRECTION('ref_axis',(0.,0.,1.));
#13277=DIRECTION('center_axis',(0.,1.,0.));
#13278=DIRECTION('ref_axis',(0.,0.,1.));
#13279=DIRECTION('center_axis',(0.,1.,0.));
#13280=DIRECTION('ref_axis',(0.,0.,1.));
#13281=DIRECTION('center_axis',(0.724563445309589,-1.0182026595163E-14,
0.68920810625028));
#13282=DIRECTION('ref_axis',(0.689208106250281,9.56120314610186E-29,-0.724563445309589));
#13283=DIRECTION('center_axis',(0.,-1.,0.));
#13284=DIRECTION('ref_axis',(0.,0.,-1.));
#13285=DIRECTION('center_axis',(0.724563445309596,-1.34013438274573E-14,
-0.689208106250273));
#13286=DIRECTION('ref_axis',(0.689208106250273,-2.63677968348471E-14,0.724563445309596));
#13287=DIRECTION('center_axis',(0.,1.,0.));
#13288=DIRECTION('ref_axis',(0.,0.,1.));
#13289=DIRECTION('center_axis',(0.,1.,0.));
#13290=DIRECTION('ref_axis',(0.,0.,1.));
#13291=DIRECTION('center_axis',(0.724563445309589,1.0182026595163E-14,0.68920810625028));
#13292=DIRECTION('ref_axis',(0.68920810625028,-9.81293834229342E-29,-0.724563445309589));
#13293=DIRECTION('center_axis',(0.,-1.,0.));
#13294=DIRECTION('ref_axis',(-2.66454616931092E-15,0.,1.));
#13295=DIRECTION('center_axis',(0.724563445309603,9.43334816904809E-15,
-0.689208106250266));
#13296=DIRECTION('ref_axis',(0.689208106250266,-3.33066907387548E-14,0.724563445309603));
#13297=DIRECTION('center_axis',(0.,1.,0.));
#13298=DIRECTION('ref_axis',(0.,0.,1.));
#13299=DIRECTION('center_axis',(0.,1.,0.));
#13300=DIRECTION('ref_axis',(0.,0.,1.));
#13301=DIRECTION('center_axis',(0.707106781186548,0.,-0.707106781186548));
#13302=DIRECTION('ref_axis',(-0.707106781186548,0.,-0.707106781186548));
#13303=DIRECTION('center_axis',(0.,-1.,0.));
#13304=DIRECTION('ref_axis',(0.,0.,1.));
#13305=DIRECTION('center_axis',(-0.707106781186541,0.,0.707106781186554));
#13306=DIRECTION('ref_axis',(0.707106781186555,0.,0.707106781186541));
#13307=DIRECTION('center_axis',(0.,1.,0.));
#13308=DIRECTION('ref_axis',(0.,0.,1.));
#13309=DIRECTION('center_axis',(0.,1.,0.));
#13310=DIRECTION('ref_axis',(0.,0.,1.));
#13311=DIRECTION('center_axis',(0.707106781186548,9.81307786677359E-15,
0.707106781186548));
#13312=DIRECTION('ref_axis',(0.707106781186548,3.73353565333889E-32,-0.707106781186548));
#13313=DIRECTION('center_axis',(0.,-1.,0.));
#13314=DIRECTION('ref_axis',(0.,0.,1.));
#13315=DIRECTION('center_axis',(-0.707106781186548,9.81307786677359E-15,
-0.707106781186548));
#13316=DIRECTION('ref_axis',(-0.707106781186548,3.73353565333889E-32,0.707106781186548));
#13317=DIRECTION('center_axis',(0.,-1.,0.));
#13318=DIRECTION('ref_axis',(0.,0.,-1.));
#13319=DIRECTION('center_axis',(0.,-1.,0.));
#13320=DIRECTION('ref_axis',(0.,0.,-1.));
#13321=DIRECTION('center_axis',(-0.707106781186548,-9.81307786677366E-15,
-0.707106781186548));
#13322=DIRECTION('ref_axis',(-0.707106781186548,-1.63063665584286E-31,0.707106781186548));
#13323=DIRECTION('center_axis',(0.,1.,0.));
#13324=DIRECTION('ref_axis',(0.,0.,-1.));
#13325=DIRECTION('center_axis',(0.707106781186548,-9.81307786677359E-15,
0.707106781186548));
#13326=DIRECTION('ref_axis',(0.707106781186548,-3.73353565333889E-32,-0.707106781186548));
#13327=DIRECTION('center_axis',(0.,-1.,0.));
#13328=DIRECTION('ref_axis',(0.,0.,-1.));
#13329=DIRECTION('center_axis',(0.,-1.,0.));
#13330=DIRECTION('ref_axis',(0.,0.,-1.));
#13331=DIRECTION('center_axis',(-0.707106781186548,0.,0.707106781186548));
#13332=DIRECTION('ref_axis',(0.707106781186548,0.,0.707106781186548));
#13333=DIRECTION('center_axis',(0.,1.,0.));
#13334=DIRECTION('ref_axis',(0.,0.,-1.));
#13335=DIRECTION('center_axis',(0.707106781186534,0.,-0.707106781186561));
#13336=DIRECTION('ref_axis',(-0.707106781186561,0.,-0.707106781186534));
#13337=DIRECTION('center_axis',(0.,1.,0.));
#13338=DIRECTION('ref_axis',(0.,0.,1.));
#13339=DIRECTION('center_axis',(-1.47242188377274E-14,1.,-1.47242188377274E-14));
#13340=DIRECTION('ref_axis',(7.97092275109852E-30,1.47242188377274E-14,
1.));
#13341=DIRECTION('',(0.,-1.,0.));
#13342=DIRECTION('center_axis',(2.01169630281381E-14,1.,-1.91353484389564E-14));
#13343=DIRECTION('ref_axis',(1.,-2.01169630281381E-14,-3.99449913460622E-29));
#13344=DIRECTION('',(0.,1.,0.));
#13345=DIRECTION('center_axis',(0.,1.,0.));
#13346=DIRECTION('ref_axis',(0.,0.,1.));
#13347=DIRECTION('center_axis',(1.50877222711036E-14,1.,1.43515113292173E-14));
#13348=DIRECTION('ref_axis',(-1.,1.50877222711036E-14,-2.55233473732763E-30));
#13349=DIRECTION('',(0.,-1.,0.));
#13350=DIRECTION('center_axis',(-1.9632291783637E-14,1.,1.9632291783637E-14));
#13351=DIRECTION('ref_axis',(5.04975666092008E-29,1.9632291783637E-14,-1.));
#13352=DIRECTION('',(0.,1.,0.));
#13353=DIRECTION('center_axis',(0.,-1.,0.));
#13354=DIRECTION('ref_axis',(0.,0.,-1.));
#13355=DIRECTION('center_axis',(0.,1.,0.));
#13356=DIRECTION('ref_axis',(0.,0.,-1.));
#13357=DIRECTION('',(0.,1.,0.));
#13358=DIRECTION('center_axis',(0.,1.,0.));
#13359=DIRECTION('ref_axis',(0.,0.,1.));
#13360=DIRECTION('',(0.,-1.,0.));
#13361=DIRECTION('center_axis',(0.,-1.,0.));
#13362=DIRECTION('ref_axis',(0.,0.,-1.));
#13363=DIRECTION('center_axis',(-0.456384763068618,0.,-0.8897825285084));
#13364=DIRECTION('ref_axis',(-0.8897825285084,0.,0.456384763068618));
#13365=DIRECTION('center_axis',(0.,-1.,0.));
#13366=DIRECTION('ref_axis',(0.,0.,-1.));
#13367=DIRECTION('center_axis',(-0.313163806483749,0.,0.949699126201877));
#13368=DIRECTION('ref_axis',(-0.949699126201877,0.,-0.313163806483749));
#13369=DIRECTION('center_axis',(0.,-1.,0.));
#13370=DIRECTION('ref_axis',(0.,0.,-1.));
#13371=DIRECTION('center_axis',(0.,-1.,0.));
#13372=DIRECTION('ref_axis',(2.22044604925031E-14,0.,1.));
#13373=DIRECTION('',(0.,1.,0.));
#13374=DIRECTION('center_axis',(0.,-1.,0.));
#13375=DIRECTION('ref_axis',(0.,0.,-1.));
#13376=DIRECTION('',(0.,-1.,0.));
#13377=DIRECTION('center_axis',(0.,-1.,0.));
#13378=DIRECTION('ref_axis',(0.,0.,-1.));
#13379=DIRECTION('center_axis',(0.,-1.,0.));
#13380=DIRECTION('ref_axis',(0.,0.,-1.));
#13381=DIRECTION('',(0.,1.,0.));
#13382=DIRECTION('center_axis',(0.,-1.,0.));
#13383=DIRECTION('ref_axis',(2.22044604925031E-14,0.,1.));
#13384=DIRECTION('',(0.,-1.,0.));
#13385=DIRECTION('center_axis',(0.,-1.,0.));
#13386=DIRECTION('ref_axis',(0.,0.,-1.));
#13387=DIRECTION('center_axis',(0.,-1.,0.));
#13388=DIRECTION('ref_axis',(0.,0.,1.));
#13389=DIRECTION('',(0.,1.,0.));
#13390=DIRECTION('center_axis',(0.,-1.,0.));
#13391=DIRECTION('ref_axis',(0.,0.,-1.));
#13392=DIRECTION('',(0.,-1.,0.));
#13393=DIRECTION('center_axis',(0.,-1.,0.));
#13394=DIRECTION('ref_axis',(0.,0.,-1.));
#13395=DIRECTION('center_axis',(0.,-1.,0.));
#13396=DIRECTION('ref_axis',(0.,0.,-1.));
#13397=DIRECTION('',(0.,1.,0.));
#13398=DIRECTION('center_axis',(0.,-1.,0.));
#13399=DIRECTION('ref_axis',(0.,0.,1.));
#13400=DIRECTION('',(0.,-1.,0.));
#13401=DIRECTION('center_axis',(0.,1.,0.));
#13402=DIRECTION('ref_axis',(0.,0.,1.));
#13403=DIRECTION('center_axis',(0.,-1.,0.));
#13404=DIRECTION('ref_axis',(0.,0.,1.));
#13405=DIRECTION('center_axis',(-0.313163806483745,0.,0.949699126201878));
#13406=DIRECTION('ref_axis',(0.949699126201878,0.,0.313163806483745));
#13407=DIRECTION('center_axis',(0.,1.,0.));
#13408=DIRECTION('ref_axis',(0.,0.,1.));
#13409=DIRECTION('center_axis',(0.456384763068627,0.,0.889782528508396));
#13410=DIRECTION('ref_axis',(0.889782528508395,0.,-0.456384763068626));
#13411=DIRECTION('center_axis',(0.,1.,0.));
#13412=DIRECTION('ref_axis',(0.,0.,1.));
#13413=DIRECTION('center_axis',(0.,1.,0.));
#13414=DIRECTION('ref_axis',(0.,0.,1.));
#13415=DIRECTION('center_axis',(0.,0.,1.));
#13416=DIRECTION('ref_axis',(1.,0.,0.));
#13417=DIRECTION('center_axis',(0.,-1.,0.));
#13418=DIRECTION('ref_axis',(-1.48029736616687E-14,0.,1.));
#13419=DIRECTION('center_axis',(0.808689828521621,0.,-0.588235294117645));
#13420=DIRECTION('ref_axis',(-0.588235294117644,0.,-0.808689828521621));
#13421=DIRECTION('center_axis',(0.,1.,0.));
#13422=DIRECTION('ref_axis',(0.,0.,1.));
#13423=DIRECTION('center_axis',(0.,-1.,0.));
#13424=DIRECTION('ref_axis',(0.,0.,1.));
#13425=DIRECTION('center_axis',(-0.808689828521621,0.,0.588235294117645));
#13426=DIRECTION('ref_axis',(0.588235294117644,0.,0.808689828521621));
#13427=DIRECTION('center_axis',(0.,1.,0.));
#13428=DIRECTION('ref_axis',(0.,0.,1.));
#13429=DIRECTION('center_axis',(0.,0.,-1.));
#13430=DIRECTION('ref_axis',(-1.,0.,0.));
#13431=DIRECTION('center_axis',(0.,1.,0.));
#13432=DIRECTION('ref_axis',(1.,0.,7.40148683083437E-15));
#13433=DIRECTION('center_axis',(0.,-1.,0.));
#13434=DIRECTION('ref_axis',(0.,0.,1.));
#13435=DIRECTION('',(0.,-1.,0.));
#13436=DIRECTION('center_axis',(0.,1.,0.));
#13437=DIRECTION('ref_axis',(0.,0.,1.));
#13438=DIRECTION('',(0.,1.,0.));
#13439=DIRECTION('center_axis',(0.,1.,0.));
#13440=DIRECTION('ref_axis',(1.,0.,1.11022302462516E-14));
#13441=DIRECTION('center_axis',(0.,1.,0.));
#13442=DIRECTION('ref_axis',(0.,0.,1.));
#13443=DIRECTION('',(0.,1.,0.));
#13444=DIRECTION('center_axis',(0.,-1.,0.));
#13445=DIRECTION('ref_axis',(-3.1720657846433E-15,0.,1.));
#13446=DIRECTION('',(0.,-1.,0.));
#13447=DIRECTION('center_axis',(0.,-1.,0.));
#13448=DIRECTION('ref_axis',(-1.,0.,-9.86864910777916E-15));
#13449=DIRECTION('',(0.,-1.,0.));
#13450=DIRECTION('center_axis',(0.,-1.,0.));
#13451=DIRECTION('ref_axis',(-1.,0.,-9.86864910777916E-15));
#13452=DIRECTION('',(0.,-1.,0.));
#13453=DIRECTION('center_axis',(0.,-1.,0.));
#13454=DIRECTION('ref_axis',(-1.,0.,-7.40148683083437E-15));
#13455=DIRECTION('',(0.,1.,0.));
#13456=DIRECTION('center_axis',(0.,1.,0.));
#13457=DIRECTION('ref_axis',(0.,0.,-1.));
#13458=DIRECTION('',(0.,-1.,0.));
#13459=DIRECTION('center_axis',(0.,1.,0.));
#13460=DIRECTION('ref_axis',(0.,0.,-1.));
#13461=DIRECTION('center_axis',(0.,-1.,0.));
#13462=DIRECTION('ref_axis',(0.,0.,1.));
#13463=DIRECTION('',(0.,-1.,0.));
#13464=DIRECTION('center_axis',(0.,1.,0.));
#13465=DIRECTION('ref_axis',(0.,0.,1.));
#13466=DIRECTION('',(0.,1.,0.));
#13467=DIRECTION('center_axis',(0.,1.,0.));
#13468=DIRECTION('ref_axis',(0.,0.,-1.));
#13469=DIRECTION('center_axis',(0.,1.,0.));
#13470=DIRECTION('ref_axis',(0.,0.,1.));
#13471=DIRECTION('',(0.,1.,0.));
#13472=DIRECTION('center_axis',(0.,-1.,0.));
#13473=DIRECTION('ref_axis',(0.,0.,1.));
#13474=DIRECTION('',(0.,-1.,0.));
#13475=DIRECTION('center_axis',(0.,-1.,0.));
#13476=DIRECTION('ref_axis',(0.,0.,1.));
#13477=DIRECTION('',(0.,-1.,0.));
#13478=DIRECTION('center_axis',(0.,-1.,0.));
#13479=DIRECTION('ref_axis',(0.,0.,1.));
#13480=DIRECTION('',(0.,-1.,0.));
#13481=DIRECTION('center_axis',(0.,-1.,0.));
#13482=DIRECTION('ref_axis',(0.,0.,1.));
#13483=DIRECTION('center_axis',(0.,1.,0.));
#13484=DIRECTION('ref_axis',(3.55274999902112E-15,0.,-1.));
#13485=DIRECTION('center_axis',(0.,1.,0.));
#13486=DIRECTION('ref_axis',(0.,0.,-1.));
#13487=DIRECTION('center_axis',(0.,-1.,0.));
#13488=DIRECTION('ref_axis',(0.,0.,1.));
#13489=DIRECTION('',(0.,1.,0.));
#13490=DIRECTION('center_axis',(0.,1.,0.));
#13491=DIRECTION('ref_axis',(0.,0.,-1.));
#13492=DIRECTION('',(0.,-1.,0.));
#13493=DIRECTION('center_axis',(0.,1.,0.));
#13494=DIRECTION('ref_axis',(-1.,0.,0.));
#13495=DIRECTION('center_axis',(0.,-1.,0.));
#13496=DIRECTION('ref_axis',(0.,0.,1.));
#13497=DIRECTION('',(0.,-1.,0.));
#13498=DIRECTION('center_axis',(0.,1.,0.));
#13499=DIRECTION('ref_axis',(0.,0.,1.));
#13500=DIRECTION('',(0.,1.,0.));
#13501=DIRECTION('center_axis',(0.,1.,0.));
#13502=DIRECTION('ref_axis',(-1.,0.,-3.1720657846433E-15));
#13503=DIRECTION('',(0.,1.,0.));
#13504=DIRECTION('',(0.,-1.,0.));
#13505=DIRECTION('center_axis',(0.,-1.,0.));
#13506=DIRECTION('ref_axis',(1.,0.,2.46716227694479E-15));
#13507=DIRECTION('',(0.,-1.,0.));
#13508=DIRECTION('center_axis',(0.,-1.,0.));
#13509=DIRECTION('ref_axis',(1.,0.,2.46716227694479E-15));
#13510=DIRECTION('',(0.,-1.,0.));
#13511=DIRECTION('center_axis',(0.,-1.,0.));
#13512=DIRECTION('ref_axis',(1.,0.,3.49157860180481E-15));
#13513=DIRECTION('center_axis',(0.,-1.,0.));
#13514=DIRECTION('ref_axis',(0.,0.,-1.));
#13515=DIRECTION('center_axis',(0.,1.,0.));
#13516=DIRECTION('ref_axis',(1.77625045523519E-15,0.,-1.));
#13517=DIRECTION('center_axis',(0.,1.,0.));
#13518=DIRECTION('ref_axis',(-5.32900045425631E-15,0.,-1.));
#13519=DIRECTION('center_axis',(0.,-1.,0.));
#13520=DIRECTION('ref_axis',(1.,0.,0.));
#13521=DIRECTION('center_axis',(0.,-1.,0.));
#13522=DIRECTION('ref_axis',(0.,0.,1.));
#13523=DIRECTION('',(0.,1.,0.));
#13524=DIRECTION('',(0.,-1.,0.));
#13525=DIRECTION('center_axis',(0.,1.,0.));
#13526=DIRECTION('ref_axis',(0.,0.,1.));
#13527=DIRECTION('',(0.,-1.,0.));
#13528=DIRECTION('',(0.,1.,0.));
#13529=DIRECTION('center_axis',(0.,1.,0.));
#13530=DIRECTION('ref_axis',(0.,0.,1.));
#13531=DIRECTION('',(0.,1.,0.));
#13532=DIRECTION('',(0.,-1.,0.));
#13533=DIRECTION('center_axis',(0.,-1.,0.));
#13534=DIRECTION('ref_axis',(0.,0.,-1.));
#13535=DIRECTION('center_axis',(0.,-1.,0.));
#13536=DIRECTION('ref_axis',(9.28647839630166E-15,0.,-1.));
#13537=DIRECTION('center_axis',(0.,1.,0.));
#13538=DIRECTION('ref_axis',(0.,0.,1.));
#13539=DIRECTION('center_axis',(0.,-1.,0.));
#13540=DIRECTION('ref_axis',(-0.996210606090467,0.,-0.086973721967411));
#13541=DIRECTION('center_axis',(0.,-1.,0.));
#13542=DIRECTION('ref_axis',(-1.,0.,-9.25030661388722E-15));
#13543=DIRECTION('center_axis',(0.,1.,0.));
#13544=DIRECTION('ref_axis',(0.,0.,1.));
#13545=DIRECTION('center_axis',(-4.73766340797087E-15,-1.,7.24463663858484E-14));
#13546=DIRECTION('ref_axis',(-0.0869737219674231,7.25670419811831E-14,0.996210606090466));
#13547=DIRECTION('',(0.,-1.,0.));
#13548=DIRECTION('center_axis',(2.63036692491839E-16,1.,-1.20858413416517E-14));
#13549=DIRECTION('ref_axis',(-1.28631872178907E-14,1.20792265079216E-14,
1.));
#13550=DIRECTION('center_axis',(0.,-1.,0.));
#13551=DIRECTION('ref_axis',(0.,0.,1.));
#13552=DIRECTION('',(0.,-1.,0.));
#13553=DIRECTION('center_axis',(0.,-1.,0.));
#13554=DIRECTION('ref_axis',(0.,0.,-1.));
#13555=DIRECTION('',(0.,1.,0.));
#13556=DIRECTION('center_axis',(0.,-1.,0.));
#13557=DIRECTION('ref_axis',(0.,0.,-1.));
#13558=DIRECTION('',(0.,-1.,0.));
#13559=DIRECTION('center_axis',(0.,-1.,0.));
#13560=DIRECTION('ref_axis',(0.,0.,-1.));
#13561=DIRECTION('center_axis',(0.,-1.,0.));
#13562=DIRECTION('ref_axis',(0.,0.,1.));
#13563=DIRECTION('center_axis',(-4.57877760372757E-17,1.,-2.10629550201326E-15));
#13564=DIRECTION('ref_axis',(-0.996210606090468,1.37524400469719E-16,0.0869737219674006));
#13565=DIRECTION('center_axis',(-7.24349194418465E-14,1.,-5.26423728347428E-15));
#13566=DIRECTION('ref_axis',(-1.,-7.24295175807043E-14,-2.03897830519296E-14));
#13567=DIRECTION('center_axis',(0.,-1.,0.));
#13568=DIRECTION('ref_axis',(8.88066502056514E-16,0.,1.));
#13569=DIRECTION('',(0.,-1.,0.));
#13570=DIRECTION('center_axis',(0.,-1.,0.));
#13571=DIRECTION('ref_axis',(0.,0.,-1.));
#13572=DIRECTION('center_axis',(0.,-1.,0.));
#13573=DIRECTION('ref_axis',(0.,0.,-1.));
#13574=DIRECTION('',(0.,-1.,0.));
#13575=DIRECTION('center_axis',(0.,-1.,0.));
#13576=DIRECTION('ref_axis',(0.,0.,-1.));
#13577=DIRECTION('',(0.,1.,0.));
#13578=DIRECTION('center_axis',(0.,-1.,0.));
#13579=DIRECTION('ref_axis',(0.,0.,1.));
#13580=DIRECTION('center_axis',(0.,1.,0.));
#13581=DIRECTION('ref_axis',(-0.0869737219674249,0.,-0.996210606090466));
#13582=DIRECTION('center_axis',(-2.63036692491925E-16,1.,1.20858413416538E-14));
#13583=DIRECTION('ref_axis',(1.108575596911E-14,1.20792265079196E-14,-1.));
#13584=DIRECTION('center_axis',(0.,-1.,0.));
#13585=DIRECTION('ref_axis',(0.,0.,1.));
#13586=DIRECTION('',(0.,-1.,0.));
#13587=DIRECTION('center_axis',(0.,-1.,0.));
#13588=DIRECTION('ref_axis',(0.,0.,-1.));
#13589=DIRECTION('',(0.,1.,0.));
#13590=DIRECTION('center_axis',(0.,-1.,0.));
#13591=DIRECTION('ref_axis',(0.,0.,-1.));
#13592=DIRECTION('center_axis',(0.,-1.,0.));
#13593=DIRECTION('ref_axis',(0.,0.,-1.));
#13594=DIRECTION('',(0.,1.,0.));
#13595=DIRECTION('center_axis',(0.,-1.,0.));
#13596=DIRECTION('ref_axis',(-2.66447930027857E-15,0.,1.));
#13597=DIRECTION('center_axis',(-1.20629474536324E-14,1.,1.31618444349839E-15));
#13598=DIRECTION('ref_axis',(0.996210606090468,1.21250679747461E-14,-0.0869737219674049));
#13599=DIRECTION('center_axis',(-1.21087352296684E-14,1.,7.90111058514839E-16));
#13600=DIRECTION('ref_axis',(1.,1.21021472413359E-14,-7.38620634189485E-15));
#13601=DIRECTION('center_axis',(0.,-1.,0.));
#13602=DIRECTION('ref_axis',(-1.77641279822206E-15,0.,1.));
#13603=DIRECTION('center_axis',(0.,-1.,0.));
#13604=DIRECTION('ref_axis',(0.,0.,-1.));
#13605=DIRECTION('',(0.,1.,0.));
#13606=DIRECTION('center_axis',(0.,-1.,0.));
#13607=DIRECTION('ref_axis',(0.,0.,-1.));
#13608=DIRECTION('',(0.,-1.,0.));
#13609=DIRECTION('center_axis',(0.,-1.,0.));
#13610=DIRECTION('ref_axis',(0.,0.,-1.));
#13611=DIRECTION('',(0.,1.,0.));
#13612=DIRECTION('center_axis',(0.,-1.,0.));
#13613=DIRECTION('ref_axis',(1.77641279822206E-15,0.,1.));
#13614=DIRECTION('center_axis',(5.26073384983703E-16,1.,2.4171682683304E-14));
#13615=DIRECTION('ref_axis',(0.086973721967389,-2.41355322824308E-14,0.996210606090469));
#13616=DIRECTION('center_axis',(-7.36903131392929E-15,-1.,-1.44938520547765E-13));
#13617=DIRECTION('ref_axis',(1.04987703118978E-14,-1.44950718095046E-13,
1.));
#13618=DIRECTION('center_axis',(0.,1.,0.));
#13619=DIRECTION('ref_axis',(0.,0.,1.));
#13620=DIRECTION('center_axis',(-1.4493852054775E-13,-1.,-7.36903131392888E-15));
#13621=DIRECTION('ref_axis',(0.996210606090468,-1.45042401028705E-13,0.0869737219673961));
#13622=DIRECTION('center_axis',(7.24463663858355E-14,-1.,-4.73766340796999E-15));
#13623=DIRECTION('ref_axis',(1.,7.24295175807267E-14,1.93479640910857E-14));
#13624=DIRECTION('center_axis',(0.,1.,0.));
#13625=DIRECTION('ref_axis',(0.,0.,1.));
#13626=DIRECTION('center_axis',(0.,-1.,0.));
#13627=DIRECTION('ref_axis',(0.0869737219673973,0.,-0.996210606090468));
#13628=DIRECTION('center_axis',(0.,-1.,0.));
#13629=DIRECTION('ref_axis',(0.,0.,-1.));
#13630=DIRECTION('',(0.,-1.,0.));
#13631=DIRECTION('center_axis',(0.,-1.,0.));
#13632=DIRECTION('ref_axis',(0.,0.,-1.));
#13633=DIRECTION('',(0.,-1.,0.));
#13634=DIRECTION('center_axis',(0.,-1.,0.));
#13635=DIRECTION('ref_axis',(0.,0.,-1.));
#13636=DIRECTION('center_axis',(0.,-1.,0.));
#13637=DIRECTION('ref_axis',(0.,0.,-1.));
#13638=DIRECTION('center_axis',(0.,1.,0.));
#13639=DIRECTION('ref_axis',(0.,0.,-1.));
#13640=DIRECTION('center_axis',(0.,1.,0.));
#13641=DIRECTION('ref_axis',(0.,0.,-1.));
#13642=DIRECTION('center_axis',(0.,-1.,0.));
#13643=DIRECTION('ref_axis',(0.,0.,-1.));
#13644=DIRECTION('center_axis',(0.,-1.,0.));
#13645=DIRECTION('ref_axis',(0.,0.,1.));
#13646=DIRECTION('',(0.,1.,0.));
#13647=DIRECTION('',(0.,-1.,0.));
#13648=DIRECTION('center_axis',(0.,1.,0.));
#13649=DIRECTION('ref_axis',(0.,0.,1.));
#13650=DIRECTION('center_axis',(0.,1.,0.));
#13651=DIRECTION('ref_axis',(0.,0.,-1.));
#13652=DIRECTION('',(0.,1.,0.));
#13653=DIRECTION('center_axis',(0.,1.,0.));
#13654=DIRECTION('ref_axis',(0.,0.,1.));
#13655=DIRECTION('',(0.,1.,0.));
#13656=DIRECTION('center_axis',(0.,1.,0.));
#13657=DIRECTION('ref_axis',(0.,0.,1.));
#13658=DIRECTION('',(3.29601953873307E-15,0.,-1.));
#13659=DIRECTION('',(1.,0.,0.));
#13660=DIRECTION('',(-3.46944695195362E-15,0.,-1.));
#13661=DIRECTION('',(0.,0.,1.));
#13662=DIRECTION('center_axis',(0.,1.,0.));
#13663=DIRECTION('ref_axis',(0.,0.,1.));
#13664=DIRECTION('center_axis',(0.,-1.,0.));
#13665=DIRECTION('ref_axis',(1.11022302462516E-14,0.,1.));
#13666=DIRECTION('',(-1.,0.,-1.03892784411108E-15));
#13667=DIRECTION('center_axis',(0.,-1.,0.));
#13668=DIRECTION('ref_axis',(0.,0.,1.));
#13669=DIRECTION('center_axis',(0.,1.,0.));
#13670=DIRECTION('ref_axis',(0.,0.,1.));
#13671=DIRECTION('center_axis',(0.,-1.,0.));
#13672=DIRECTION('ref_axis',(5.55111512312578E-15,0.,1.));
#13673=DIRECTION('',(0.,0.,1.));
#13674=DIRECTION('',(-3.46944695195362E-15,0.,-1.));
#13675=DIRECTION('',(1.,0.,0.));
#13676=DIRECTION('',(3.29601953873307E-15,0.,-1.));
#13677=DIRECTION('center_axis',(0.,1.,0.));
#13678=DIRECTION('ref_axis',(0.,0.,1.));
#13679=DIRECTION('',(-1.,0.,1.95461800110063E-16));
#13680=DIRECTION('center_axis',(0.,1.,0.));
#13681=DIRECTION('ref_axis',(0.,0.,1.));
#13682=DIRECTION('',(0.,0.,1.));
#13683=DIRECTION('center_axis',(0.,1.,0.));
#13684=DIRECTION('ref_axis',(0.,0.,1.));
#13685=DIRECTION('',(1.,0.,-1.95461800110063E-16));
#13686=DIRECTION('center_axis',(0.,1.,0.));
#13687=DIRECTION('ref_axis',(0.,0.,1.));
#13688=DIRECTION('center_axis',(0.,1.,0.));
#13689=DIRECTION('ref_axis',(0.,0.,1.));
#13690=DIRECTION('center_axis',(0.,-1.,0.));
#13691=DIRECTION('ref_axis',(1.38777878078144E-14,0.,1.));
#13692=DIRECTION('',(-1.,0.,-1.04744440165294E-14));
#13693=DIRECTION('center_axis',(0.,-1.,0.));
#13694=DIRECTION('ref_axis',(-5.55111512312578E-15,0.,1.));
#13695=DIRECTION('center_axis',(0.,1.,0.));
#13696=DIRECTION('ref_axis',(0.,0.,1.));
#13697=DIRECTION('',(1.15133718606405E-14,0.,-1.));
#13698=DIRECTION('center_axis',(0.,-1.,0.));
#13699=DIRECTION('ref_axis',(0.,0.,1.));
#13700=DIRECTION('center_axis',(0.,1.,0.));
#13701=DIRECTION('ref_axis',(0.,0.,1.));
#13702=DIRECTION('center_axis',(0.,-1.,0.));
#13703=DIRECTION('ref_axis',(0.,0.,1.));
#13704=DIRECTION('',(1.,0.,3.49148133884313E-15));
#13705=DIRECTION('center_axis',(0.,-1.,0.));
#13706=DIRECTION('ref_axis',(0.,0.,1.));
#13707=DIRECTION('center_axis',(0.,-1.,0.));
#13708=DIRECTION('ref_axis',(0.,0.,1.));
#13709=DIRECTION('',(-4.53040918295421E-15,0.,1.));
#13710=DIRECTION('center_axis',(0.,1.,0.));
#13711=DIRECTION('ref_axis',(0.,0.,1.));
#13712=DIRECTION('',(0.,0.,-1.));
#13713=DIRECTION('center_axis',(0.,-1.,0.));
#13714=DIRECTION('ref_axis',(0.,0.,1.));
#13715=DIRECTION('center_axis',(0.,-1.,0.));
#13716=DIRECTION('ref_axis',(5.55111512312578E-15,0.,1.));
#13717=DIRECTION('',(1.,0.,1.03892784411108E-15));
#13718=DIRECTION('center_axis',(0.,-1.,0.));
#13719=DIRECTION('ref_axis',(0.,0.,1.));
#13720=DIRECTION('center_axis',(0.,-1.,0.));
#13721=DIRECTION('ref_axis',(-3.55264982748976E-15,0.,1.));
#13722=DIRECTION('',(-1.,0.,0.));
#13723=DIRECTION('center_axis',(0.,-1.,0.));
#13724=DIRECTION('ref_axis',(0.,0.,1.));
#13725=DIRECTION('',(0.,0.,-1.));
#13726=DIRECTION('center_axis',(0.,-1.,0.));
#13727=DIRECTION('ref_axis',(1.77632491374488E-15,0.,1.));
#13728=DIRECTION('',(1.,0.,0.));
#13729=DIRECTION('center_axis',(0.,-1.,0.));
#13730=DIRECTION('ref_axis',(0.,0.,1.));
#13731=DIRECTION('',(-3.49148133884313E-15,0.,1.));
#13732=DIRECTION('center_axis',(-1.,0.,-3.29601953873307E-15));
#13733=DIRECTION('ref_axis',(-3.29601953873307E-15,0.,1.));
#13734=DIRECTION('',(0.,-1.,0.));
#13735=DIRECTION('',(-3.29601953873307E-15,0.,1.));
#13736=DIRECTION('',(0.,-1.,0.));
#13737=DIRECTION('',(3.29601953873307E-15,0.,-1.));
#13738=DIRECTION('center_axis',(-1.,0.,-3.29601953873307E-15));
#13739=DIRECTION('ref_axis',(-3.29601953873307E-15,0.,1.));
#13740=DIRECTION('',(0.,-1.,0.));
#13741=DIRECTION('',(-3.29601953873307E-15,0.,1.));
#13742=DIRECTION('',(0.,-1.,0.));
#13743=DIRECTION('',(3.29601953873307E-15,0.,-1.));
#13744=DIRECTION('center_axis',(0.,-1.,0.));
#13745=DIRECTION('ref_axis',(0.,0.,1.));
#13746=DIRECTION('',(-3.46944695195362E-15,0.,-1.));
#13747=DIRECTION('',(0.949699126201879,0.,0.313163806483743));
#13748=DIRECTION('',(-0.313163806483745,0.,0.949699126201879));
#13749=DIRECTION('',(-0.949699126201879,0.,-0.313163806483744));
#13750=DIRECTION('',(-3.46944695195362E-15,0.,-1.));
#13751=DIRECTION('',(1.,0.,0.));
#13752=DIRECTION('',(3.29601953873307E-15,0.,-1.));
#13753=DIRECTION('center_axis',(0.,-1.,0.));
#13754=DIRECTION('ref_axis',(0.,0.,-1.));
#13755=DIRECTION('',(0.707106781186547,0.,0.707106781186548));
#13756=DIRECTION('center_axis',(0.,-1.,0.));
#13757=DIRECTION('ref_axis',(0.,0.,-1.));
#13758=DIRECTION('',(-0.707106781186548,0.,-0.707106781186547));
#13759=DIRECTION('center_axis',(0.,-1.,0.));
#13760=DIRECTION('ref_axis',(0.,0.,-1.));
#13761=DIRECTION('',(1.,0.,-1.95461800110063E-16));
#13762=DIRECTION('center_axis',(0.,1.,0.));
#13763=DIRECTION('ref_axis',(0.,0.,-1.));
#13764=DIRECTION('',(3.29601953873307E-15,0.,-1.));
#13765=DIRECTION('',(1.,0.,0.));
#13766=DIRECTION('',(-3.46944695195362E-15,0.,-1.));
#13767=DIRECTION('',(1.,0.,0.));
#13768=DIRECTION('center_axis',(0.,1.,0.));
#13769=DIRECTION('ref_axis',(0.,0.,-1.));
#13770=DIRECTION('',(-1.,0.,0.));
#13771=DIRECTION('',(-3.29601953873307E-15,0.,1.));
#13772=DIRECTION('center_axis',(0.,-1.,0.));
#13773=DIRECTION('ref_axis',(2.35106052273563E-14,0.,1.));
#13774=DIRECTION('',(-1.,0.,1.95461800110063E-16));
#13775=DIRECTION('center_axis',(0.,1.,0.));
#13776=DIRECTION('ref_axis',(0.,0.,1.));
#13777=DIRECTION('',(0.707106781186548,0.,0.707106781186547));
#13778=DIRECTION('',(-0.707106781186547,0.,-0.707106781186548));
#13779=DIRECTION('center_axis',(0.,1.,0.));
#13780=DIRECTION('ref_axis',(0.,0.,1.));
#13781=DIRECTION('',(-3.29601953873307E-15,0.,1.));
#13782=DIRECTION('',(-1.,0.,0.));
#13783=DIRECTION('',(3.46944695195362E-15,0.,1.));
#13784=DIRECTION('',(-1.,0.,0.));
#13785=DIRECTION('',(3.46944695195362E-15,0.,1.));
#13786=DIRECTION('',(-1.,0.,0.));
#13787=DIRECTION('',(3.46944695195362E-15,0.,1.));
#13788=DIRECTION('center_axis',(1.,0.,0.));
#13789=DIRECTION('ref_axis',(0.,0.,-1.));
#13790=DIRECTION('',(0.,1.,0.));
#13791=DIRECTION('',(0.,0.,1.));
#13792=DIRECTION('',(0.,1.,0.));
#13793=DIRECTION('',(0.,0.,-1.));
#13794=DIRECTION('center_axis',(3.29601953873307E-15,0.,-1.));
#13795=DIRECTION('ref_axis',(-1.,0.,-3.29601953873307E-15));
#13796=DIRECTION('center_axis',(0.,0.,1.));
#13797=DIRECTION('ref_axis',(-1.,0.,0.));
#13798=DIRECTION('center_axis',(0.,0.,1.));
#13799=DIRECTION('ref_axis',(1.,0.,0.));
#13800=DIRECTION('center_axis',(-3.29601953873307E-15,0.,1.));
#13801=DIRECTION('ref_axis',(1.,0.,3.29601953873307E-15));
#13802=DIRECTION('center_axis',(0.,0.,1.));
#13803=DIRECTION('ref_axis',(-1.,0.,0.));
#13804=DIRECTION('center_axis',(0.,0.,1.));
#13805=DIRECTION('ref_axis',(1.,0.,0.));
#13806=DIRECTION('center_axis',(3.29601953873307E-15,0.,-1.));
#13807=DIRECTION('ref_axis',(-1.,0.,-3.29601953873307E-15));
#13808=DIRECTION('',(-3.29601953873307E-15,0.,1.));
#13809=DIRECTION('center_axis',(0.,0.,1.));
#13810=DIRECTION('ref_axis',(-1.,0.,0.));
#13811=DIRECTION('center_axis',(0.,0.,1.));
#13812=DIRECTION('ref_axis',(1.,0.,0.));
#13813=DIRECTION('center_axis',(-3.29601953873307E-15,0.,1.));
#13814=DIRECTION('ref_axis',(1.,0.,3.29601953873307E-15));
#13815=DIRECTION('center_axis',(0.,0.,1.));
#13816=DIRECTION('ref_axis',(-1.,0.,0.));
#13817=DIRECTION('center_axis',(0.,0.,1.));
#13818=DIRECTION('ref_axis',(1.,0.,0.));
#13819=DIRECTION('center_axis',(0.,0.,1.));
#13820=DIRECTION('ref_axis',(1.,0.,0.));
#13821=DIRECTION('center_axis',(0.,0.,1.));
#13822=DIRECTION('ref_axis',(-1.,0.,0.));
#13823=DIRECTION('center_axis',(0.,0.,-1.));
#13824=DIRECTION('ref_axis',(-1.,0.,0.));
#13825=DIRECTION('center_axis',(0.,0.,1.));
#13826=DIRECTION('ref_axis',(-1.,0.,0.));
#13827=DIRECTION('',(0.,0.,-1.));
#13828=DIRECTION('center_axis',(-0.313163806483744,0.,0.949699126201879));
#13829=DIRECTION('ref_axis',(0.949699126201879,0.,0.313163806483744));
#13830=DIRECTION('',(0.949699126201879,0.,0.313163806483744));
#13831=DIRECTION('',(0.,-1.,0.));
#13832=DIRECTION('',(-0.949699126201879,0.,-0.313163806483744));
#13833=DIRECTION('',(0.,1.,0.));
#13834=DIRECTION('center_axis',(-0.949699126201879,0.,-0.313163806483744));
#13835=DIRECTION('ref_axis',(-0.313163806483744,0.,0.949699126201879));
#13836=DIRECTION('center_axis',(0.949699126201879,0.,0.313163806483743));
#13837=DIRECTION('ref_axis',(-0.313163806483743,-5.55111512312581E-15,0.949699126201879));
#13838=DIRECTION('',(0.949699126201879,0.,0.313163806483744));
#13839=DIRECTION('center_axis',(-0.949699126201878,0.,-0.313163806483745));
#13840=DIRECTION('ref_axis',(-0.313163806483745,0.,0.949699126201878));
#13841=DIRECTION('center_axis',(-0.949699126201879,0.,-0.313163806483744));
#13842=DIRECTION('ref_axis',(-0.313163806483744,0.,0.949699126201879));
#13843=DIRECTION('center_axis',(0.949699126201879,0.,0.313163806483743));
#13844=DIRECTION('ref_axis',(-0.313163806483743,0.,0.949699126201879));
#13845=DIRECTION('center_axis',(0.949699126201877,0.,0.313163806483749));
#13846=DIRECTION('ref_axis',(-0.313163806483749,0.,0.949699126201877));
#13847=DIRECTION('',(-0.949699126201879,0.,-0.313163806483744));
#13848=DIRECTION('center_axis',(0.,1.,0.));
#13849=DIRECTION('ref_axis',(0.,0.,1.));
#13850=DIRECTION('',(-0.949699126201879,0.,-0.313163806483743));
#13851=DIRECTION('center_axis',(0.,-1.,0.));
#13852=DIRECTION('ref_axis',(0.,0.,1.));
#13853=DIRECTION('center_axis',(0.,1.,0.));
#13854=DIRECTION('ref_axis',(0.,0.,1.));
#13855=DIRECTION('',(-0.949699126201879,0.,-0.313163806483743));
#13856=DIRECTION('',(-0.313163806483742,0.,0.949699126201879));
#13857=DIRECTION('center_axis',(0.,0.,1.));
#13858=DIRECTION('ref_axis',(1.,0.,0.));
#13859=DIRECTION('center_axis',(3.53117861454706E-12,8.1303226733511E-11,
-1.));
#13860=DIRECTION('ref_axis',(6.36382861148608E-5,0.999999997975084,8.13034512870338E-11));
#13861=DIRECTION('center_axis',(-3.61565657182522E-12,8.32482800044714E-11,
-1.));
#13862=DIRECTION('ref_axis',(-6.36384976265908E-5,0.999999997975071,8.32485099308517E-11));
#13863=DIRECTION('',(1.,0.,0.));
#13864=DIRECTION('center_axis',(-1.,0.,-3.49148133884313E-15));
#13865=DIRECTION('ref_axis',(-3.49148133884313E-15,0.,1.));
#13866=DIRECTION('center_axis',(1.,8.24701670271546E-11,3.58608928678165E-12));
#13867=DIRECTION('ref_axis',(-8.24703950728649E-11,0.999999997975082,6.36383222378267E-5));
#13868=DIRECTION('center_axis',(1.,8.30538663463606E-11,-3.60298487823237E-12));
#13869=DIRECTION('ref_axis',(-8.30540954665947E-11,0.999999997975073,-6.36384608246681E-5));
#13870=DIRECTION('',(-3.49148133884313E-15,0.,1.));
#13871=DIRECTION('center_axis',(1.,0.,0.));
#13872=DIRECTION('ref_axis',(0.,0.,-1.));
#13873=DIRECTION('center_axis',(-1.,-8.28592693501252E-11,3.59876098036562E-12));
#13874=DIRECTION('ref_axis',(-8.28594982030728E-11,0.999999997975053,-6.36387730413301E-5));
#13875=DIRECTION('center_axis',(-1.,0.,0.));
#13876=DIRECTION('ref_axis',(0.,0.999999997975064,6.3638598276304E-5));
#13877=DIRECTION('',(0.,0.,1.));
#13878=DIRECTION('center_axis',(0.,0.,-1.));
#13879=DIRECTION('ref_axis',(-1.,0.,0.));
#13880=DIRECTION('center_axis',(-3.58186538891853E-12,8.2470258696193E-11,
1.));
#13881=DIRECTION('ref_axis',(6.3638285669282E-5,-0.999999997975084,8.24704864729705E-11));
#13882=DIRECTION('center_axis',(3.61565657182547E-12,8.32482800044776E-11,
1.));
#13883=DIRECTION('ref_axis',(-6.36385026828668E-5,-0.99999999797507,8.32485099308762E-11));
#13884=DIRECTION('',(-1.,0.,0.));
#13885=DIRECTION('center_axis',(0.,-1.,0.));
#13886=DIRECTION('ref_axis',(0.,0.,-1.));
#13887=DIRECTION('center_axis',(0.,1.,0.));
#13888=DIRECTION('ref_axis',(3.5527735616222E-15,0.,-1.));
#13889=DIRECTION('center_axis',(0.285050819318021,0.0292578032183599,-0.958065765674237));
#13890=DIRECTION('ref_axis',(0.665144932848858,0.713664621963304,0.219693025978211));
#13891=DIRECTION('center_axis',(0.,1.,0.));
#13892=DIRECTION('ref_axis',(0.,0.,1.));
#13893=DIRECTION('center_axis',(0.,-1.,0.));
#13894=DIRECTION('ref_axis',(0.,0.,-1.));
#13895=DIRECTION('center_axis',(0.289353946523101,0.0248003127138381,-0.956900850726345));
#13896=DIRECTION('ref_axis',(-0.668092365814573,0.72113931848567,-0.183332141410909));
#13897=DIRECTION('center_axis',(0.,-1.,0.));
#13898=DIRECTION('ref_axis',(0.,0.,-1.));
#13899=DIRECTION('',(-0.949699126201879,0.,-0.313163806483743));
#13900=DIRECTION('',(-0.313163806483743,0.,0.949699126201879));
#13901=DIRECTION('center_axis',(0.,-1.,0.));
#13902=DIRECTION('ref_axis',(0.,0.,-1.));
#13903=DIRECTION('center_axis',(0.,1.,0.));
#13904=DIRECTION('ref_axis',(-1.7762059938806E-15,0.,-1.));
#13905=DIRECTION('',(0.313163806483747,0.,-0.949699126201878));
#13906=DIRECTION('center_axis',(0.,1.,0.));
#13907=DIRECTION('ref_axis',(-5.32920569145862E-15,0.,-1.));
#13908=DIRECTION('',(-0.313163806483747,0.,0.949699126201878));
#13909=DIRECTION('center_axis',(0.,-1.,0.));
#13910=DIRECTION('ref_axis',(0.,0.,-1.));
#13911=DIRECTION('center_axis',(0.,1.,0.));
#13912=DIRECTION('ref_axis',(-1.7762059938806E-15,0.,-1.));
#13913=DIRECTION('',(-0.949699126201879,0.,-0.313163806483744));
#13914=DIRECTION('center_axis',(0.,1.,0.));
#13915=DIRECTION('ref_axis',(0.,0.,-1.));
#13916=DIRECTION('',(0.949699126201879,0.,0.313163806483744));
#13917=DIRECTION('center_axis',(0.,-1.,0.));
#13918=DIRECTION('ref_axis',(0.,0.,-1.));
#13919=DIRECTION('center_axis',(0.,1.,0.));
#13920=DIRECTION('ref_axis',(0.,0.,-1.));
#13921=DIRECTION('',(-0.313163806483754,0.,0.949699126201876));
#13922=DIRECTION('center_axis',(0.,1.,0.));
#13923=DIRECTION('ref_axis',(8.88172787481047E-15,0.,-1.));
#13924=DIRECTION('',(0.313163806483754,0.,-0.949699126201876));
#13925=DIRECTION('center_axis',(0.,1.,0.));
#13926=DIRECTION('ref_axis',(-1.7762059938806E-15,0.,-1.));
#13927=DIRECTION('',(0.949699126201879,0.,0.313163806483744));
#13928=DIRECTION('center_axis',(0.,1.,0.));
#13929=DIRECTION('ref_axis',(0.,0.,-1.));
#13930=DIRECTION('',(-0.949699126201879,0.,-0.313163806483744));
#13931=DIRECTION('',(0.313163806483743,0.,-0.949699126201879));
#13932=DIRECTION('',(-0.949699126201879,0.,-0.313163806483743));
#13933=DIRECTION('center_axis',(0.,1.,0.));
#13934=DIRECTION('ref_axis',(0.,0.,1.));
#13935=DIRECTION('center_axis',(0.,1.,0.));
#13936=DIRECTION('ref_axis',(0.,0.,-1.));
#13937=DIRECTION('center_axis',(0.313163806483744,0.,-0.949699126201879));
#13938=DIRECTION('ref_axis',(-0.949699126201879,0.,-0.313163806483744));
#13939=DIRECTION('',(0.,1.,0.));
#13940=DIRECTION('',(-0.949699126201879,0.,-0.313163806483744));
#13941=DIRECTION('',(-0.949699126201879,0.,-0.313163806483744));
#13942=DIRECTION('center_axis',(-0.313163806461999,-2.38433636067788E-11,
0.949699126209049));
#13943=DIRECTION('ref_axis',(-0.658107038058548,0.720972457655595,-0.217011155841942));
#13944=DIRECTION('',(0.949699126201879,0.,0.313163806483744));
#13945=DIRECTION('center_axis',(0.313163806483744,0.,-0.949699126201879));
#13946=DIRECTION('ref_axis',(-0.949699126201879,0.,-0.313163806483744));
#13947=DIRECTION('',(0.,1.,0.));
#13948=DIRECTION('',(0.949699126201879,0.,0.313163806483744));
#13949=DIRECTION('',(0.,-1.,0.));
#13950=DIRECTION('',(-0.949699126201879,0.,-0.313163806483744));
#13951=DIRECTION('center_axis',(0.313163806494915,-1.26989761058302E-11,
-0.949699126198195));
#13952=DIRECTION('ref_axis',(-0.641714392326136,0.737174116651431,-0.211605671995528));
#13953=DIRECTION('',(0.949699126201879,0.,0.313163806483744));
#13954=DIRECTION('center_axis',(0.,-1.,0.));
#13955=DIRECTION('ref_axis',(0.,0.,-1.));
#13956=DIRECTION('center_axis',(0.,1.,0.));
#13957=DIRECTION('ref_axis',(0.,0.,1.));
#13958=DIRECTION('center_axis',(0.,1.,0.));
#13959=DIRECTION('ref_axis',(-2.66445855087016E-15,0.,-1.));
#13960=DIRECTION('center_axis',(-0.298581522051401,-0.0150877415291002,
0.954264866137814));
#13961=DIRECTION('ref_axis',(-0.649648952678908,0.73568412721389,-0.191637948352447));
#13962=DIRECTION('center_axis',(0.,-1.,0.));
#13963=DIRECTION('ref_axis',(0.,0.,-1.));
#13964=DIRECTION('center_axis',(0.,-1.,0.));
#13965=DIRECTION('ref_axis',(0.,0.,-1.));
#13966=DIRECTION('center_axis',(0.,-1.,0.));
#13967=DIRECTION('ref_axis',(0.,0.,-1.));
#13968=DIRECTION('center_axis',(0.,1.,0.));
#13969=DIRECTION('ref_axis',(0.,0.,-1.));
#13970=DIRECTION('center_axis',(0.,1.,0.));
#13971=DIRECTION('ref_axis',(-8.88249771892961E-16,0.,-1.));
#13972=DIRECTION('center_axis',(0.,1.,0.));
#13973=DIRECTION('ref_axis',(0.,0.,1.));
#13974=DIRECTION('',(0.,1.,0.));
#13975=DIRECTION('center_axis',(0.,-1.,0.));
#13976=DIRECTION('ref_axis',(0.,0.,1.));
#13977=DIRECTION('',(0.,-1.,0.));
#13978=DIRECTION('center_axis',(0.,1.,0.));
#13979=DIRECTION('ref_axis',(0.,0.,1.));
#13980=DIRECTION('center_axis',(0.,1.,0.));
#13981=DIRECTION('ref_axis',(1.65389215948552E-15,0.,-1.));
#13982=DIRECTION('center_axis',(0.,-1.,0.));
#13983=DIRECTION('ref_axis',(1.77645503129512E-15,0.,1.));
#13984=DIRECTION('center_axis',(0.,1.,0.));
#13985=DIRECTION('ref_axis',(0.,0.,1.));
#13986=DIRECTION('center_axis',(0.,1.,0.));
#13987=DIRECTION('ref_axis',(0.,0.,1.));
#13988=DIRECTION('',(0.500130397801055,-0.706999113223839,0.500021838619139));
#13989=DIRECTION('center_axis',(0.,1.,0.));
#13990=DIRECTION('ref_axis',(0.,0.,1.));
#13991=DIRECTION('',(-0.500130397801063,0.706999113223845,0.500021838619122));
#13992=DIRECTION('center_axis',(0.,-1.,0.));
#13993=DIRECTION('ref_axis',(0.,0.,1.));
#13994=DIRECTION('center_axis',(0.,-1.,0.));
#13995=DIRECTION('ref_axis',(0.,0.,1.));
#13996=DIRECTION('center_axis',(0.,1.,0.));
#13997=DIRECTION('ref_axis',(4.56335677841536E-15,0.,-1.));
#13998=DIRECTION('',(-0.500021838619135,-0.706999113223842,0.500130397801054));
#13999=DIRECTION('center_axis',(0.,1.,0.));
#14000=DIRECTION('ref_axis',(0.,0.,1.));
#14001=DIRECTION('',(-0.500021838619135,0.706999113223842,-0.500130397801054));
#14002=DIRECTION('center_axis',(0.,-1.,0.));
#14003=DIRECTION('ref_axis',(0.,0.,1.));
#14004=DIRECTION('center_axis',(0.,-1.,0.));
#14005=DIRECTION('ref_axis',(0.,0.,1.));
#14006=DIRECTION('center_axis',(0.,-1.,0.));
#14007=DIRECTION('ref_axis',(0.,0.,-1.));
#14008=DIRECTION('',(-1.,0.,1.95461800110063E-16));
#14009=DIRECTION('center_axis',(0.,1.,0.));
#14010=DIRECTION('ref_axis',(0.,0.,-1.));
#14011=DIRECTION('',(0.,0.,1.));
#14012=DIRECTION('center_axis',(0.,-1.,0.));
#14013=DIRECTION('ref_axis',(0.,0.,-1.));
#14014=DIRECTION('',(-0.707106781186547,0.,-0.707106781186548));
#14015=DIRECTION('',(0.707106781186548,0.,0.707106781186547));
#14016=DIRECTION('center_axis',(0.,-1.,0.));
#14017=DIRECTION('ref_axis',(0.,0.,-1.));
#14018=DIRECTION('center_axis',(0.,1.,0.));
#14019=DIRECTION('ref_axis',(0.,0.,1.));
#14020=DIRECTION('',(0.,0.,-1.));
#14021=DIRECTION('center_axis',(0.,-1.,0.));
#14022=DIRECTION('ref_axis',(0.,0.,1.));
#14023=DIRECTION('',(1.,0.,-1.95461800110063E-16));
#14024=DIRECTION('center_axis',(0.,1.,0.));
#14025=DIRECTION('ref_axis',(0.,0.,1.));
#14026=DIRECTION('',(-0.707106781186548,0.,-0.707106781186547));
#14027=DIRECTION('center_axis',(0.,1.,0.));
#14028=DIRECTION('ref_axis',(0.,0.,1.));
#14029=DIRECTION('',(0.707106781186547,0.,0.707106781186548));
#14030=DIRECTION('center_axis',(0.,1.,0.));
#14031=DIRECTION('ref_axis',(0.,0.,1.));
#14032=DIRECTION('center_axis',(1.95461800110063E-16,0.,1.));
#14033=DIRECTION('ref_axis',(1.,0.,-1.95461800110063E-16));
#14034=DIRECTION('',(1.,0.,-1.95461800110063E-16));
#14035=DIRECTION('',(0.,-1.,0.));
#14036=DIRECTION('',(-1.,0.,1.95461800110063E-16));
#14037=DIRECTION('',(0.,-1.,0.));
#14038=DIRECTION('',(1.,0.,-1.95461800110063E-16));
#14039=DIRECTION('center_axis',(1.,0.,0.));
#14040=DIRECTION('ref_axis',(0.,0.,-1.));
#14041=DIRECTION('',(0.,-1.,0.));
#14042=DIRECTION('',(0.,0.,-1.));
#14043=DIRECTION('',(0.,0.,-1.));
#14044=DIRECTION('',(0.,-1.,0.));
#14045=DIRECTION('',(0.,0.,1.));
#14046=DIRECTION('center_axis',(0.,-1.,0.));
#14047=DIRECTION('ref_axis',(0.,0.,-1.));
#14048=DIRECTION('center_axis',(0.,-1.,0.));
#14049=DIRECTION('ref_axis',(0.,0.,-1.));
#14050=DIRECTION('center_axis',(0.,1.,0.));
#14051=DIRECTION('ref_axis',(0.,0.,1.));
#14052=DIRECTION('center_axis',(1.95461800110063E-16,0.,1.));
#14053=DIRECTION('ref_axis',(1.,0.,-1.95461800110063E-16));
#14054=DIRECTION('',(0.,-1.,0.));
#14055=DIRECTION('',(-1.,0.,1.95461800110063E-16));
#14056=DIRECTION('',(-1.,0.,1.95461800110063E-16));
#14057=DIRECTION('',(0.,-1.,0.));
#14058=DIRECTION('',(1.,0.,-1.95461800110063E-16));
#14059=DIRECTION('center_axis',(1.,0.,0.));
#14060=DIRECTION('ref_axis',(0.,0.,-1.));
#14061=DIRECTION('',(0.,0.,1.));
#14062=DIRECTION('',(0.,-1.,0.));
#14063=DIRECTION('',(0.,0.,-1.));
#14064=DIRECTION('',(0.,-1.,0.));
#14065=DIRECTION('',(0.,0.,1.));
#14066=DIRECTION('center_axis',(0.,1.,0.));
#14067=DIRECTION('ref_axis',(0.,0.,1.));
#14068=DIRECTION('',(-3.29601953873307E-15,0.,1.));
#14069=DIRECTION('',(1.,0.,0.));
#14070=DIRECTION('',(0.,0.,1.));
#14071=DIRECTION('',(0.949699126201879,0.,0.313163806483743));
#14072=DIRECTION('',(0.313163806483743,0.,-0.949699126201879));
#14073=DIRECTION('',(0.949699126201879,0.,0.313163806483744));
#14074=DIRECTION('center_axis',(0.,1.,0.));
#14075=DIRECTION('ref_axis',(0.,0.,1.));
#14076=DIRECTION('',(3.49148133884313E-15,0.,-1.));
#14077=DIRECTION('center_axis',(0.,1.,0.));
#14078=DIRECTION('ref_axis',(0.,0.,1.));
#14079=DIRECTION('',(-0.313163806483747,0.,0.949699126201878));
#14080=DIRECTION('center_axis',(0.,-1.,0.));
#14081=DIRECTION('ref_axis',(-1.7762059938806E-15,0.,1.));
#14082=DIRECTION('center_axis',(0.,1.,0.));
#14083=DIRECTION('ref_axis',(0.,0.,1.));
#14084=DIRECTION('',(-0.313163806483743,0.,0.949699126201879));
#14085=DIRECTION('',(0.949699126201879,0.,0.313163806483743));
#14086=DIRECTION('',(-3.46944695195362E-15,0.,-1.));
#14087=DIRECTION('',(1.,0.,0.));
#14088=DIRECTION('',(-3.46944695195362E-15,0.,-1.));
#14089=DIRECTION('',(1.,0.,0.));
#14090=DIRECTION('center_axis',(0.,-1.,0.));
#14091=DIRECTION('ref_axis',(2.35106052273563E-14,0.,1.));
#14092=DIRECTION('',(-1.,0.,1.95461800110063E-16));
#14093=DIRECTION('center_axis',(0.,-1.,0.));
#14094=DIRECTION('ref_axis',(-1.30614473485313E-15,0.,1.));
#14095=DIRECTION('',(0.,0.,-1.));
#14096=DIRECTION('center_axis',(0.,-1.,0.));
#14097=DIRECTION('ref_axis',(0.,0.,1.));
#14098=DIRECTION('',(1.,0.,-1.95461800110063E-16));
#14099=DIRECTION('center_axis',(0.,-1.,0.));
#14100=DIRECTION('ref_axis',(0.,0.,1.));
#14101=DIRECTION('center_axis',(0.,1.,0.));
#14102=DIRECTION('ref_axis',(0.,0.,1.));
#14103=DIRECTION('',(-0.949699126201879,0.,-0.313163806483744));
#14104=DIRECTION('center_axis',(0.,-1.,0.));
#14105=DIRECTION('ref_axis',(0.,0.,1.));
#14106=DIRECTION('center_axis',(0.,1.,0.));
#14107=DIRECTION('ref_axis',(0.,0.,1.));
#14108=DIRECTION('',(-0.313163806483754,0.,0.949699126201876));
#14109=DIRECTION('center_axis',(0.,1.,0.));
#14110=DIRECTION('ref_axis',(0.,0.,1.));
#14111=DIRECTION('',(1.,0.,0.));
#14112=DIRECTION('center_axis',(0.,1.,0.));
#14113=DIRECTION('ref_axis',(0.,0.,1.));
#14114=DIRECTION('',(0.949699126201879,0.,0.313163806483744));
#14115=DIRECTION('center_axis',(0.,-1.,0.));
#14116=DIRECTION('ref_axis',(0.,0.,1.));
#14117=DIRECTION('',(0.313163806483747,0.,-0.949699126201878));
#14118=DIRECTION('center_axis',(0.,1.,0.));
#14119=DIRECTION('ref_axis',(0.,0.,1.));
#14120=DIRECTION('',(-1.,0.,0.));
#14121=DIRECTION('center_axis',(0.,-1.,0.));
#14122=DIRECTION('ref_axis',(0.,0.,1.));
#14123=DIRECTION('center_axis',(0.,1.,0.));
#14124=DIRECTION('ref_axis',(0.,0.,1.));
#14125=DIRECTION('',(-0.949699126201879,0.,-0.313163806483744));
#14126=DIRECTION('center_axis',(0.,1.,0.));
#14127=DIRECTION('ref_axis',(0.,0.,1.));
#14128=DIRECTION('',(0.,0.,1.));
#14129=DIRECTION('center_axis',(0.,1.,0.));
#14130=DIRECTION('ref_axis',(0.,0.,1.));
#14131=DIRECTION('',(0.313163806483754,0.,-0.949699126201876));
#14132=DIRECTION('center_axis',(0.,-1.,0.));
#14133=DIRECTION('ref_axis',(0.,0.,-1.));
#14134=DIRECTION('center_axis',(0.,1.,0.));
#14135=DIRECTION('ref_axis',(0.,0.,1.));
#14136=DIRECTION('center_axis',(0.,-1.,0.));
#14137=DIRECTION('ref_axis',(0.,0.,1.));
#14138=DIRECTION('center_axis',(0.,1.,0.));
#14139=DIRECTION('ref_axis',(0.,0.,1.));
#14140=DIRECTION('center_axis',(0.,-1.,0.));
#14141=DIRECTION('ref_axis',(0.,0.,-1.));
#14142=DIRECTION('center_axis',(0.,1.,0.));
#14143=DIRECTION('ref_axis',(0.,0.,-1.));
#14144=DIRECTION('center_axis',(0.,0.,1.));
#14145=DIRECTION('ref_axis',(1.,0.,0.));
#14146=DIRECTION('center_axis',(0.,0.,-1.));
#14147=DIRECTION('ref_axis',(-6.36384622448961E-5,0.999999997975073,0.));
#14148=DIRECTION('',(-1.,0.,0.));
#14149=DIRECTION('center_axis',(-3.53117861453752E-12,-8.13032267332511E-11,
-1.));
#14150=DIRECTION('ref_axis',(6.36387635293006E-5,0.999999997975054,-8.13034512884572E-11));
#14151=DIRECTION('center_axis',(1.,0.,0.));
#14152=DIRECTION('ref_axis',(0.,0.,-1.));
#14153=DIRECTION('center_axis',(-1.,8.324828000444E-11,3.61565657182464E-12));
#14154=DIRECTION('ref_axis',(8.32485099311225E-11,0.999999997975066,6.36385813081935E-5));
#14155=DIRECTION('',(0.,0.,-1.));
#14156=DIRECTION('center_axis',(-1.,8.28592693503832E-11,-3.59876098037523E-12));
#14157=DIRECTION('ref_axis',(8.28594982014715E-11,0.999999997975086,-6.36382556169485E-5));
#14158=DIRECTION('center_axis',(-0.707106781186547,0.,0.707106781186548));
#14159=DIRECTION('ref_axis',(0.707106781186548,0.,0.707106781186547));
#14160=DIRECTION('',(-0.707106781186548,0.,-0.707106781186547));
#14161=DIRECTION('',(0.707106781186548,0.,0.707106781186547));
#14162=DIRECTION('',(0.500076792314969,-0.706998163771264,0.500076792314972));
#14163=DIRECTION('center_axis',(0.707106781186548,0.,-0.707106781186547));
#14164=DIRECTION('ref_axis',(-0.707106781186547,0.,-0.707106781186548));
#14165=DIRECTION('',(0.707106781186547,0.,0.707106781186548));
#14166=DIRECTION('',(0.,1.,0.));
#14167=DIRECTION('',(-0.500076792314964,0.706998163771268,-0.500076792314971));
#14168=DIRECTION('',(-0.707106781186547,0.,-0.707106781186548));
#14169=DIRECTION('center_axis',(0.,-1.,0.));
#14170=DIRECTION('ref_axis',(0.,0.,-1.));
#14171=DIRECTION('',(0.,-1.,0.));
#14172=DIRECTION('center_axis',(0.,1.,0.));
#14173=DIRECTION('ref_axis',(0.,0.,1.));
#14174=DIRECTION('',(0.,-1.,0.));
#14175=DIRECTION('center_axis',(0.,-1.,0.));
#14176=DIRECTION('ref_axis',(0.,0.,-1.));
#14177=DIRECTION('center_axis',(0.,-1.,0.));
#14178=DIRECTION('ref_axis',(0.,0.,-1.));
#14179=DIRECTION('',(-0.949699126201879,0.,-0.313163806483744));
#14180=DIRECTION('center_axis',(0.,-1.,0.));
#14181=DIRECTION('ref_axis',(0.,0.,-1.));
#14182=DIRECTION('',(0.949699126201879,0.,0.313163806483744));
#14183=DIRECTION('center_axis',(0.,1.,0.));
#14184=DIRECTION('ref_axis',(0.,0.,-1.));
#14185=DIRECTION('center_axis',(0.313163806483744,0.,-0.949699126201879));
#14186=DIRECTION('ref_axis',(-0.949699126201879,0.,-0.313163806483744));
#14187=DIRECTION('',(-0.949699126201879,0.,-0.313163806483744));
#14188=DIRECTION('',(0.,-1.,0.));
#14189=DIRECTION('center_axis',(0.,-1.,0.));
#14190=DIRECTION('ref_axis',(0.,0.,-1.));
#14191=DIRECTION('',(-0.949699126201879,0.,-0.313163806483744));
#14192=DIRECTION('center_axis',(0.,-1.,0.));
#14193=DIRECTION('ref_axis',(0.,0.,-1.));
#14194=DIRECTION('',(0.949699126201879,0.,0.313163806483744));
#14195=DIRECTION('center_axis',(0.,1.,0.));
#14196=DIRECTION('ref_axis',(0.,0.,-1.));
#14197=DIRECTION('center_axis',(0.313163806483744,0.,-0.949699126201879));
#14198=DIRECTION('ref_axis',(-0.949699126201879,0.,-0.313163806483744));
#14199=DIRECTION('',(0.,1.,0.));
#14200=DIRECTION('',(0.949699126201879,0.,0.313163806483744));
#14201=DIRECTION('center_axis',(0.,1.,0.));
#14202=DIRECTION('ref_axis',(0.,0.,1.));
#14203=DIRECTION('center_axis',(0.,-1.,0.));
#14204=DIRECTION('ref_axis',(0.,0.,1.));
#14205=DIRECTION('',(0.,-1.,0.));
#14206=DIRECTION('center_axis',(0.,1.,0.));
#14207=DIRECTION('ref_axis',(0.,0.,1.));
#14208=DIRECTION('center_axis',(-1.,0.,0.));
#14209=DIRECTION('ref_axis',(0.,0.,1.));
#14210=DIRECTION('',(0.,1.,0.));
#14211=DIRECTION('',(0.,0.,1.));
#14212=DIRECTION('',(0.,0.,-1.));
#14213=DIRECTION('center_axis',(1.03892784411108E-15,0.,-1.));
#14214=DIRECTION('ref_axis',(-1.,0.,-1.03892784411108E-15));
#14215=DIRECTION('',(0.,1.,0.));
#14216=DIRECTION('',(-1.,0.,-1.03892784411108E-15));
#14217=DIRECTION('',(0.,-1.,0.));
#14218=DIRECTION('',(1.,0.,1.03892784411108E-15));
#14219=DIRECTION('center_axis',(0.,1.,0.));
#14220=DIRECTION('ref_axis',(0.,0.,1.));
#14221=DIRECTION('center_axis',(0.,1.,0.));
#14222=DIRECTION('ref_axis',(0.,0.,1.));
#14223=DIRECTION('',(0.,0.,1.));
#14224=DIRECTION('center_axis',(0.,-1.,0.));
#14225=DIRECTION('ref_axis',(0.,0.,1.));
#14226=DIRECTION('center_axis',(0.,1.,0.));
#14227=DIRECTION('ref_axis',(0.,0.,1.));
#14228=DIRECTION('',(-1.,0.,-1.03892784411108E-15));
#14229=DIRECTION('center_axis',(0.,1.,0.));
#14230=DIRECTION('ref_axis',(0.,0.,1.));
#14231=DIRECTION('center_axis',(0.,1.,0.));
#14232=DIRECTION('ref_axis',(0.,0.,1.));
#14233=DIRECTION('center_axis',(0.,-1.,0.));
#14234=DIRECTION('ref_axis',(-3.70074341541718E-15,0.,1.));
#14235=DIRECTION('center_axis',(0.,1.,0.));
#14236=DIRECTION('ref_axis',(0.,0.,1.));
#14237=DIRECTION('center_axis',(0.,1.,0.));
#14238=DIRECTION('ref_axis',(-0.453742606486518,0.,-0.891132788679005));
#14239=DIRECTION('center_axis',(0.,-1.,0.));
#14240=DIRECTION('ref_axis',(0.,0.,1.));
#14241=DIRECTION('center_axis',(0.,1.,0.));
#14242=DIRECTION('ref_axis',(0.,0.,1.));
#14243=DIRECTION('center_axis',(0.,1.,0.));
#14244=DIRECTION('ref_axis',(0.,0.,1.));
#14245=DIRECTION('center_axis',(0.,-1.,0.));
#14246=DIRECTION('ref_axis',(7.40148683083437E-15,0.,1.));
#14247=DIRECTION('center_axis',(0.,1.,0.));
#14248=DIRECTION('ref_axis',(0.,0.,1.));
#14249=DIRECTION('center_axis',(0.,-1.,0.));
#14250=DIRECTION('ref_axis',(1.,0.,3.49155068656687E-15));
#14251=DIRECTION('center_axis',(0.,1.,0.));
#14252=DIRECTION('ref_axis',(-2.22044698990993E-14,0.,-1.));
#14253=DIRECTION('center_axis',(0.958065765674362,0.0292578032189066,0.285050819317542));
#14254=DIRECTION('ref_axis',(0.219693026012008,-0.713664621834887,-0.665144932975479));
#14255=DIRECTION('center_axis',(0.,1.,0.));
#14256=DIRECTION('ref_axis',(0.,0.,1.));
#14257=DIRECTION('center_axis',(0.,-1.,0.));
#14258=DIRECTION('ref_axis',(0.,0.,-1.));
#14259=DIRECTION('center_axis',(0.956900850725464,0.0248003127102221,0.289353946526324));
#14260=DIRECTION('ref_axis',(0.183332141415881,0.721139318485221,-0.668092365813694));
#14261=DIRECTION('center_axis',(0.949699126201878,0.,0.313163806483747));
#14262=DIRECTION('ref_axis',(0.313163806483747,0.,-0.949699126201878));
#14263=DIRECTION('',(0.,1.,0.));
#14264=DIRECTION('',(0.313163806483747,0.,-0.949699126201878));
#14265=DIRECTION('',(0.,-1.,0.));
#14266=DIRECTION('',(0.313163806483747,0.,-0.949699126201878));
#14267=DIRECTION('center_axis',(-0.949699126194824,2.35739471213281E-11,
-0.313163806505138));
#14268=DIRECTION('ref_axis',(0.21701115590481,0.72097245765419,-0.658107038039357));
#14269=DIRECTION('',(-0.313163806483747,0.,0.949699126201878));
#14270=DIRECTION('center_axis',(0.949699126201878,0.,0.313163806483747));
#14271=DIRECTION('ref_axis',(0.313163806483747,0.,-0.949699126201878));
#14272=DIRECTION('',(-0.313163806483747,0.,0.949699126201878));
#14273=DIRECTION('',(0.,-1.,0.));
#14274=DIRECTION('',(0.313163806483747,0.,-0.949699126201878));
#14275=DIRECTION('center_axis',(0.949699126207133,1.83236368242976E-11,
0.31316380646781));
#14276=DIRECTION('ref_axis',(0.211605671956001,0.737174116650109,-0.64171439234069));
#14277=DIRECTION('',(-0.313163806483747,0.,0.949699126201878));
#14278=DIRECTION('center_axis',(0.,-1.,0.));
#14279=DIRECTION('ref_axis',(1.,0.,3.49155068656687E-15));
#14280=DIRECTION('center_axis',(0.,1.,0.));
#14281=DIRECTION('ref_axis',(0.,0.,1.));
#14282=DIRECTION('center_axis',(0.,1.,0.));
#14283=DIRECTION('ref_axis',(-1.95400113482291E-14,0.,-1.));
#14284=DIRECTION('center_axis',(-0.954264865962622,-0.0150877408549486,
-0.29858152264538));
#14285=DIRECTION('ref_axis',(0.191637949226221,0.735684127227363,-0.649648952405898));
#14286=DIRECTION('center_axis',(0.,-1.,0.));
#14287=DIRECTION('ref_axis',(0.,0.,-1.));
#14288=DIRECTION('center_axis',(0.,1.,0.));
#14289=DIRECTION('ref_axis',(1.,0.,1.59271860898362E-15));
#14290=DIRECTION('',(0.,1.,0.));
#14291=DIRECTION('center_axis',(0.,-1.,0.));
#14292=DIRECTION('ref_axis',(0.,0.,1.));
#14293=DIRECTION('',(0.,-1.,0.));
#14294=DIRECTION('center_axis',(0.,1.,0.));
#14295=DIRECTION('ref_axis',(0.,0.,1.));
#14296=DIRECTION('center_axis',(0.,1.,0.));
#14297=DIRECTION('ref_axis',(1.,0.,5.39036164761359E-15));
#14298=DIRECTION('',(-0.500130397801065,-0.706999113223837,-0.500021838619131));
#14299=DIRECTION('center_axis',(0.,1.,0.));
#14300=DIRECTION('ref_axis',(0.,0.,1.));
#14301=DIRECTION('',(0.500130397801061,0.706999113223842,-0.500021838619127));
#14302=DIRECTION('center_axis',(0.,-1.,0.));
#14303=DIRECTION('ref_axis',(3.55276338872479E-15,0.,1.));
#14304=DIRECTION('center_axis',(0.,-1.,0.));
#14305=DIRECTION('ref_axis',(-1.7763816943624E-15,0.,1.));
#14306=DIRECTION('center_axis',(0.,-1.,0.));
#14307=DIRECTION('ref_axis',(1.,0.,3.49148133884313E-15));
#14308=DIRECTION('',(3.29601953873307E-15,0.,-1.));
#14309=DIRECTION('center_axis',(0.,1.,0.));
#14310=DIRECTION('ref_axis',(1.56737368182375E-14,0.,-1.));
#14311=DIRECTION('',(-1.,0.,1.95461800110063E-16));
#14312=DIRECTION('center_axis',(0.,-1.,0.));
#14313=DIRECTION('ref_axis',(0.,0.,-1.));
#14314=DIRECTION('',(0.707106781186551,0.,-0.707106781186544));
#14315=DIRECTION('',(-0.707106781186549,0.,0.707106781186546));
#14316=DIRECTION('center_axis',(0.,-1.,0.));
#14317=DIRECTION('ref_axis',(0.,0.,-1.));
#14318=DIRECTION('center_axis',(0.,1.,0.));
#14319=DIRECTION('ref_axis',(-1.,0.,-3.49148133884313E-15));
#14320=DIRECTION('',(1.,0.,-1.95461800110063E-16));
#14321=DIRECTION('center_axis',(0.,-1.,0.));
#14322=DIRECTION('ref_axis',(0.,0.,1.));
#14323=DIRECTION('',(-3.29601953873307E-15,0.,1.));
#14324=DIRECTION('center_axis',(0.,1.,0.));
#14325=DIRECTION('ref_axis',(0.,0.,1.));
#14326=DIRECTION('',(0.707106781186549,0.,-0.707106781186546));
#14327=DIRECTION('center_axis',(0.,1.,0.));
#14328=DIRECTION('ref_axis',(0.,0.,1.));
#14329=DIRECTION('',(-0.707106781186551,0.,0.707106781186544));
#14330=DIRECTION('center_axis',(0.,1.,0.));
#14331=DIRECTION('ref_axis',(0.,0.,1.));
#14332=DIRECTION('center_axis',(-1.,0.,-3.29601953873307E-15));
#14333=DIRECTION('ref_axis',(-3.29601953873307E-15,0.,1.));
#14334=DIRECTION('',(-3.29601953873307E-15,0.,1.));
#14335=DIRECTION('',(0.,-1.,0.));
#14336=DIRECTION('',(3.29601953873307E-15,0.,-1.));
#14337=DIRECTION('',(0.,-1.,0.));
#14338=DIRECTION('',(-3.29601953873307E-15,0.,1.));
#14339=DIRECTION('center_axis',(0.,-1.,0.));
#14340=DIRECTION('ref_axis',(1.,0.,3.70074341541719E-15));
#14341=DIRECTION('center_axis',(0.,-1.,0.));
#14342=DIRECTION('ref_axis',(0.,0.,-1.));
#14343=DIRECTION('center_axis',(0.,1.,0.));
#14344=DIRECTION('ref_axis',(0.,0.,1.));
#14345=DIRECTION('center_axis',(-1.,0.,-3.29601953873307E-15));
#14346=DIRECTION('ref_axis',(-3.29601953873307E-15,0.,1.));
#14347=DIRECTION('',(-3.29601953873307E-15,0.,1.));
#14348=DIRECTION('',(0.,-1.,0.));
#14349=DIRECTION('',(3.29601953873307E-15,0.,-1.));
#14350=DIRECTION('',(3.29601953873307E-15,0.,-1.));
#14351=DIRECTION('',(0.,-1.,0.));
#14352=DIRECTION('center_axis',(0.,-1.,0.));
#14353=DIRECTION('ref_axis',(1.,0.,3.70074341541719E-15));
#14354=DIRECTION('center_axis',(0.,1.,0.));
#14355=DIRECTION('ref_axis',(0.,0.,1.));
#14356=DIRECTION('center_axis',(0.,-1.,0.));
#14357=DIRECTION('ref_axis',(0.,0.,1.));
#14358=DIRECTION('center_axis',(0.,1.,0.));
#14359=DIRECTION('ref_axis',(-1.,0.,-3.49151141721823E-15));
#14360=DIRECTION('center_axis',(0.,-1.,0.));
#14361=DIRECTION('ref_axis',(0.,0.,-1.));
#14362=DIRECTION('center_axis',(0.,1.,0.));
#14363=DIRECTION('ref_axis',(1.77631540548237E-15,0.,-1.));
#14364=DIRECTION('center_axis',(-1.,0.,-3.49148133884313E-15));
#14365=DIRECTION('ref_axis',(-3.49148133884313E-15,0.,1.));
#14366=DIRECTION('center_axis',(1.,-1.94413658113135E-13,1.26716935928603E-14));
#14367=DIRECTION('ref_axis',(1.94414464126846E-13,0.999999997975072,-6.36384851394666E-5));
#14368=DIRECTION('',(3.49148133884313E-15,0.,-1.));
#14369=DIRECTION('center_axis',(1.,-8.26648556920426E-11,-3.58608928677283E-12));
#14370=DIRECTION('ref_axis',(8.26650837388721E-11,0.999999997975055,6.36387448952208E-5));
#14371=DIRECTION('center_axis',(-0.707106781186546,0.,-0.707106781186549));
#14372=DIRECTION('ref_axis',(-0.707106781186549,0.,0.707106781186546));
#14373=DIRECTION('',(0.707106781186549,0.,-0.707106781186546));
#14374=DIRECTION('',(-0.707106781186549,0.,0.707106781186546));
#14375=DIRECTION('',(-0.50007679231497,-0.706998163771266,0.50007679231497));
#14376=DIRECTION('',(0.,-1.,0.));
#14377=DIRECTION('center_axis',(0.707106781186544,0.,0.707106781186551));
#14378=DIRECTION('ref_axis',(0.707106781186551,0.,-0.707106781186544));
#14379=DIRECTION('',(-0.707106781186551,0.,0.707106781186544));
#14380=DIRECTION('',(0.50007679231497,0.70699816377127,-0.500076792314963));
#14381=DIRECTION('',(0.707106781186551,0.,-0.707106781186544));
#14382=DIRECTION('center_axis',(0.,-1.,0.));
#14383=DIRECTION('ref_axis',(1.,0.,3.49175053950189E-15));
#14384=DIRECTION('',(0.,-1.,0.));
#14385=DIRECTION('center_axis',(0.,1.,0.));
#14386=DIRECTION('ref_axis',(0.,0.,1.));
#14387=DIRECTION('center_axis',(0.,-1.,0.));
#14388=DIRECTION('ref_axis',(0.,0.,-1.));
#14389=DIRECTION('center_axis',(0.,-1.,0.));
#14390=DIRECTION('ref_axis',(1.,0.,3.49148133884313E-15));
#14391=DIRECTION('',(0.313163806483747,0.,-0.949699126201878));
#14392=DIRECTION('center_axis',(0.,-1.,0.));
#14393=DIRECTION('ref_axis',(0.,0.,-1.));
#14394=DIRECTION('',(-0.313163806483747,0.,0.949699126201878));
#14395=DIRECTION('center_axis',(0.,1.,0.));
#14396=DIRECTION('ref_axis',(6.75015932572764E-14,0.,-1.));
#14397=DIRECTION('center_axis',(0.949699126201878,0.,0.313163806483747));
#14398=DIRECTION('ref_axis',(0.313163806483747,0.,-0.949699126201878));
#14399=DIRECTION('',(0.313163806483747,0.,-0.949699126201878));
#14400=DIRECTION('',(0.,-1.,0.));
#14401=DIRECTION('center_axis',(0.,-1.,0.));
#14402=DIRECTION('ref_axis',(1.,0.,3.49148133884313E-15));
#14403=DIRECTION('',(0.313163806483747,0.,-0.949699126201878));
#14404=DIRECTION('center_axis',(0.,-1.,0.));
#14405=DIRECTION('ref_axis',(0.,0.,-1.));
#14406=DIRECTION('',(-0.313163806483747,0.,0.949699126201878));
#14407=DIRECTION('center_axis',(0.,1.,0.));
#14408=DIRECTION('ref_axis',(3.73035047474275E-14,0.,-1.));
#14409=DIRECTION('center_axis',(0.949699126201878,0.,0.313163806483747));
#14410=DIRECTION('ref_axis',(0.313163806483747,0.,-0.949699126201878));
#14411=DIRECTION('',(0.,1.,0.));
#14412=DIRECTION('',(-0.313163806483747,0.,0.949699126201878));
#14413=DIRECTION('center_axis',(0.,1.,0.));
#14414=DIRECTION('ref_axis',(-1.,0.,-3.49137740498798E-15));
#14415=DIRECTION('center_axis',(0.,-1.,0.));
#14416=DIRECTION('ref_axis',(-3.55273339156727E-15,0.,1.));
#14417=DIRECTION('',(0.,-1.,0.));
#14418=DIRECTION('center_axis',(0.,1.,0.));
#14419=DIRECTION('ref_axis',(0.,0.,1.));
#14420=DIRECTION('center_axis',(3.49148133884313E-15,0.,-1.));
#14421=DIRECTION('ref_axis',(-1.,0.,-3.49148133884313E-15));
#14422=DIRECTION('',(0.,1.,0.));
#14423=DIRECTION('',(-1.,0.,-3.49148133884313E-15));
#14424=DIRECTION('',(1.,0.,3.49148133884313E-15));
#14425=DIRECTION('center_axis',(1.,0.,4.53040918295421E-15));
#14426=DIRECTION('ref_axis',(4.53040918295421E-15,0.,-1.));
#14427=DIRECTION('',(0.,1.,0.));
#14428=DIRECTION('',(4.53040918295421E-15,0.,-1.));
#14429=DIRECTION('',(0.,-1.,0.));
#14430=DIRECTION('',(-4.53040918295421E-15,0.,1.));
#14431=DIRECTION('center_axis',(0.,1.,0.));
#14432=DIRECTION('ref_axis',(-1.,0.,-3.49148133884313E-15));
#14433=DIRECTION('center_axis',(0.,1.,0.));
#14434=DIRECTION('ref_axis',(0.,0.,1.));
#14435=DIRECTION('',(-1.,0.,-3.49148133884313E-15));
#14436=DIRECTION('center_axis',(0.,1.,0.));
#14437=DIRECTION('ref_axis',(0.,0.,1.));
#14438=DIRECTION('center_axis',(0.,-1.,0.));
#14439=DIRECTION('ref_axis',(-3.55275288159092E-15,0.,1.));
#14440=DIRECTION('',(4.53040918295421E-15,0.,-1.));
#14441=DIRECTION('center_axis',(0.,1.,0.));
#14442=DIRECTION('ref_axis',(0.,0.,1.));
#14443=DIRECTION('center_axis',(0.,1.,0.));
#14444=DIRECTION('ref_axis',(-1.,0.,-3.70074341541718E-15));
#14445=DIRECTION('center_axis',(0.,1.,0.));
#14446=DIRECTION('ref_axis',(0.891132788679008,0.,-0.453742606486513));
#14447=DIRECTION('center_axis',(0.,-1.,0.));
#14448=DIRECTION('ref_axis',(0.,0.,1.));
#14449=DIRECTION('center_axis',(0.,1.,0.));
#14450=DIRECTION('ref_axis',(0.,0.,1.));
#14451=DIRECTION('center_axis',(0.,1.,0.));
#14452=DIRECTION('ref_axis',(-1.,0.,0.));
#14453=DIRECTION('center_axis',(0.,-1.,0.));
#14454=DIRECTION('ref_axis',(0.,0.,1.));
#14455=DIRECTION('center_axis',(0.,1.,0.));
#14456=DIRECTION('ref_axis',(0.,0.,1.));
#14457=DIRECTION('center_axis',(0.,-1.,0.));
#14458=DIRECTION('ref_axis',(0.,0.,1.));
#14459=DIRECTION('center_axis',(0.,1.,0.));
#14460=DIRECTION('ref_axis',(0.,0.,-1.));
#14461=DIRECTION('center_axis',(-0.285050819317539,0.0292578032188915,0.958065765674363));
#14462=DIRECTION('ref_axis',(0.665144932827453,-0.713664621985,0.219693025972537));
#14463=DIRECTION('center_axis',(0.,1.,0.));
#14464=DIRECTION('ref_axis',(0.,0.,1.));
#14465=DIRECTION('center_axis',(0.,-1.,0.));
#14466=DIRECTION('ref_axis',(0.,0.,-1.));
#14467=DIRECTION('center_axis',(-0.289353946523101,0.0248003127138381,0.956900850726345));
#14468=DIRECTION('ref_axis',(0.668092365814573,0.72113931848567,0.183332141410909));
#14469=DIRECTION('center_axis',(-0.313163806483744,0.,0.949699126201879));
#14470=DIRECTION('ref_axis',(0.949699126201879,0.,0.313163806483744));
#14471=DIRECTION('',(-0.949699126201879,0.,-0.313163806483744));
#14472=DIRECTION('',(0.,1.,0.));
#14473=DIRECTION('',(0.949699126201879,0.,0.313163806483744));
#14474=DIRECTION('',(0.,-1.,0.));
#14475=DIRECTION('',(0.949699126201879,0.,0.313163806483744));
#14476=DIRECTION('center_axis',(0.313163806486104,2.55945706169953E-12,
-0.949699126201101));
#14477=DIRECTION('ref_axis',(0.658107038053724,0.720972457648934,0.217011155878702));
#14478=DIRECTION('center_axis',(-0.313163806483744,0.,0.949699126201879));
#14479=DIRECTION('ref_axis',(0.949699126201879,0.,0.313163806483744));
#14480=DIRECTION('',(0.,1.,0.));
#14481=DIRECTION('',(-0.949699126201879,0.,-0.313163806483744));
#14482=DIRECTION('',(0.,-1.,0.));
#14483=DIRECTION('',(0.949699126201879,0.,0.313163806483744));
#14484=DIRECTION('center_axis',(-0.313163806482752,1.15972384695759E-12,
0.949699126202206));
#14485=DIRECTION('ref_axis',(0.641714392333106,0.737174116650406,0.211605671977966));
#14486=DIRECTION('',(-0.949699126201879,0.,-0.313163806483744));
#14487=DIRECTION('center_axis',(0.,-1.,0.));
#14488=DIRECTION('ref_axis',(0.,0.,1.));
#14489=DIRECTION('center_axis',(0.,1.,0.));
#14490=DIRECTION('ref_axis',(0.,0.,1.));
#14491=DIRECTION('center_axis',(0.,1.,0.));
#14492=DIRECTION('ref_axis',(0.,0.,-1.));
#14493=DIRECTION('center_axis',(0.298581521665074,-0.0150877419673539,-0.954264866251763));
#14494=DIRECTION('ref_axis',(0.649648952857147,0.735684127204403,0.191637947784642));
#14495=DIRECTION('center_axis',(0.,-1.,0.));
#14496=DIRECTION('ref_axis',(0.,0.,-1.));
#14497=DIRECTION('center_axis',(0.,1.,0.));
#14498=DIRECTION('ref_axis',(-5.20660583828602E-15,0.,1.));
#14499=DIRECTION('',(0.,1.,0.));
#14500=DIRECTION('',(0.,-1.,0.));
#14501=DIRECTION('center_axis',(0.,1.,0.));
#14502=DIRECTION('ref_axis',(-1.12246949261663E-14,0.,1.));
#14503=DIRECTION('',(0.500021838619129,-0.706999113223846,-0.500130397801055));
#14504=DIRECTION('',(0.500021838619127,0.706999113223842,0.500130397801061));
#14505=DIRECTION('center_axis',(0.,-1.,0.));
#14506=DIRECTION('ref_axis',(3.55276338872479E-15,0.,1.));
#14507=DIRECTION('center_axis',(0.,-1.,0.));
#14508=DIRECTION('ref_axis',(0.,0.,1.));
#14509=DIRECTION('center_axis',(-1.95461800110063E-16,0.,-1.));
#14510=DIRECTION('ref_axis',(-1.,0.,1.95461800110063E-16));
#14511=DIRECTION('',(-1.,0.,1.95461800110063E-16));
#14512=DIRECTION('',(0.,-1.,0.));
#14513=DIRECTION('',(1.,0.,-1.95461800110063E-16));
#14514=DIRECTION('',(0.,-1.,0.));
#14515=DIRECTION('',(-1.,0.,1.95461800110063E-16));
#14516=DIRECTION('center_axis',(0.,-1.,0.));
#14517=DIRECTION('ref_axis',(0.,0.,1.));
#14518=DIRECTION('center_axis',(0.,-1.,0.));
#14519=DIRECTION('ref_axis',(0.,0.,-1.));
#14520=DIRECTION('center_axis',(0.,1.,0.));
#14521=DIRECTION('ref_axis',(0.,0.,1.));
#14522=DIRECTION('center_axis',(-1.95461800110063E-16,0.,-1.));
#14523=DIRECTION('ref_axis',(-1.,0.,1.95461800110063E-16));
#14524=DIRECTION('',(0.,-1.,0.));
#14525=DIRECTION('',(1.,0.,-1.95461800110063E-16));
#14526=DIRECTION('',(1.,0.,-1.95461800110063E-16));
#14527=DIRECTION('',(0.,-1.,0.));
#14528=DIRECTION('',(-1.,0.,1.95461800110063E-16));
#14529=DIRECTION('center_axis',(0.,-1.,0.));
#14530=DIRECTION('ref_axis',(0.,0.,1.));
#14531=DIRECTION('center_axis',(0.,1.,0.));
#14532=DIRECTION('ref_axis',(0.,0.,1.));
#14533=DIRECTION('center_axis',(0.,-1.,0.));
#14534=DIRECTION('ref_axis',(2.34380416309755E-14,0.,1.));
#14535=DIRECTION('center_axis',(0.,1.,0.));
#14536=DIRECTION('ref_axis',(0.,0.,-1.));
#14537=DIRECTION('center_axis',(0.,-1.,0.));
#14538=DIRECTION('ref_axis',(0.,0.,-1.));
#14539=DIRECTION('center_axis',(0.,1.,0.));
#14540=DIRECTION('ref_axis',(-1.77631540548237E-15,0.,-1.));
#14541=DIRECTION('center_axis',(0.,0.,-1.));
#14542=DIRECTION('ref_axis',(-1.,0.,0.));
#14543=DIRECTION('center_axis',(-3.61565657183125E-12,-8.32482800045515E-11,
1.));
#14544=DIRECTION('ref_axis',(-6.3638448448845E-5,-0.999999997975074,-8.32485099307542E-11));
#14545=DIRECTION('',(1.,0.,0.));
#14546=DIRECTION('center_axis',(3.58186538890928E-12,-8.24702586959293E-11,
1.));
#14547=DIRECTION('ref_axis',(6.36387679980598E-5,-0.999999997975054,-8.2470486474432E-11));
#14548=DIRECTION('center_axis',(0.707106781186547,0.,-0.707106781186548));
#14549=DIRECTION('ref_axis',(-0.707106781186548,0.,-0.707106781186547));
#14550=DIRECTION('',(0.707106781186548,0.,0.707106781186547));
#14551=DIRECTION('',(-0.707106781186548,0.,-0.707106781186547));
#14552=DIRECTION('',(-0.500076792314973,-0.706998163771266,-0.500076792314966));
#14553=DIRECTION('',(0.,-1.,0.));
#14554=DIRECTION('center_axis',(-0.707106781186548,0.,0.707106781186547));
#14555=DIRECTION('ref_axis',(0.707106781186547,0.,0.707106781186548));
#14556=DIRECTION('',(-0.707106781186547,0.,-0.707106781186548));
#14557=DIRECTION('',(0.,1.,0.));
#14558=DIRECTION('',(0.500076792314966,0.706998163771266,0.500076792314973));
#14559=DIRECTION('',(0.707106781186547,0.,0.707106781186548));
#14560=DIRECTION('center_axis',(0.,-1.,0.));
#14561=DIRECTION('ref_axis',(0.,0.,1.));
#14562=DIRECTION('',(0.,-1.,0.));
#14563=DIRECTION('center_axis',(0.,1.,0.));
#14564=DIRECTION('ref_axis',(0.,0.,1.));
#14565=DIRECTION('center_axis',(0.,-1.,0.));
#14566=DIRECTION('ref_axis',(0.,0.,-1.));
#14567=DIRECTION('center_axis',(0.,-1.,0.));
#14568=DIRECTION('ref_axis',(0.,0.,1.));
#14569=DIRECTION('',(0.949699126201879,0.,0.313163806483744));
#14570=DIRECTION('center_axis',(0.,-1.,0.));
#14571=DIRECTION('ref_axis',(0.,0.,-1.));
#14572=DIRECTION('',(-0.949699126201879,0.,-0.313163806483744));
#14573=DIRECTION('center_axis',(0.,1.,0.));
#14574=DIRECTION('ref_axis',(0.,0.,-1.));
#14575=DIRECTION('center_axis',(-0.313163806483744,0.,0.949699126201879));
#14576=DIRECTION('ref_axis',(0.949699126201879,0.,0.313163806483744));
#14577=DIRECTION('',(0.949699126201879,0.,0.313163806483744));
#14578=DIRECTION('',(0.,-1.,0.));
#14579=DIRECTION('center_axis',(0.,-1.,0.));
#14580=DIRECTION('ref_axis',(0.,0.,1.));
#14581=DIRECTION('',(0.949699126201879,0.,0.313163806483744));
#14582=DIRECTION('center_axis',(0.,-1.,0.));
#14583=DIRECTION('ref_axis',(0.,0.,-1.));
#14584=DIRECTION('',(-0.949699126201879,0.,-0.313163806483744));
#14585=DIRECTION('center_axis',(0.,1.,0.));
#14586=DIRECTION('ref_axis',(-5.50671843416529E-14,0.,-1.));
#14587=DIRECTION('center_axis',(-0.313163806483744,0.,0.949699126201879));
#14588=DIRECTION('ref_axis',(0.949699126201879,0.,0.313163806483744));
#14589=DIRECTION('',(-0.949699126201879,0.,-0.313163806483744));
#14590=DIRECTION('center_axis',(0.,1.,0.));
#14591=DIRECTION('ref_axis',(0.,0.,-1.));
#14592=DIRECTION('center_axis',(0.,-1.,0.));
#14593=DIRECTION('ref_axis',(1.77636669578364E-15,0.,1.));
#14594=DIRECTION('',(0.,-1.,0.));
#14595=DIRECTION('center_axis',(0.,1.,0.));
#14596=DIRECTION('ref_axis',(0.,0.,1.));
#14597=DIRECTION('center_axis',(1.,0.,0.));
#14598=DIRECTION('ref_axis',(0.,0.,-1.));
#14599=DIRECTION('',(0.,0.,1.));
#14600=DIRECTION('',(0.,1.,0.));
#14601=DIRECTION('',(0.,0.,-1.));
#14602=DIRECTION('center_axis',(-1.03892784411108E-15,0.,1.));
#14603=DIRECTION('ref_axis',(1.,0.,1.03892784411108E-15));
#14604=DIRECTION('',(0.,1.,0.));
#14605=DIRECTION('',(1.,0.,1.03892784411108E-15));
#14606=DIRECTION('',(0.,-1.,0.));
#14607=DIRECTION('',(-1.,0.,-1.03892784411108E-15));
#14608=DIRECTION('center_axis',(0.,1.,0.));
#14609=DIRECTION('ref_axis',(0.,0.,-1.));
#14610=DIRECTION('',(-1.,0.,0.));
#14611=DIRECTION('',(0.,0.,-1.));
#14612=DIRECTION('center_axis',(0.,1.,0.));
#14613=DIRECTION('ref_axis',(0.,0.,1.));
#14614=DIRECTION('center_axis',(0.,-1.,0.));
#14615=DIRECTION('ref_axis',(3.55275288159092E-15,0.,1.));
#14616=DIRECTION('center_axis',(0.,1.,0.));
#14617=DIRECTION('ref_axis',(0.,0.,1.));
#14618=DIRECTION('',(1.,0.,1.03892784411108E-15));
#14619=DIRECTION('center_axis',(0.,1.,0.));
#14620=DIRECTION('ref_axis',(0.,0.,1.));
#14621=DIRECTION('center_axis',(0.,-1.,0.));
#14622=DIRECTION('ref_axis',(1.48029736616688E-15,0.,1.));
#14623=DIRECTION('',(-1.,0.,0.));
#14624=DIRECTION('',(3.46944695195362E-15,0.,1.));
#14625=DIRECTION('center_axis',(0.,1.,0.));
#14626=DIRECTION('ref_axis',(0.,0.,-1.));
#14627=DIRECTION('center_axis',(0.,-1.,0.));
#14628=DIRECTION('ref_axis',(0.,0.,1.));
#14629=DIRECTION('center_axis',(0.,1.,0.));
#14630=DIRECTION('ref_axis',(0.,0.,1.));
#14631=DIRECTION('center_axis',(0.,1.,0.));
#14632=DIRECTION('ref_axis',(0.453742606486519,0.,0.891132788679005));
#14633=DIRECTION('center_axis',(0.,1.,0.));
#14634=DIRECTION('ref_axis',(0.,0.,-1.));
#14635=DIRECTION('center_axis',(0.,-1.,0.));
#14636=DIRECTION('ref_axis',(-7.40148683083437E-15,0.,1.));
#14637=DIRECTION('center_axis',(0.,1.,0.));
#14638=DIRECTION('ref_axis',(0.,0.,1.));
#14639=DIRECTION('center_axis',(0.,-1.,0.));
#14640=DIRECTION('ref_axis',(-1.,0.,-1.04743722655916E-14));
#14641=DIRECTION('center_axis',(0.,1.,0.));
#14642=DIRECTION('ref_axis',(3.90797794557653E-14,0.,-1.));
#14643=DIRECTION('center_axis',(-0.958065765673929,0.0292578032171867,-0.285050819319174));
#14644=DIRECTION('ref_axis',(0.219693026019329,0.713664621806868,-0.665144933003125));
#14645=DIRECTION('center_axis',(0.,1.,0.));
#14646=DIRECTION('ref_axis',(0.,0.,1.));
#14647=DIRECTION('center_axis',(0.,-1.,0.));
#14648=DIRECTION('ref_axis',(0.,0.,-1.));
#14649=DIRECTION('center_axis',(-0.956900850717379,0.024800312678508,-0.289353946555781));
#14650=DIRECTION('ref_axis',(-0.183332141458518,0.721139318485025,0.668092365802205));
#14651=DIRECTION('center_axis',(-0.949699126201876,0.,-0.313163806483754));
#14652=DIRECTION('ref_axis',(-0.313163806483754,0.,0.949699126201876));
#14653=DIRECTION('',(-0.313163806483754,0.,0.949699126201876));
#14654=DIRECTION('',(0.,-1.,0.));
#14655=DIRECTION('',(-0.313163806483754,0.,0.949699126201876));
#14656=DIRECTION('center_axis',(0.949699126200346,5.25362244862842E-12,
0.313163806488392));
#14657=DIRECTION('ref_axis',(-0.217011155881437,0.720972457651555,0.65810703804995));
#14658=DIRECTION('',(0.313163806483754,0.,-0.949699126201876));
#14659=DIRECTION('center_axis',(-0.949699126201876,0.,-0.313163806483754));
#14660=DIRECTION('ref_axis',(-0.313163806483754,0.,0.949699126201876));
#14661=DIRECTION('',(0.,1.,0.));
#14662=DIRECTION('',(0.313163806483754,0.,-0.949699126201876));
#14663=DIRECTION('',(-0.313163806483754,0.,0.949699126201876));
#14664=DIRECTION('center_axis',(-0.949699126201081,-2.78333723603669E-12,
-0.313163806486162));
#14665=DIRECTION('ref_axis',(-0.211605671983048,0.737174116650356,0.641714392331488));
#14666=DIRECTION('',(0.313163806483754,0.,-0.949699126201876));
#14667=DIRECTION('center_axis',(0.,-1.,0.));
#14668=DIRECTION('ref_axis',(-1.,0.,-1.04743722655916E-14));
#14669=DIRECTION('center_axis',(0.,1.,0.));
#14670=DIRECTION('ref_axis',(0.,0.,1.));
#14671=DIRECTION('center_axis',(0.,1.,0.));
#14672=DIRECTION('ref_axis',(0.,0.,-1.));
#14673=DIRECTION('center_axis',(0.954264863821462,-0.0150877326158706,0.298581529904847));
#14674=DIRECTION('ref_axis',(-0.191637959901166,0.735684127399272,0.649648949062253));
#14675=DIRECTION('center_axis',(0.,-1.,0.));
#14676=DIRECTION('ref_axis',(0.,0.,-1.));
#14677=DIRECTION('center_axis',(0.,-1.,0.));
#14678=DIRECTION('ref_axis',(-1.,0.,-1.04744440165294E-14));
#14679=DIRECTION('',(0.,0.,1.));
#14680=DIRECTION('center_axis',(0.,1.,0.));
#14681=DIRECTION('ref_axis',(0.,0.,-1.));
#14682=DIRECTION('',(1.,0.,-1.95461800110063E-16));
#14683=DIRECTION('center_axis',(0.,-1.,0.));
#14684=DIRECTION('ref_axis',(0.,0.,-1.));
#14685=DIRECTION('',(-0.707106781186556,0.,0.707106781186539));
#14686=DIRECTION('center_axis',(0.,-1.,0.));
#14687=DIRECTION('ref_axis',(0.,0.,-1.));
#14688=DIRECTION('',(0.707106781186554,0.,-0.707106781186541));
#14689=DIRECTION('center_axis',(0.,-1.,0.));
#14690=DIRECTION('ref_axis',(0.,0.,-1.));
#14691=DIRECTION('center_axis',(0.,1.,0.));
#14692=DIRECTION('ref_axis',(1.,0.,1.04744440165294E-14));
#14693=DIRECTION('',(-1.,0.,1.95461800110063E-16));
#14694=DIRECTION('center_axis',(0.,-1.,0.));
#14695=DIRECTION('ref_axis',(-1.30614473485313E-15,0.,1.));
#14696=DIRECTION('',(0.,0.,-1.));
#14697=DIRECTION('center_axis',(0.,1.,0.));
#14698=DIRECTION('ref_axis',(0.,0.,1.));
#14699=DIRECTION('',(-0.707106781186554,0.,0.707106781186541));
#14700=DIRECTION('',(0.707106781186556,0.,-0.707106781186539));
#14701=DIRECTION('center_axis',(0.,1.,0.));
#14702=DIRECTION('ref_axis',(0.,0.,1.));
#14703=DIRECTION('center_axis',(0.,-1.,0.));
#14704=DIRECTION('ref_axis',(-1.,0.,-9.86864910777917E-15));
#14705=DIRECTION('center_axis',(0.,-1.,0.));
#14706=DIRECTION('ref_axis',(0.,0.,-1.));
#14707=DIRECTION('center_axis',(0.,1.,0.));
#14708=DIRECTION('ref_axis',(0.,0.,1.));
#14709=DIRECTION('center_axis',(0.,-1.,0.));
#14710=DIRECTION('ref_axis',(-1.,0.,-9.86864910777917E-15));
#14711=DIRECTION('center_axis',(0.,1.,0.));
#14712=DIRECTION('ref_axis',(0.,0.,1.));
#14713=DIRECTION('center_axis',(0.,-1.,0.));
#14714=DIRECTION('ref_axis',(-1.2335811384724E-15,0.,1.));
#14715=DIRECTION('center_axis',(0.,1.,0.));
#14716=DIRECTION('ref_axis',(1.,0.,1.04745342516547E-14));
#14717=DIRECTION('center_axis',(0.,-1.,0.));
#14718=DIRECTION('ref_axis',(0.,0.,-1.));
#14719=DIRECTION('center_axis',(0.,1.,0.));
#14720=DIRECTION('ref_axis',(-1.77631540548237E-15,0.,-1.));
#14721=DIRECTION('center_axis',(0.707106781186541,0.,0.707106781186554));
#14722=DIRECTION('ref_axis',(0.707106781186554,0.,-0.707106781186541));
#14723=DIRECTION('',(-0.707106781186554,0.,0.707106781186541));
#14724=DIRECTION('',(0.707106781186554,0.,-0.707106781186541));
#14725=DIRECTION('',(0.500076792314976,-0.706998163771267,-0.500076792314961));
#14726=DIRECTION('',(0.,-1.,0.));
#14727=DIRECTION('center_axis',(-0.707106781186539,0.,-0.707106781186556));
#14728=DIRECTION('ref_axis',(-0.707106781186556,0.,0.707106781186539));
#14729=DIRECTION('',(0.707106781186556,0.,-0.707106781186539));
#14730=DIRECTION('',(0.,1.,0.));
#14731=DIRECTION('',(-0.500076792314971,0.706998163771271,0.50007679231496));
#14732=DIRECTION('',(-0.707106781186556,0.,0.707106781186539));
#14733=DIRECTION('center_axis',(0.,-1.,0.));
#14734=DIRECTION('ref_axis',(-1.,0.,-1.04746320744071E-14));
#14735=DIRECTION('center_axis',(0.,1.,0.));
#14736=DIRECTION('ref_axis',(0.,0.,1.));
#14737=DIRECTION('center_axis',(0.,-1.,0.));
#14738=DIRECTION('ref_axis',(0.,0.,-1.));
#14739=DIRECTION('center_axis',(0.,-1.,0.));
#14740=DIRECTION('ref_axis',(-1.,0.,-1.04744440165294E-14));
#14741=DIRECTION('',(-0.313163806483754,0.,0.949699126201876));
#14742=DIRECTION('center_axis',(0.,-1.,0.));
#14743=DIRECTION('ref_axis',(0.,0.,-1.));
#14744=DIRECTION('',(0.313163806483754,0.,-0.949699126201876));
#14745=DIRECTION('center_axis',(0.,1.,0.));
#14746=DIRECTION('ref_axis',(-2.84216649503149E-14,0.,-1.));
#14747=DIRECTION('center_axis',(-0.949699126201876,0.,-0.313163806483754));
#14748=DIRECTION('ref_axis',(-0.313163806483754,0.,0.949699126201876));
#14749=DIRECTION('',(-0.313163806483754,0.,0.949699126201876));
#14750=DIRECTION('center_axis',(0.,-1.,0.));
#14751=DIRECTION('ref_axis',(-1.,0.,-1.04744440165294E-14));
#14752=DIRECTION('',(-0.313163806483753,0.,0.949699126201876));
#14753=DIRECTION('center_axis',(0.,-1.,0.));
#14754=DIRECTION('ref_axis',(0.,0.,-1.));
#14755=DIRECTION('',(0.313163806483754,0.,-0.949699126201876));
#14756=DIRECTION('center_axis',(0.,1.,0.));
#14757=DIRECTION('ref_axis',(0.,0.,-1.));
#14758=DIRECTION('center_axis',(-0.949699126201876,0.,-0.313163806483753));
#14759=DIRECTION('ref_axis',(-0.313163806483754,0.,0.949699126201876));
#14760=DIRECTION('',(0.,1.,0.));
#14761=DIRECTION('',(0.313163806483753,0.,-0.949699126201876));
#14762=DIRECTION('center_axis',(0.,1.,0.));
#14763=DIRECTION('ref_axis',(1.,0.,1.04743786245486E-14));
#14764=DIRECTION('center_axis',(0.,-1.,0.));
#14765=DIRECTION('ref_axis',(0.,0.,1.));
#14766=DIRECTION('',(0.,-1.,0.));
#14767=DIRECTION('center_axis',(0.,1.,0.));
#14768=DIRECTION('ref_axis',(0.,0.,1.));
#14769=DIRECTION('center_axis',(-1.04744440165294E-14,0.,1.));
#14770=DIRECTION('ref_axis',(1.,0.,1.04744440165294E-14));
#14771=DIRECTION('',(0.,1.,0.));
#14772=DIRECTION('',(1.,0.,1.04744440165294E-14));
#14773=DIRECTION('',(-1.,0.,-1.04744440165294E-14));
#14774=DIRECTION('center_axis',(-1.,0.,-1.15133718606405E-14));
#14775=DIRECTION('ref_axis',(-1.15133718606405E-14,0.,1.));
#14776=DIRECTION('',(0.,1.,0.));
#14777=DIRECTION('',(-1.15133718606405E-14,0.,1.));
#14778=DIRECTION('',(0.,-1.,0.));
#14779=DIRECTION('',(1.15133718606405E-14,0.,-1.));
#14780=DIRECTION('center_axis',(0.,1.,0.));
#14781=DIRECTION('ref_axis',(1.,0.,1.04744440165294E-14));
#14782=DIRECTION('center_axis',(0.,-1.,0.));
#14783=DIRECTION('ref_axis',(0.,0.,1.));
#14784=DIRECTION('center_axis',(0.,1.,0.));
#14785=DIRECTION('ref_axis',(0.,0.,1.));
#14786=DIRECTION('',(1.,0.,1.04744440165294E-14));
#14787=DIRECTION('center_axis',(0.,1.,0.));
#14788=DIRECTION('ref_axis',(0.,0.,1.));
#14789=DIRECTION('center_axis',(0.,-1.,0.));
#14790=DIRECTION('ref_axis',(0.,0.,1.));
#14791=DIRECTION('center_axis',(0.,1.,0.));
#14792=DIRECTION('ref_axis',(0.,0.,1.));
#14793=DIRECTION('',(-1.15133718606405E-14,0.,1.));
#14794=DIRECTION('center_axis',(0.,1.,0.));
#14795=DIRECTION('ref_axis',(1.,0.,1.11022302462516E-14));
#14796=DIRECTION('center_axis',(0.,-1.,0.));
#14797=DIRECTION('ref_axis',(0.,0.,1.));
#14798=DIRECTION('center_axis',(0.,1.,0.));
#14799=DIRECTION('ref_axis',(0.,0.,1.));
#14800=DIRECTION('center_axis',(0.,1.,0.));
#14801=DIRECTION('ref_axis',(-0.891132788679008,0.,0.453742606486513));
#14802=DIRECTION('center_axis',(0.,-1.,0.));
#14803=DIRECTION('ref_axis',(-7.40148683083437E-15,0.,1.));
#14804=DIRECTION('center_axis',(0.,1.,0.));
#14805=DIRECTION('ref_axis',(0.,0.,1.));
#14806=DIRECTION('center_axis',(0.,1.,0.));
#14807=DIRECTION('ref_axis',(1.,0.,7.40148683083437E-15));
#14808=DIRECTION('center_axis',(0.,1.,0.));
#14809=DIRECTION('ref_axis',(0.707106781186556,0.,-0.707106781186539));
#14810=DIRECTION('center_axis',(-0.588235294117663,0.,0.808689828521608));
#14811=DIRECTION('ref_axis',(0.808689828521608,0.,0.588235294117663));
#14812=DIRECTION('center_axis',(0.,1.,0.));
#14813=DIRECTION('ref_axis',(0.,0.,1.));
#14814=DIRECTION('center_axis',(1.,0.,0.));
#14815=DIRECTION('ref_axis',(0.,0.,-1.));
#14816=DIRECTION('center_axis',(-1.,0.,-1.04744440165294E-14));
#14817=DIRECTION('ref_axis',(-1.04744440165294E-14,0.,1.));
#14818=DIRECTION('center_axis',(1.,0.,1.38777878078144E-14));
#14819=DIRECTION('ref_axis',(1.38777878078144E-14,0.,-1.));
#14820=DIRECTION('center_axis',(1.15133718606405E-14,0.,-1.));
#14821=DIRECTION('ref_axis',(-1.,0.,-1.15133718606405E-14));
#14822=DIRECTION('center_axis',(1.38777878078144E-14,0.,-1.));
#14823=DIRECTION('ref_axis',(-1.,0.,-1.38777878078144E-14));
#14824=DIRECTION('center_axis',(0.,1.,0.));
#14825=DIRECTION('ref_axis',(0.,0.,1.));
#14826=DIRECTION('center_axis',(-0.84916201117318,1.46586199943604E-14,
-0.528132444354937));
#14827=DIRECTION('ref_axis',(-0.528132444354937,1.80922966162518E-29,0.84916201117318));
#14828=DIRECTION('center_axis',(0.,1.,0.));
#14829=DIRECTION('ref_axis',(-0.274625188963796,0.,-0.961551353587836));
#14830=DIRECTION('center_axis',(0.528132444354927,0.,0.849162011173186));
#14831=DIRECTION('ref_axis',(0.849162011173186,0.,-0.528132444354927));
#14832=DIRECTION('center_axis',(0.,1.,0.));
#14833=DIRECTION('ref_axis',(0.,0.,1.));
#14834=DIRECTION('center_axis',(0.,1.,0.));
#14835=DIRECTION('ref_axis',(0.707106781186556,0.,-0.707106781186539));
#14836=DIRECTION('center_axis',(0.588235294117663,0.,-0.808689828521608));
#14837=DIRECTION('ref_axis',(-0.808689828521608,0.,-0.588235294117663));
#14838=DIRECTION('center_axis',(0.,1.,0.));
#14839=DIRECTION('ref_axis',(0.,0.,1.));
#14840=DIRECTION('center_axis',(-1.,0.,0.));
#14841=DIRECTION('ref_axis',(0.,0.,1.));
#14842=DIRECTION('center_axis',(1.,0.,1.04744440165294E-14));
#14843=DIRECTION('ref_axis',(1.04744440165294E-14,0.,-1.));
#14844=DIRECTION('center_axis',(-1.,0.,-1.38777878078144E-14));
#14845=DIRECTION('ref_axis',(-1.38777878078144E-14,0.,1.));
#14846=DIRECTION('center_axis',(-1.15133718606405E-14,0.,1.));
#14847=DIRECTION('ref_axis',(1.,0.,1.15133718606405E-14));
#14848=DIRECTION('center_axis',(-1.38777878078144E-14,-3.85185988877446E-28,
1.));
#14849=DIRECTION('ref_axis',(1.,-1.06910588403687E-42,1.38777878078144E-14));
#14850=DIRECTION('center_axis',(0.,1.,0.));
#14851=DIRECTION('ref_axis',(0.,0.,1.));
#14852=DIRECTION('center_axis',(0.84916201117318,0.,0.528132444354937));
#14853=DIRECTION('ref_axis',(0.528132444354937,0.,-0.84916201117318));
#14854=DIRECTION('center_axis',(0.,1.,0.));
#14855=DIRECTION('ref_axis',(-0.274625188963804,0.,-0.961551353587834));
#14856=DIRECTION('center_axis',(-0.528132444354927,0.,-0.849162011173186));
#14857=DIRECTION('ref_axis',(-0.849162011173186,0.,0.528132444354927));
#14858=DIRECTION('center_axis',(0.,1.,0.));
#14859=DIRECTION('ref_axis',(0.,0.,1.));
#14860=DIRECTION('center_axis',(0.0822611166554848,-0.0232075739979077,
0.996340562857763));
#14861=DIRECTION('ref_axis',(0.996607302542249,-0.000737174163025255,-0.0823003104108089));
#14862=DIRECTION('center_axis',(-0.996340562857417,-0.0232075739986902,
0.0822611166594516));
#14863=DIRECTION('ref_axis',(0.0823003104147849,-0.000737174163321746,0.99660730254192));
#14864=DIRECTION('center_axis',(-0.224812648466097,0.696171426497067,0.681765808777984));
#14865=DIRECTION('ref_axis',(3.9236749875465E-16,-0.69967611234192,0.714460172310604));
#14866=DIRECTION('center_axis',(-0.839824053586503,0.,-0.542858691574091));
#14867=DIRECTION('ref_axis',(0.542858691574091,2.77555756156287E-14,-0.839824053586503));
#14868=DIRECTION('center_axis',(-0.825680763412087,3.74339213057468E-15,
-0.564137640058907));
#14869=DIRECTION('ref_axis',(0.564137640058907,-1.66533453693773E-14,-0.825680763412087));
#14870=DIRECTION('center_axis',(0.,-1.,0.));
#14871=DIRECTION('ref_axis',(0.,0.,1.));
#14872=DIRECTION('center_axis',(0.,-1.,0.));
#14873=DIRECTION('ref_axis',(0.,0.,-1.));
#14874=DIRECTION('center_axis',(-0.823608768724453,0.,-0.567158351856156));
#14875=DIRECTION('ref_axis',(-0.567158351856156,0.,0.823608768724453));
#14876=DIRECTION('center_axis',(0.313163806483747,0.,-0.949699126201878));
#14877=DIRECTION('ref_axis',(-0.949699126201878,0.,-0.313163806483747));
#14878=DIRECTION('center_axis',(-0.313163806483745,3.07054667648618E-14,
0.949699126201878));
#14879=DIRECTION('ref_axis',(0.949699126201878,1.07892897725893E-28,0.313163806483745));
#14880=DIRECTION('center_axis',(0.,-1.,0.));
#14881=DIRECTION('ref_axis',(0.,0.,-1.));
#14882=DIRECTION('center_axis',(0.,-1.,0.));
#14883=DIRECTION('ref_axis',(0.,0.,-1.));
#14884=DIRECTION('center_axis',(0.,1.,0.));
#14885=DIRECTION('ref_axis',(0.,0.,1.));
#14886=DIRECTION('center_axis',(1.,0.,0.));
#14887=DIRECTION('ref_axis',(0.,0.,-1.));
#14888=DIRECTION('center_axis',(-1.,0.,0.));
#14889=DIRECTION('ref_axis',(0.,0.,1.));
#14890=DIRECTION('center_axis',(1.,0.,0.));
#14891=DIRECTION('ref_axis',(0.,0.,-1.));
#14892=DIRECTION('center_axis',(0.846153846153842,0.,0.532938710021199));
#14893=DIRECTION('ref_axis',(-0.532938710021199,0.,0.846153846153842));
#14894=DIRECTION('center_axis',(0.,1.,0.));
#14895=DIRECTION('ref_axis',(1.,0.,0.));
#14896=DIRECTION('center_axis',(0.313163806483745,6.14109335297236E-14,
-0.949699126201878));
#14897=DIRECTION('ref_axis',(0.949699126201878,3.88578058618798E-14,0.313163806483745));
#14898=DIRECTION('center_axis',(-0.225935650513581,0.692454480471778,0.68517141964735));
#14899=DIRECTION('ref_axis',(2.12986048996937E-14,0.703358708234097,-0.710835091671241));
#14900=DIRECTION('center_axis',(0.72431261840463,0.,0.689471704147334));
#14901=DIRECTION('ref_axis',(-0.689471704147334,-9.99200722162653E-14,0.72431261840463));
#14902=DIRECTION('center_axis',(0.233246104178629,-0.667281700967051,-0.707341067972171));
#14903=DIRECTION('ref_axis',(-1.1771509218523E-15,-0.727404531188479,0.68620889531284));
#14904=DIRECTION('center_axis',(0.,1.,0.));
#14905=DIRECTION('ref_axis',(-0.948898229383528,0.,0.315582240109938));
#14906=DIRECTION('center_axis',(0.819571610992504,0.,0.572976766069229));
#14907=DIRECTION('ref_axis',(-0.572976766069229,0.,0.819571610992504));
#14908=DIRECTION('center_axis',(-0.846153846153842,0.,0.532938710021199));
#14909=DIRECTION('ref_axis',(-0.532938710021199,0.,-0.846153846153842));
#14910=DIRECTION('center_axis',(0.,1.,0.));
#14911=DIRECTION('ref_axis',(0.,0.,1.));
#14912=DIRECTION('center_axis',(0.827607008689209,0.,0.561307971766392));
#14913=DIRECTION('ref_axis',(0.561307971766392,0.,-0.827607008689208));
#14914=DIRECTION('center_axis',(-0.313163806483747,0.,0.949699126201878));
#14915=DIRECTION('ref_axis',(0.949699126201878,0.,0.313163806483747));
#14916=DIRECTION('center_axis',(0.313163806483745,0.,-0.949699126201878));
#14917=DIRECTION('ref_axis',(-0.949699126201878,0.,-0.313163806483745));
#14918=DIRECTION('center_axis',(0.,-1.,0.));
#14919=DIRECTION('ref_axis',(0.,0.,-1.));
#14920=DIRECTION('center_axis',(0.,-1.,0.));
#14921=DIRECTION('ref_axis',(0.210852528929983,0.,0.977517882723294));
#14922=DIRECTION('center_axis',(0.,-1.,0.));
#14923=DIRECTION('ref_axis',(0.,0.,-1.));
#14924=DIRECTION('center_axis',(0.,1.,0.));
#14925=DIRECTION('ref_axis',(0.,0.,1.));
#14926=DIRECTION('center_axis',(-0.313163806483747,0.,0.949699126201878));
#14927=DIRECTION('ref_axis',(0.949699126201878,0.,0.313163806483747));
#14928=DIRECTION('center_axis',(-0.313163806483725,0.,0.949699126201885));
#14929=DIRECTION('ref_axis',(0.949699126201885,0.,0.313163806483725));
#14930=DIRECTION('center_axis',(0.,-1.,0.));
#14931=DIRECTION('ref_axis',(0.,0.,-1.));
#14932=DIRECTION('center_axis',(0.74528868282298,0.,0.666741913528756));
#14933=DIRECTION('ref_axis',(0.666741913528756,0.,-0.74528868282298));
#14934=DIRECTION('center_axis',(0.661925770683741,-7.41191641853799E-15,
0.749569392454585));
#14935=DIRECTION('ref_axis',(-0.749569392454585,-3.03668228410464E-29,0.661925770683741));
#14936=DIRECTION('center_axis',(0.,1.,0.));
#14937=DIRECTION('ref_axis',(0.,0.,1.));
#14938=DIRECTION('center_axis',(-0.749569392454584,-4.86640976974696E-15,
0.661925770683743));
#14939=DIRECTION('ref_axis',(0.661925770683743,3.23979850088036E-29,0.749569392454583));
#14940=DIRECTION('center_axis',(0.707341067972173,0.66728170096705,0.233246104178626));
#14941=DIRECTION('ref_axis',(-0.686208895312839,0.727404531188481,-7.51299950387033E-16));
#14942=DIRECTION('center_axis',(0.,1.,0.));
#14943=DIRECTION('ref_axis',(0.,0.,1.));
#14944=DIRECTION('center_axis',(-0.658838329408371,0.,0.752284557665773));
#14945=DIRECTION('ref_axis',(0.752284557665773,0.,0.658838329408371));
#14946=DIRECTION('center_axis',(-0.949699126201879,0.,-0.313163806483744));
#14947=DIRECTION('ref_axis',(0.221440263540013,-0.707106741740204,-0.671538729686443));
#14948=DIRECTION('center_axis',(0.94969912620188,0.,0.313163806483739));
#14949=DIRECTION('ref_axis',(0.313163806483739,0.,-0.94969912620188));
#14950=DIRECTION('center_axis',(-0.949699126201878,0.,-0.313163806483745));
#14951=DIRECTION('ref_axis',(-0.313163806483745,0.,0.949699126201878));
#14952=DIRECTION('center_axis',(-0.313163806483749,0.,0.949699126201877));
#14953=DIRECTION('ref_axis',(-0.949699126201877,-3.33066907387545E-14,-0.31316380648375));
#14954=DIRECTION('center_axis',(0.,-1.,0.));
#14955=DIRECTION('ref_axis',(2.22044604925031E-14,0.,1.));
#14956=DIRECTION('center_axis',(0.,1.,0.));
#14957=DIRECTION('ref_axis',(1.,0.,0.));
#14958=DIRECTION('center_axis',(-0.676807035378407,-2.98251420004092E-14,
-0.736160469505319));
#14959=DIRECTION('ref_axis',(0.736160469505319,9.88665375602713E-29,-0.676807035378407));
#14960=DIRECTION('center_axis',(0.,1.,0.));
#14961=DIRECTION('ref_axis',(1.,0.,0.));
#14962=DIRECTION('center_axis',(-0.230857726232391,0.675697700970532,0.70009808394392));
#14963=DIRECTION('ref_axis',(-4.57530847286819E-14,0.719534496560286,-0.694456700061088));
#14964=DIRECTION('center_axis',(0.313163806483745,0.,-0.949699126201878));
#14965=DIRECTION('ref_axis',(0.949699126201878,0.,0.313163806483745));
#14966=DIRECTION('center_axis',(-0.532938710021185,0.,-0.846153846153851));
#14967=DIRECTION('ref_axis',(0.846153846153851,0.,-0.532938710021185));
#14968=DIRECTION('center_axis',(0.,0.,1.));
#14969=DIRECTION('ref_axis',(-1.,0.,0.));
#14970=DIRECTION('center_axis',(-3.49148133884313E-15,0.,1.));
#14971=DIRECTION('ref_axis',(1.,0.,3.49148133884313E-15));
#14972=DIRECTION('center_axis',(0.,0.,1.));
#14973=DIRECTION('ref_axis',(1.,0.,0.));
#14974=DIRECTION('center_axis',(0.,1.,0.));
#14975=DIRECTION('ref_axis',(0.,0.,1.));
#14976=DIRECTION('center_axis',(0.,-1.,0.));
#14977=DIRECTION('ref_axis',(2.22044604925031E-14,0.,1.));
#14978=DIRECTION('center_axis',(0.689471704147334,0.,-0.72431261840463));
#14979=DIRECTION('ref_axis',(0.72431261840463,-9.99200722162653E-14,0.689471704147334));
#14980=DIRECTION('center_axis',(0.,1.,0.));
#14981=DIRECTION('ref_axis',(0.,0.,1.));
#14982=DIRECTION('center_axis',(-0.313163806483747,0.,0.949699126201878));
#14983=DIRECTION('ref_axis',(-0.671538702807596,-0.707106770042692,-0.221440254676701));
#14984=DIRECTION('center_axis',(0.,-1.,0.));
#14985=DIRECTION('ref_axis',(0.,0.,-1.));
#14986=DIRECTION('center_axis',(0.,-1.,0.));
#14987=DIRECTION('ref_axis',(0.,0.,-1.));
#14988=DIRECTION('center_axis',(0.,-1.,0.));
#14989=DIRECTION('ref_axis',(0.,0.,-1.));
#14990=DIRECTION('center_axis',(0.313163806483747,0.,-0.949699126201878));
#14991=DIRECTION('ref_axis',(-0.949699126201878,0.,-0.313163806483747));
#14992=DIRECTION('center_axis',(0.313163806483745,0.,-0.949699126201878));
#14993=DIRECTION('ref_axis',(-0.949699126201878,0.,-0.313163806483745));
#14994=DIRECTION('center_axis',(0.,1.,0.));
#14995=DIRECTION('ref_axis',(0.,0.,1.));
#14996=DIRECTION('center_axis',(-0.75228455766577,0.,-0.658838329408374));
#14997=DIRECTION('ref_axis',(-0.658838329408373,0.,0.75228455766577));
#14998=DIRECTION('center_axis',(-0.532938710021199,0.,0.846153846153842));
#14999=DIRECTION('ref_axis',(-0.846153846153842,2.22044604925029E-14,-0.532938710021199));
#15000=DIRECTION('center_axis',(-0.0822611166573683,-0.0232075739980745,
0.996340562857604));
#15001=DIRECTION('ref_axis',(-0.920256040566064,-0.382000889613719,-0.0848772062216844));
#15002=DIRECTION('center_axis',(0.,-1.,0.));
#15003=DIRECTION('ref_axis',(0.,0.,-1.));
#15004=DIRECTION('center_axis',(0.,-1.,0.));
#15005=DIRECTION('ref_axis',(0.,0.,-1.));
#15006=DIRECTION('center_axis',(0.949699126201879,0.,0.313163806483744));
#15007=DIRECTION('ref_axis',(0.313163806483744,0.,-0.949699126201879));
#15008=DIRECTION('center_axis',(0.94969912620188,0.,0.313163806483741));
#15009=DIRECTION('ref_axis',(0.313163806483741,0.,-0.94969912620188));
#15010=DIRECTION('center_axis',(0.,-1.,0.));
#15011=DIRECTION('ref_axis',(0.,0.,-1.));
#15012=DIRECTION('center_axis',(0.666741913528764,1.03429581957828E-14,
-0.745288682822973));
#15013=DIRECTION('ref_axis',(-0.745288682822973,7.03701836569442E-29,-0.666741913528764));
#15014=DIRECTION('center_axis',(-0.700098083943913,-0.675697700970539,-0.230857726232389));
#15015=DIRECTION('ref_axis',(0.694456700061088,-0.719534496560286,-1.51950613122166E-15));
#15016=DIRECTION('center_axis',(-0.788816507333645,0.,-0.614628764180419));
#15017=DIRECTION('ref_axis',(0.614628764180419,0.,-0.788816507333645));
#15018=DIRECTION('center_axis',(-0.313163806483745,4.34602085546888E-15,
0.949699126201878));
#15019=DIRECTION('ref_axis',(-0.949699126201878,-3.01782747192566E-29,-0.313163806483745));
#15020=DIRECTION('center_axis',(0.,1.,0.));
#15021=DIRECTION('ref_axis',(0.,0.,1.));
#15022=DIRECTION('center_axis',(-0.561307971766392,0.,0.827607008689209));
#15023=DIRECTION('ref_axis',(0.827607008689208,0.,0.561307971766392));
#15024=DIRECTION('center_axis',(-0.68176580877798,0.69617142649707,-0.224812648466096));
#15025=DIRECTION('ref_axis',(-0.714460172310607,-0.699676112341916,-6.69170701730011E-16));
#15026=DIRECTION('center_axis',(0.68176580877798,0.69617142649707,0.224812648466096));
#15027=DIRECTION('ref_axis',(-0.714460172310607,0.699676112341916,-6.69170701730011E-16));
#15028=DIRECTION('center_axis',(0.,1.,0.));
#15029=DIRECTION('ref_axis',(0.,0.,1.));
#15030=DIRECTION('center_axis',(-0.564137640058907,-1.99148461346573E-14,
0.825680763412087));
#15031=DIRECTION('ref_axis',(0.825680763412087,-1.41167664996661E-28,0.564137640058907));
#15032=DIRECTION('center_axis',(0.,1.,0.));
#15033=DIRECTION('ref_axis',(1.,0.,0.));
#15034=DIRECTION('center_axis',(-0.736160469505319,-2.04325575765918E-14,
0.676807035378407));
#15035=DIRECTION('ref_axis',(-0.676807035378407,6.6818274548834E-29,-0.736160469505319));
#15036=DIRECTION('center_axis',(0.,1.,0.));
#15037=DIRECTION('ref_axis',(-0.966074959183014,0.,0.258261830783294));
#15038=DIRECTION('center_axis',(-0.949699126201878,0.,-0.313163806483745));
#15039=DIRECTION('ref_axis',(0.313163806483745,0.,-0.949699126201878));
#15040=DIRECTION('center_axis',(0.,-1.,0.));
#15041=DIRECTION('ref_axis',(0.0776244824205716,0.,0.996982667717417));
#15042=DIRECTION('center_axis',(0.,-1.,0.));
#15043=DIRECTION('ref_axis',(0.,0.,-1.));
#15044=DIRECTION('center_axis',(-0.313163806483747,0.,0.949699126201878));
#15045=DIRECTION('ref_axis',(0.949699126201878,0.,0.313163806483747));
#15046=DIRECTION('center_axis',(-0.313163806483745,0.,0.949699126201878));
#15047=DIRECTION('ref_axis',(0.949699126201878,0.,0.313163806483745));
#15048=DIRECTION('center_axis',(0.,-1.,0.));
#15049=DIRECTION('ref_axis',(0.,0.,-1.));
#15050=DIRECTION('center_axis',(-0.708724510210478,-9.83552836689824E-15,
-0.705485342602465));
#15051=DIRECTION('ref_axis',(-0.705485342602465,5.77298571474757E-29,0.708724510210478));
#15052=DIRECTION('center_axis',(0.313163806483747,0.,-0.949699126201878));
#15053=DIRECTION('ref_axis',(0.671538729685915,-0.707106741740759,0.221440263539842));
#15054=DIRECTION('center_axis',(-0.313163806483747,0.,0.949699126201878));
#15055=DIRECTION('ref_axis',(0.949699126201878,0.,0.313163806483747));
#15056=DIRECTION('center_axis',(-0.949699126201878,0.,-0.313163806483745));
#15057=DIRECTION('ref_axis',(0.313163806483745,-3.33066907387545E-14,-0.949699126201878));
#15058=DIRECTION('center_axis',(0.542858691574087,-1.16549000115722E-14,
-0.839824053586506));
#15059=DIRECTION('ref_axis',(0.839824053586506,4.4408920985006E-14,0.542858691574087));
#15060=DIRECTION('center_axis',(-0.542858691574087,-1.16549000115722E-14,
0.839824053586506));
#15061=DIRECTION('ref_axis',(-0.839824053586506,-2.22044604925029E-14,-0.542858691574087));
#15062=DIRECTION('center_axis',(-0.564137640058907,9.65795169688271E-15,
0.825680763412087));
#15063=DIRECTION('ref_axis',(-0.825680763412087,3.33066907387545E-14,-0.564137640058907));
#15064=DIRECTION('center_axis',(0.,-1.,0.));
#15065=DIRECTION('ref_axis',(0.,0.,1.));
#15066=DIRECTION('center_axis',(0.,-1.,0.));
#15067=DIRECTION('ref_axis',(0.,0.,-1.));
#15068=DIRECTION('center_axis',(-0.567158351856161,0.,0.823608768724449));
#15069=DIRECTION('ref_axis',(0.823608768724449,0.,0.567158351856161));
#15070=DIRECTION('center_axis',(-0.949699126201879,0.,-0.313163806483744));
#15071=DIRECTION('ref_axis',(-0.313163806483744,0.,0.949699126201879));
#15072=DIRECTION('center_axis',(0.949699126201878,4.34602085546888E-15,
0.313163806483745));
#15073=DIRECTION('ref_axis',(0.313163806483745,1.5175460366485E-29,-0.949699126201878));
#15074=DIRECTION('center_axis',(0.,-1.,0.));
#15075=DIRECTION('ref_axis',(0.315582053959229,0.,0.948898291293052));
#15076=DIRECTION('center_axis',(0.,-1.,0.));
#15077=DIRECTION('ref_axis',(0.,0.,-1.));
#15078=DIRECTION('center_axis',(0.,-1.,0.));
#15079=DIRECTION('ref_axis',(0.,0.,-1.));
#15080=DIRECTION('center_axis',(-0.949699126201879,0.,-0.313163806483744));
#15081=DIRECTION('ref_axis',(-0.313163806483744,0.,0.949699126201879));
#15082=DIRECTION('center_axis',(-0.949699126201878,0.,-0.313163806483745));
#15083=DIRECTION('ref_axis',(-0.313163806483745,0.,0.949699126201878));
#15084=DIRECTION('center_axis',(0.,-1.,0.));
#15085=DIRECTION('ref_axis',(0.0776244824205756,0.,0.996982667717417));
#15086=DIRECTION('center_axis',(-0.456384763068626,1.59504337716007E-16,
-0.889782528508396));
#15087=DIRECTION('ref_axis',(0.889782528508396,6.01132322447566E-31,-0.456384763068626));
#15088=DIRECTION('center_axis',(0.,1.,0.));
#15089=DIRECTION('ref_axis',(0.,0.,1.));
#15090=DIRECTION('center_axis',(-0.889782528508396,0.,0.456384763068626));
#15091=DIRECTION('ref_axis',(0.456384763068626,0.,0.889782528508396));
#15092=DIRECTION('center_axis',(-0.949699126201879,0.,-0.313163806483744));
#15093=DIRECTION('ref_axis',(0.221440254677041,-0.707106770041599,-0.671538702808635));
#15094=DIRECTION('center_axis',(-0.949699126201879,0.,-0.313163806483743));
#15095=DIRECTION('ref_axis',(0.313163806483743,-3.33066907387549E-14,-0.949699126201879));
#15096=DIRECTION('center_axis',(0.685171419647361,-0.692454480471773,0.225935650513563));
#15097=DIRECTION('ref_axis',(0.710835091671237,0.703358708234102,-1.55285432707423E-15));
#15098=DIRECTION('center_axis',(0.,-1.,0.));
#15099=DIRECTION('ref_axis',(0.,0.,-1.));
#15100=DIRECTION('center_axis',(0.567158351856161,0.,-0.823608768724449));
#15101=DIRECTION('ref_axis',(-0.823608768724449,0.,-0.567158351856161));
#15102=DIRECTION('center_axis',(0.949699126201879,0.,0.313163806483744));
#15103=DIRECTION('ref_axis',(0.313163806483744,0.,-0.949699126201879));
#15104=DIRECTION('center_axis',(-0.949699126201878,4.34602085546888E-15,
-0.313163806483745));
#15105=DIRECTION('ref_axis',(-0.313163806483745,1.5175460366485E-29,0.949699126201878));
#15106=DIRECTION('center_axis',(0.,1.,0.));
#15107=DIRECTION('ref_axis',(0.,0.,1.));
#15108=DIRECTION('center_axis',(0.,0.,-1.));
#15109=DIRECTION('ref_axis',(-1.,0.,0.));
#15110=DIRECTION('center_axis',(0.,0.,1.));
#15111=DIRECTION('ref_axis',(1.,0.,0.));
#15112=DIRECTION('center_axis',(0.,0.,-1.));
#15113=DIRECTION('ref_axis',(-1.,0.,0.));
#15114=DIRECTION('center_axis',(0.532938710021199,0.,-0.846153846153842));
#15115=DIRECTION('ref_axis',(0.846153846153842,0.,0.532938710021199));
#15116=DIRECTION('center_axis',(0.,1.,0.));
#15117=DIRECTION('ref_axis',(1.,0.,0.));
#15118=DIRECTION('center_axis',(-0.949699126201878,6.14109335297236E-14,
-0.313163806483745));
#15119=DIRECTION('ref_axis',(0.313163806483745,6.66133814775086E-14,-0.949699126201878));
#15120=DIRECTION('center_axis',(0.685171419647361,0.692454480471773,0.225935650513563));
#15121=DIRECTION('ref_axis',(0.71083509167124,-0.703358708234099,-2.35087979245205E-14));
#15122=DIRECTION('center_axis',(0.,1.,0.));
#15123=DIRECTION('ref_axis',(1.,0.,0.));
#15124=DIRECTION('center_axis',(0.57297676606922,0.,-0.81957161099251));
#15125=DIRECTION('ref_axis',(0.81957161099251,0.,0.57297676606922));
#15126=DIRECTION('center_axis',(0.,-1.,0.));
#15127=DIRECTION('ref_axis',(0.,0.,1.));
#15128=DIRECTION('center_axis',(0.,-1.,0.));
#15129=DIRECTION('ref_axis',(0.,0.,-1.));
#15130=DIRECTION('center_axis',(-0.949699126201879,0.,-0.313163806483742));
#15131=DIRECTION('ref_axis',(-0.313163806483742,0.,0.949699126201879));
#15132=DIRECTION('center_axis',(0.313163806483747,0.,-0.949699126201878));
#15133=DIRECTION('ref_axis',(-0.949699126201878,0.,-0.313163806483747));
#15134=DIRECTION('center_axis',(-0.313163806483745,3.29493073867411E-15,
0.949699126201878));
#15135=DIRECTION('ref_axis',(0.949699126201878,-5.77669955272155E-30,0.313163806483745));
#15136=DIRECTION('center_axis',(0.,1.,0.));
#15137=DIRECTION('ref_axis',(0.,0.,1.));
#15138=DIRECTION('center_axis',(0.,-1.,0.));
#15139=DIRECTION('ref_axis',(0.,0.,1.));
#15140=DIRECTION('center_axis',(0.,1.,0.));
#15141=DIRECTION('ref_axis',(1.,0.,0.));
#15142=DIRECTION('center_axis',(0.949699126201878,6.14109335297236E-14,
0.313163806483745));
#15143=DIRECTION('ref_axis',(-0.313163806483745,9.43689570931373E-14,0.949699126201878));
#15144=DIRECTION('center_axis',(0.,1.,0.));
#15145=DIRECTION('ref_axis',(1.,0.,0.));
#15146=DIRECTION('center_axis',(-0.57297676606922,0.,0.81957161099251));
#15147=DIRECTION('ref_axis',(-0.81957161099251,0.,-0.57297676606922));
#15148=DIRECTION('center_axis',(0.532938710021199,0.,0.846153846153842));
#15149=DIRECTION('ref_axis',(-0.846153846153842,0.,0.532938710021199));
#15150=DIRECTION('center_axis',(0.,1.,0.));
#15151=DIRECTION('ref_axis',(0.,0.,1.));
#15152=DIRECTION('center_axis',(0.561307971766392,0.,-0.827607008689209));
#15153=DIRECTION('ref_axis',(-0.827607008689208,0.,-0.561307971766392));
#15154=DIRECTION('center_axis',(0.949699126201879,0.,0.313163806483744));
#15155=DIRECTION('ref_axis',(0.313163806483744,0.,-0.949699126201879));
#15156=DIRECTION('center_axis',(-0.949699126201878,0.,-0.313163806483745));
#15157=DIRECTION('ref_axis',(-0.313163806483745,0.,0.949699126201878));
#15158=DIRECTION('center_axis',(0.,-1.,0.));
#15159=DIRECTION('ref_axis',(0.,0.,-1.));
#15160=DIRECTION('center_axis',(0.,-1.,0.));
#15161=DIRECTION('ref_axis',(0.,0.,-1.));
#15162=DIRECTION('center_axis',(0.,-1.,0.));
#15163=DIRECTION('ref_axis',(0.,0.,-1.));
#15164=DIRECTION('center_axis',(-0.949699126201879,0.,-0.313163806483744));
#15165=DIRECTION('ref_axis',(-0.313163806483744,0.,0.949699126201879));
#15166=DIRECTION('center_axis',(0.,-1.,0.));
#15167=DIRECTION('ref_axis',(0.,0.,-1.));
#15168=DIRECTION('center_axis',(-0.889782528508396,0.,0.456384763068626));
#15169=DIRECTION('ref_axis',(0.456384763068626,0.,0.889782528508396));
#15170=DIRECTION('center_axis',(0.,-1.,0.));
#15171=DIRECTION('ref_axis',(0.,0.,-1.));
#15172=DIRECTION('center_axis',(0.,-1.,0.));
#15173=DIRECTION('ref_axis',(0.,0.,-1.));
#15174=DIRECTION('center_axis',(-0.949699126201879,0.,-0.313163806483744));
#15175=DIRECTION('ref_axis',(-0.313163806483744,0.,0.949699126201879));
#15176=DIRECTION('center_axis',(0.949699126201878,0.,0.313163806483745));
#15177=DIRECTION('ref_axis',(0.313163806483745,0.,-0.949699126201878));
#15178=DIRECTION('center_axis',(0.,-1.,0.));
#15179=DIRECTION('ref_axis',(0.,0.,-1.));
#15180=DIRECTION('center_axis',(0.,1.,0.));
#15181=DIRECTION('ref_axis',(0.,0.,1.));
#15182=DIRECTION('center_axis',(0.661925770683734,-1.7968282226759E-15,
0.749569392454591));
#15183=DIRECTION('ref_axis',(0.749569392454591,-9.3759599088471E-30,-0.661925770683734));
#15184=DIRECTION('center_axis',(0.233246104178643,0.667281700967055,-0.707341067972163));
#15185=DIRECTION('ref_axis',(1.28973797951009E-15,0.727404531188473,0.686208895312847));
#15186=DIRECTION('center_axis',(0.,1.,0.));
#15187=DIRECTION('ref_axis',(0.,0.,1.));
#15188=DIRECTION('center_axis',(0.75228455766577,0.,0.658838329408374));
#15189=DIRECTION('ref_axis',(0.658838329408373,0.,-0.75228455766577));
#15190=DIRECTION('center_axis',(-0.313163806483754,0.,0.949699126201876));
#15191=DIRECTION('ref_axis',(-0.671538729686488,-0.707106741740154,-0.221440263540036));
#15192=DIRECTION('center_axis',(0.313163806483747,0.,-0.949699126201878));
#15193=DIRECTION('ref_axis',(-0.949699126201878,0.,-0.313163806483747));
#15194=DIRECTION('center_axis',(-0.313163806483745,-8.69204171093777E-15,
0.949699126201878));
#15195=DIRECTION('ref_axis',(0.949699126201878,-6.03565494385133E-29,0.313163806483745));
#15196=DIRECTION('center_axis',(0.949699126201878,0.,0.313163806483745));
#15197=DIRECTION('ref_axis',(-0.313163806483745,-3.33066907387545E-14,0.949699126201878));
#15198=DIRECTION('center_axis',(0.705485342602465,9.83552836689824E-15,
-0.708724510210478));
#15199=DIRECTION('ref_axis',(0.708724510210478,5.71963539909091E-29,0.705485342602465));
#15200=DIRECTION('center_axis',(0.,-1.,0.));
#15201=DIRECTION('ref_axis',(0.,0.,-1.));
#15202=DIRECTION('center_axis',(0.,-1.,0.));
#15203=DIRECTION('ref_axis',(-2.22044604925031E-14,0.,1.));
#15204=DIRECTION('center_axis',(-0.724312618404621,0.,-0.689471704147344));
#15205=DIRECTION('ref_axis',(0.689471704147344,-5.55111512312576E-15,-0.724312618404621));
#15206=DIRECTION('center_axis',(0.,1.,0.));
#15207=DIRECTION('ref_axis',(0.,0.,1.));
#15208=DIRECTION('center_axis',(0.889782528508396,0.,-0.456384763068626));
#15209=DIRECTION('ref_axis',(-0.456384763068626,0.,-0.889782528508396));
#15210=DIRECTION('center_axis',(0.949699126201879,0.,0.313163806483744));
#15211=DIRECTION('ref_axis',(-0.221440254676618,-0.707106770042951,0.671538702807351));
#15212=DIRECTION('center_axis',(0.949699126201878,0.,0.313163806483745));
#15213=DIRECTION('ref_axis',(0.313163806483745,0.,-0.949699126201878));
#15214=DIRECTION('center_axis',(0.,-1.,0.));
#15215=DIRECTION('ref_axis',(0.,0.,-1.));
#15216=DIRECTION('center_axis',(0.614628764180404,0.,-0.788816507333657));
#15217=DIRECTION('ref_axis',(-0.788816507333657,0.,-0.614628764180404));
#15218=DIRECTION('center_axis',(-0.949699126201879,0.,-0.313163806483744));
#15219=DIRECTION('ref_axis',(-0.313163806483744,0.,0.949699126201879));
#15220=DIRECTION('center_axis',(-0.949699126201879,0.,-0.313163806483743));
#15221=DIRECTION('ref_axis',(0.313163806483743,0.,-0.949699126201879));
#15222=DIRECTION('center_axis',(0.,-1.,0.));
#15223=DIRECTION('ref_axis',(0.297486285481071,0.,0.954726091583693));
#15224=DIRECTION('center_axis',(0.,-1.,0.));
#15225=DIRECTION('ref_axis',(0.,0.,-1.));
#15226=DIRECTION('center_axis',(0.313163806483754,0.,-0.949699126201876));
#15227=DIRECTION('ref_axis',(-0.949699126201876,0.,-0.313163806483754));
#15228=DIRECTION('center_axis',(0.313163806483745,0.,-0.949699126201878));
#15229=DIRECTION('ref_axis',(-0.949699126201878,0.,-0.313163806483745));
#15230=DIRECTION('center_axis',(0.,-1.,0.));
#15231=DIRECTION('ref_axis',(0.,0.,-1.));
#15232=DIRECTION('center_axis',(-0.745288682822956,1.03429581957826E-14,
-0.666741913528783));
#15233=DIRECTION('ref_axis',(-0.666741913528783,1.71777308129412E-29,0.745288682822956));
#15234=DIRECTION('center_axis',(-0.230857726232396,-0.675697700970517,0.700098083943933));
#15235=DIRECTION('ref_axis',(-1.21960194499758E-15,-0.719534496560307,-0.694456700061066));
#15236=DIRECTION('center_axis',(0.,1.,0.));
#15237=DIRECTION('ref_axis',(0.,0.,1.));
#15238=DIRECTION('center_axis',(0.,-1.,0.));
#15239=DIRECTION('ref_axis',(-5.55111512312578E-15,0.,1.));
#15240=DIRECTION('center_axis',(0.614628764180404,0.,-0.788816507333657));
#15241=DIRECTION('ref_axis',(0.788816507333657,0.,0.614628764180404));
#15242=DIRECTION('center_axis',(0.,1.,0.));
#15243=DIRECTION('ref_axis',(1.,0.,0.));
#15244=DIRECTION('center_axis',(0.676807035378399,-2.98251420004093E-14,
0.736160469505326));
#15245=DIRECTION('ref_axis',(-0.736160469505326,-4.54993050005069E-29,0.676807035378399));
#15246=DIRECTION('center_axis',(0.,1.,0.));
#15247=DIRECTION('ref_axis',(1.,0.,0.));
#15248=DIRECTION('center_axis',(-0.313163806483749,0.,0.949699126201877));
#15249=DIRECTION('ref_axis',(-0.949699126201877,0.,-0.31316380648375));
#15250=DIRECTION('center_axis',(0.,-1.,0.));
#15251=DIRECTION('ref_axis',(0.,0.,-1.));
#15252=DIRECTION('center_axis',(0.,-1.,0.));
#15253=DIRECTION('ref_axis',(0.,0.,-1.));
#15254=DIRECTION('center_axis',(0.949699126201879,0.,0.313163806483744));
#15255=DIRECTION('ref_axis',(0.313163806483744,0.,-0.949699126201879));
#15256=DIRECTION('center_axis',(0.949699126201877,0.,0.313163806483749));
#15257=DIRECTION('ref_axis',(0.313163806483749,0.,-0.949699126201877));
#15258=DIRECTION('center_axis',(0.,-1.,0.));
#15259=DIRECTION('ref_axis',(0.,0.,-1.));
#15260=DIRECTION('center_axis',(0.705485342602465,-9.83552836689824E-15,
-0.708724510210478));
#15261=DIRECTION('ref_axis',(-0.708724510210478,5.71963539909091E-29,-0.705485342602465));
#15262=DIRECTION('center_axis',(0.,-1.,0.));
#15263=DIRECTION('ref_axis',(0.,0.,-1.));
#15264=DIRECTION('center_axis',(0.,-1.,0.));
#15265=DIRECTION('ref_axis',(0.,0.,-1.));
#15266=DIRECTION('center_axis',(0.,1.,0.));
#15267=DIRECTION('ref_axis',(0.,0.,1.));
#15268=DIRECTION('center_axis',(0.949699126201879,0.,0.313163806483744));
#15269=DIRECTION('ref_axis',(0.313163806483744,0.,-0.949699126201879));
#15270=DIRECTION('center_axis',(0.949699126201878,0.,0.313163806483745));
#15271=DIRECTION('ref_axis',(0.313163806483745,0.,-0.949699126201878));
#15272=DIRECTION('center_axis',(-0.949699126201878,0.,-0.313163806483745));
#15273=DIRECTION('ref_axis',(-0.313163806483745,0.,0.949699126201878));
#15274=DIRECTION('center_axis',(0.,-1.,0.));
#15275=DIRECTION('ref_axis',(0.,0.,-1.));
#15276=DIRECTION('center_axis',(-0.313163806483754,0.,0.949699126201876));
#15277=DIRECTION('ref_axis',(0.949699126201876,0.,0.313163806483754));
#15278=DIRECTION('center_axis',(-0.313163806483758,0.,0.949699126201874));
#15279=DIRECTION('ref_axis',(0.949699126201874,0.,0.313163806483758));
#15280=DIRECTION('center_axis',(0.,-1.,0.));
#15281=DIRECTION('ref_axis',(0.,0.,-1.));
#15282=DIRECTION('center_axis',(-0.889782528508396,0.,0.456384763068626));
#15283=DIRECTION('ref_axis',(-0.456384763068626,0.,-0.889782528508396));
#15284=DIRECTION('center_axis',(0.,1.,0.));
#15285=DIRECTION('ref_axis',(1.,0.,0.));
#15286=DIRECTION('center_axis',(-0.700098083943913,0.675697700970539,-0.230857726232389));
#15287=DIRECTION('ref_axis',(0.69445670006108,0.719534496560294,4.50025703477272E-14));
#15288=DIRECTION('center_axis',(0.666741913528764,-1.03429581957828E-14,
-0.745288682822973));
#15289=DIRECTION('ref_axis',(0.745288682822973,5.55111512312587E-15,0.666741913528764));
#15290=DIRECTION('center_axis',(0.,-1.,0.));
#15291=DIRECTION('ref_axis',(0.,0.,-1.));
#15292=DIRECTION('center_axis',(0.689471704147334,0.,-0.72431261840463));
#15293=DIRECTION('ref_axis',(-0.72431261840463,0.,-0.689471704147334));
#15294=DIRECTION('center_axis',(-0.949699126201879,0.,-0.313163806483744));
#15295=DIRECTION('ref_axis',(-0.313163806483744,0.,0.949699126201879));
#15296=DIRECTION('center_axis',(-0.94969912620188,0.,-0.313163806483741));
#15297=DIRECTION('ref_axis',(-0.313163806483741,0.,0.94969912620188));
#15298=DIRECTION('center_axis',(0.,-1.,0.));
#15299=DIRECTION('ref_axis',(0.,0.,-1.));
#15300=DIRECTION('center_axis',(-0.736160469505319,2.04325575765918E-14,
0.676807035378407));
#15301=DIRECTION('ref_axis',(0.676807035378407,6.6818274548834E-29,0.736160469505319));
#15302=DIRECTION('center_axis',(0.,-1.,0.));
#15303=DIRECTION('ref_axis',(0.,0.,1.));
#15304=DIRECTION('center_axis',(0.,-1.,0.));
#15305=DIRECTION('ref_axis',(0.,0.,-1.));
#15306=DIRECTION('center_axis',(-0.313163806483752,0.,0.949699126201876));
#15307=DIRECTION('ref_axis',(0.949699126201876,0.,0.313163806483752));
#15308=DIRECTION('center_axis',(0.949699126201879,0.,0.313163806483744));
#15309=DIRECTION('ref_axis',(0.313163806483744,0.,-0.949699126201879));
#15310=DIRECTION('center_axis',(-0.949699126201879,0.,-0.313163806483742));
#15311=DIRECTION('ref_axis',(-0.313163806483742,0.,0.949699126201879));
#15312=DIRECTION('center_axis',(0.707341067972173,-0.66728170096705,0.233246104178626));
#15313=DIRECTION('ref_axis',(-0.686208895312839,-0.727404531188481,-7.51299950387033E-16));
#15314=DIRECTION('center_axis',(0.,1.,0.));
#15315=DIRECTION('ref_axis',(-0.977517882722095,0.,0.210852528935538));
#15316=DIRECTION('center_axis',(0.,1.,0.));
#15317=DIRECTION('ref_axis',(0.,0.,-1.));
#15318=DIRECTION('center_axis',(0.,-1.,0.));
#15319=DIRECTION('ref_axis',(0.225340727186267,0.,0.974280019640742));
#15320=DIRECTION('center_axis',(0.,-1.,0.));
#15321=DIRECTION('ref_axis',(0.,0.,-1.));
#15322=DIRECTION('center_axis',(-0.313163806483754,0.,0.949699126201876));
#15323=DIRECTION('ref_axis',(0.949699126201876,0.,0.313163806483754));
#15324=DIRECTION('center_axis',(0.,-1.,0.));
#15325=DIRECTION('ref_axis',(0.,0.,-1.));
#15326=DIRECTION('center_axis',(-0.949699126201878,4.34602085546888E-15,
-0.313163806483745));
#15327=DIRECTION('ref_axis',(0.313163806483745,-3.02285113016155E-29,-0.949699126201878));
#15328=DIRECTION('center_axis',(-0.658838329408371,0.,0.752284557665773));
#15329=DIRECTION('ref_axis',(-0.752284557665773,-2.77555756156289E-14,-0.658838329408371));
#15330=DIRECTION('center_axis',(0.,1.,0.));
#15331=DIRECTION('ref_axis',(0.,0.,1.));
#15332=DIRECTION('center_axis',(-0.846153846153842,0.,0.532938710021199));
#15333=DIRECTION('ref_axis',(0.532938710021199,0.,0.846153846153842));
#15334=DIRECTION('center_axis',(0.,-1.,0.));
#15335=DIRECTION('ref_axis',(0.,0.,-1.));
#15336=DIRECTION('center_axis',(0.,1.,0.));
#15337=DIRECTION('ref_axis',(0.,0.,1.));
#15338=DIRECTION('center_axis',(-0.708724510210478,-9.83552836689824E-15,
-0.705485342602465));
#15339=DIRECTION('ref_axis',(0.705485342602465,-5.77298571474757E-29,-0.708724510210478));
#15340=DIRECTION('center_axis',(0.949699126201879,0.,0.313163806483744));
#15341=DIRECTION('ref_axis',(-0.221440263539776,-0.707106741740963,0.671538729685723));
#15342=DIRECTION('center_axis',(-0.949699126201879,0.,-0.313163806483744));
#15343=DIRECTION('ref_axis',(-0.313163806483744,0.,0.949699126201879));
#15344=DIRECTION('center_axis',(-1.,0.,0.));
#15345=DIRECTION('ref_axis',(0.,0.,-1.));
#15346=DIRECTION('center_axis',(-0.749569392454584,4.86640976974694E-15,
0.661925770683743));
#15347=DIRECTION('ref_axis',(-0.661925770683743,3.17031459090513E-29,-0.749569392454584));
#15348=DIRECTION('center_axis',(0.,-1.,0.));
#15349=DIRECTION('ref_axis',(0.,0.,-1.));
#15350=DIRECTION('center_axis',(-0.788816507333645,0.,-0.614628764180419));
#15351=DIRECTION('ref_axis',(-0.614628764180419,0.,0.788816507333645));
#15352=DIRECTION('center_axis',(0.313163806483754,0.,-0.949699126201876));
#15353=DIRECTION('ref_axis',(-0.949699126201876,0.,-0.313163806483754));
#15354=DIRECTION('center_axis',(0.,1.,0.));
#15355=DIRECTION('ref_axis',(0.,0.,1.));
#15356=DIRECTION('center_axis',(-0.456384763068618,0.,-0.8897825285084));
#15357=DIRECTION('ref_axis',(-0.8897825285084,0.,0.456384763068618));
#15358=DIRECTION('center_axis',(-1.,0.,0.));
#15359=DIRECTION('ref_axis',(0.,0.,1.));
#15360=DIRECTION('center_axis',(-1.,0.,0.));
#15361=DIRECTION('ref_axis',(0.,0.,1.));
#15362=DIRECTION('center_axis',(0.,1.,0.));
#15363=DIRECTION('ref_axis',(0.,0.,1.));
#15364=DIRECTION('center_axis',(0.,1.,0.));
#15365=DIRECTION('ref_axis',(-1.11022302462516E-14,0.,-1.));
#15366=DIRECTION('center_axis',(0.,1.,0.));
#15367=DIRECTION('ref_axis',(-0.0776244824205643,0.,-0.996982667717418));
#15368=DIRECTION('center_axis',(-0.313163806483752,0.,0.949699126201876));
#15369=DIRECTION('ref_axis',(-0.949699126201876,0.,-0.313163806483752));
#15370=DIRECTION('center_axis',(-0.846153846153842,0.,-0.532938710021199));
#15371=DIRECTION('ref_axis',(0.532938710021199,0.,-0.846153846153842));
#15372=DIRECTION('center_axis',(-0.996340562857841,-0.0232075739972549,
-0.0822611166547301));
#15373=DIRECTION('ref_axis',(0.0848772062189317,-0.382000889613913,-0.920256040566237));
#15374=DIRECTION('center_axis',(0.,-1.,0.));
#15375=DIRECTION('ref_axis',(0.,0.,-1.));
#15376=DIRECTION('center_axis',(0.,1.,0.));
#15377=DIRECTION('ref_axis',(0.,0.,1.));
#15378=DIRECTION('center_axis',(0.313163806483754,0.,-0.949699126201876));
#15379=DIRECTION('ref_axis',(0.671538702806552,-0.70710677004379,0.221440254676362));
#15380=DIRECTION('center_axis',(-0.313163806483745,0.,0.949699126201878));
#15381=DIRECTION('ref_axis',(0.949699126201878,0.,0.313163806483745));
#15382=DIRECTION('center_axis',(0.,1.,0.));
#15383=DIRECTION('ref_axis',(0.,0.,1.));
#15384=DIRECTION('center_axis',(-0.827607008689209,0.,-0.561307971766392));
#15385=DIRECTION('ref_axis',(-0.561307971766392,0.,0.827607008689208));
#15386=DIRECTION('center_axis',(0.,1.,0.));
#15387=DIRECTION('ref_axis',(0.,0.,1.));
#15388=DIRECTION('center_axis',(-0.825680763412081,7.71138778898377E-15,
-0.564137640058916));
#15389=DIRECTION('ref_axis',(-0.564137640058916,-2.44199728449863E-29,0.825680763412081));
#15390=DIRECTION('center_axis',(0.,-1.,0.));
#15391=DIRECTION('ref_axis',(0.,0.,-1.));
#15392=DIRECTION('center_axis',(0.,-1.,0.));
#15393=DIRECTION('ref_axis',(0.,0.,-1.));
#15394=DIRECTION('center_axis',(0.,1.,0.));
#15395=DIRECTION('ref_axis',(0.,0.,1.));
#15396=DIRECTION('center_axis',(0.,-1.,0.));
#15397=DIRECTION('ref_axis',(0.,0.,-1.));
#15398=DIRECTION('center_axis',(0.819571610992504,0.,0.572976766069229));
#15399=DIRECTION('ref_axis',(0.572976766069229,0.,-0.819571610992504));
#15400=DIRECTION('center_axis',(0.313163806483758,0.,-0.949699126201874));
#15401=DIRECTION('ref_axis',(0.949699126201874,5.55111512312577E-15,0.313163806483758));
#15402=DIRECTION('center_axis',(0.,1.,0.));
#15403=DIRECTION('ref_axis',(1.,0.,0.));
#15404=DIRECTION('center_axis',(-0.313163806483745,-4.34602085546888E-15,
0.949699126201878));
#15405=DIRECTION('ref_axis',(-0.949699126201878,1.50881680010028E-29,-0.313163806483745));
#15406=DIRECTION('center_axis',(0.313163806483754,0.,-0.949699126201876));
#15407=DIRECTION('ref_axis',(-0.949699126201876,0.,-0.313163806483754));
#15408=DIRECTION('center_axis',(0.313163806483745,-5.70649126742547E-14,
-0.949699126201878));
#15409=DIRECTION('ref_axis',(-0.949699126201878,-3.98789244989641E-28,-0.313163806483745));
#15410=DIRECTION('center_axis',(-0.225935650513579,-0.692454480471764,0.685171419647365));
#15411=DIRECTION('ref_axis',(5.0708331257006E-16,-0.70335870823411,-0.710835091671229));
#15412=DIRECTION('center_axis',(0.224812648466099,0.69617142649706,-0.68176580877799));
#15413=DIRECTION('ref_axis',(1.59296345262975E-15,0.699676112341926,0.714460172310597));
#15414=DIRECTION('center_axis',(-0.313163806483753,0.,0.949699126201876));
#15415=DIRECTION('ref_axis',(0.949699126201876,0.,0.313163806483754));
#15416=DIRECTION('center_axis',(0.,1.,0.));
#15417=DIRECTION('ref_axis',(-0.947774827752477,0.,0.318940238726257));
#15418=DIRECTION('center_axis',(-0.823608768724459,0.,-0.567158351856147));
#15419=DIRECTION('ref_axis',(0.567158351856147,4.44089209850067E-14,-0.823608768724459));
#15420=DIRECTION('center_axis',(0.839824053586503,0.,0.542858691574091));
#15421=DIRECTION('ref_axis',(-0.542858691574091,6.66133814775089E-14,0.839824053586503));
#15422=DIRECTION('center_axis',(0.,-1.,0.));
#15423=DIRECTION('ref_axis',(0.,0.,-1.));
#15424=DIRECTION('center_axis',(0.500078040677557,0.706998150315573,-0.500075562972692));
#15425=DIRECTION('ref_axis',(-0.487455410628725,0.707106781187,0.512237467048381));
#15426=DIRECTION('center_axis',(0.500078143315287,0.706996252576076,-0.500078143315344));
#15427=DIRECTION('ref_axis',(2.88606387015194E-15,0.57747058809669,0.816411489313608));
#15428=DIRECTION('center_axis',(-0.500075464669955,-0.707000041916729,0.500075464669955));
#15429=DIRECTION('ref_axis',(2.20421081150854E-15,-0.577466463418735,-0.816414406797589));
#15430=DIRECTION('center_axis',(0.,1.,0.));
#15431=DIRECTION('ref_axis',(1.,0.,0.));
#15432=DIRECTION('center_axis',(0.724563445309596,1.40751544109608E-14,
0.689208106250273));
#15433=DIRECTION('ref_axis',(-0.689208106250273,5.95362936016406E-29,0.724563445309596));
#15434=DIRECTION('center_axis',(0.,1.,0.));
#15435=DIRECTION('ref_axis',(1.,0.,0.));
#15436=DIRECTION('center_axis',(-0.707106781186534,0.,0.707106781186561));
#15437=DIRECTION('ref_axis',(-0.707106781186561,0.,-0.707106781186534));
#15438=DIRECTION('center_axis',(0.724265465251865,-1.96202318550286E-14,
0.68952123668782));
#15439=DIRECTION('ref_axis',(-0.68952123668782,-2.7755575615629E-14,0.724265465251865));
#15440=DIRECTION('center_axis',(0.,1.,0.));
#15441=DIRECTION('ref_axis',(-7.65709097232158E-16,0.,-1.));
#15442=DIRECTION('center_axis',(0.724563445309603,-9.43334816904809E-15,
-0.689208106250266));
#15443=DIRECTION('ref_axis',(-0.689208106250266,2.1657800856212E-29,-0.724563445309603));
#15444=DIRECTION('center_axis',(0.,1.,0.));
#15445=DIRECTION('ref_axis',(0.,0.,1.));
#15446=DIRECTION('center_axis',(0.707106781186551,0.,-0.707106781186544));
#15447=DIRECTION('ref_axis',(-0.707106781186544,0.,-0.707106781186551));
#15448=DIRECTION('center_axis',(-0.707106781186548,0.,0.707106781186548));
#15449=DIRECTION('ref_axis',(0.707106781186548,0.,0.707106781186548));
#15450=DIRECTION('center_axis',(0.,1.,0.));
#15451=DIRECTION('ref_axis',(1.,0.,0.));
#15452=DIRECTION('center_axis',(0.724563445309596,1.49735685222987E-16,
0.689208106250273));
#15453=DIRECTION('ref_axis',(-0.689208106250273,-1.38777878078143E-15,0.724563445309596));
#15454=DIRECTION('center_axis',(-0.500078143315301,0.706996252576096,0.500078143315301));
#15455=DIRECTION('ref_axis',(-6.82379179808067E-16,0.577470588096647,-0.816411489313638));
#15456=DIRECTION('center_axis',(0.,1.,0.));
#15457=DIRECTION('ref_axis',(1.,0.,0.));
#15458=DIRECTION('center_axis',(0.500078143315295,-0.706996252576104,0.500078143315295));
#15459=DIRECTION('ref_axis',(-2.4326062740384E-14,0.577470588096627,0.816411489313652));
#15460=DIRECTION('center_axis',(1.,0.,0.));
#15461=DIRECTION('ref_axis',(0.,0.,1.));
#15462=DIRECTION('center_axis',(-0.985559589508073,-0.169328956556991,-1.055202794374E-16));
#15463=DIRECTION('ref_axis',(-0.169328956556991,0.985559589508073,-2.75791750167464E-32));
#15464=DIRECTION('center_axis',(0.,1.,0.));
#15465=DIRECTION('ref_axis',(0.707106781186548,0.,-0.707106781186548));
#15466=DIRECTION('center_axis',(0.707106781186548,9.81307786677359E-15,
-0.707106781186548));
#15467=DIRECTION('ref_axis',(-0.707106781186548,-3.73353565333889E-32,-0.707106781186548));
#15468=DIRECTION('center_axis',(-0.500065457858295,0.707014197674946,0.500065457858294));
#15469=DIRECTION('ref_axis',(-0.816425305441283,-0.577451054752788,2.42893944196122E-17));
#15470=DIRECTION('center_axis',(0.,1.,0.));
#15471=DIRECTION('ref_axis',(1.89882616186822E-15,0.,-1.));
#15472=DIRECTION('center_axis',(0.724563445309596,1.34013438274573E-14,
-0.689208106250273));
#15473=DIRECTION('ref_axis',(-0.689208106250273,5.6910531650358E-29,-0.724563445309596));
#15474=DIRECTION('center_axis',(-0.500076315109388,0.706998838848565,-0.500076315109401));
#15475=DIRECTION('ref_axis',(-0.707106781188416,-2.6290097559751E-12,0.707106781184679));
#15476=DIRECTION('center_axis',(0.50007546466997,-0.707000041916716,0.50007546466996));
#15477=DIRECTION('ref_axis',(0.816414406797577,0.577466463418752,-1.98804944403104E-15));
#15478=DIRECTION('center_axis',(0.,1.,0.));
#15479=DIRECTION('ref_axis',(0.,0.,1.));
#15480=DIRECTION('center_axis',(0.724265465251897,0.,-0.689521236687785));
#15481=DIRECTION('ref_axis',(-0.689521236687785,0.,-0.724265465251897));
#15482=DIRECTION('center_axis',(-0.985559589508072,0.169328956556993,0.));
#15483=DIRECTION('ref_axis',(-0.169328956556993,-0.985559589508072,0.));
#15484=DIRECTION('center_axis',(-1.,0.,1.95461800110063E-16));
#15485=DIRECTION('ref_axis',(1.95461800110063E-16,0.,1.));
#15486=DIRECTION('center_axis',(1.,0.,0.));
#15487=DIRECTION('ref_axis',(0.,0.,-1.));
#15488=DIRECTION('center_axis',(-0.707106781186549,0.,0.707106781186546));
#15489=DIRECTION('ref_axis',(0.707106781186546,0.,0.707106781186549));
#15490=DIRECTION('center_axis',(0.707106781186548,-9.81307786677359E-15,
-0.707106781186548));
#15491=DIRECTION('ref_axis',(-0.707106781186548,3.73353565333889E-32,-0.707106781186548));
#15492=DIRECTION('center_axis',(0.,1.,0.));
#15493=DIRECTION('ref_axis',(1.,0.,0.));
#15494=DIRECTION('center_axis',(0.723101268110532,0.,0.690742032930486));
#15495=DIRECTION('ref_axis',(-0.690742032930486,-5.55111512312578E-15,0.723101268110532));
#15496=DIRECTION('center_axis',(-0.707106781186548,1.96261557335472E-14,
0.707106781186548));
#15497=DIRECTION('ref_axis',(-0.707106781186548,7.46707130667779E-32,-0.707106781186548));
#15498=DIRECTION('center_axis',(0.,1.,0.));
#15499=DIRECTION('ref_axis',(1.,0.,0.));
#15500=DIRECTION('center_axis',(0.50007814331529,0.706996252576075,0.500078143315342));
#15501=DIRECTION('ref_axis',(2.42101966234701E-15,0.577470588096689,-0.816411489313609));
#15502=DIRECTION('center_axis',(0.,1.,0.));
#15503=DIRECTION('ref_axis',(1.,0.,0.));
#15504=DIRECTION('center_axis',(0.707106781186548,0.,0.707106781186548));
#15505=DIRECTION('ref_axis',(-0.707106781186548,-4.99600361081318E-14,0.707106781186548));
#15506=DIRECTION('center_axis',(-1.,0.,0.));
#15507=DIRECTION('ref_axis',(0.,0.,-1.));
#15508=DIRECTION('center_axis',(0.,1.,0.));
#15509=DIRECTION('ref_axis',(0.,0.,1.));
#15510=DIRECTION('center_axis',(0.,0.,1.));
#15511=DIRECTION('ref_axis',(1.,0.,0.));
#15512=DIRECTION('center_axis',(0.,1.,0.));
#15513=DIRECTION('ref_axis',(-0.999924538176052,0.,-0.0122848668453797));
#15514=DIRECTION('center_axis',(0.50007546466995,0.707000041916716,-0.50007546466998));
#15515=DIRECTION('ref_axis',(1.4509032190736E-15,-0.577466463418761,-0.81641440679757));
#15516=DIRECTION('center_axis',(-0.689521236687775,0.,-0.724265465251907));
#15517=DIRECTION('ref_axis',(0.724265465251907,-6.66133814775095E-14,-0.689521236687775));
#15518=DIRECTION('center_axis',(0.707106781186551,0.,-0.707106781186544));
#15519=DIRECTION('ref_axis',(-0.707106781186544,0.,-0.707106781186551));
#15520=DIRECTION('center_axis',(0.,-1.,0.));
#15521=DIRECTION('ref_axis',(0.,0.,-1.));
#15522=DIRECTION('center_axis',(0.50006545785829,0.707014197674953,0.50006545785829));
#15523=DIRECTION('ref_axis',(1.98508446711413E-15,-0.577451054752781,0.816425305441288));
#15524=DIRECTION('center_axis',(0.707106781186548,0.,0.707106781186547));
#15525=DIRECTION('ref_axis',(0.707106781186547,0.,-0.707106781186548));
#15526=DIRECTION('center_axis',(0.707106781186548,0.,0.707106781186548));
#15527=DIRECTION('ref_axis',(0.707106781186548,0.,-0.707106781186548));
#15528=DIRECTION('center_axis',(-1.,0.,1.95461800110063E-16));
#15529=DIRECTION('ref_axis',(1.95461800110063E-16,0.,1.));
#15530=DIRECTION('center_axis',(-1.,0.,0.));
#15531=DIRECTION('ref_axis',(0.,0.,1.));
#15532=DIRECTION('center_axis',(3.29601953873307E-15,0.,-1.));
#15533=DIRECTION('ref_axis',(-1.,0.,-3.29601953873307E-15));
#15534=DIRECTION('center_axis',(0.,0.,1.));
#15535=DIRECTION('ref_axis',(1.,0.,0.));
#15536=DIRECTION('center_axis',(0.,1.,0.));
#15537=DIRECTION('ref_axis',(0.,0.,1.));
#15538=DIRECTION('center_axis',(0.500076315108452,0.706998838849897,-0.500076315108454));
#15539=DIRECTION('ref_axis',(-0.707106781185304,-1.76214707967051E-12,-0.707106781187791));
#15540=DIRECTION('center_axis',(0.500078143315292,0.706996252576109,-0.500078143315292));
#15541=DIRECTION('ref_axis',(-2.6156794477156E-15,0.577470588096634,0.816411489313647));
#15542=DIRECTION('center_axis',(-0.928799626502546,0.370582317183012,0.));
#15543=DIRECTION('ref_axis',(0.370582317183012,0.928799626502546,0.));
#15544=DIRECTION('center_axis',(1.,0.,0.));
#15545=DIRECTION('ref_axis',(0.,0.,1.));
#15546=DIRECTION('center_axis',(0.,1.,0.));
#15547=DIRECTION('ref_axis',(1.,0.,0.));
#15548=DIRECTION('center_axis',(0.707106781186527,0.,0.707106781186568));
#15549=DIRECTION('ref_axis',(-0.707106781186568,-1.11022302462515E-14,0.707106781186527));
#15550=DIRECTION('center_axis',(-0.723101268110554,1.00350459623997E-14,
0.690742032930463));
#15551=DIRECTION('ref_axis',(-0.690742032930463,-1.66533453693774E-14,-0.723101268110554));
#15552=DIRECTION('center_axis',(0.,1.,0.));
#15553=DIRECTION('ref_axis',(-0.707106781186543,0.,-0.707106781186552));
#15554=DIRECTION('center_axis',(-0.707106781186534,0.,-0.707106781186561));
#15555=DIRECTION('ref_axis',(-0.707106781186561,0.,0.707106781186534));
#15556=DIRECTION('center_axis',(0.,1.,0.));
#15557=DIRECTION('ref_axis',(0.,0.,1.));
#15558=DIRECTION('center_axis',(0.,0.,1.));
#15559=DIRECTION('ref_axis',(1.,0.,0.));
#15560=DIRECTION('center_axis',(-3.41934671378744E-15,-0.16932895655699,
0.985559589508073));
#15561=DIRECTION('ref_axis',(2.22044604925031E-14,0.985559589508073,0.16932895655699));
#15562=DIRECTION('center_axis',(0.,1.,0.));
#15563=DIRECTION('ref_axis',(-0.999921859736202,0.,-0.0125009768296196));
#15564=DIRECTION('center_axis',(1.9135348438956E-14,1.,2.01169630281381E-14));
#15565=DIRECTION('ref_axis',(-3.99449913460614E-29,2.01169630281381E-14,
-1.));
#15566=DIRECTION('center_axis',(-0.689208106250273,-1.49735685222987E-16,
-0.724563445309596));
#15567=DIRECTION('ref_axis',(0.724563445309596,-3.33066907387544E-14,-0.689208106250273));
#15568=DIRECTION('center_axis',(-0.707106781186549,0.,0.707106781186546));
#15569=DIRECTION('ref_axis',(0.707106781186546,0.,0.707106781186549));
#15570=DIRECTION('center_axis',(0.707106781186548,0.,-0.707106781186548));
#15571=DIRECTION('ref_axis',(-0.707106781186548,0.,-0.707106781186548));
#15572=DIRECTION('center_axis',(1.,0.,-1.95461800110063E-16));
#15573=DIRECTION('ref_axis',(-1.95461800110063E-16,0.,-1.));
#15574=DIRECTION('center_axis',(1.,0.,0.));
#15575=DIRECTION('ref_axis',(0.,0.,-1.));
#15576=DIRECTION('center_axis',(-0.928799626502548,-0.370582317183008,0.));
#15577=DIRECTION('ref_axis',(0.370582317183008,-0.928799626502548,0.));
#15578=DIRECTION('center_axis',(0.,-1.,0.));
#15579=DIRECTION('ref_axis',(0.,0.,-1.));
#15580=DIRECTION('center_axis',(0.707106781186548,0.,0.707106781186547));
#15581=DIRECTION('ref_axis',(0.707106781186547,0.,-0.707106781186548));
#15582=DIRECTION('center_axis',(-0.707106781186547,0.,-0.707106781186548));
#15583=DIRECTION('ref_axis',(-0.707106781186548,0.,0.707106781186547));
#15584=DIRECTION('center_axis',(-0.707106781186554,0.,-0.707106781186541));
#15585=DIRECTION('ref_axis',(-0.707106781186541,0.,0.707106781186555));
#15586=DIRECTION('center_axis',(0.,1.,0.));
#15587=DIRECTION('ref_axis',(0.,0.,1.));
#15588=DIRECTION('center_axis',(-0.689521236687795,-4.82173031558679E-16,
0.724265465251888));
#15589=DIRECTION('ref_axis',(0.724265465251888,1.69629386130297E-30,0.689521236687795));
#15590=DIRECTION('center_axis',(0.,0.,1.));
#15591=DIRECTION('ref_axis',(1.,0.,0.));
#15592=DIRECTION('center_axis',(0.,0.,1.));
#15593=DIRECTION('ref_axis',(1.,0.,0.));
#15594=DIRECTION('center_axis',(-2.13887076994181E-15,0.169328956556989,
0.985559589508073));
#15595=DIRECTION('ref_axis',(3.73711604924882E-30,-0.985559589508073,0.169328956556989));
#15596=DIRECTION('center_axis',(0.,1.,0.));
#15597=DIRECTION('ref_axis',(0.,0.,1.));
#15598=DIRECTION('center_axis',(0.689208106250273,-1.34013438274573E-14,
-0.724563445309596));
#15599=DIRECTION('ref_axis',(-0.724563445309596,5.71414998426326E-29,-0.689208106250273));
#15600=DIRECTION('center_axis',(0.,1.,0.));
#15601=DIRECTION('ref_axis',(0.,0.,1.));
#15602=DIRECTION('center_axis',(1.47242188377274E-14,1.,-1.47242188377274E-14));
#15603=DIRECTION('ref_axis',(-7.97092275109852E-30,1.47242188377274E-14,
1.));
#15604=DIRECTION('center_axis',(-0.500065457858282,0.707014197674965,0.500065457858282));
#15605=DIRECTION('ref_axis',(6.38344604276266E-16,-0.577451054752767,0.816425305441298));
#15606=DIRECTION('center_axis',(0.50007814331533,-0.706996252576075,-0.500078143315302));
#15607=DIRECTION('ref_axis',(0.816411489313614,0.577470588096681,1.159905104889E-15));
#15608=DIRECTION('center_axis',(0.,1.,0.));
#15609=DIRECTION('ref_axis',(-0.999934544283097,0.,-0.0114414662240507));
#15610=DIRECTION('center_axis',(-0.690742032930436,0.,-0.72310126811058));
#15611=DIRECTION('ref_axis',(0.72310126811058,2.22044604925031E-14,-0.690742032930436));
#15612=DIRECTION('center_axis',(0.,-1.,0.));
#15613=DIRECTION('ref_axis',(0.,0.,-1.));
#15614=DIRECTION('center_axis',(0.,0.,1.));
#15615=DIRECTION('ref_axis',(1.,0.,0.));
#15616=DIRECTION('center_axis',(-1.,0.,0.));
#15617=DIRECTION('ref_axis',(0.,0.,-1.));
#15618=DIRECTION('center_axis',(0.,1.,0.));
#15619=DIRECTION('ref_axis',(1.,0.,0.));
#15620=DIRECTION('center_axis',(-0.500075464669968,0.707000041916711,-0.500075464669968));
#15621=DIRECTION('ref_axis',(2.74612154635474E-15,-0.577466463418753,-0.816414406797576));
#15622=DIRECTION('center_axis',(-1.17495566440827E-15,-0.16932895655699,
0.985559589508073));
#15623=DIRECTION('ref_axis',(2.22044604925031E-14,0.985559589508073,0.16932895655699));
#15624=DIRECTION('center_axis',(0.,0.,1.));
#15625=DIRECTION('ref_axis',(-1.,0.,0.));
#15626=DIRECTION('center_axis',(0.,1.,0.));
#15627=DIRECTION('ref_axis',(-0.999921859736202,0.,0.0125009768296196));
#15628=DIRECTION('center_axis',(-1.96322917836366E-14,1.,-1.96322917836366E-14));
#15629=DIRECTION('ref_axis',(-5.04975666092073E-29,-1.96322917836366E-14,
-1.));
#15630=DIRECTION('center_axis',(-0.500078143315344,-0.706996252576076,-0.500078143315287));
#15631=DIRECTION('ref_axis',(-0.816411489313608,0.57747058809669,2.88849236575815E-15));
#15632=DIRECTION('center_axis',(0.,1.,0.));
#15633=DIRECTION('ref_axis',(-0.999921859736202,0.,-0.0125009768296196));
#15634=DIRECTION('center_axis',(-0.689208106250266,4.79154192713555E-15,
-0.724563445309603));
#15635=DIRECTION('ref_axis',(0.724563445309603,1.06481884149609E-29,-0.689208106250266));
#15636=DIRECTION('center_axis',(0.,-1.,0.));
#15637=DIRECTION('ref_axis',(0.,0.,-1.));
#15638=DIRECTION('center_axis',(-3.29601953873307E-15,0.,1.));
#15639=DIRECTION('ref_axis',(1.,0.,3.29601953873307E-15));
#15640=DIRECTION('center_axis',(0.,0.,1.));
#15641=DIRECTION('ref_axis',(1.,0.,0.));
#15642=DIRECTION('center_axis',(1.,0.,-1.95461800110063E-16));
#15643=DIRECTION('ref_axis',(-1.95461800110063E-16,0.,-1.));
#15644=DIRECTION('center_axis',(-1.,0.,0.));
#15645=DIRECTION('ref_axis',(0.,0.,1.));
#15646=DIRECTION('center_axis',(-0.707106781186547,0.,-0.707106781186548));
#15647=DIRECTION('ref_axis',(-0.707106781186548,0.,0.707106781186547));
#15648=DIRECTION('center_axis',(-0.707106781186548,-3.92523114670943E-14,
-0.707106781186548));
#15649=DIRECTION('ref_axis',(-0.707106781186548,-1.49341426133556E-31,0.707106781186548));
#15650=DIRECTION('center_axis',(-0.500075562974082,0.706998150315597,-0.500078040676132));
#15651=DIRECTION('ref_axis',(0.512237467050394,0.70710678118697,0.487455410626653));
#15652=DIRECTION('center_axis',(-0.500078143315344,0.706996252576076,-0.500078143315287));
#15653=DIRECTION('ref_axis',(-0.816411489313608,-0.57747058809669,2.88849236575815E-15));
#15654=DIRECTION('center_axis',(0.,0.169328956556991,0.985559589508073));
#15655=DIRECTION('ref_axis',(0.,-0.985559589508073,0.169328956556991));
#15656=DIRECTION('center_axis',(3.29601953873307E-15,0.,-1.));
#15657=DIRECTION('ref_axis',(-1.,0.,-3.29601953873307E-15));
#15658=DIRECTION('center_axis',(0.,0.,1.));
#15659=DIRECTION('ref_axis',(-1.,0.,0.));
#15660=DIRECTION('center_axis',(0.,1.,0.));
#15661=DIRECTION('ref_axis',(0.,0.,1.));
#15662=DIRECTION('center_axis',(0.689521236687795,-4.82173031558679E-16,
-0.724265465251888));
#15663=DIRECTION('ref_axis',(-0.724265465251888,1.69629386130297E-30,-0.689521236687795));
#15664=DIRECTION('center_axis',(0.500075562974512,0.706998150315606,0.500078040675689));
#15665=DIRECTION('ref_axis',(-0.512237467041965,0.707106781187116,-0.487455410635299));
#15666=DIRECTION('center_axis',(-0.500075464669968,-0.707000041916711,-0.500075464669968));
#15667=DIRECTION('ref_axis',(2.74612154635474E-15,0.577466463418753,-0.816414406797576));
#15668=DIRECTION('center_axis',(0.,1.,0.));
#15669=DIRECTION('ref_axis',(0.,0.,1.));
#15670=DIRECTION('center_axis',(-1.43515113292173E-14,1.,1.50877222711036E-14));
#15671=DIRECTION('ref_axis',(-2.55233473732771E-30,-1.50877222711036E-14,
1.));
#15672=DIRECTION('center_axis',(0.,1.,0.));
#15673=DIRECTION('ref_axis',(0.,0.,1.));
#15674=DIRECTION('center_axis',(0.689208106250266,9.43334816904809E-15,
-0.724563445309603));
#15675=DIRECTION('ref_axis',(-0.724563445309603,2.1210382338014E-29,-0.689208106250266));
#15676=DIRECTION('center_axis',(0.,0.370582317183008,0.928799626502548));
#15677=DIRECTION('ref_axis',(-2.22044604925031E-14,0.928799626502548,-0.370582317183008));
#15678=DIRECTION('center_axis',(0.,-1.,0.));
#15679=DIRECTION('ref_axis',(0.,0.,-1.));
#15680=DIRECTION('center_axis',(0.,0.,1.));
#15681=DIRECTION('ref_axis',(1.,0.,0.));
#15682=DIRECTION('center_axis',(0.,1.,0.));
#15683=DIRECTION('ref_axis',(1.,0.,0.));
#15684=DIRECTION('center_axis',(-0.500065457858323,-0.707014197674947,-0.500065457858266));
#15685=DIRECTION('ref_axis',(-0.816425305441277,0.577451054752798,2.3871826158738E-14));
#15686=DIRECTION('center_axis',(0.690742032930456,0.,-0.723101268110561));
#15687=DIRECTION('ref_axis',(0.723101268110561,5.55111512312578E-15,0.690742032930456));
#15688=DIRECTION('center_axis',(0.,1.,0.));
#15689=DIRECTION('ref_axis',(1.,0.,0.));
#15690=DIRECTION('center_axis',(0.689208106250273,1.34013438274573E-14,
-0.724563445309596));
#15691=DIRECTION('ref_axis',(0.724563445309596,-6.10622663543829E-14,0.689208106250273));
#15692=DIRECTION('center_axis',(1.96322917836366E-14,1.,1.96322917836366E-14));
#15693=DIRECTION('ref_axis',(-5.04975666092073E-29,1.96322917836366E-14,
-1.));
#15694=DIRECTION('center_axis',(0.,0.,1.));
#15695=DIRECTION('ref_axis',(-1.,0.,0.));
#15696=DIRECTION('center_axis',(0.,1.,0.));
#15697=DIRECTION('ref_axis',(0.,0.,1.));
#15698=DIRECTION('center_axis',(-1.,0.,0.));
#15699=DIRECTION('ref_axis',(0.,0.,1.));
#15700=DIRECTION('center_axis',(0.,1.,0.));
#15701=DIRECTION('ref_axis',(-0.999924538176025,0.,0.0122848668475855));
#15702=DIRECTION('center_axis',(-0.707106781186554,0.,-0.707106781186541));
#15703=DIRECTION('ref_axis',(0.707106781186541,0.,-0.707106781186555));
#15704=DIRECTION('center_axis',(0.,1.,0.));
#15705=DIRECTION('ref_axis',(-0.999921859736202,0.,0.0125009768296196));
#15706=DIRECTION('center_axis',(-0.500078143315298,0.7069962525761,-0.500078143315298));
#15707=DIRECTION('ref_axis',(-7.12726278488012E-16,-0.577470588096643,-0.816411489313641));
#15708=DIRECTION('center_axis',(0.,-0.370582317183023,0.928799626502542));
#15709=DIRECTION('ref_axis',(0.,-0.928799626502542,-0.370582317183023));
#15710=DIRECTION('center_axis',(0.,0.,-1.));
#15711=DIRECTION('ref_axis',(-1.,0.,0.));
#15712=DIRECTION('center_axis',(0.,0.,1.));
#15713=DIRECTION('ref_axis',(1.,0.,0.));
#15714=DIRECTION('center_axis',(0.,-1.,0.));
#15715=DIRECTION('ref_axis',(0.,0.,-1.));
#15716=DIRECTION('center_axis',(-0.500078143315298,-0.7069962525761,-0.500078143315298));
#15717=DIRECTION('ref_axis',(-2.68615379510983E-16,0.577470588096642,-0.816411489313641));
#15718=DIRECTION('center_axis',(0.,1.,0.));
#15719=DIRECTION('ref_axis',(0.,0.,1.));
#15720=DIRECTION('center_axis',(1.43515113292173E-14,1.,-1.50877222711036E-14));
#15721=DIRECTION('ref_axis',(-2.55233473732771E-30,1.50877222711036E-14,
1.));
#15722=DIRECTION('center_axis',(0.,1.,0.));
#15723=DIRECTION('ref_axis',(0.,0.,1.));
#15724=DIRECTION('center_axis',(-0.689208106250259,-5.54022035325041E-15,
-0.724563445309609));
#15725=DIRECTION('ref_axis',(-0.72456344530961,-4.03502369944906E-29,0.689208106250259));
#15726=DIRECTION('center_axis',(-0.500076315109219,0.706998838848823,0.500076315109206));
#15727=DIRECTION('ref_axis',(0.707106781184693,-2.61479889240196E-12,0.707106781188402));
#15728=DIRECTION('center_axis',(0.500075464669981,-0.707000041916716,-0.500075464669948));
#15729=DIRECTION('ref_axis',(0.816414406797569,0.577466463418763,-2.91626173010388E-15));
#15730=DIRECTION('center_axis',(-0.5000781433153,0.706996252576104,0.50007814331529));
#15731=DIRECTION('ref_axis',(-0.816411489313642,-0.577470588096642,-1.83698748637925E-16));
#15732=DIRECTION('center_axis',(0.,1.,0.));
#15733=DIRECTION('ref_axis',(0.,0.,1.));
#15734=DIRECTION('center_axis',(-0.689521236687795,0.,-0.724265465251888));
#15735=DIRECTION('ref_axis',(-0.724265465251888,0.,0.689521236687795));
#15736=DIRECTION('center_axis',(0.,0.,1.));
#15737=DIRECTION('ref_axis',(1.,0.,0.));
#15738=DIRECTION('center_axis',(0.,2.77555756156289E-14,1.));
#15739=DIRECTION('ref_axis',(0.,-1.,2.77555756156289E-14));
#15740=DIRECTION('center_axis',(1.,0.,-1.95461800110063E-16));
#15741=DIRECTION('ref_axis',(-1.95461800110063E-16,0.,-1.));
#15742=DIRECTION('center_axis',(-1.,0.,0.));
#15743=DIRECTION('ref_axis',(0.,0.,1.));
#15744=DIRECTION('center_axis',(0.707106781186547,0.,0.707106781186548));
#15745=DIRECTION('ref_axis',(0.707106781186548,0.,-0.707106781186547));
#15746=DIRECTION('center_axis',(-0.500065457858323,0.707014197674947,-0.500065457858266));
#15747=DIRECTION('ref_axis',(-0.816425305441268,-0.57745105475281,-2.24141339905632E-15));
#15748=DIRECTION('center_axis',(0.,-1.,0.));
#15749=DIRECTION('ref_axis',(0.,0.,-1.));
#15750=DIRECTION('center_axis',(0.690742032930456,0.,-0.723101268110561));
#15751=DIRECTION('ref_axis',(-0.723101268110561,0.,-0.690742032930456));
#15752=DIRECTION('center_axis',(0.,0.,1.));
#15753=DIRECTION('ref_axis',(-1.,0.,0.));
#15754=DIRECTION('center_axis',(0.,0.370582317183012,0.928799626502546));
#15755=DIRECTION('ref_axis',(2.22044604925031E-14,0.928799626502546,-0.370582317183012));
#15756=DIRECTION('center_axis',(0.,1.,0.));
#15757=DIRECTION('ref_axis',(1.,0.,0.));
#15758=DIRECTION('center_axis',(0.689208106250266,-9.43334816904809E-15,
-0.724563445309603));
#15759=DIRECTION('ref_axis',(0.724563445309603,-1.38777878078143E-15,0.689208106250266));
#15760=DIRECTION('center_axis',(0.,1.,0.));
#15761=DIRECTION('ref_axis',(1.,0.,0.));
#15762=DIRECTION('center_axis',(-1.91353484389562E-14,1.,-2.01169630281383E-14));
#15763=DIRECTION('ref_axis',(-3.99449913460581E-29,-2.01169630281383E-14,
-1.));
#15764=DIRECTION('center_axis',(0.,1.,0.));
#15765=DIRECTION('ref_axis',(1.,0.,0.));
#15766=DIRECTION('center_axis',(0.707106781186554,-3.92523114670943E-14,
-0.707106781186541));
#15767=DIRECTION('ref_axis',(0.707106781186541,-3.33066907387542E-14,0.707106781186555));
#15768=DIRECTION('center_axis',(0.,1.,0.));
#15769=DIRECTION('ref_axis',(0.,0.,1.));
#15770=DIRECTION('center_axis',(1.,0.,0.));
#15771=DIRECTION('ref_axis',(0.,0.,-1.));
#15772=DIRECTION('center_axis',(-0.985559589508072,-0.169328956556993,0.));
#15773=DIRECTION('ref_axis',(-0.169328956556993,0.985559589508072,2.22044604925031E-14));
#15774=DIRECTION('center_axis',(0.,1.,0.));
#15775=DIRECTION('ref_axis',(-0.999934544283124,0.,0.0114414662216631));
#15776=DIRECTION('center_axis',(-0.707106781186548,3.92523114670943E-14,
-0.707106781186548));
#15777=DIRECTION('ref_axis',(0.707106781186548,-1.49341426133556E-31,-0.707106781186548));
#15778=DIRECTION('center_axis',(-3.29601953873307E-15,0.,1.));
#15779=DIRECTION('ref_axis',(1.,0.,3.29601953873307E-15));
#15780=DIRECTION('center_axis',(0.,0.,1.));
#15781=DIRECTION('ref_axis',(-1.,0.,0.));
#15782=DIRECTION('center_axis',(0.,-0.370582317183008,0.928799626502548));
#15783=DIRECTION('ref_axis',(0.,-0.928799626502548,-0.370582317183008));
#15784=DIRECTION('center_axis',(0.,1.,0.));
#15785=DIRECTION('ref_axis',(0.,0.,1.));
#15786=DIRECTION('center_axis',(-0.689208106250266,3.72093177779119E-14,
-0.724563445309603));
#15787=DIRECTION('ref_axis',(-0.724563445309603,-8.3586004851558E-29,0.689208106250266));
#15788=DIRECTION('center_axis',(0.,1.,0.));
#15789=DIRECTION('ref_axis',(0.,0.,1.));
#15790=DIRECTION('center_axis',(-1.47242188377277E-14,1.,1.47242188377274E-14));
#15791=DIRECTION('ref_axis',(-1.,-1.47242188377277E-14,7.9709227510944E-30));
#15792=DIRECTION('center_axis',(0.707106781186554,0.,-0.707106781186541));
#15793=DIRECTION('ref_axis',(-0.707106781186541,0.,-0.707106781186554));
#15794=DIRECTION('center_axis',(1.,0.,-1.95461800110063E-16));
#15795=DIRECTION('ref_axis',(-1.95461800110063E-16,0.,-1.));
#15796=DIRECTION('center_axis',(1.,0.,0.));
#15797=DIRECTION('ref_axis',(0.,0.,-1.));
#15798=DIRECTION('center_axis',(-0.985559589508073,0.169328956556991,-1.055202794374E-16));
#15799=DIRECTION('ref_axis',(-0.169328956556991,-0.985559589508073,-2.75791750167464E-32));
#15800=DIRECTION('center_axis',(0.,1.,0.));
#15801=DIRECTION('ref_axis',(0.,0.,1.));
#15802=DIRECTION('center_axis',(-0.724265465251897,0.,0.689521236687785));
#15803=DIRECTION('ref_axis',(0.689521236687785,0.,0.724265465251897));
#15804=DIRECTION('center_axis',(-0.707106781186548,0.,-0.707106781186547));
#15805=DIRECTION('ref_axis',(-0.707106781186547,0.,0.707106781186548));
#15806=DIRECTION('center_axis',(0.707106781186548,0.,0.707106781186548));
#15807=DIRECTION('ref_axis',(0.707106781186548,0.,-0.707106781186548));
#15808=DIRECTION('center_axis',(0.707106781186547,0.,0.707106781186548));
#15809=DIRECTION('ref_axis',(0.707106781186548,0.,-0.707106781186547));
#15810=DIRECTION('center_axis',(-0.707106781186548,0.,-0.707106781186548));
#15811=DIRECTION('ref_axis',(-0.707106781186548,0.,0.707106781186548));
#15812=DIRECTION('center_axis',(0.,-1.,0.));
#15813=DIRECTION('ref_axis',(0.,0.,-1.));
#15814=DIRECTION('center_axis',(-1.,0.,0.));
#15815=DIRECTION('ref_axis',(0.,0.,1.));
#15816=DIRECTION('center_axis',(0.,0.,1.));
#15817=DIRECTION('ref_axis',(-1.,0.,0.));
#15818=DIRECTION('center_axis',(0.,1.,0.));
#15819=DIRECTION('ref_axis',(1.,0.,0.));
#15820=DIRECTION('center_axis',(0.500078143315342,0.706996252576075,-0.50007814331529));
#15821=DIRECTION('ref_axis',(0.816411489313607,-0.577470588096692,-3.592237284197E-15));
#15822=DIRECTION('center_axis',(0.,1.,0.));
#15823=DIRECTION('ref_axis',(1.,0.,0.));
#15824=DIRECTION('center_axis',(0.50007546466997,0.707000041916716,0.50007546466996));
#15825=DIRECTION('ref_axis',(0.816414406797577,-0.577466463418752,-1.98804944403104E-15));
#15826=DIRECTION('center_axis',(0.,-1.,0.));
#15827=DIRECTION('ref_axis',(0.707106781186548,0.,0.707106781186548));
#15828=DIRECTION('center_axis',(0.707106781186561,0.,0.707106781186534));
#15829=DIRECTION('ref_axis',(0.707106781186534,0.,-0.707106781186561));
#15830=DIRECTION('center_axis',(-1.,0.,1.95461800110063E-16));
#15831=DIRECTION('ref_axis',(1.95461800110063E-16,0.,1.));
#15832=DIRECTION('center_axis',(-1.,0.,0.));
#15833=DIRECTION('ref_axis',(0.,0.,1.));
#15834=DIRECTION('center_axis',(0.,0.,-1.));
#15835=DIRECTION('ref_axis',(-1.,0.,0.));
#15836=DIRECTION('center_axis',(-2.77555756156289E-14,0.,1.));
#15837=DIRECTION('ref_axis',(1.,0.,2.77555756156289E-14));
#15838=DIRECTION('center_axis',(0.,-1.,0.));
#15839=DIRECTION('ref_axis',(0.,0.,-1.));
#15840=DIRECTION('center_axis',(-0.690742032930428,1.0933195161307E-14,
-0.723101268110587));
#15841=DIRECTION('ref_axis',(-0.723101268110587,-7.09354204639614E-29,0.690742032930428));
#15842=DIRECTION('center_axis',(0.500065457858296,0.707014197674951,-0.500065457858286));
#15843=DIRECTION('ref_axis',(-0.816425305441284,0.577451054752786,1.01752225400829E-15));
#15844=DIRECTION('center_axis',(-0.707106781186556,0.,0.707106781186539));
#15845=DIRECTION('ref_axis',(0.707106781186539,0.,0.707106781186556));
#15846=DIRECTION('center_axis',(-0.707106781186541,0.,0.707106781186554));
#15847=DIRECTION('ref_axis',(0.707106781186554,0.,0.707106781186541));
#15848=DIRECTION('center_axis',(0.,1.,0.));
#15849=DIRECTION('ref_axis',(0.,0.,1.));
#15850=DIRECTION('center_axis',(0.724265465251865,1.96202318550286E-14,
0.68952123668782));
#15851=DIRECTION('ref_axis',(0.68952123668782,-2.20983281568644E-29,-0.724265465251865));
#15852=DIRECTION('center_axis',(0.500076315110995,0.706998838846295,0.500076315111003));
#15853=DIRECTION('ref_axis',(0.707106781192132,-7.88702926797483E-12,-0.707106781180963));
#15854=DIRECTION('center_axis',(0.500078143315295,0.706996252576104,0.500078143315295));
#15855=DIRECTION('ref_axis',(1.82105156671187E-15,-0.577470588096639,0.816411489313644));
#15856=DIRECTION('center_axis',(-0.707106781186548,0.,-0.707106781186547));
#15857=DIRECTION('ref_axis',(-0.707106781186547,0.,0.707106781186548));
#15858=DIRECTION('center_axis',(0.707106781186527,0.,0.707106781186568));
#15859=DIRECTION('ref_axis',(0.707106781186568,0.,-0.707106781186527));
#15860=DIRECTION('center_axis',(0.,-1.,0.));
#15861=DIRECTION('ref_axis',(0.,0.,-1.));
#15862=DIRECTION('center_axis',(-0.723101268110554,-1.00350459623997E-14,
0.690742032930463));
#15863=DIRECTION('ref_axis',(0.690742032930463,-8.19100136791555E-29,0.723101268110554));
#15864=DIRECTION('center_axis',(-0.928799626502548,0.370582317183008,0.));
#15865=DIRECTION('ref_axis',(0.370582317183008,0.928799626502548,-2.22044604925031E-14));
#15866=DIRECTION('center_axis',(0.,-1.,0.));
#15867=DIRECTION('ref_axis',(0.,0.,-1.));
#15868=DIRECTION('center_axis',(1.,0.,0.));
#15869=DIRECTION('ref_axis',(0.,0.,-1.));
#15870=DIRECTION('center_axis',(0.,1.,0.));
#15871=DIRECTION('ref_axis',(1.,0.,0.));
#15872=DIRECTION('center_axis',(0.707106781186554,0.,-0.707106781186541));
#15873=DIRECTION('ref_axis',(0.707106781186541,0.,0.707106781186555));
#15874=DIRECTION('center_axis',(0.,1.,0.));
#15875=DIRECTION('ref_axis',(1.,0.,0.));
#15876=DIRECTION('center_axis',(-0.50007546466996,0.707000041916729,0.50007546466995));
#15877=DIRECTION('ref_axis',(0.816414406797587,0.577466463418738,-1.14723735947441E-16));
#15878=DIRECTION('center_axis',(0.,1.,0.));
#15879=DIRECTION('ref_axis',(1.,0.,0.));
#15880=DIRECTION('center_axis',(-2.01169630281381E-14,1.,1.91353484389564E-14));
#15881=DIRECTION('ref_axis',(1.,2.01169630281381E-14,-3.99449913460622E-29));
#15882=DIRECTION('center_axis',(0.,1.,0.));
#15883=DIRECTION('ref_axis',(1.,0.,0.));
#15884=DIRECTION('center_axis',(0.50006545785829,-0.707014197674953,0.50006545785829));
#15885=DIRECTION('ref_axis',(1.98508446711413E-15,0.577451054752781,0.816425305441288));
#15886=DIRECTION('center_axis',(-0.928799626502548,-0.370582317183008,0.));
#15887=DIRECTION('ref_axis',(0.370582317183008,-0.928799626502548,0.));
#15888=DIRECTION('center_axis',(-1.,0.,1.95461800110063E-16));
#15889=DIRECTION('ref_axis',(1.95461800110063E-16,0.,1.));
#15890=DIRECTION('center_axis',(1.,0.,0.));
#15891=DIRECTION('ref_axis',(0.,0.,-1.));
#15892=DIRECTION('center_axis',(0.707106781186554,0.,-0.707106781186541));
#15893=DIRECTION('ref_axis',(-0.707106781186541,0.,-0.707106781186554));
#15894=DIRECTION('center_axis',(0.707106781186554,-9.81307786677349E-15,
-0.707106781186541));
#15895=DIRECTION('ref_axis',(-0.707106781186541,-9.64572967081383E-29,-0.707106781186555));
#15896=DIRECTION('center_axis',(-0.50007804067718,0.706998150315576,0.500075562973064));
#15897=DIRECTION('ref_axis',(0.487455410632167,0.707106781187069,-0.512237467045011));
#15898=DIRECTION('center_axis',(-0.500078143315285,0.706996252576076,0.500078143315346));
#15899=DIRECTION('ref_axis',(-1.79407009105894E-15,-0.577470588096693,0.816411489313605));
#15900=DIRECTION('center_axis',(0.,1.,0.));
#15901=DIRECTION('ref_axis',(0.0125009768296248,0.,-0.999921859736202));
#15902=DIRECTION('center_axis',(1.47242188377274E-14,1.,1.47242188377274E-14));
#15903=DIRECTION('ref_axis',(7.97092275109852E-30,-1.47242188377274E-14,
1.));
#15904=DIRECTION('center_axis',(0.50007814331529,-0.706996252576075,0.500078143315342));
#15905=DIRECTION('ref_axis',(2.42101966234701E-15,-0.577470588096689,-0.816411489313609));
#15906=DIRECTION('center_axis',(0.,-1.,0.));
#15907=DIRECTION('ref_axis',(-0.707106781186559,0.,0.707106781186536));
#15908=DIRECTION('center_axis',(-0.707106781186548,1.96261557335473E-14,
0.707106781186548));
#15909=DIRECTION('ref_axis',(0.707106781186548,-3.26127331168573E-31,0.707106781186548));
#15910=DIRECTION('center_axis',(0.,1.,0.));
#15911=DIRECTION('ref_axis',(1.,0.,0.));
#15912=DIRECTION('center_axis',(1.96322917836368E-14,1.,-1.96322917836364E-14));
#15913=DIRECTION('ref_axis',(1.,-1.96322917836368E-14,-5.0497566609203E-29));
#15914=DIRECTION('center_axis',(0.,1.,0.));
#15915=DIRECTION('ref_axis',(1.,0.,0.));
#15916=DIRECTION('center_axis',(0.,-1.,0.));
#15917=DIRECTION('ref_axis',(0.,0.,-1.));
#15918=DIRECTION('center_axis',(0.723101268110551,0.,0.690742032930466));
#15919=DIRECTION('ref_axis',(0.690742032930466,0.,-0.723101268110551));
#15920=DIRECTION('center_axis',(-0.707106781186556,0.,0.707106781186539));
#15921=DIRECTION('ref_axis',(0.707106781186539,0.,0.707106781186556));
#15922=DIRECTION('center_axis',(-0.707106781186548,-9.81307786677359E-15,
0.707106781186548));
#15923=DIRECTION('ref_axis',(0.707106781186548,3.73353565333889E-32,0.707106781186548));
#15924=DIRECTION('center_axis',(0.,1.,0.));
#15925=DIRECTION('ref_axis',(-0.0125009768300713,0.,-0.999921859736197));
#15926=DIRECTION('center_axis',(-1.63450324603621E-14,1.,-1.55474706066522E-14));
#15927=DIRECTION('ref_axis',(-1.,-1.63450324603621E-14,-4.79348589056631E-30));
#15928=DIRECTION('center_axis',(0.,1.,0.));
#15929=DIRECTION('ref_axis',(1.,0.,0.));
#15930=DIRECTION('center_axis',(-0.500065457858285,-0.707014197674951,0.500065457858298));
#15931=DIRECTION('ref_axis',(-3.21586666640058E-16,0.577451054752787,0.816425305441284));
#15932=DIRECTION('center_axis',(0.,1.,0.));
#15933=DIRECTION('ref_axis',(1.,0.,0.));
#15934=DIRECTION('center_axis',(0.500078143315307,0.706996252576094,-0.500078143315297));
#15935=DIRECTION('ref_axis',(0.816411489313626,-0.577470588096664,-2.37338946977257E-14));
#15936=DIRECTION('center_axis',(-0.0822611166573126,0.0232075739978801,
0.996340562857613));
#15937=DIRECTION('ref_axis',(-0.996607302542098,0.000737174162972365,-0.0823003104126366));
#15938=DIRECTION('center_axis',(-0.99634056285741,0.0232075739985405,0.0822611166595799));
#15939=DIRECTION('ref_axis',(0.0848772062239051,0.382000889613703,0.920256040565866));
#15940=DIRECTION('center_axis',(0.996340562857634,0.0232075739980609,0.0822611166570035));
#15941=DIRECTION('ref_axis',(-0.082300310412331,0.000737174163135013,0.996607302542123));
#15942=DIRECTION('center_axis',(1.,0.,0.));
#15943=DIRECTION('ref_axis',(0.,0.,-1.));
#15944=DIRECTION('center_axis',(1.,0.,0.));
#15945=DIRECTION('ref_axis',(0.,0.,-1.));
#15946=DIRECTION('center_axis',(-1.,0.,0.));
#15947=DIRECTION('ref_axis',(0.,0.,1.));
#15948=DIRECTION('center_axis',(0.905882352941173,0.,0.423529411764713));
#15949=DIRECTION('ref_axis',(-0.423529411764713,0.,0.905882352941173));
#15950=DIRECTION('center_axis',(-0.905882352941173,0.,0.423529411764713));
#15951=DIRECTION('ref_axis',(-0.423529411764713,0.,-0.905882352941173));
#15952=DIRECTION('center_axis',(0.,1.,0.));
#15953=DIRECTION('ref_axis',(0.,0.,1.));
#15954=DIRECTION('center_axis',(0.423529411764713,0.,0.905882352941173));
#15955=DIRECTION('ref_axis',(0.905882352941173,0.,-0.423529411764713));
#15956=DIRECTION('center_axis',(-3.49148133884313E-15,0.,1.));
#15957=DIRECTION('ref_axis',(1.,0.,3.49148133884313E-15));
#15958=DIRECTION('center_axis',(0.,0.,1.));
#15959=DIRECTION('ref_axis',(1.,0.,0.));
#15960=DIRECTION('center_axis',(0.,0.,-1.));
#15961=DIRECTION('ref_axis',(-1.,0.,0.));
#15962=DIRECTION('center_axis',(0.,1.,0.));
#15963=DIRECTION('ref_axis',(0.,0.,1.));
#15964=DIRECTION('center_axis',(-0.423529411764713,0.,0.905882352941173));
#15965=DIRECTION('ref_axis',(0.905882352941173,0.,0.423529411764713));
#15966=DIRECTION('center_axis',(-0.423529411764713,0.,0.905882352941173));
#15967=DIRECTION('ref_axis',(-0.905882352941173,6.66133814775091E-14,-0.423529411764713));
#15968=DIRECTION('center_axis',(0.,0.,1.));
#15969=DIRECTION('ref_axis',(-1.,0.,0.));
#15970=DIRECTION('center_axis',(0.,1.,0.));
#15971=DIRECTION('ref_axis',(0.,0.,1.));
#15972=DIRECTION('center_axis',(0.,1.,0.));
#15973=DIRECTION('ref_axis',(0.,0.,1.));
#15974=DIRECTION('center_axis',(0.,1.,0.));
#15975=DIRECTION('ref_axis',(0.,0.,1.));
#15976=DIRECTION('center_axis',(-0.905882352941173,0.,0.423529411764713));
#15977=DIRECTION('ref_axis',(0.423529411764713,0.,0.905882352941173));
#15978=DIRECTION('center_axis',(0.,0.,-1.));
#15979=DIRECTION('ref_axis',(-1.,0.,0.));
#15980=DIRECTION('center_axis',(0.,0.,1.));
#15981=DIRECTION('ref_axis',(1.,0.,0.));
#15982=DIRECTION('center_axis',(0.0822611166581281,0.0232075739987885,0.996340562857524));
#15983=DIRECTION('ref_axis',(0.920256040566017,0.382000889613614,-0.0848772062226595));
#15984=DIRECTION('center_axis',(-1.,0.,0.));
#15985=DIRECTION('ref_axis',(0.,-1.56541446472147E-12,-1.));
#15986=DIRECTION('center_axis',(0.423529411764713,0.,0.905882352941173));
#15987=DIRECTION('ref_axis',(-0.905882352941173,4.44089209850061E-14,0.423529411764713));
#15988=DIRECTION('center_axis',(0.,1.,0.));
#15989=DIRECTION('ref_axis',(0.,0.,1.));
#15990=DIRECTION('center_axis',(0.,1.,0.));
#15991=DIRECTION('ref_axis',(0.,0.,1.));
#15992=DIRECTION('center_axis',(-1.,0.,0.));
#15993=DIRECTION('ref_axis',(0.,0.,1.));
#15994=DIRECTION('center_axis',(-1.,0.,0.));
#15995=DIRECTION('ref_axis',(0.,0.,1.));
#15996=DIRECTION('center_axis',(0.,1.,0.));
#15997=DIRECTION('ref_axis',(0.,0.,1.));
#15998=DIRECTION('center_axis',(0.905882352941173,0.,0.423529411764713));
#15999=DIRECTION('ref_axis',(0.423529411764713,0.,-0.905882352941173));
#16000=DIRECTION('center_axis',(0.997972229653585,-0.0634588605921735,0.00493982313395358));
#16001=DIRECTION('ref_axis',(-0.028904578164028,-0.382679269643752,0.923428991285244));
#16002=DIRECTION('center_axis',(0.,1.,0.));
#16003=DIRECTION('ref_axis',(0.,0.,1.));
#16004=DIRECTION('center_axis',(0.,0.,1.));
#16005=DIRECTION('ref_axis',(1.,0.,0.));
#16006=DIRECTION('center_axis',(-1.,0.,0.));
#16007=DIRECTION('ref_axis',(0.,0.,1.));
#16008=DIRECTION('center_axis',(-1.,0.,1.95461800110063E-16));
#16009=DIRECTION('ref_axis',(1.95461800110063E-16,0.,1.));
#16010=DIRECTION('center_axis',(-1.,0.,0.));
#16011=DIRECTION('ref_axis',(0.,0.,1.));
#16012=DIRECTION('center_axis',(3.29601953873307E-15,0.,-1.));
#16013=DIRECTION('ref_axis',(-1.,0.,-3.29601953873307E-15));
#16014=DIRECTION('center_axis',(0.,0.,1.));
#16015=DIRECTION('ref_axis',(-1.,0.,0.));
#16016=DIRECTION('center_axis',(0.,1.,0.));
#16017=DIRECTION('ref_axis',(0.,0.,1.));
#16018=DIRECTION('center_axis',(0.,0.,1.));
#16019=DIRECTION('ref_axis',(1.,0.,0.));
#16020=DIRECTION('center_axis',(0.,1.,0.));
#16021=DIRECTION('ref_axis',(0.,0.,1.));
#16022=DIRECTION('center_axis',(-1.,0.,0.));
#16023=DIRECTION('ref_axis',(0.,0.,1.));
#16024=DIRECTION('center_axis',(0.,0.,1.));
#16025=DIRECTION('ref_axis',(1.,0.,0.));
#16026=DIRECTION('center_axis',(0.,2.77555756156289E-14,1.));
#16027=DIRECTION('ref_axis',(0.,-1.,2.77555756156289E-14));
#16028=DIRECTION('center_axis',(1.,0.,-1.95461800110063E-16));
#16029=DIRECTION('ref_axis',(-1.95461800110063E-16,0.,-1.));
#16030=DIRECTION('center_axis',(-1.,0.,0.));
#16031=DIRECTION('ref_axis',(0.,0.,1.));
#16032=DIRECTION('center_axis',(0.,1.,0.));
#16033=DIRECTION('ref_axis',(0.,0.,1.));
#16034=DIRECTION('center_axis',(0.,1.,0.));
#16035=DIRECTION('ref_axis',(0.,0.,1.));
#16036=DIRECTION('center_axis',(0.,0.,1.));
#16037=DIRECTION('ref_axis',(1.,0.,0.));
#16038=DIRECTION('center_axis',(-1.,0.,0.));
#16039=DIRECTION('ref_axis',(0.,0.,1.));
#16040=DIRECTION('center_axis',(1.,0.,-1.95461800110063E-16));
#16041=DIRECTION('ref_axis',(-1.95461800110063E-16,0.,-1.));
#16042=DIRECTION('center_axis',(-1.,0.,0.));
#16043=DIRECTION('ref_axis',(0.,0.,1.));
#16044=DIRECTION('center_axis',(-3.29601953873307E-15,0.,1.));
#16045=DIRECTION('ref_axis',(1.,0.,3.29601953873307E-15));
#16046=DIRECTION('center_axis',(0.,0.,1.));
#16047=DIRECTION('ref_axis',(-1.,0.,0.));
#16048=DIRECTION('center_axis',(0.,1.,0.));
#16049=DIRECTION('ref_axis',(0.,0.,1.));
#16050=DIRECTION('center_axis',(0.,0.,1.));
#16051=DIRECTION('ref_axis',(1.,0.,0.));
#16052=DIRECTION('center_axis',(0.,1.,0.));
#16053=DIRECTION('ref_axis',(0.,0.,1.));
#16054=DIRECTION('center_axis',(-1.,0.,0.));
#16055=DIRECTION('ref_axis',(0.,0.,1.));
#16056=DIRECTION('center_axis',(0.,0.,-1.));
#16057=DIRECTION('ref_axis',(-1.,0.,0.));
#16058=DIRECTION('center_axis',(-2.77555756156289E-14,0.,1.));
#16059=DIRECTION('ref_axis',(1.,0.,2.77555756156289E-14));
#16060=DIRECTION('center_axis',(-1.,0.,1.95461800110063E-16));
#16061=DIRECTION('ref_axis',(1.95461800110063E-16,0.,1.));
#16062=DIRECTION('center_axis',(-1.,0.,0.));
#16063=DIRECTION('ref_axis',(0.,0.,1.));
#16064=DIRECTION('center_axis',(0.,1.,0.));
#16065=DIRECTION('ref_axis',(0.,0.,1.));
#16066=DIRECTION('center_axis',(0.,1.,0.));
#16067=DIRECTION('ref_axis',(-0.707106781186548,0.,-0.707106781186548));
#16068=DIRECTION('center_axis',(0.588235294117631,0.,0.80868982852163));
#16069=DIRECTION('ref_axis',(0.80868982852163,0.,-0.588235294117631));
#16070=DIRECTION('center_axis',(0.,1.,0.));
#16071=DIRECTION('ref_axis',(0.,0.,1.));
#16072=DIRECTION('center_axis',(-1.,0.,0.));
#16073=DIRECTION('ref_axis',(0.,0.,1.));
#16074=DIRECTION('center_axis',(0.,0.,1.));
#16075=DIRECTION('ref_axis',(1.,0.,0.));
#16076=DIRECTION('center_axis',(0.,0.,1.));
#16077=DIRECTION('ref_axis',(-1.,0.,0.));
#16078=DIRECTION('center_axis',(0.,0.,-1.));
#16079=DIRECTION('ref_axis',(-1.,0.,0.));
#16080=DIRECTION('center_axis',(-1.,0.,-1.03892784411108E-15));
#16081=DIRECTION('ref_axis',(-1.03892784411108E-15,0.,1.));
#16082=DIRECTION('center_axis',(-1.,0.,0.));
#16083=DIRECTION('ref_axis',(0.,0.,1.));
#16084=DIRECTION('center_axis',(0.,1.,0.));
#16085=DIRECTION('ref_axis',(0.27462518896381,0.,-0.961551353587832));
#16086=DIRECTION('center_axis',(-0.528132444354927,1.46586199943601E-14,
0.849162011173186));
#16087=DIRECTION('ref_axis',(0.849162011173186,-1.56277058526093E-29,0.528132444354927));
#16088=DIRECTION('center_axis',(0.,1.,0.));
#16089=DIRECTION('ref_axis',(0.,0.,1.));
#16090=DIRECTION('center_axis',(0.849162011173186,0.,-0.528132444354927));
#16091=DIRECTION('ref_axis',(-0.528132444354927,0.,-0.849162011173186));
#16092=DIRECTION('center_axis',(0.,1.,0.));
#16093=DIRECTION('ref_axis',(0.,0.,1.));
#16094=DIRECTION('center_axis',(0.,1.,0.));
#16095=DIRECTION('ref_axis',(-0.707106781186547,0.,-0.707106781186548));
#16096=DIRECTION('center_axis',(-0.588235294117645,0.,-0.808689828521621));
#16097=DIRECTION('ref_axis',(-0.808689828521621,0.,0.588235294117644));
#16098=DIRECTION('center_axis',(0.,1.,0.));
#16099=DIRECTION('ref_axis',(0.,0.,1.));
#16100=DIRECTION('center_axis',(1.,0.,0.));
#16101=DIRECTION('ref_axis',(0.,0.,-1.));
#16102=DIRECTION('center_axis',(0.,0.,-1.));
#16103=DIRECTION('ref_axis',(-1.,0.,0.));
#16104=DIRECTION('center_axis',(0.,0.,1.));
#16105=DIRECTION('ref_axis',(-1.,0.,0.));
#16106=DIRECTION('center_axis',(0.,0.,1.));
#16107=DIRECTION('ref_axis',(1.,0.,0.));
#16108=DIRECTION('center_axis',(1.,0.,1.03892784411108E-15));
#16109=DIRECTION('ref_axis',(1.03892784411108E-15,0.,-1.));
#16110=DIRECTION('center_axis',(1.,0.,0.));
#16111=DIRECTION('ref_axis',(0.,0.,-1.));
#16112=DIRECTION('center_axis',(0.,1.,0.));
#16113=DIRECTION('ref_axis',(0.274625188963811,0.,-0.961551353587832));
#16114=DIRECTION('center_axis',(0.528132444354927,0.,-0.849162011173186));
#16115=DIRECTION('ref_axis',(-0.849162011173186,0.,-0.528132444354927));
#16116=DIRECTION('center_axis',(0.,1.,0.));
#16117=DIRECTION('ref_axis',(0.,0.,1.));
#16118=DIRECTION('center_axis',(-0.849162011173186,0.,0.528132444354927));
#16119=DIRECTION('ref_axis',(0.528132444354927,0.,0.849162011173186));
#16120=DIRECTION('center_axis',(0.,1.,0.));
#16121=DIRECTION('ref_axis',(0.,0.,1.));
#16122=DIRECTION('center_axis',(0.,1.,0.));
#16123=DIRECTION('ref_axis',(0.,0.,1.));
#16124=DIRECTION('center_axis',(-1.,0.,0.));
#16125=DIRECTION('ref_axis',(0.,0.,1.));
#16126=DIRECTION('center_axis',(0.,1.,0.));
#16127=DIRECTION('ref_axis',(0.453742606486508,0.,-0.891132788679011));
#16128=DIRECTION('center_axis',(0.,0.,1.));
#16129=DIRECTION('ref_axis',(1.,0.,0.));
#16130=DIRECTION('center_axis',(1.,0.,3.49148133884313E-15));
#16131=DIRECTION('ref_axis',(3.49148133884313E-15,0.,-1.));
#16132=DIRECTION('center_axis',(-1.,0.,0.));
#16133=DIRECTION('ref_axis',(0.,0.,1.));
#16134=DIRECTION('center_axis',(-4.53040918295421E-15,0.,1.));
#16135=DIRECTION('ref_axis',(1.,0.,4.53040918295421E-15));
#16136=DIRECTION('center_axis',(0.,1.,0.));
#16137=DIRECTION('ref_axis',(0.,0.,1.));
#16138=DIRECTION('center_axis',(0.849162011173186,1.46586199943601E-14,
0.528132444354927));
#16139=DIRECTION('ref_axis',(0.528132444354927,-1.61399174840201E-29,-0.849162011173186));
#16140=DIRECTION('center_axis',(0.,1.,0.));
#16141=DIRECTION('ref_axis',(0.,0.,1.));
#16142=DIRECTION('center_axis',(0.,1.,0.));
#16143=DIRECTION('ref_axis',(0.,0.,1.));
#16144=DIRECTION('center_axis',(1.,0.,0.));
#16145=DIRECTION('ref_axis',(0.,0.,-1.));
#16146=DIRECTION('center_axis',(0.,1.,0.));
#16147=DIRECTION('ref_axis',(0.45374260648651,0.,-0.891132788679009));
#16148=DIRECTION('center_axis',(0.,0.,-1.));
#16149=DIRECTION('ref_axis',(-1.,0.,0.));
#16150=DIRECTION('center_axis',(-1.,0.,-3.49148133884313E-15));
#16151=DIRECTION('ref_axis',(-3.49148133884313E-15,0.,1.));
#16152=DIRECTION('center_axis',(1.,0.,0.));
#16153=DIRECTION('ref_axis',(0.,0.,-1.));
#16154=DIRECTION('center_axis',(4.53040918295421E-15,0.,-1.));
#16155=DIRECTION('ref_axis',(-1.,0.,-4.53040918295421E-15));
#16156=DIRECTION('center_axis',(0.,1.,0.));
#16157=DIRECTION('ref_axis',(0.,0.,1.));
#16158=DIRECTION('center_axis',(-0.849162011173186,0.,-0.528132444354927));
#16159=DIRECTION('ref_axis',(-0.528132444354927,0.,0.849162011173186));
#16160=DIRECTION('center_axis',(0.,1.,0.));
#16161=DIRECTION('ref_axis',(0.,0.,1.));
#16162=DIRECTION('center_axis',(0.,1.,0.));
#16163=DIRECTION('ref_axis',(-0.453742606486517,0.,-0.891132788679006));
#16164=DIRECTION('center_axis',(0.,0.,1.));
#16165=DIRECTION('ref_axis',(1.,0.,0.));
#16166=DIRECTION('center_axis',(0.,1.,0.));
#16167=DIRECTION('ref_axis',(0.,0.,1.));
#16168=DIRECTION('center_axis',(1.,0.,0.));
#16169=DIRECTION('ref_axis',(0.,0.,-1.));
#16170=DIRECTION('center_axis',(0.,0.,-1.));
#16171=DIRECTION('ref_axis',(-1.,0.,0.));
#16172=DIRECTION('center_axis',(1.,0.,1.03892784411108E-15));
#16173=DIRECTION('ref_axis',(1.03892784411108E-15,0.,-1.));
#16174=DIRECTION('center_axis',(1.,0.,0.));
#16175=DIRECTION('ref_axis',(0.,0.,-1.));
#16176=DIRECTION('center_axis',(0.,1.,0.));
#16177=DIRECTION('ref_axis',(0.,0.,1.));
#16178=DIRECTION('center_axis',(-0.849162011173186,0.,0.528132444354927));
#16179=DIRECTION('ref_axis',(0.528132444354927,0.,0.849162011173186));
#16180=DIRECTION('center_axis',(0.,1.,0.));
#16181=DIRECTION('ref_axis',(0.,0.,1.));
#16182=DIRECTION('center_axis',(0.,1.,0.));
#16183=DIRECTION('ref_axis',(-0.45374260648651,0.,-0.891132788679009));
#16184=DIRECTION('center_axis',(0.,0.,-1.));
#16185=DIRECTION('ref_axis',(-1.,0.,0.));
#16186=DIRECTION('center_axis',(0.,1.,0.));
#16187=DIRECTION('ref_axis',(0.,0.,1.));
#16188=DIRECTION('center_axis',(-1.,0.,0.));
#16189=DIRECTION('ref_axis',(0.,0.,1.));
#16190=DIRECTION('center_axis',(0.,0.,1.));
#16191=DIRECTION('ref_axis',(1.,0.,0.));
#16192=DIRECTION('center_axis',(-1.,0.,-1.03892784411108E-15));
#16193=DIRECTION('ref_axis',(-1.03892784411108E-15,0.,1.));
#16194=DIRECTION('center_axis',(-1.,0.,0.));
#16195=DIRECTION('ref_axis',(0.,0.,1.));
#16196=DIRECTION('center_axis',(0.,1.,0.));
#16197=DIRECTION('ref_axis',(0.,0.,1.));
#16198=DIRECTION('center_axis',(0.849162011173186,0.,-0.528132444354927));
#16199=DIRECTION('ref_axis',(-0.528132444354927,0.,-0.849162011173186));
#16200=DIRECTION('center_axis',(0.,1.,0.));
#16201=DIRECTION('ref_axis',(0.,0.,1.));
#16202=DIRECTION('center_axis',(0.,1.,0.));
#16203=DIRECTION('ref_axis',(-0.0332934199937196,0.,-0.999445620424204));
#16204=DIRECTION('',(0.,1.,0.));
#16205=DIRECTION('',(0.,1.,0.));
#16206=DIRECTION('center_axis',(0.313163806483743,0.,-0.949699126201879));
#16207=DIRECTION('ref_axis',(-0.949699126201879,0.,-0.313163806483743));
#16208=DIRECTION('',(0.,-1.,0.));
#16209=DIRECTION('',(0.,1.,0.));
#16210=DIRECTION('center_axis',(0.313163806483743,0.,-0.949699126201879));
#16211=DIRECTION('ref_axis',(-0.949699126201879,0.,-0.313163806483743));
#16212=DIRECTION('',(0.,1.,0.));
#16213=DIRECTION('',(0.,1.,0.));
#16214=DIRECTION('',(-0.949699126201879,0.,-0.313163806483743));
#16215=DIRECTION('',(0.,-1.,0.));
#16216=DIRECTION('center_axis',(0.,1.,0.));
#16217=DIRECTION('ref_axis',(0.,0.,1.));
#16218=DIRECTION('center_axis',(0.,1.,0.));
#16219=DIRECTION('ref_axis',(0.,0.,1.));
#16220=DIRECTION('center_axis',(0.,1.,0.));
#16221=DIRECTION('ref_axis',(0.,0.,1.));
#16222=DIRECTION('center_axis',(0.,1.,0.));
#16223=DIRECTION('ref_axis',(0.,0.,1.));
#16224=DIRECTION('center_axis',(0.949699126201879,0.,0.313163806483743));
#16225=DIRECTION('ref_axis',(0.313163806483743,0.,-0.949699126201879));
#16226=DIRECTION('',(0.,-1.,0.));
#16227=DIRECTION('',(0.313163806483748,0.,-0.949699126201877));
#16228=DIRECTION('center_axis',(-0.949699126201879,0.,-0.313163806483743));
#16229=DIRECTION('ref_axis',(-0.313163806483743,0.,0.949699126201879));
#16230=DIRECTION('center_axis',(1.,0.,0.));
#16231=DIRECTION('ref_axis',(0.,0.,-1.));
#16232=DIRECTION('',(0.,-1.,0.));
#16233=DIRECTION('',(0.,-1.,0.));
#16234=DIRECTION('center_axis',(0.313163806483743,0.,-0.949699126201879));
#16235=DIRECTION('ref_axis',(-0.949699126201879,0.,-0.313163806483743));
#16236=DIRECTION('',(0.,-1.,0.));
#16237=DIRECTION('',(0.949699126201879,0.,0.313163806483743));
#16238=DIRECTION('center_axis',(0.,-1.,0.));
#16239=DIRECTION('ref_axis',(0.,0.,-1.));
#16240=DIRECTION('',(0.313163806483745,0.,-0.949699126201879));
#16241=DIRECTION('center_axis',(0.,0.,-1.));
#16242=DIRECTION('ref_axis',(-1.,0.,0.));
#16243=DIRECTION('',(0.,-1.,0.));
#16244=DIRECTION('center_axis',(-1.,0.,3.46944695195362E-15));
#16245=DIRECTION('ref_axis',(3.46944695195362E-15,0.,1.));
#16246=DIRECTION('',(0.,-1.,0.));
#16247=DIRECTION('center_axis',(-1.,0.,3.46944695195362E-15));
#16248=DIRECTION('ref_axis',(3.46944695195362E-15,0.,1.));
#16249=DIRECTION('',(0.,-1.,0.));
#16250=DIRECTION('center_axis',(0.,0.,-1.));
#16251=DIRECTION('ref_axis',(-1.,0.,0.));
#16252=DIRECTION('center_axis',(0.,0.,-1.));
#16253=DIRECTION('ref_axis',(-1.,0.,0.));
#16254=DIRECTION('center_axis',(0.,0.,-1.));
#16255=DIRECTION('ref_axis',(-1.,0.,0.));
#16256=DIRECTION('',(0.,-1.,0.));
#16257=DIRECTION('center_axis',(-1.,0.,3.46944695195362E-15));
#16258=DIRECTION('ref_axis',(3.46944695195362E-15,0.,1.));
#16259=DIRECTION('',(0.,-1.,0.));
#16260=DIRECTION('center_axis',(0.,0.,-1.));
#16261=DIRECTION('ref_axis',(-1.,0.,0.));
#16262=DIRECTION('',(0.,-1.,0.));
#16263=DIRECTION('center_axis',(0.,0.,-1.));
#16264=DIRECTION('ref_axis',(-1.,0.,0.));
#16265=DIRECTION('',(0.,-1.,0.));
#16266=DIRECTION('center_axis',(-1.,0.,3.46944695195362E-15));
#16267=DIRECTION('ref_axis',(3.46944695195362E-15,0.,1.));
#16268=DIRECTION('',(0.,-1.,0.));
#16269=DIRECTION('center_axis',(0.,0.,-1.));
#16270=DIRECTION('ref_axis',(-1.,0.,0.));
#16271=DIRECTION('',(0.,-1.,0.));
#16272=DIRECTION('center_axis',(-1.,0.,3.46944695195362E-15));
#16273=DIRECTION('ref_axis',(3.46944695195362E-15,0.,1.));
#16274=DIRECTION('center_axis',(-0.949699126201879,0.,-0.313163806483745));
#16275=DIRECTION('ref_axis',(-0.313163806483745,0.,0.949699126201879));
#16374=CARTESIAN_POINT('',(0.,0.,0.));
#16375=CARTESIAN_POINT('Origin',(0.0835265683620477,-15.7044045823054,0.0824317919394229));
#16376=CARTESIAN_POINT('',(0.0835265683620474,-14.7669045823054,-2.10506820806058));
#16377=CARTESIAN_POINT('Origin',(0.0835265683620477,-14.7669045823054,0.0824317919394229));
#16378=CARTESIAN_POINT('',(0.0835265683620474,-14.4544045823054,-2.10506820806058));
#16379=CARTESIAN_POINT('',(0.0835265683620474,-15.7044045823054,-2.10506820806058));
#16380=CARTESIAN_POINT('Origin',(0.0835265683620477,-14.4544045823054,0.0824317919394229));
#16381=CARTESIAN_POINT('Origin',(0.0835265683620477,-22.3021228236204,0.0824317919394229));
#16382=CARTESIAN_POINT('',(0.0835265683620474,-11.3294045823054,-2.48006820806058));
#16383=CARTESIAN_POINT('Origin',(0.0835265683620477,-11.3294045823054,0.0824317919394229));
#16384=CARTESIAN_POINT('',(0.0835265683620474,-10.0794045823054,-2.48006820806058));
#16385=CARTESIAN_POINT('',(0.0835265683620474,-22.3021228236204,-2.48006820806058));
#16386=CARTESIAN_POINT('Origin',(0.0835265683620477,-10.0794045823054,0.0824317919394229));
#16387=CARTESIAN_POINT('Origin',(0.0835265683620477,-22.3021228236204,0.0824317919394229));
#16388=CARTESIAN_POINT('',(0.0835265683620473,-10.0794045823054,-3.35506820806058));
#16389=CARTESIAN_POINT('Origin',(0.0835265683620477,-10.0794045823054,0.0824317919394229));
#16390=CARTESIAN_POINT('',(0.0835265683620473,-12.5794045823054,-3.35506820806058));
#16391=CARTESIAN_POINT('',(0.0835265683620473,-22.3021228236204,-3.35506820806058));
#16392=CARTESIAN_POINT('Origin',(0.0835265683620477,-12.5794045823054,0.0824317919394229));
#16393=CARTESIAN_POINT('Origin',(0.0835265683620477,-17.1192738307565,0.0824317919394229));
#16394=CARTESIAN_POINT('',(0.0835265683620475,-14.4544045823054,-1.23006820806058));
#16395=CARTESIAN_POINT('Origin',(0.0835265683620477,-14.4544045823054,0.0824317919394229));
#16396=CARTESIAN_POINT('',(0.0835265683620475,-11.3294045823054,-1.23006820806058));
#16397=CARTESIAN_POINT('',(0.0835265683620475,-17.1192738307565,-1.23006820806058));
#16398=CARTESIAN_POINT('Origin',(0.0835265683620477,-11.3294045823054,0.0824317919394229));
#16399=CARTESIAN_POINT('Origin',(-44.291473431638,16.1705954176946,-44.2925682080606));
#16400=CARTESIAN_POINT('',(-44.291473431638,16.1705954176946,-41.4800682080606));
#16401=CARTESIAN_POINT('',(-44.291473431638,16.1705954176946,-47.1050682080606));
#16402=CARTESIAN_POINT('Origin',(-44.291473431638,16.1705954176946,-44.2925682080606));
#16403=CARTESIAN_POINT('Origin',(-44.291473431638,16.1705954176946,-44.2925682080606));
#16404=CARTESIAN_POINT('',(-44.291473431638,16.4830954176946,-47.4175682080606));
#16405=CARTESIAN_POINT('Origin',(-44.291473431638,16.1705954176946,-47.4175682080606));
#16406=CARTESIAN_POINT('Origin',(-44.291473431638,16.4830954176946,-44.2925682080606));
#16407=CARTESIAN_POINT('Origin',(-44.291473431638,-14.4544045823054,-44.2925682080606));
#16408=CARTESIAN_POINT('',(-44.291473431638,-14.7669045823054,-47.4175682080606));
#16409=CARTESIAN_POINT('Origin',(-44.291473431638,-14.7669045823054,-44.2925682080606));
#16410=CARTESIAN_POINT('',(-44.291473431638,-14.4544045823054,-47.1050682080606));
#16411=CARTESIAN_POINT('Origin',(-44.291473431638,-14.4544045823054,-47.4175682080606));
#16412=CARTESIAN_POINT('',(-44.291473431638,-14.4544045823054,-41.4800682080606));
#16413=CARTESIAN_POINT('Origin',(-44.291473431638,-14.4544045823054,-44.2925682080606));
#16414=CARTESIAN_POINT('Origin',(-44.291473431638,-14.4544045823054,-44.2925682080606));
#16415=CARTESIAN_POINT('Origin',(-44.291473431638,-8.87385981233827,-44.2925682080606));
#16416=CARTESIAN_POINT('',(-44.291473431638,-8.56135981233827,-41.1675682080606));
#16417=CARTESIAN_POINT('Origin',(-44.291473431638,-8.56135981233827,-44.2925682080606));
#16418=CARTESIAN_POINT('',(-44.291473431638,-8.87385981233827,-41.4800682080606));
#16419=CARTESIAN_POINT('Origin',(-44.291473431638,-8.87385981233827,-41.1675682080606));
#16420=CARTESIAN_POINT('Origin',(-44.291473431638,-8.87385981233827,-44.2925682080606));
#16421=CARTESIAN_POINT('Origin',(-44.291473431638,13.4386401876617,-44.2925682080606));
#16422=CARTESIAN_POINT('',(-44.291473431638,13.1261401876617,-47.4175682080606));
#16423=CARTESIAN_POINT('Origin',(-44.291473431638,13.1261401876617,-44.2925682080606));
#16424=CARTESIAN_POINT('',(-44.291473431638,13.4386401876617,-47.1050682080606));
#16425=CARTESIAN_POINT('Origin',(-44.291473431638,13.4386401876617,-47.4175682080606));
#16426=CARTESIAN_POINT('',(-44.291473431638,13.4386401876617,-41.4800682080606));
#16427=CARTESIAN_POINT('Origin',(-44.291473431638,13.4386401876617,-44.2925682080606));
#16428=CARTESIAN_POINT('Origin',(-44.291473431638,13.4386401876617,-44.2925682080606));
#16429=CARTESIAN_POINT('Origin',(-47.4164734316379,15.8580954176946,-29.4599768141645));
#16430=CARTESIAN_POINT('',(-48.0414734316379,15.5455954176946,-29.4599768141645));
#16431=CARTESIAN_POINT('',(-46.8857471746547,15.5455954176946,-29.1298940364426));
#16432=CARTESIAN_POINT('Origin',(-47.4164734316379,15.5455954176946,-29.4599768141645));
#16433=CARTESIAN_POINT('',(-48.3539734316379,15.8580954176946,-29.4599768141645));
#16434=CARTESIAN_POINT('Origin',(-48.0414734316379,15.8580954176946,-29.4599768141645));
#16435=CARTESIAN_POINT('',(-46.6203840461631,15.8580954176946,-28.9648526475817));
#16436=CARTESIAN_POINT('Origin',(-47.4164734316379,15.8580954176946,-29.4599768141645));
#16437=CARTESIAN_POINT('Origin',(-46.8857471746547,15.8580954176946,-29.1298940364426));
#16438=CARTESIAN_POINT('Origin',(-44.291473431638,15.8580954176946,-44.2925682080606));
#16439=CARTESIAN_POINT('',(-46.8650028434027,15.8580954176946,-40.7545502082785));
#16440=CARTESIAN_POINT('',(-40.7534554318559,15.8580954176946,-46.8660976198253));
#16441=CARTESIAN_POINT('Origin',(-44.291473431638,15.8580954176946,-44.2925682080606));
#16442=CARTESIAN_POINT('',(-47.0488263728144,15.5455954176946,-40.5018346368655));
#16443=CARTESIAN_POINT('Origin',(-47.0488263728144,15.8580954176946,-40.5018346368655));
#16444=CARTESIAN_POINT('',(-40.5007398604429,15.5455954176946,-47.049921149237));
#16445=CARTESIAN_POINT('Origin',(-44.291473431638,15.5455954176946,-44.2925682080606));
#16446=CARTESIAN_POINT('Origin',(-40.5007398604429,15.8580954176946,-47.049921149237));
#16447=CARTESIAN_POINT('Origin',(-47.4164734316379,16.1705954176946,-29.4599768141645));
#16448=CARTESIAN_POINT('',(-46.3550209176715,16.4830954176946,-28.7998112587208));
#16449=CARTESIAN_POINT('',(-48.6664734316379,16.4830954176946,-29.4599768141645));
#16450=CARTESIAN_POINT('Origin',(-47.4164734316379,16.4830954176946,-29.4599768141645));
#16451=CARTESIAN_POINT('',(-46.6203840461631,16.1705954176946,-28.9648526475817));
#16452=CARTESIAN_POINT('Origin',(-46.3550209176715,16.1705954176946,-28.7998112587208));
#16453=CARTESIAN_POINT('',(-48.3539734316379,16.1705954176946,-29.4599768141645));
#16454=CARTESIAN_POINT('Origin',(-47.4164734316379,16.1705954176946,-29.4599768141645));
#16455=CARTESIAN_POINT('Origin',(-48.6664734316379,16.1705954176946,-29.4599768141645));
#16456=CARTESIAN_POINT('Origin',(-44.291473431638,16.1705954176946,-44.2925682080606));
#16457=CARTESIAN_POINT('',(-40.7534554318559,16.1705954176946,-46.8660976198253));
#16458=CARTESIAN_POINT('',(-46.8650028434027,16.1705954176946,-40.7545502082785));
#16459=CARTESIAN_POINT('Origin',(-44.291473431638,16.1705954176946,-44.2925682080606));
#16460=CARTESIAN_POINT('',(-41.0061710032689,16.4830954176946,-46.6822740904135));
#16461=CARTESIAN_POINT('Origin',(-41.0061710032689,16.1705954176946,-46.6822740904135));
#16462=CARTESIAN_POINT('',(-46.6811793139909,16.4830954176946,-41.0072657796915));
#16463=CARTESIAN_POINT('Origin',(-44.291473431638,16.4830954176946,-44.2925682080606));
#16464=CARTESIAN_POINT('Origin',(-46.6811793139909,16.1705954176946,-41.0072657796915));
#16465=CARTESIAN_POINT('Origin',(44.4585265683622,16.1705954176946,-44.2925682080604));
#16466=CARTESIAN_POINT('',(41.6460265683622,16.1705954176946,-44.2925682080604));
#16467=CARTESIAN_POINT('',(44.4585265683622,16.1705954176946,-47.1050682080604));
#16468=CARTESIAN_POINT('Origin',(44.4585265683622,16.1705954176946,-44.2925682080604));
#16469=CARTESIAN_POINT('Origin',(44.4585265683622,16.1705954176946,-44.2925682080604));
#16470=CARTESIAN_POINT('',(44.4585265683622,16.4830954176946,-47.4175682080604));
#16471=CARTESIAN_POINT('Origin',(44.4585265683622,16.1705954176946,-47.4175682080604));
#16472=CARTESIAN_POINT('Origin',(44.4585265683622,16.4830954176946,-44.2925682080604));
#16473=CARTESIAN_POINT('Origin',(44.4585265683622,-14.4544045823054,-44.2925682080604));
#16474=CARTESIAN_POINT('',(44.4585265683622,-14.7669045823054,-47.4175682080604));
#16475=CARTESIAN_POINT('Origin',(44.4585265683622,-14.7669045823054,-44.2925682080604));
#16476=CARTESIAN_POINT('',(44.4585265683622,-14.4544045823054,-47.1050682080604));
#16477=CARTESIAN_POINT('Origin',(44.4585265683622,-14.4544045823054,-47.4175682080604));
#16478=CARTESIAN_POINT('',(41.6460265683622,-14.4544045823054,-44.2925682080604));
#16479=CARTESIAN_POINT('Origin',(44.4585265683622,-14.4544045823054,-44.2925682080604));
#16480=CARTESIAN_POINT('Origin',(44.4585265683622,-14.4544045823054,-44.2925682080604));
#16481=CARTESIAN_POINT('Origin',(44.4585265683622,-8.87385981233827,-44.2925682080604));
#16482=CARTESIAN_POINT('',(44.4585265683622,-8.56135981233827,-41.1675682080604));
#16483=CARTESIAN_POINT('Origin',(44.4585265683622,-8.56135981233827,-44.2925682080604));
#16484=CARTESIAN_POINT('',(44.4585265683622,-8.87385981233827,-41.4800682080604));
#16485=CARTESIAN_POINT('Origin',(44.4585265683622,-8.87385981233827,-41.1675682080604));
#16486=CARTESIAN_POINT('',(41.6460265683622,-8.87385981233827,-44.2925682080604));
#16487=CARTESIAN_POINT('Origin',(44.4585265683622,-8.87385981233827,-44.2925682080604));
#16488=CARTESIAN_POINT('Origin',(44.4585265683622,-8.87385981233827,-44.2925682080604));
#16489=CARTESIAN_POINT('Origin',(44.4585265683622,13.4386401876617,-44.2925682080604));
#16490=CARTESIAN_POINT('',(44.4585265683622,13.1261401876617,-47.4175682080604));
#16491=CARTESIAN_POINT('Origin',(44.4585265683622,13.1261401876617,-44.2925682080604));
#16492=CARTESIAN_POINT('',(44.4585265683622,13.4386401876617,-47.1050682080604));
#16493=CARTESIAN_POINT('Origin',(44.4585265683622,13.4386401876617,-47.4175682080604));
#16494=CARTESIAN_POINT('',(41.6460265683622,13.4386401876617,-44.2925682080604));
#16495=CARTESIAN_POINT('Origin',(44.4585265683622,13.4386401876617,-44.2925682080604));
#16496=CARTESIAN_POINT('Origin',(44.4585265683622,13.4386401876617,-44.2925682080604));
#16497=CARTESIAN_POINT('Origin',(47.5835265683621,15.8580954176946,-29.4599768141643));
#16498=CARTESIAN_POINT('',(47.0528003113789,15.5455954176946,-29.1298940364425));
#16499=CARTESIAN_POINT('',(48.2085265683621,15.5455954176946,-29.4599768141643));
#16500=CARTESIAN_POINT('Origin',(47.5835265683621,15.5455954176946,-29.4599768141643));
#16501=CARTESIAN_POINT('',(46.7874371828873,15.8580954176946,-28.9648526475816));
#16502=CARTESIAN_POINT('Origin',(47.0528003113789,15.8580954176946,-29.1298940364425));
#16503=CARTESIAN_POINT('',(48.5210265683621,15.8580954176946,-29.4599768141643));
#16504=CARTESIAN_POINT('Origin',(47.5835265683621,15.8580954176946,-29.4599768141643));
#16505=CARTESIAN_POINT('Origin',(48.2085265683621,15.8580954176946,-29.4599768141643));
#16506=CARTESIAN_POINT('Origin',(44.4585265683622,15.8580954176946,-44.2925682080604));
#16507=CARTESIAN_POINT('',(40.9205085685801,15.8580954176946,-46.8660976198251));
#16508=CARTESIAN_POINT('',(47.0320559801269,15.8580954176946,-40.7545502082783));
#16509=CARTESIAN_POINT('Origin',(44.4585265683622,15.8580954176946,-44.2925682080604));
#16510=CARTESIAN_POINT('',(40.6677929971671,15.5455954176946,-47.0499211492369));
#16511=CARTESIAN_POINT('Origin',(40.6677929971671,15.8580954176946,-47.0499211492369));
#16512=CARTESIAN_POINT('',(47.2158795095386,15.5455954176946,-40.5018346368653));
#16513=CARTESIAN_POINT('Origin',(44.4585265683622,15.5455954176946,-44.2925682080604));
#16514=CARTESIAN_POINT('Origin',(47.2158795095386,15.8580954176946,-40.5018346368653));
#16515=CARTESIAN_POINT('Origin',(47.5835265683621,16.1705954176946,-29.4599768141643));
#16516=CARTESIAN_POINT('',(48.8335265683621,16.4830954176946,-29.4599768141643));
#16517=CARTESIAN_POINT('',(46.5220740543957,16.4830954176946,-28.7998112587207));
#16518=CARTESIAN_POINT('Origin',(47.5835265683621,16.4830954176946,-29.4599768141643));
#16519=CARTESIAN_POINT('',(48.5210265683621,16.1705954176946,-29.4599768141643));
#16520=CARTESIAN_POINT('Origin',(48.8335265683621,16.1705954176946,-29.4599768141643));
#16521=CARTESIAN_POINT('',(46.7874371828873,16.1705954176946,-28.9648526475816));
#16522=CARTESIAN_POINT('Origin',(47.5835265683621,16.1705954176946,-29.4599768141643));
#16523=CARTESIAN_POINT('Origin',(46.5220740543957,16.1705954176946,-28.7998112587207));
#16524=CARTESIAN_POINT('Origin',(44.4585265683622,16.1705954176946,-44.2925682080604));
#16525=CARTESIAN_POINT('',(47.0320559801269,16.1705954176946,-40.7545502082783));
#16526=CARTESIAN_POINT('',(40.9205085685801,16.1705954176946,-46.8660976198251));
#16527=CARTESIAN_POINT('Origin',(44.4585265683622,16.1705954176946,-44.2925682080604));
#16528=CARTESIAN_POINT('',(46.8482324507151,16.4830954176946,-41.0072657796913));
#16529=CARTESIAN_POINT('Origin',(46.8482324507151,16.1705954176946,-41.0072657796913));
#16530=CARTESIAN_POINT('',(41.1732241399931,16.4830954176946,-46.6822740904134));
#16531=CARTESIAN_POINT('Origin',(44.4585265683622,16.4830954176946,-44.2925682080604));
#16532=CARTESIAN_POINT('Origin',(41.1732241399931,16.1705954176946,-46.6822740904134));
#16533=CARTESIAN_POINT('Origin',(44.4585265683621,16.1705954176946,44.4574317919394));
#16534=CARTESIAN_POINT('',(44.4585265683621,16.1705954176946,41.6449317919394));
#16535=CARTESIAN_POINT('Origin',(44.4585265683621,16.1705954176946,44.4574317919394));
#16536=CARTESIAN_POINT('',(44.4585265683621,16.4830954176946,41.3324317919394));
#16537=CARTESIAN_POINT('Origin',(44.4585265683621,16.1705954176946,41.3324317919394));
#16538=CARTESIAN_POINT('Origin',(44.4585265683621,16.4830954176946,44.4574317919394));
#16539=CARTESIAN_POINT('Origin',(44.4585265683621,-14.4544045823054,44.4574317919394));
#16540=CARTESIAN_POINT('',(44.4585265683621,-14.7669045823054,41.3324317919394));
#16541=CARTESIAN_POINT('Origin',(44.4585265683621,-14.7669045823054,44.4574317919394));
#16542=CARTESIAN_POINT('',(44.4585265683621,-14.4544045823054,41.6449317919394));
#16543=CARTESIAN_POINT('Origin',(44.4585265683621,-14.4544045823054,41.3324317919394));
#16544=CARTESIAN_POINT('Origin',(44.4585265683621,-14.4544045823054,44.4574317919394));
#16545=CARTESIAN_POINT('Origin',(44.4585265683621,-8.87385981233827,44.4574317919394));
#16546=CARTESIAN_POINT('',(44.4585265683621,-8.56135981233827,47.5824317919394));
#16547=CARTESIAN_POINT('Origin',(44.4585265683621,-8.56135981233827,44.4574317919394));
#16548=CARTESIAN_POINT('',(44.4585265683621,-8.87385981233827,47.2699317919394));
#16549=CARTESIAN_POINT('Origin',(44.4585265683621,-8.87385981233827,47.5824317919394));
#16550=CARTESIAN_POINT('',(44.4585265683621,-8.87385981233827,41.6449317919394));
#16551=CARTESIAN_POINT('Origin',(44.4585265683621,-8.87385981233827,44.4574317919394));
#16552=CARTESIAN_POINT('Origin',(44.4585265683621,-8.87385981233827,44.4574317919394));
#16553=CARTESIAN_POINT('Origin',(44.4585265683621,13.4386401876617,44.4574317919394));
#16554=CARTESIAN_POINT('',(44.4585265683621,13.1261401876617,41.3324317919394));
#16555=CARTESIAN_POINT('Origin',(44.4585265683621,13.1261401876617,44.4574317919394));
#16556=CARTESIAN_POINT('',(44.4585265683621,13.4386401876617,41.6449317919394));
#16557=CARTESIAN_POINT('Origin',(44.4585265683621,13.4386401876617,41.3324317919394));
#16558=CARTESIAN_POINT('Origin',(44.4585265683621,13.4386401876617,44.4574317919394));
#16559=CARTESIAN_POINT('Origin',(47.583526568362,15.8580954176946,40.1612670779183));
#16560=CARTESIAN_POINT('',(47.2158795095385,15.5455954176946,40.6666982207443));
#16561=CARTESIAN_POINT('',(48.2085265683621,15.5455954176946,40.1612670779183));
#16562=CARTESIAN_POINT('Origin',(47.583526568362,15.5455954176946,40.1612670779183));
#16563=CARTESIAN_POINT('',(47.0320559801268,15.8580954176946,40.9194137921573));
#16564=CARTESIAN_POINT('Origin',(47.2158795095385,15.8580954176946,40.6666982207443));
#16565=CARTESIAN_POINT('',(48.5210265683621,15.8580954176946,40.1612670779183));
#16566=CARTESIAN_POINT('Origin',(47.583526568362,15.8580954176946,40.1612670779183));
#16567=CARTESIAN_POINT('Origin',(48.2085265683621,15.8580954176946,40.1612670779183));
#16568=CARTESIAN_POINT('Origin',(47.583526568362,16.1705954176946,40.1612670779183));
#16569=CARTESIAN_POINT('',(48.8335265683621,16.4830954176946,40.1612670779183));
#16570=CARTESIAN_POINT('',(46.848232450715,16.4830954176946,41.1721293635703));
#16571=CARTESIAN_POINT('Origin',(47.583526568362,16.4830954176946,40.1612670779183));
#16572=CARTESIAN_POINT('',(48.5210265683621,16.1705954176946,40.1612670779183));
#16573=CARTESIAN_POINT('Origin',(48.8335265683621,16.1705954176946,40.1612670779183));
#16574=CARTESIAN_POINT('',(47.0320559801268,16.1705954176946,40.9194137921573));
#16575=CARTESIAN_POINT('Origin',(47.583526568362,16.1705954176946,40.1612670779183));
#16576=CARTESIAN_POINT('Origin',(46.848232450715,16.1705954176946,41.1721293635703));
#16577=CARTESIAN_POINT('Origin',(-44.2914734316384,16.1705954176946,44.457431791939));
#16578=CARTESIAN_POINT('',(-44.2914734316384,16.1705954176946,41.644931791939));
#16579=CARTESIAN_POINT('',(-41.4789734316384,16.1705954176946,44.457431791939));
#16580=CARTESIAN_POINT('Origin',(-44.2914734316384,16.1705954176946,44.457431791939));
#16581=CARTESIAN_POINT('',(-44.2914734316384,16.4830954176946,41.332431791939));
#16582=CARTESIAN_POINT('Origin',(-44.2914734316384,16.1705954176946,41.332431791939));
#16583=CARTESIAN_POINT('Origin',(-44.2914734316384,16.4830954176946,44.457431791939));
#16584=CARTESIAN_POINT('Origin',(-44.2914734316384,16.1705954176946,44.457431791939));
#16585=CARTESIAN_POINT('Origin',(-44.2914734316384,-14.4544045823054,44.457431791939));
#16586=CARTESIAN_POINT('',(-44.2914734316384,-14.7669045823054,41.332431791939));
#16587=CARTESIAN_POINT('Origin',(-44.2914734316384,-14.7669045823054,44.457431791939));
#16588=CARTESIAN_POINT('',(-44.2914734316384,-14.4544045823054,41.644931791939));
#16589=CARTESIAN_POINT('Origin',(-44.2914734316384,-14.4544045823054,41.332431791939));
#16590=CARTESIAN_POINT('',(-41.4789734316384,-14.4544045823054,44.457431791939));
#16591=CARTESIAN_POINT('Origin',(-44.2914734316384,-14.4544045823054,44.457431791939));
#16592=CARTESIAN_POINT('Origin',(-44.2914734316384,-14.4544045823054,44.457431791939));
#16593=CARTESIAN_POINT('Origin',(-44.2914734316384,-8.87385981233827,44.457431791939));
#16594=CARTESIAN_POINT('',(-44.2914734316384,-8.56135981233827,47.582431791939));
#16595=CARTESIAN_POINT('Origin',(-44.2914734316384,-8.56135981233827,44.457431791939));
#16596=CARTESIAN_POINT('',(-44.2914734316384,-8.87385981233827,47.269931791939));
#16597=CARTESIAN_POINT('Origin',(-44.2914734316384,-8.87385981233827,47.582431791939));
#16598=CARTESIAN_POINT('',(-41.4789734316384,-8.87385981233827,44.457431791939));
#16599=CARTESIAN_POINT('Origin',(-44.2914734316384,-8.87385981233827,44.457431791939));
#16600=CARTESIAN_POINT('Origin',(-44.2914734316384,-8.87385981233827,44.457431791939));
#16601=CARTESIAN_POINT('Origin',(-44.2914734316384,13.4386401876617,44.457431791939));
#16602=CARTESIAN_POINT('',(-44.2914734316384,13.1261401876617,41.332431791939));
#16603=CARTESIAN_POINT('Origin',(-44.2914734316384,13.1261401876617,44.457431791939));
#16604=CARTESIAN_POINT('',(-44.2914734316384,13.4386401876617,41.644931791939));
#16605=CARTESIAN_POINT('Origin',(-44.2914734316384,13.4386401876617,41.332431791939));
#16606=CARTESIAN_POINT('',(-41.4789734316384,13.4386401876617,44.457431791939));
#16607=CARTESIAN_POINT('Origin',(-44.2914734316384,13.4386401876617,44.457431791939));
#16608=CARTESIAN_POINT('Origin',(-44.2914734316384,13.4386401876617,44.457431791939));
#16609=CARTESIAN_POINT('Origin',(0.0835265683620477,-3.61941807409668,0.0824317919394229));
#16610=CARTESIAN_POINT('',(-34.1615012109487,-3.61941807409668,36.0841779807597));
#16611=CARTESIAN_POINT('',(34.3285543476724,-3.61941807409668,36.0841779807601));
#16612=CARTESIAN_POINT('Origin',(0.0835265683620477,-3.61941807409668,0.0824317919394229));
#16613=CARTESIAN_POINT('',(-34.2245838299087,-3.84038894321748,36.1504966431758));
#16614=CARTESIAN_POINT('Origin',(-34.3768787441519,-3.61941807409668,36.310604057419));
#16615=CARTESIAN_POINT('',(34.3916369666324,-3.84038894321748,36.1504966431761));
#16616=CARTESIAN_POINT('Origin',(0.0835265683620477,-3.84038894321747,0.0824317919394229));
#16617=CARTESIAN_POINT('Origin',(34.5439318808756,-3.61941807409668,36.3106040574193));
#16618=CARTESIAN_POINT('Origin',(0.0835265683620477,11.9341984494201,0.0824317919394229));
#16619=CARTESIAN_POINT('',(-34.2245838299085,12.155169318541,36.1504966431761));
#16620=CARTESIAN_POINT('',(34.3916369666327,12.1551693185413,36.1504966431763));
#16621=CARTESIAN_POINT('Origin',(0.0835265683620477,12.1551693185409,0.0824317919394229));
#16622=CARTESIAN_POINT('',(-34.1615012109487,11.9341984494201,36.0841779807597));
#16623=CARTESIAN_POINT('Origin',(-34.3768787441519,11.9341984494201,36.310604057419));
#16624=CARTESIAN_POINT('',(34.3285543476724,11.9341984494201,36.0841779807601));
#16625=CARTESIAN_POINT('Origin',(0.0835265683620477,11.9341984494201,0.0824317919394229));
#16626=CARTESIAN_POINT('Origin',(34.5439318808756,11.9341984494201,36.3106040574193));
#16627=CARTESIAN_POINT('Origin',(-39.6912298733817,12.8136401876617,39.8571882336823));
#16628=CARTESIAN_POINT('',(-40.5751133498648,13.1261401876617,38.9733047571991));
#16629=CARTESIAN_POINT('',(-38.8073463968985,13.1261401876617,40.7410717101655));
#16630=CARTESIAN_POINT('Origin',(-39.6912298733817,13.1261401876617,39.8571882336823));
#16631=CARTESIAN_POINT('',(-40.354142480744,12.8136401876617,39.1942756263199));
#16632=CARTESIAN_POINT('Origin',(-40.5751133498648,12.8136401876617,38.9733047571991));
#16633=CARTESIAN_POINT('',(-39.0283172660193,12.8136401876617,40.5201008410447));
#16634=CARTESIAN_POINT('Origin',(-39.6912298733817,12.8136401876617,39.8571882336823));
#16635=CARTESIAN_POINT('Origin',(-38.8073463968985,12.8136401876617,40.7410717101655));
#16636=CARTESIAN_POINT('Origin',(39.8582830101054,12.8136401876617,39.8571882336827));
#16637=CARTESIAN_POINT('',(38.9743995336222,13.1261401876617,40.7410717101659));
#16638=CARTESIAN_POINT('',(40.7421664865885,13.1261401876617,38.9733047571995));
#16639=CARTESIAN_POINT('Origin',(39.8582830101054,13.1261401876617,39.8571882336827));
#16640=CARTESIAN_POINT('',(39.195370402743,12.8136401876617,40.5201008410451));
#16641=CARTESIAN_POINT('Origin',(38.9743995336222,12.8136401876617,40.7410717101659));
#16642=CARTESIAN_POINT('',(40.5211956174677,12.8136401876617,39.1942756263203));
#16643=CARTESIAN_POINT('Origin',(39.8582830101054,12.8136401876617,39.8571882336827));
#16644=CARTESIAN_POINT('Origin',(40.7421664865885,12.8136401876617,38.9733047571995));
#16645=CARTESIAN_POINT('Origin',(-39.6912298733813,-8.24885981233827,-39.6923246498039));
#16646=CARTESIAN_POINT('',(-40.5751133498644,-8.56135981233827,-38.8084411733207));
#16647=CARTESIAN_POINT('',(-38.8073463968981,-8.56135981233827,-40.576208126287));
#16648=CARTESIAN_POINT('Origin',(-39.6912298733813,-8.56135981233827,-39.6923246498039));
#16649=CARTESIAN_POINT('',(-40.3541424807436,-8.24885981233828,-39.0294120424415));
#16650=CARTESIAN_POINT('Origin',(-40.5751133498644,-8.24885981233827,-38.8084411733207));
#16651=CARTESIAN_POINT('',(-39.0283172660189,-8.24885981233828,-40.3552372571663));
#16652=CARTESIAN_POINT('Origin',(-39.6912298733813,-8.24885981233827,-39.6923246498039));
#16653=CARTESIAN_POINT('Origin',(-38.8073463968981,-8.24885981233827,-40.576208126287));
#16654=CARTESIAN_POINT('Origin',(39.8582830101055,-8.24885981233827,-39.6923246498037));
#16655=CARTESIAN_POINT('',(38.9743995336223,-8.56135981233827,-40.5762081262869));
#16656=CARTESIAN_POINT('',(40.7421664865887,-8.56135981233827,-38.8084411733206));
#16657=CARTESIAN_POINT('Origin',(39.8582830101055,-8.56135981233827,-39.6923246498037));
#16658=CARTESIAN_POINT('',(39.1953704027431,-8.24885981233828,-40.3552372571661));
#16659=CARTESIAN_POINT('Origin',(38.9743995336223,-8.24885981233827,-40.5762081262869));
#16660=CARTESIAN_POINT('',(40.5211956174679,-8.24885981233828,-39.0294120424414));
#16661=CARTESIAN_POINT('Origin',(39.8582830101055,-8.24885981233827,-39.6923246498037));
#16662=CARTESIAN_POINT('Origin',(40.7421664865887,-8.24885981233827,-38.8084411733206));
#16663=CARTESIAN_POINT('Origin',(-34.3768787441515,11.4830954176946,-36.1457404735405));
#16664=CARTESIAN_POINT('',(-34.5978496132723,-3.61941807409669,-35.9247696044197));
#16665=CARTESIAN_POINT('',(-34.1615012109483,-3.61941807409668,-35.9193143968812));
#16666=CARTESIAN_POINT('Origin',(-34.3768787441515,-3.61941807409669,-36.1457404735405));
#16667=CARTESIAN_POINT('',(-34.5978496132723,11.9341984494202,-35.9247696044197));
#16668=CARTESIAN_POINT('',(-34.5978496132723,-3.74885981233827,-35.9247696044197));
#16669=CARTESIAN_POINT('',(-34.1615012109483,11.9341984494201,-35.9193143968812));
#16670=CARTESIAN_POINT('Origin',(-34.3768787441515,11.9341984494201,-36.1457404735405));
#16671=CARTESIAN_POINT('',(-34.1615012109483,11.4830954176946,-35.9193143968812));
#16672=CARTESIAN_POINT('Origin',(34.5439318808757,11.4830954176946,-36.1457404735404));
#16673=CARTESIAN_POINT('',(34.3285543476725,-3.61941807409668,-35.9193143968811));
#16674=CARTESIAN_POINT('',(34.7649027499965,-3.61941807409669,-35.9247696044196));
#16675=CARTESIAN_POINT('Origin',(34.5439318808757,-3.61941807409668,-36.1457404735404));
#16676=CARTESIAN_POINT('',(34.3285543476725,11.9341984494201,-35.9193143968811));
#16677=CARTESIAN_POINT('',(34.3285543476725,11.4830954176946,-35.9193143968811));
#16678=CARTESIAN_POINT('',(34.7649027499969,11.9341984494207,-35.92476960442));
#16679=CARTESIAN_POINT('Origin',(34.5439318808757,11.9341984494202,-36.1457404735404));
#16680=CARTESIAN_POINT('',(34.7649027499965,12.0636401876617,-35.9247696044196));
#16681=CARTESIAN_POINT('Origin',(-19.6585232829181,-11.0169045823054,10.2084687225244));
#16682=CARTESIAN_POINT('',(-19.3804662427592,-11.3294045823054,10.0658484840654));
#16683=CARTESIAN_POINT('',(-19.9553042598562,-11.3294045823054,10.1106050329982));
#16684=CARTESIAN_POINT('Origin',(-19.6585232829181,-11.3294045823054,10.2084687225244));
#16685=CARTESIAN_POINT('',(-19.9553042598562,-14.4544045823054,10.1106050329982));
#16686=CARTESIAN_POINT('',(-19.9553042598562,-11.0169045823054,10.1106050329982));
#16687=CARTESIAN_POINT('',(-19.3804662427592,-14.4544045823054,10.0658484840654));
#16688=CARTESIAN_POINT('Origin',(-19.6585232829181,-14.4544045823054,10.2084687225244));
#16689=CARTESIAN_POINT('',(-19.3804662427592,-11.0169045823054,10.0658484840654));
#16690=CARTESIAN_POINT('Origin',(-19.6585232829181,-11.3294045823054,10.2084687225244));
#16691=CARTESIAN_POINT('',(-19.1024092026003,-11.0169045823054,9.9232282456065));
#16692=CARTESIAN_POINT('Origin',(-19.1024092026003,-11.3294045823054,9.9232282456065));
#16693=CARTESIAN_POINT('',(-20.2520852367942,-11.0169045823054,10.012741343472));
#16694=CARTESIAN_POINT('Origin',(-19.6585232829181,-11.0169045823054,10.2084687225244));
#16695=CARTESIAN_POINT('Origin',(-20.2520852367942,-11.3294045823054,10.012741343472));
#16696=CARTESIAN_POINT('Origin',(-35.8042963200226,-14.7669045823054,33.0767747666364));
#16697=CARTESIAN_POINT('',(-36.1010780564215,-7.07885853810828,32.9789133801876));
#16698=CARTESIAN_POINT('',(-35.5742461733022,-7.07886995352308,32.8652725680806));
#16699=CARTESIAN_POINT('Origin',(-35.8042963200226,-7.07886995352308,33.0767747666364));
#16700=CARTESIAN_POINT('',(-35.5742461733022,-12.8919045823054,32.8652725680806));
#16701=CARTESIAN_POINT('',(-35.5742461733022,-14.7669045823054,32.8652725680806));
#16702=CARTESIAN_POINT('',(-36.1010772969607,-12.8919045823054,32.9789110771102));
#16703=CARTESIAN_POINT('Origin',(-35.8042963200226,-12.8919045823054,33.0767747666364));
#16704=CARTESIAN_POINT('',(-36.1010772969607,16.4855954176946,32.9789110771102));
#16705=CARTESIAN_POINT('Origin',(-38.2816342705276,-14.7669045823054,-28.971484618867));
#16706=CARTESIAN_POINT('',(-38.5307586915594,-11.3294045823054,-29.1601464137424));
#16707=CARTESIAN_POINT('',(-38.1837705810015,-11.3294045823054,-29.2682655958051));
#16708=CARTESIAN_POINT('Origin',(-38.2816342705276,-11.3294045823054,-28.971484618867));
#16709=CARTESIAN_POINT('',(-38.5307586915594,-12.8919045823054,-29.1601464137424));
#16710=CARTESIAN_POINT('',(-38.5307586915594,-14.7669045823054,-29.1601464137424));
#16711=CARTESIAN_POINT('',(-38.1837705810015,-12.8919045823054,-29.2682655958051));
#16712=CARTESIAN_POINT('Origin',(-38.2816342705276,-12.8919045823054,-28.971484618867));
#16713=CARTESIAN_POINT('',(-38.1837705810015,-11.0169045823054,-29.2682655958051));
#16714=CARTESIAN_POINT('Origin',(40.0376426042469,-14.7669045823054,28.0150491378139));
#16715=CARTESIAN_POINT('',(39.7815264758118,-6.59535043767467,27.8359938984173));
#16716=CARTESIAN_POINT('',(40.1355064102017,-6.5953500105935,27.7182681992682));
#16717=CARTESIAN_POINT('Origin',(40.0376426042469,-6.59535043767467,28.0150491378139));
#16718=CARTESIAN_POINT('',(40.1355062937731,-12.8919045823054,27.7182681608758));
#16719=CARTESIAN_POINT('',(40.1355062937731,-6.01690458230549,27.7182681608758));
#16720=CARTESIAN_POINT('',(39.7815264758118,-12.8919045823054,27.8359938984173));
#16721=CARTESIAN_POINT('Origin',(40.0376426042469,-12.8919045823054,28.0150491378139));
#16722=CARTESIAN_POINT('',(39.7815264758118,-14.7669045823054,27.8359938984173));
#16723=CARTESIAN_POINT('Origin',(34.5286855795389,-14.7669045823054,-33.5262969209224));
#16724=CARTESIAN_POINT('',(34.2319046026008,-11.3294045823054,-33.6241606104486));
#16725=CARTESIAN_POINT('',(34.7523554432479,-11.3294045823054,-33.7445354190578));
#16726=CARTESIAN_POINT('Origin',(34.5286855795389,-11.3294045823054,-33.5262969209224));
#16727=CARTESIAN_POINT('',(34.2319046026008,-12.8919045823054,-33.6241606104486));
#16728=CARTESIAN_POINT('',(34.2319046026008,-11.0169045823054,-33.6241606104486));
#16729=CARTESIAN_POINT('',(34.7523554432479,-12.8919045823054,-33.7445354190578));
#16730=CARTESIAN_POINT('Origin',(34.5286855795389,-12.8919045823054,-33.5262969209224));
#16731=CARTESIAN_POINT('',(34.7523554432479,-14.7669045823054,-33.7445354190578));
#16732=CARTESIAN_POINT('Origin',(19.8255764196421,-14.4544045823054,-10.0436051386457));
#16733=CARTESIAN_POINT('',(20.1223573965802,-14.4544045823054,-9.94574144911951));
#16734=CARTESIAN_POINT('',(19.5475193794832,-14.4544045823054,-9.90098490018674));
#16735=CARTESIAN_POINT('Origin',(19.8255764196421,-14.4544045823054,-10.0436051386457));
#16736=CARTESIAN_POINT('',(20.4191383735183,-14.7669045823054,-9.84787775959334));
#16737=CARTESIAN_POINT('Origin',(20.4191383735183,-14.4544045823054,-9.84787775959334));
#16738=CARTESIAN_POINT('',(19.2694623393243,-14.7669045823054,-9.75836466172779));
#16739=CARTESIAN_POINT('Origin',(19.8255764196421,-14.7669045823054,-10.0436051386457));
#16740=CARTESIAN_POINT('Origin',(19.2694623393243,-14.4544045823054,-9.75836466172779));
#16741=CARTESIAN_POINT('Origin',(-47.4164734316384,15.8580954176946,40.1612670779178));
#16742=CARTESIAN_POINT('',(-48.0414734316384,15.5455954176946,40.1612670779178));
#16743=CARTESIAN_POINT('',(-47.0488263728148,15.5455954176946,40.6666982207438));
#16744=CARTESIAN_POINT('Origin',(-47.4164734316384,15.5455954176946,40.1612670779178));
#16745=CARTESIAN_POINT('',(-48.3539734316384,15.8580954176946,40.1612670779178));
#16746=CARTESIAN_POINT('Origin',(-48.0414734316384,15.8580954176946,40.1612670779178));
#16747=CARTESIAN_POINT('',(-46.8650028434031,15.8580954176946,40.9194137921568));
#16748=CARTESIAN_POINT('Origin',(-47.4164734316384,15.8580954176946,40.1612670779178));
#16749=CARTESIAN_POINT('Origin',(-47.0488263728148,15.8580954176946,40.6666982207438));
#16750=CARTESIAN_POINT('Origin',(-47.4164734316384,16.1705954176946,40.1612670779178));
#16751=CARTESIAN_POINT('',(-46.6811793139913,16.4830954176946,41.1721293635699));
#16752=CARTESIAN_POINT('',(-48.6664734316384,16.4830954176946,40.1612670779178));
#16753=CARTESIAN_POINT('Origin',(-47.4164734316384,16.4830954176946,40.1612670779178));
#16754=CARTESIAN_POINT('',(-46.8650028434031,16.1705954176946,40.9194137921568));
#16755=CARTESIAN_POINT('Origin',(-46.6811793139913,16.1705954176946,41.1721293635698));
#16756=CARTESIAN_POINT('',(-48.3539734316384,16.1705954176946,40.1612670779178));
#16757=CARTESIAN_POINT('Origin',(-47.4164734316384,16.1705954176946,40.1612670779178));
#16758=CARTESIAN_POINT('Origin',(-48.6664734316384,16.1705954176946,40.1612670779178));
#16759=CARTESIAN_POINT('Origin',(-29.4588820377423,15.5455954176946,47.5824317919391));
#16760=CARTESIAN_POINT('',(-28.9637578711596,15.8580954176946,46.7863424064643));
#16761=CARTESIAN_POINT('',(-29.4588820377423,15.8580954176946,48.5199317919391));
#16762=CARTESIAN_POINT('Origin',(-29.4588820377423,15.8580954176946,47.5824317919391));
#16763=CARTESIAN_POINT('',(-29.4588820377423,16.1705954176946,48.5199317919391));
#16764=CARTESIAN_POINT('',(-29.4588820377423,15.5455954176946,48.5199317919391));
#16765=CARTESIAN_POINT('',(-28.9637578711596,16.1705954176946,46.7863424064643));
#16766=CARTESIAN_POINT('Origin',(-29.4588820377423,16.1705954176946,47.5824317919391));
#16767=CARTESIAN_POINT('',(-28.9637578711596,15.5455954176946,46.7863424064643));
#16768=CARTESIAN_POINT('Origin',(-44.2914734316384,15.5455954176946,44.457431791939));
#16769=CARTESIAN_POINT('',(-40.7534554318564,15.8580954176946,47.0309612037037));
#16770=CARTESIAN_POINT('Origin',(-44.2914734316384,15.8580954176946,44.457431791939));
#16771=CARTESIAN_POINT('',(-46.8650028434031,15.5455954176946,40.9194137921568));
#16772=CARTESIAN_POINT('',(-40.7534554318564,16.1705954176946,47.0309612037037));
#16773=CARTESIAN_POINT('Origin',(-44.2914734316384,16.1705954176946,44.457431791939));
#16774=CARTESIAN_POINT('',(-40.7534554318564,15.5455954176946,47.0309612037037));
#16775=CARTESIAN_POINT('Origin',(-44.2914734316384,16.4830954176946,44.457431791939));
#16776=CARTESIAN_POINT('',(-41.4789734316384,16.4830954176946,44.457431791939));
#16777=CARTESIAN_POINT('Origin',(-44.2914734316384,16.4830954176946,44.457431791939));
#16778=CARTESIAN_POINT('',(-41.4789734316384,16.4830954176946,44.457431791939));
#16779=CARTESIAN_POINT('Origin',(-39.6912298733817,13.1261401876617,39.8571882336823));
#16780=CARTESIAN_POINT('',(-40.354142480744,-8.24885981233828,39.1942756263199));
#16781=CARTESIAN_POINT('',(-40.354142480744,16.4855954176946,39.1942756263199));
#16782=CARTESIAN_POINT('',(-39.0283172660193,-8.24885981233828,40.5201008410447));
#16783=CARTESIAN_POINT('Origin',(-39.6912298733817,-8.24885981233827,39.8571882336823));
#16784=CARTESIAN_POINT('',(-39.0283172660193,16.4855954176946,40.5201008410447));
#16785=CARTESIAN_POINT('Origin',(47.583526568362,15.5455954176946,29.6248403980433));
#16786=CARTESIAN_POINT('',(46.7874371828872,15.8580954176946,29.1297162314606));
#16787=CARTESIAN_POINT('',(48.5210265683621,15.8580954176946,29.6248403980433));
#16788=CARTESIAN_POINT('Origin',(47.583526568362,15.8580954176946,29.6248403980433));
#16789=CARTESIAN_POINT('',(48.5210265683621,16.1705954176946,29.6248403980433));
#16790=CARTESIAN_POINT('',(48.5210265683621,15.5455954176946,29.6248403980433));
#16791=CARTESIAN_POINT('',(46.7874371828872,16.1705954176946,29.1297162314606));
#16792=CARTESIAN_POINT('Origin',(47.583526568362,16.1705954176946,29.6248403980433));
#16793=CARTESIAN_POINT('',(46.7874371828872,15.5455954176946,29.1297162314606));
#16794=CARTESIAN_POINT('Origin',(44.4585265683621,15.5455954176946,44.4574317919394));
#16795=CARTESIAN_POINT('',(40.92050856858,15.8580954176946,47.0309612037041));
#16796=CARTESIAN_POINT('Origin',(44.4585265683621,15.8580954176946,44.4574317919394));
#16797=CARTESIAN_POINT('',(40.92050856858,16.1705954176946,47.0309612037041));
#16798=CARTESIAN_POINT('',(40.92050856858,15.5455954176946,47.0309612037041));
#16799=CARTESIAN_POINT('Origin',(44.4585265683621,16.1705954176946,44.4574317919394));
#16800=CARTESIAN_POINT('',(47.0320559801268,15.5455954176946,40.9194137921573));
#16801=CARTESIAN_POINT('Origin',(44.4585265683621,16.4830954176946,44.4574317919394));
#16802=CARTESIAN_POINT('',(44.4585265683621,16.4830954176946,41.6449317919394));
#16803=CARTESIAN_POINT('Origin',(44.4585265683621,16.4830954176946,44.4574317919394));
#16804=CARTESIAN_POINT('',(44.4585265683621,16.4830954176946,41.6449317919394));
#16805=CARTESIAN_POINT('Origin',(0.0835265683620477,-8.56135981233827,0.0824317919394229));
#16806=CARTESIAN_POINT('',(-37.498691208412,-8.46983068145907,39.4252660733572));
#16807=CARTESIAN_POINT('Ctrl Pts',(-34.2245838299087,-3.84038894321748,
36.1504966431758));
#16808=CARTESIAN_POINT('Ctrl Pts',(-34.3287551251596,-3.98768003220409,
36.2546909526594));
#16809=CARTESIAN_POINT('Ctrl Pts',(-34.4329263800975,-4.13497132206384,
36.3588850184894));
#16810=CARTESIAN_POINT('Ctrl Pts',(-34.9537824584041,-4.87142874967366,
36.8798541610334));
#16811=CARTESIAN_POINT('Ctrl Pts',(-35.370466693267,-5.46059781902367,37.2966256819533));
#16812=CARTESIAN_POINT('Ctrl Pts',(-36.3576649944858,-6.85645163869056,
38.2840240167437));
#16813=CARTESIAN_POINT('Ctrl Pts',(-36.9281785657525,-7.66313885272879,
38.8546478427941));
#16814=CARTESIAN_POINT('Ctrl Pts',(-37.498691208412,-8.46983068145907,39.4252660733572));
#16815=CARTESIAN_POINT('',(-21.6249416886588,-8.46983068145907,49.9725521390571));
#16816=CARTESIAN_POINT('Origin',(0.0835265683620477,-8.46983068145906,0.0824317919394229));
#16817=CARTESIAN_POINT('',(0.0835265683492263,-3.96983068145906,49.9909026610602));
#16818=CARTESIAN_POINT('Ctrl Pts',(-21.6249416886588,-8.46983068145907,
49.9725521390571));
#16819=CARTESIAN_POINT('Ctrl Pts',(-18.1505891136337,-7.08833344112081,
49.9777178959269));
#16820=CARTESIAN_POINT('Ctrl Pts',(-14.6164545138694,-5.9615388332069,49.9823364948316));
#16821=CARTESIAN_POINT('Ctrl Pts',(-9.19340825173301,-4.7904640513231,49.9872996399547));
#16822=CARTESIAN_POINT('Ctrl Pts',(-7.36536697272742,-4.48684598729498,
49.9886233704762));
#16823=CARTESIAN_POINT('Ctrl Pts',(-4.58873775481838,-4.17869234558141,
49.9899767682438));
#16824=CARTESIAN_POINT('Ctrl Pts',(-3.65694097482046,-4.10048196518639,
49.9903229073071));
#16825=CARTESIAN_POINT('Ctrl Pts',(-1.7832453138779,-3.99585474310376,49.9907867430663));
#16826=CARTESIAN_POINT('Ctrl Pts',(-0.848713204691103,-3.9698306814593,
49.9909026610602));
#16827=CARTESIAN_POINT('Ctrl Pts',(0.0835265683492263,-3.96983068145906,
49.9909026610602));
#16828=CARTESIAN_POINT('',(21.7919948253829,-8.46983068145907,49.9725521390571));
#16829=CARTESIAN_POINT('Ctrl Pts',(0.0835265683492263,-3.96983068145906,
49.9909026610602));
#16830=CARTESIAN_POINT('Ctrl Pts',(3.7948657945546,-3.96983068145811,49.9909026610602));
#16831=CARTESIAN_POINT('Ctrl Pts',(7.46954951636237,-4.38596719587718,49.9890155336001));
#16832=CARTESIAN_POINT('Ctrl Pts',(12.022537961721,-5.36440184532963,49.9848668452853));
#16833=CARTESIAN_POINT('Ctrl Pts',(12.9310838207197,-5.58285881740927,49.9839501483763));
#16834=CARTESIAN_POINT('Ctrl Pts',(14.7347887768393,-6.06008817135185,49.9819775669644));
#16835=CARTESIAN_POINT('Ctrl Pts',(15.6315620628568,-6.31922781225809,49.9809201793626));
#16836=CARTESIAN_POINT('Ctrl Pts',(18.3027695373097,-7.15188128916169,49.9775797432466));
#16837=CARTESIAN_POINT('Ctrl Pts',(20.0580108836304,-7.78035142493754,49.9751302710301));
#16838=CARTESIAN_POINT('Ctrl Pts',(21.7919948253829,-8.46983068145907,49.9725521390571));
#16839=CARTESIAN_POINT('',(37.6657443451356,-8.46983068145907,39.4252660733575));
#16840=CARTESIAN_POINT('Origin',(0.0835265683620477,-8.46983068145906,0.0824317919394229));
#16841=CARTESIAN_POINT('Ctrl Pts',(37.6657443451356,-8.46983068145907,39.4252660733575));
#16842=CARTESIAN_POINT('Ctrl Pts',(37.5615737916312,-8.32253590125116,39.3210762404375));
#16843=CARTESIAN_POINT('Ctrl Pts',(37.457403207105,-8.17524127521396,39.2168862205796));
#16844=CARTESIAN_POINT('Ctrl Pts',(36.9365501255862,-7.43876893481716,38.6959351635992));
#16845=CARTESIAN_POINT('Ctrl Pts',(36.5198671524687,-6.84959358714928,38.2791712566788));
#16846=CARTESIAN_POINT('Ctrl Pts',(35.5326691698879,-5.45373818194082,37.2917748447513));
#16847=CARTESIAN_POINT('Ctrl Pts',(34.9621536716281,-4.64706055617428,36.7211393906113));
#16848=CARTESIAN_POINT('Ctrl Pts',(34.3916369666324,-3.84038894321748,36.1504966431761));
#16849=CARTESIAN_POINT('Origin',(39.8582830101054,13.1261401876617,39.8571882336827));
#16850=CARTESIAN_POINT('',(39.195370402743,-8.24885981233828,40.5201008410451));
#16851=CARTESIAN_POINT('',(39.195370402743,16.4855954176946,40.5201008410451));
#16852=CARTESIAN_POINT('',(40.5211956174677,-8.24885981233828,39.1942756263203));
#16853=CARTESIAN_POINT('Origin',(39.8582830101054,-8.24885981233827,39.8571882336827));
#16854=CARTESIAN_POINT('',(40.5211956174677,16.4855954176946,39.1942756263203));
#16855=CARTESIAN_POINT('Origin',(29.6259351744661,15.5455954176946,-47.4175682080605));
#16856=CARTESIAN_POINT('',(29.1308110078834,15.8580954176946,-46.6214788225856));
#16857=CARTESIAN_POINT('',(29.6259351744661,15.8580954176946,-48.3550682080605));
#16858=CARTESIAN_POINT('Origin',(29.6259351744661,15.8580954176946,-47.4175682080605));
#16859=CARTESIAN_POINT('',(29.6259351744661,16.1705954176946,-48.3550682080605));
#16860=CARTESIAN_POINT('',(29.6259351744661,15.5455954176946,-48.3550682080605));
#16861=CARTESIAN_POINT('',(29.1308110078834,16.1705954176946,-46.6214788225856));
#16862=CARTESIAN_POINT('Origin',(29.6259351744661,16.1705954176946,-47.4175682080605));
#16863=CARTESIAN_POINT('',(29.1308110078834,15.5455954176946,-46.6214788225856));
#16864=CARTESIAN_POINT('Origin',(44.4585265683622,15.5455954176946,-44.2925682080604));
#16865=CARTESIAN_POINT('',(47.0320559801269,15.5455954176946,-40.7545502082783));
#16866=CARTESIAN_POINT('',(40.9205085685801,15.5455954176946,-46.8660976198251));
#16867=CARTESIAN_POINT('Origin',(44.4585265683622,16.4830954176946,-44.2925682080604));
#16868=CARTESIAN_POINT('',(41.6460265683622,16.4830954176946,-44.2925682080604));
#16869=CARTESIAN_POINT('Origin',(44.4585265683622,16.4830954176946,-44.2925682080604));
#16870=CARTESIAN_POINT('',(41.6460265683622,16.4830954176946,-44.2925682080604));
#16871=CARTESIAN_POINT('Origin',(0.0835265683620477,-8.56135981233827,0.0824317919394229));
#16872=CARTESIAN_POINT('',(36.1515914195989,-3.84038894321748,-34.2256786063308));
#16873=CARTESIAN_POINT('',(36.1515914195988,-3.84038894321748,34.3905421902098));
#16874=CARTESIAN_POINT('Origin',(0.0835265683620477,-3.84038894321747,0.0824317919394229));
#16875=CARTESIAN_POINT('',(39.4263608497802,-8.46983068145907,37.664649568713));
#16876=CARTESIAN_POINT('Ctrl Pts',(36.1515914195988,-3.84038894321748,34.3905421902098));
#16877=CARTESIAN_POINT('Ctrl Pts',(36.2557857290823,-3.98768003220409,34.4947134854607));
#16878=CARTESIAN_POINT('Ctrl Pts',(36.3599797949124,-4.13497132206384,34.5988847403986));
#16879=CARTESIAN_POINT('Ctrl Pts',(36.8809489374564,-4.87142874967365,35.1197408187052));
#16880=CARTESIAN_POINT('Ctrl Pts',(37.2977204583763,-5.46059781902367,35.536425053568));
#16881=CARTESIAN_POINT('Ctrl Pts',(38.2851187931668,-6.85645163869055,36.5236233547868));
#16882=CARTESIAN_POINT('Ctrl Pts',(38.8557426192171,-7.66313885272879,37.0941369260536));
#16883=CARTESIAN_POINT('Ctrl Pts',(39.4263608497802,-8.46983068145907,37.664649568713));
#16884=CARTESIAN_POINT('',(49.9736469154797,-8.46983068145907,21.7909000489604));
#16885=CARTESIAN_POINT('Origin',(0.0835265683620477,-8.46983068145906,0.0824317919394229));
#16886=CARTESIAN_POINT('',(49.9919974374829,-3.96983068145906,0.0824317919524185));
#16887=CARTESIAN_POINT('Ctrl Pts',(49.9736469154797,-8.46983068145907,21.7909000489604));
#16888=CARTESIAN_POINT('Ctrl Pts',(49.9788126723494,-7.08833344112081,18.3165474739353));
#16889=CARTESIAN_POINT('Ctrl Pts',(49.9834312712542,-5.9615388332069,14.7824128741711));
#16890=CARTESIAN_POINT('Ctrl Pts',(49.9883944163773,-4.7904640513231,9.35936661203465));
#16891=CARTESIAN_POINT('Ctrl Pts',(49.9897181468988,-4.48684598729498,7.53132533302907));
#16892=CARTESIAN_POINT('Ctrl Pts',(49.9910715446664,-4.17869234558141,4.75469611512003));
#16893=CARTESIAN_POINT('Ctrl Pts',(49.9914176837298,-4.10048196518639,3.8228993351221));
#16894=CARTESIAN_POINT('Ctrl Pts',(49.9918815194889,-3.99585474310375,1.94920367417954));
#16895=CARTESIAN_POINT('Ctrl Pts',(49.9919974374829,-3.9698306814593,1.01467156499275));
#16896=CARTESIAN_POINT('Ctrl Pts',(49.9919974374829,-3.96983068145906,0.0824317919524185));
#16897=CARTESIAN_POINT('',(49.9736469154798,-8.46983068145907,-21.6260364650812));
#16898=CARTESIAN_POINT('Ctrl Pts',(49.9919974374829,-3.96983068145906,0.0824317919524185));
#16899=CARTESIAN_POINT('Ctrl Pts',(49.9919974374829,-3.96983068145811,-3.62890743425295));
#16900=CARTESIAN_POINT('Ctrl Pts',(49.9901103100228,-4.38596719587718,-7.30359115606072));
#16901=CARTESIAN_POINT('Ctrl Pts',(49.9859616217079,-5.36440184532962,-11.8565796014193));
#16902=CARTESIAN_POINT('Ctrl Pts',(49.985044924799,-5.58285881740927,-12.7651254604181));
#16903=CARTESIAN_POINT('Ctrl Pts',(49.9830723433871,-6.06008817135185,-14.5688304165376));
#16904=CARTESIAN_POINT('Ctrl Pts',(49.9820149557853,-6.31922781225809,-15.4656037025551));
#16905=CARTESIAN_POINT('Ctrl Pts',(49.9786745196693,-7.15188128916169,-18.136811177008));
#16906=CARTESIAN_POINT('Ctrl Pts',(49.9762250474528,-7.78035142493754,-19.8920525233287));
#16907=CARTESIAN_POINT('Ctrl Pts',(49.9736469154798,-8.46983068145907,-21.6260364650812));
#16908=CARTESIAN_POINT('',(39.4263608497803,-8.46983068145907,-37.499785984834));
#16909=CARTESIAN_POINT('Origin',(0.0835265683620477,-8.46983068145906,0.0824317919394229));
#16910=CARTESIAN_POINT('Ctrl Pts',(39.4263608497803,-8.46983068145907,-37.499785984834));
#16911=CARTESIAN_POINT('Ctrl Pts',(39.3221710168602,-8.32253590125115,-37.3956154313296));
#16912=CARTESIAN_POINT('Ctrl Pts',(39.2179809970023,-8.17524127521395,-37.2914448468034));
#16913=CARTESIAN_POINT('Ctrl Pts',(38.6970299400219,-7.43876893481715,-36.7705917652845));
#16914=CARTESIAN_POINT('Ctrl Pts',(38.2802660331016,-6.84959358714927,-36.3539087921671));
#16915=CARTESIAN_POINT('Ctrl Pts',(37.292869621174,-5.45373818194082,-35.3667108095863));
#16916=CARTESIAN_POINT('Ctrl Pts',(36.7222341670341,-4.64706055617428,-34.7961953113265));
#16917=CARTESIAN_POINT('Ctrl Pts',(36.1515914195989,-3.84038894321748,-34.2256786063308));
#16918=CARTESIAN_POINT('Origin',(39.8582830101055,13.1261401876617,-39.6923246498037));
#16919=CARTESIAN_POINT('',(39.1953704027431,12.8136401876617,-40.3552372571661));
#16920=CARTESIAN_POINT('',(40.5211956174679,12.8136401876617,-39.0294120424414));
#16921=CARTESIAN_POINT('Origin',(39.8582830101055,12.8136401876617,-39.6923246498037));
#16922=CARTESIAN_POINT('',(40.5211956174679,16.4855954176946,-39.0294120424414));
#16923=CARTESIAN_POINT('',(39.1953704027431,16.4855954176946,-40.3552372571661));
#16924=CARTESIAN_POINT('Origin',(-47.4164734316379,15.5455954176946,-29.4599768141645));
#16925=CARTESIAN_POINT('',(-48.3539734316379,15.5455954176946,-29.4599768141645));
#16926=CARTESIAN_POINT('',(-46.6203840461631,15.5455954176946,-28.9648526475817));
#16927=CARTESIAN_POINT('Origin',(-44.291473431638,15.5455954176946,-44.2925682080606));
#16928=CARTESIAN_POINT('',(-40.7534554318559,15.5455954176946,-46.8660976198253));
#16929=CARTESIAN_POINT('',(-46.8650028434027,15.5455954176946,-40.7545502082785));
#16930=CARTESIAN_POINT('Origin',(0.0835265683620477,-14.7669045823054,0.0824317919394229));
#16931=CARTESIAN_POINT('',(-4.12926308943375,11.3536536794531,-48.1715194405676));
#16932=CARTESIAN_POINT('',(0.0835265683620358,11.3536536794531,-48.3550682080606));
#16933=CARTESIAN_POINT('Origin',(0.083526568361586,11.3536536794531,0.08243179193129));
#16934=CARTESIAN_POINT('',(-48.170424664145,11.3536536794531,-4.13035786585642));
#16935=CARTESIAN_POINT('Origin',(0.0835265683620477,11.3536536794531,0.0824317919394229));
#16936=CARTESIAN_POINT('',(-48.3539734316379,11.3536536794531,0.0824317919394318));
#16937=CARTESIAN_POINT('Origin',(0.0835265683582076,11.3536536794531,0.0824317919397211));
#16938=CARTESIAN_POINT('',(-48.170424664145,11.3536536794531,4.29522144973529));
#16939=CARTESIAN_POINT('Origin',(0.0835265683498587,11.3536536794531,0.0824317919398798));
#16940=CARTESIAN_POINT('',(-4.12926308943382,11.3536536794531,48.3363830244465));
#16941=CARTESIAN_POINT('Origin',(0.0835265683620477,11.3536536794531,0.0824317919394229));
#16942=CARTESIAN_POINT('',(0.0835265683619891,11.353653679453,48.5199317919394));
#16943=CARTESIAN_POINT('Origin',(0.083526568362857,11.3536536794495,0.0824317919438222));
#16944=CARTESIAN_POINT('',(0.0835265683620321,-5.88746284406389,48.5199317919394));
#16945=CARTESIAN_POINT('',(0.0835265683620418,-14.7669045823054,48.5199317919394));
#16946=CARTESIAN_POINT('',(-4.12926308943386,-5.88746284406389,48.3363830244465));
#16947=CARTESIAN_POINT('Origin',(0.0835265683626552,-5.88746284406448,0.0824317919388395));
#16948=CARTESIAN_POINT('',(-27.2418903719914,-5.88746284406389,40.0763437697123));
#16949=CARTESIAN_POINT('Origin',(0.0835265683620477,-5.88746284406389,0.0824317919394229));
#16950=CARTESIAN_POINT('',(-27.6700355381162,-6.59535043767466,39.7804316993888));
#16951=CARTESIAN_POINT('Ctrl Pts',(-27.6700355381162,-6.59535043767466,
39.7804316993888));
#16952=CARTESIAN_POINT('Ctrl Pts',(-27.6700355381162,-6.5748915141942,39.7804316993888));
#16953=CARTESIAN_POINT('Ctrl Pts',(-27.6696020394875,-6.5545035776552,39.7807360426617));
#16954=CARTESIAN_POINT('Ctrl Pts',(-27.6687133155359,-6.53419088775616,
39.781359050409));
#16955=CARTESIAN_POINT('Ctrl Pts',(-27.6675053825142,-6.5065823498666,39.782205828117));
#16956=CARTESIAN_POINT('Ctrl Pts',(-27.6654348566091,-6.479110981132,39.783656417799));
#16957=CARTESIAN_POINT('Ctrl Pts',(-27.662458871153,-6.45179259387541,39.7857387782774));
#16958=CARTESIAN_POINT('Ctrl Pts',(-27.659628589561,-6.42581171133553,39.7877191866554));
#16959=CARTESIAN_POINT('Ctrl Pts',(-27.6559796057934,-6.39996806268515,
39.7902708432567));
#16960=CARTESIAN_POINT('Ctrl Pts',(-27.651437028073,-6.37426951908202,39.7934443375415));
#16961=CARTESIAN_POINT('Ctrl Pts',(-27.6502134107345,-6.36734719755818,
39.794299169945));
#16962=CARTESIAN_POINT('Ctrl Pts',(-27.6489247207208,-6.36043542154694,
39.795199285491));
#16963=CARTESIAN_POINT('Ctrl Pts',(-27.6475689488363,-6.3535344231453,39.7961460526717));
#16964=CARTESIAN_POINT('Ctrl Pts',(-27.6456220716296,-6.3436246465487,39.7975056025083));
#16965=CARTESIAN_POINT('Ctrl Pts',(-27.6435418871642,-6.33375626741061,
39.7989578438024));
#16966=CARTESIAN_POINT('Ctrl Pts',(-27.6413233490211,-6.32393813773166,
39.8005062057689));
#16967=CARTESIAN_POINT('Ctrl Pts',(-27.6327865713909,-6.2861586701688,39.8064641929417));
#16968=CARTESIAN_POINT('Ctrl Pts',(-27.6222074393751,-6.24912973385534,
39.813841101647));
#16969=CARTESIAN_POINT('Ctrl Pts',(-27.6092852505015,-6.21334185676859,
39.8228414839607));
#16970=CARTESIAN_POINT('Ctrl Pts',(-27.5986999063164,-6.18402584844163,
39.8302142398862));
#16971=CARTESIAN_POINT('Ctrl Pts',(-27.5865425257292,-6.15554336971624,
39.8386762248601));
#16972=CARTESIAN_POINT('Ctrl Pts',(-27.5726642605709,-6.12818087652873,
39.8483281744703));
#16973=CARTESIAN_POINT('Ctrl Pts',(-27.5725963897865,-6.12804706197383,
39.8483753767238));
#16974=CARTESIAN_POINT('Ctrl Pts',(-27.5725284783993,-6.12791327327701,
39.8484226070511));
#16975=CARTESIAN_POINT('Ctrl Pts',(-27.5724605263936,-6.12777951046925,
39.8484698654626));
#16976=CARTESIAN_POINT('Ctrl Pts',(-27.5485439724826,-6.08070002591405,
39.8651030514228));
#16977=CARTESIAN_POINT('Ctrl Pts',(-27.5191242797118,-6.03703191462283,
39.8855326916264));
#16978=CARTESIAN_POINT('Ctrl Pts',(-27.4849266552093,-6.00042962270608,
39.9092043716615));
#16979=CARTESIAN_POINT('Ctrl Pts',(-27.4687964376931,-5.98316517996187,
39.9203697480142));
#16980=CARTESIAN_POINT('Ctrl Pts',(-27.4516032390886,-5.96747341995239,
39.9322563953063));
#16981=CARTESIAN_POINT('Ctrl Pts',(-27.4334232937986,-5.95374197151968,
39.9448059878606));
#16982=CARTESIAN_POINT('Ctrl Pts',(-27.4332934621217,-5.95364390868465,
39.944895610498));
#16983=CARTESIAN_POINT('Ctrl Pts',(-27.4331635831385,-5.95354594807983,
39.9449852648623));
#16984=CARTESIAN_POINT('Ctrl Pts',(-27.4330336568643,-5.95344808981852,
39.945074950941));
#16985=CARTESIAN_POINT('Ctrl Pts',(-27.4150725570453,-5.93992009472891,
39.957473217735));
#16986=CARTESIAN_POINT('Ctrl Pts',(-27.396127418154,-5.9283828834484,39.970530680642));
#16987=CARTESIAN_POINT('Ctrl Pts',(-27.3764749543957,-5.91890173045426,
39.9840541937056));
#16988=CARTESIAN_POINT('Ctrl Pts',(-27.3568153303916,-5.90941712306448,
39.9975826339721));
#16989=CARTESIAN_POINT('Ctrl Pts',(-27.3364466141785,-5.9019896316863,40.0115783367673));
#16990=CARTESIAN_POINT('Ctrl Pts',(-27.3156304996253,-5.89673275177562,
40.0258579998765));
#16991=CARTESIAN_POINT('Ctrl Pts',(-27.2957189352997,-5.89170430603829,
40.0395171498498));
#16992=CARTESIAN_POINT('Ctrl Pts',(-27.27539694813,-5.88866186034996,40.0534368547936));
#16993=CARTESIAN_POINT('Ctrl Pts',(-27.254896375492,-5.88775186306171,40.0674541942025));
#16994=CARTESIAN_POINT('Ctrl Pts',(-27.2505682042467,-5.88755974042368,
40.0704135966757));
#16995=CARTESIAN_POINT('Ctrl Pts',(-27.2462321146088,-5.88746284473751,
40.0733773200353));
#16996=CARTESIAN_POINT('Ctrl Pts',(-27.2418903719914,-5.88746284406389,
40.0763437697123));
#16997=CARTESIAN_POINT('',(-27.6700355381162,-12.8919045823054,39.7804316993888));
#16998=CARTESIAN_POINT('',(-27.6700355381162,-14.7669045823054,39.7804316993888));
#16999=CARTESIAN_POINT('',(-29.1590516373201,-12.8919045823054,38.6967170518605));
#17000=CARTESIAN_POINT('Origin',(0.0835265683620477,-12.8919045823054,0.0824317919394229));
#17001=CARTESIAN_POINT('',(-29.1590516373201,-11.3294045823054,38.6967170518605));
#17002=CARTESIAN_POINT('',(-29.1590516373202,-14.7669045823054,38.6967170518605));
#17003=CARTESIAN_POINT('',(-29.687554196627,-10.7044045823054,38.2907313659129));
#17004=CARTESIAN_POINT('Ctrl Pts',(-29.687554196627,-10.7044045823054,38.2907313659129));
#17005=CARTESIAN_POINT('Ctrl Pts',(-29.6583757220387,-10.7044045890531,
38.313466602321));
#17006=CARTESIAN_POINT('Ctrl Pts',(-29.6292220155259,-10.7074293129566,
38.3361197336984));
#17007=CARTESIAN_POINT('Ctrl Pts',(-29.6004506138901,-10.7132787489596,
38.3584250011361));
#17008=CARTESIAN_POINT('Ctrl Pts',(-29.5697316292104,-10.7195241428141,
38.382240148461));
#17009=CARTESIAN_POINT('Ctrl Pts',(-29.5394474529814,-10.7289894494766,
38.4056595080039));
#17010=CARTESIAN_POINT('Ctrl Pts',(-29.5100173969805,-10.7414871419677,
38.4283705160146));
#17011=CARTESIAN_POINT('Ctrl Pts',(-29.4803562185471,-10.7540829823212,
38.4512598799011));
#17012=CARTESIAN_POINT('Ctrl Pts',(-29.4515613322926,-10.769759396561,38.4734306970218));
#17013=CARTESIAN_POINT('Ctrl Pts',(-29.4240644721472,-10.7883769193556,
38.4945600707541));
#17014=CARTESIAN_POINT('Ctrl Pts',(-29.3976983269581,-10.8062288597759,
38.5148205707761));
#17015=CARTESIAN_POINT('Ctrl Pts',(-29.3725246545643,-10.8267856372238,
38.5341242584425));
#17016=CARTESIAN_POINT('Ctrl Pts',(-29.3489428815995,-10.8499643578231,
38.5521714250646));
#17017=CARTESIAN_POINT('Ctrl Pts',(-29.3390845628995,-10.8596541811907,
38.5597160113203));
#17018=CARTESIAN_POINT('Ctrl Pts',(-29.3295047666208,-10.869802668699,38.5670407550077));
#17019=CARTESIAN_POINT('Ctrl Pts',(-29.3202343227628,-10.8804055842375,
38.5741224750986));
#17020=CARTESIAN_POINT('Ctrl Pts',(-29.320109404838,-10.8805484570304,38.574217900279));
#17021=CARTESIAN_POINT('Ctrl Pts',(-29.3199845450897,-10.8806914099898,
38.5743132797999));
#17022=CARTESIAN_POINT('Ctrl Pts',(-29.3198597435962,-10.8808344430918,
38.5744086136027));
#17023=CARTESIAN_POINT('Ctrl Pts',(-29.2975936746061,-10.9063532475959,
38.5914172965067));
#17024=CARTESIAN_POINT('Ctrl Pts',(-29.2772105079594,-10.9345143821537,
38.6069608464538));
#17025=CARTESIAN_POINT('Ctrl Pts',(-29.2589893852,-10.9647671393855,38.6208380965538));
#17026=CARTESIAN_POINT('Ctrl Pts',(-29.2363360171296,-11.0023788087523,
38.6380909551439));
#17027=CARTESIAN_POINT('Ctrl Pts',(-29.2170205823372,-11.0432205203856,
38.6527712187733));
#17028=CARTESIAN_POINT('Ctrl Pts',(-29.2015725997599,-11.0862730506022,
38.6644974939291));
#17029=CARTESIAN_POINT('Ctrl Pts',(-29.1879031237235,-11.1243689978983,
38.6748737379748));
#17030=CARTESIAN_POINT('Ctrl Pts',(-29.1772602520119,-11.1641988556188,
38.6829382142099));
#17031=CARTESIAN_POINT('Ctrl Pts',(-29.1700361140648,-11.2050768635799,
38.6884075571799));
#17032=CARTESIAN_POINT('Ctrl Pts',(-29.1628548700807,-11.2457121547251,
38.6938444254385));
#17033=CARTESIAN_POINT('Ctrl Pts',(-29.1590516538054,-11.2873849299308,
38.6967170393762));
#17034=CARTESIAN_POINT('Ctrl Pts',(-29.1590516373202,-11.3294045823054,
38.6967170518605));
#17035=CARTESIAN_POINT('',(-34.088419713945,-10.7044045823054,34.4112752552593));
#17036=CARTESIAN_POINT('Origin',(0.0835265683620477,-10.7044045823054,0.0824317919394229));
#17037=CARTESIAN_POINT('',(-34.585302306524,-11.3294045823054,33.9093990029365));
#17038=CARTESIAN_POINT('Ctrl Pts',(-34.585302306524,-11.3294045823054,33.9093990029365));
#17039=CARTESIAN_POINT('Ctrl Pts',(-34.585302306524,-11.2968266539588,33.9093990029365));
#17040=CARTESIAN_POINT('Ctrl Pts',(-34.583309967139,-11.2645751882994,33.9114431380499));
#17041=CARTESIAN_POINT('Ctrl Pts',(-34.5793977169934,-11.2329045289625,
33.9154520195086));
#17042=CARTESIAN_POINT('Ctrl Pts',(-34.5753887114088,-11.2004506097532,
33.9195600462345));
#17043=CARTESIAN_POINT('Ctrl Pts',(-34.5693637902165,-11.1686071890508,
33.9257310494866));
#17044=CARTESIAN_POINT('Ctrl Pts',(-34.561438831968,-11.137638677353,33.9338407021739));
#17045=CARTESIAN_POINT('Ctrl Pts',(-34.5562225782153,-11.1172550222857,
33.9391785228837));
#17046=CARTESIAN_POINT('Ctrl Pts',(-34.5501839428663,-11.0972501995401,
33.9453554341431));
#17047=CARTESIAN_POINT('Ctrl Pts',(-34.5433640724374,-11.0776955263552,
33.9523277291817));
#17048=CARTESIAN_POINT('Ctrl Pts',(-34.5432467507797,-11.0773591289561,
33.9524476729872));
#17049=CARTESIAN_POINT('Ctrl Pts',(-34.543129225895,-11.0770229370417,33.9525678233924));
#17050=CARTESIAN_POINT('Ctrl Pts',(-34.5430114980424,-11.0766869507352,
33.9526881801171));
#17051=CARTESIAN_POINT('Ctrl Pts',(-34.5278035526398,-11.0332846352166,
33.9682357201253));
#17052=CARTESIAN_POINT('Ctrl Pts',(-34.5091770363952,-10.9932074810414,
33.9872584511094));
#17053=CARTESIAN_POINT('Ctrl Pts',(-34.4875301338769,-10.9565169212725,
34.0093162098418));
#17054=CARTESIAN_POINT('Ctrl Pts',(-34.4702171093455,-10.9271720964961,
34.0269578339827));
#17055=CARTESIAN_POINT('Ctrl Pts',(-34.450971186212,-10.8999941023543,34.046541760117));
#17056=CARTESIAN_POINT('Ctrl Pts',(-34.4299825590917,-10.8750283402103,
34.067856520148));
#17057=CARTESIAN_POINT('Ctrl Pts',(-34.4297522092966,-10.8747543414318,
34.0680904492458));
#17058=CARTESIAN_POINT('Ctrl Pts',(-34.4295217184696,-10.8744806828914,
34.0683245168216));
#17059=CARTESIAN_POINT('Ctrl Pts',(-34.4292910866631,-10.8742073644078,
34.0685587228044));
#17060=CARTESIAN_POINT('Ctrl Pts',(-34.3965447492566,-10.8354001442594,
34.1018125409014));
#17061=CARTESIAN_POINT('Ctrl Pts',(-34.3610247157663,-10.8035158666735,
34.1377871350208));
#17062=CARTESIAN_POINT('Ctrl Pts',(-34.3229358340806,-10.7780132627796,
34.1762252785902));
#17063=CARTESIAN_POINT('Ctrl Pts',(-34.3059237294467,-10.7666227218479,
34.1933933783451));
#17064=CARTESIAN_POINT('Ctrl Pts',(-34.2883989200401,-10.7565058951398,
34.2110531805233));
#17065=CARTESIAN_POINT('Ctrl Pts',(-34.2703785428131,-10.7476174402578,
34.2291828798374));
#17066=CARTESIAN_POINT('Ctrl Pts',(-34.2275028321476,-10.7264692248246,
34.2723186994961));
#17067=CARTESIAN_POINT('Ctrl Pts',(-34.1835721667184,-10.7131720598041,
34.3163530721274));
#17068=CARTESIAN_POINT('Ctrl Pts',(-34.1386526306351,-10.7075299712003,
34.3611985567771));
#17069=CARTESIAN_POINT('Ctrl Pts',(-34.122042545285,-10.7054436724218,34.3777812598179));
#17070=CARTESIAN_POINT('Ctrl Pts',(-34.1052971897794,-10.7044045890775,
34.3944749165526));
#17071=CARTESIAN_POINT('Ctrl Pts',(-34.088419713945,-10.7044045823054,34.4112752552593));
#17072=CARTESIAN_POINT('',(-34.585302306524,-12.8919045823054,33.9093990029365));
#17073=CARTESIAN_POINT('',(-34.585302306524,-14.7669045823054,33.9093990029365));
#17074=CARTESIAN_POINT('Origin',(0.0835265683620477,-12.8919045823054,0.0824317919394229));
#17075=CARTESIAN_POINT('',(-36.2237408786571,-5.88746284406389,32.1444613094329));
#17076=CARTESIAN_POINT('Ctrl Pts',(-35.5742461733022,-7.07886995352309,
32.8652725680806));
#17077=CARTESIAN_POINT('Ctrl Pts',(-35.5742461905474,-7.03750286915196,
32.8652725493231));
#17078=CARTESIAN_POINT('Ctrl Pts',(-35.5760044206528,-6.99633891590724,
32.863362060325));
#17079=CARTESIAN_POINT('Ctrl Pts',(-35.5792938503007,-6.95552189493502,
32.8597839374456));
#17080=CARTESIAN_POINT('Ctrl Pts',(-35.5827607190485,-6.91250311370712,
32.8560128027158));
#17081=CARTESIAN_POINT('Ctrl Pts',(-35.5879288090133,-6.86986888736257,
32.8503888771501));
#17082=CARTESIAN_POINT('Ctrl Pts',(-35.5945728456146,-6.82778372080405,
32.8431525152966));
#17083=CARTESIAN_POINT('Ctrl Pts',(-35.6017074630717,-6.78259107933759,
32.8353818366108));
#17084=CARTESIAN_POINT('Ctrl Pts',(-35.6105445405223,-6.7380302650318,32.8257512854625));
#17085=CARTESIAN_POINT('Ctrl Pts',(-35.6208438312383,-6.69431754453991,
32.8145162260134));
#17086=CARTESIAN_POINT('Ctrl Pts',(-35.6227946757033,-6.68603768127784,
32.8123881325218));
#17087=CARTESIAN_POINT('Ctrl Pts',(-35.6247980718656,-6.67778831509133,
32.8102023731186));
#17088=CARTESIAN_POINT('Ctrl Pts',(-35.6268525024301,-6.66957102631489,
32.807960556045));
#17089=CARTESIAN_POINT('Ctrl Pts',(-35.6269399263545,-6.66922134906351,
32.8078651581037));
#17090=CARTESIAN_POINT('Ctrl Pts',(-35.6270274407123,-6.66887173803708,
32.8077696608134));
#17091=CARTESIAN_POINT('Ctrl Pts',(-35.6271150453592,-6.6685221934126,32.8076740643278));
#17092=CARTESIAN_POINT('Ctrl Pts',(-35.6522048178754,-6.56841340442319,
32.7802954473215));
#17093=CARTESIAN_POINT('Ctrl Pts',(-35.6848608854292,-6.47280389883387,
32.7446034716752));
#17094=CARTESIAN_POINT('Ctrl Pts',(-35.7243443623766,-6.38345298969106,
32.7012583566614));
#17095=CARTESIAN_POINT('Ctrl Pts',(-35.7361066934472,-6.35683489381763,
32.6883456237284));
#17096=CARTESIAN_POINT('Ctrl Pts',(-35.7484751158299,-6.33077245142131,
32.6747534913653));
#17097=CARTESIAN_POINT('Ctrl Pts',(-35.7614305154779,-6.30531282539103,
32.6604989221267));
#17098=CARTESIAN_POINT('Ctrl Pts',(-35.7616616260539,-6.30485865269114,
32.6602446357445));
#17099=CARTESIAN_POINT('Ctrl Pts',(-35.7618929228611,-6.3044046736758,32.6599901391734));
#17100=CARTESIAN_POINT('Ctrl Pts',(-35.7621244057861,-6.30395088860763,
32.6597354325154));
#17101=CARTESIAN_POINT('Ctrl Pts',(-35.7976459149302,-6.23431667928829,
32.6206501959543));
#17102=CARTESIAN_POINT('Ctrl Pts',(-35.8367531956665,-6.17022875422762,
32.5775022926724));
#17103=CARTESIAN_POINT('Ctrl Pts',(-35.8803413149544,-6.11310220427935,
32.5291872149407));
#17104=CARTESIAN_POINT('Ctrl Pts',(-35.9060289575148,-6.07943600303571,
32.500713849553));
#17105=CARTESIAN_POINT('Ctrl Pts',(-35.9332732469221,-6.04818793999518,
32.4704454107571));
#17106=CARTESIAN_POINT('Ctrl Pts',(-35.9622619599609,-6.01965292485596,
32.4381505401005));
#17107=CARTESIAN_POINT('Ctrl Pts',(-35.9625476299596,-6.01937172583458,
32.4378322894888));
#17108=CARTESIAN_POINT('Ctrl Pts',(-35.9628334737629,-6.01909078646767,
32.4375138371825));
#17109=CARTESIAN_POINT('Ctrl Pts',(-35.9631194915227,-6.01881010710761,
32.4371951829905));
#17110=CARTESIAN_POINT('Ctrl Pts',(-35.9944691963256,-5.98804553120513,
32.4022682789445));
#17111=CARTESIAN_POINT('Ctrl Pts',(-36.0275206206836,-5.96083151819991,
32.3653395143693));
#17112=CARTESIAN_POINT('Ctrl Pts',(-36.0618832816626,-5.93928082321596,
32.3268185345682));
#17113=CARTESIAN_POINT('Ctrl Pts',(-36.0900646290595,-5.92160676641468,
32.2952268858741));
#17114=CARTESIAN_POINT('Ctrl Pts',(-36.119127144603,-5.90774301103966,32.2625651728106));
#17115=CARTESIAN_POINT('Ctrl Pts',(-36.1488454697205,-5.89882514864856,
32.229071245035));
#17116=CARTESIAN_POINT('Ctrl Pts',(-36.1734061046961,-5.89145500372673,
32.2013902727479));
#17117=CARTESIAN_POINT('Ctrl Pts',(-36.1984144339698,-5.88746290319468,
32.1731411533038));
#17118=CARTESIAN_POINT('Ctrl Pts',(-36.2237408786571,-5.8874628440639,32.1444613094329));
#17119=CARTESIAN_POINT('',(-48.170424664145,-5.88746284406388,4.2952214497352));
#17120=CARTESIAN_POINT('Origin',(0.0835265683620477,-5.88746284406389,0.0824317919394229));
#17121=CARTESIAN_POINT('',(-48.3539734316379,-5.88746284406389,0.0824317919393457));
#17122=CARTESIAN_POINT('Origin',(0.083526568354122,-5.88746284406389,0.0824317919399243));
#17123=CARTESIAN_POINT('',(-48.170424664145,-5.8874628440639,-4.13035786585653));
#17124=CARTESIAN_POINT('Origin',(0.0835265683638564,-5.88746284406038,0.0824317919403333));
#17125=CARTESIAN_POINT('',(-39.9103854094111,-5.8874628440639,-27.2429851484136));
#17126=CARTESIAN_POINT('Origin',(0.0835265683620477,-5.8874628440639,0.0824317919394229));
#17127=CARTESIAN_POINT('',(-39.6144733390877,-6.59535043767467,-27.6711303145384));
#17128=CARTESIAN_POINT('Ctrl Pts',(-39.6144733390877,-6.59535043767467,
-27.6711303145384));
#17129=CARTESIAN_POINT('Ctrl Pts',(-39.6144733390877,-6.57489151419421,
-27.6711303145384));
#17130=CARTESIAN_POINT('Ctrl Pts',(-39.6147776823602,-6.55450357765519,
-27.6706968159101));
#17131=CARTESIAN_POINT('Ctrl Pts',(-39.6154006901076,-6.53419088775615,
-27.6698080919584));
#17132=CARTESIAN_POINT('Ctrl Pts',(-39.6162474678158,-6.50658234986474,
-27.6686001589365));
#17133=CARTESIAN_POINT('Ctrl Pts',(-39.617698057498,-6.47911098112832,-27.6665296330311));
#17134=CARTESIAN_POINT('Ctrl Pts',(-39.6197804179767,-6.45179259386993,
-27.6635536475747));
#17135=CARTESIAN_POINT('Ctrl Pts',(-39.6217608263548,-6.42581171132876,
-27.6607233659824));
#17136=CARTESIAN_POINT('Ctrl Pts',(-39.6243124829563,-6.3999680626771,-27.6570743822144));
#17137=CARTESIAN_POINT('Ctrl Pts',(-39.6274859772415,-6.37426951907271,
-27.6525318044936));
#17138=CARTESIAN_POINT('Ctrl Pts',(-39.6283408096446,-6.36734719755199,
-27.6513081871555));
#17139=CARTESIAN_POINT('Ctrl Pts',(-39.6292409251903,-6.36043542154385,
-27.6500194971424));
#17140=CARTESIAN_POINT('Ctrl Pts',(-39.6301876923705,-6.35353442314531,
-27.6486637252585));
#17141=CARTESIAN_POINT('Ctrl Pts',(-39.6315472422071,-6.3436246465487,-27.6467168480518));
#17142=CARTESIAN_POINT('Ctrl Pts',(-39.6329994835012,-6.33375626741061,
-27.6446366635865));
#17143=CARTESIAN_POINT('Ctrl Pts',(-39.6345478454677,-6.32393813773167,
-27.6424181254434));
#17144=CARTESIAN_POINT('Ctrl Pts',(-39.6405058326386,-6.2861586701808,-27.6338813478158));
#17145=CARTESIAN_POINT('Ctrl Pts',(-39.6478827413411,-6.24912973387886,
-27.623302215804));
#17146=CARTESIAN_POINT('Ctrl Pts',(-39.6568831236509,-6.21334185680268,
-27.6103800269361));
#17147=CARTESIAN_POINT('Ctrl Pts',(-39.6642558795785,-6.18402584846371,
-27.599794682748));
#17148=CARTESIAN_POINT('Ctrl Pts',(-39.6727178645552,-6.15554336972683,
-27.5876373021568));
#17149=CARTESIAN_POINT('Ctrl Pts',(-39.6823698141691,-6.12818087652871,
-27.5737590369931));
#17150=CARTESIAN_POINT('Ctrl Pts',(-39.6824170164226,-6.12804706197382,
-27.5736911662087));
#17151=CARTESIAN_POINT('Ctrl Pts',(-39.6824642467499,-6.127913273277,-27.5736232548215));
#17152=CARTESIAN_POINT('Ctrl Pts',(-39.6825115051614,-6.12777951046925,
-27.5735553028158));
#17153=CARTESIAN_POINT('Ctrl Pts',(-39.6991446911241,-6.0807000259069,-27.5496387489013));
#17154=CARTESIAN_POINT('Ctrl Pts',(-39.7195743313313,-6.03703191460944,
-27.5202190561252));
#17155=CARTESIAN_POINT('Ctrl Pts',(-39.7432460113709,-6.00042962268924,
-27.4860214316161));
#17156=CARTESIAN_POINT('Ctrl Pts',(-39.7544113877206,-5.98316517995156,
-27.4698912141044));
#17157=CARTESIAN_POINT('Ctrl Pts',(-39.7662980350091,-5.96747341994775,
-27.4526980155051));
#17158=CARTESIAN_POINT('Ctrl Pts',(-39.7788476275594,-5.95374197151949,
-27.4345180702209));
#17159=CARTESIAN_POINT('Ctrl Pts',(-39.7789372501968,-5.95364390868447,
-27.434388238544));
#17160=CARTESIAN_POINT('Ctrl Pts',(-39.7790269045611,-5.95354594807965,
-27.4342583595609));
#17161=CARTESIAN_POINT('Ctrl Pts',(-39.7791165906397,-5.95344808981835,
-27.4341284332866));
#17162=CARTESIAN_POINT('Ctrl Pts',(-39.7915148574324,-5.93992009473035,
-27.4161673334697));
#17163=CARTESIAN_POINT('Ctrl Pts',(-39.8045723203378,-5.92838288345103,
-27.3972221945806));
#17164=CARTESIAN_POINT('Ctrl Pts',(-39.8180958333997,-5.91890173045759,
-27.3775697308246));
#17165=CARTESIAN_POINT('Ctrl Pts',(-39.831624273665,-5.90941712306821,-27.3579101068224));
#17166=CARTESIAN_POINT('Ctrl Pts',(-39.845619976459,-5.90198963169007,-27.3375413906112));
#17167=CARTESIAN_POINT('Ctrl Pts',(-39.8598996395668,-5.89673275177899,
-27.3167252760599));
#17168=CARTESIAN_POINT('Ctrl Pts',(-39.8735587895391,-5.89170430604118,
-27.2968137117359));
#17169=CARTESIAN_POINT('Ctrl Pts',(-39.8874784944817,-5.88866186035204,
-27.2764917245678));
#17170=CARTESIAN_POINT('Ctrl Pts',(-39.9014958338896,-5.88775186306256,
-27.2559911519314));
#17171=CARTESIAN_POINT('Ctrl Pts',(-39.9044552363665,-5.88755974042401,
-27.2516629806806));
#17172=CARTESIAN_POINT('Ctrl Pts',(-39.90741895973,-5.88746284473756,-27.2473268910371));
#17173=CARTESIAN_POINT('Ctrl Pts',(-39.9103854094107,-5.88746284406391,
-27.2429851484142));
#17174=CARTESIAN_POINT('',(-39.6144733390877,-12.8919045823054,-27.6711303145384));
#17175=CARTESIAN_POINT('',(-39.6144733390877,-14.7669045823054,-27.6711303145384));
#17176=CARTESIAN_POINT('Origin',(0.0835265683620477,-12.8919045823054,0.0824317919394229));
#17177=CARTESIAN_POINT('',(-38.1247730056117,-10.7044045823054,-29.6886489730492));
#17178=CARTESIAN_POINT('Ctrl Pts',(-38.1247730056117,-10.7044045823054,
-29.6886489730492));
#17179=CARTESIAN_POINT('Ctrl Pts',(-38.1475082420184,-10.7044045890531,
-29.6594704984628));
#17180=CARTESIAN_POINT('Ctrl Pts',(-38.1701613733944,-10.7074293129562,
-29.6303167919518));
#17181=CARTESIAN_POINT('Ctrl Pts',(-38.1924666408307,-10.7132787489585,
-29.6015453903178));
#17182=CARTESIAN_POINT('Ctrl Pts',(-38.2162817881541,-10.7195241428122,
-29.57082640564));
#17183=CARTESIAN_POINT('Ctrl Pts',(-38.2397011476956,-10.7289894494735,
-29.5405422294129));
#17184=CARTESIAN_POINT('Ctrl Pts',(-38.262412155705,-10.741487141963,-29.5111121734136));
#17185=CARTESIAN_POINT('Ctrl Pts',(-38.2853015195902,-10.754082982315,-29.481450994982));
#17186=CARTESIAN_POINT('Ctrl Pts',(-38.3074723367097,-10.7697593965528,
-29.4526561087291));
#17187=CARTESIAN_POINT('Ctrl Pts',(-38.328601710441,-10.788376919345,-29.425159248585));
#17188=CARTESIAN_POINT('Ctrl Pts',(-38.3488622104619,-10.806228859763,-29.3987931033972));
#17189=CARTESIAN_POINT('Ctrl Pts',(-38.3681658981275,-10.8267856372082,
-29.3736194310045));
#17190=CARTESIAN_POINT('Ctrl Pts',(-38.3862130647491,-10.8499643578044,
-29.3500376580405));
#17191=CARTESIAN_POINT('Ctrl Pts',(-38.3937576510098,-10.8596541811777,
-29.3401793393339));
#17192=CARTESIAN_POINT('Ctrl Pts',(-38.4010823947021,-10.8698026686922,
-29.3305995430489));
#17193=CARTESIAN_POINT('Ctrl Pts',(-38.4081641147974,-10.8804055842374,
-29.321329099185));
#17194=CARTESIAN_POINT('Ctrl Pts',(-38.4082595399778,-10.8805484570303,
-29.3212041812602));
#17195=CARTESIAN_POINT('Ctrl Pts',(-38.4083549194988,-10.8806914099898,
-29.3210793215119));
#17196=CARTESIAN_POINT('Ctrl Pts',(-38.4084502533016,-10.8808344430917,
-29.3209545200184));
#17197=CARTESIAN_POINT('Ctrl Pts',(-38.4254589362055,-10.9063532475959,
-29.2986884510284));
#17198=CARTESIAN_POINT('Ctrl Pts',(-38.4410024861526,-10.9345143821538,
-29.2783052843817));
#17199=CARTESIAN_POINT('Ctrl Pts',(-38.4548797362525,-10.9647671393856,
-29.2600841616223));
#17200=CARTESIAN_POINT('Ctrl Pts',(-38.4721325948409,-11.0023788087487,
-29.2374307935541));
#17201=CARTESIAN_POINT('Ctrl Pts',(-38.4868128584692,-11.0432205203777,
-29.2181153587633));
#17202=CARTESIAN_POINT('Ctrl Pts',(-38.4985391336244,-11.0862730505896,
-29.2026673761867));
#17203=CARTESIAN_POINT('Ctrl Pts',(-38.50891537767,-11.1243689978829,-29.1889979001506));
#17204=CARTESIAN_POINT('Ctrl Pts',(-38.5169798539052,-11.1641988556004,
-29.1783550284388));
#17205=CARTESIAN_POINT('Ctrl Pts',(-38.5224491968758,-11.2050768635585,
-29.1711308904909));
#17206=CARTESIAN_POINT('Ctrl Pts',(-38.5278860651363,-11.2457121547105,
-29.1639496465043));
#17207=CARTESIAN_POINT('Ctrl Pts',(-38.5307586790751,-11.2873849299234,
-29.1601464302277));
#17208=CARTESIAN_POINT('Ctrl Pts',(-38.5307586915594,-11.3294045823054,
-29.1601464137424));
#17209=CARTESIAN_POINT('',(-34.2453168949582,-10.7044045823054,-34.0895144903672));
#17210=CARTESIAN_POINT('Origin',(0.0835265683620477,-10.7044045823054,0.0824317919394229));
#17211=CARTESIAN_POINT('',(-33.7434406426353,-11.3294045823054,-34.5863970829463));
#17212=CARTESIAN_POINT('Ctrl Pts',(-33.7434406426353,-11.3294045823054,
-34.5863970829463));
#17213=CARTESIAN_POINT('Ctrl Pts',(-33.7434406426353,-11.2968266539592,
-34.5863970829463));
#17214=CARTESIAN_POINT('Ctrl Pts',(-33.7454847777487,-11.2645751883002,
-34.5844047435613));
#17215=CARTESIAN_POINT('Ctrl Pts',(-33.7494936592074,-11.2329045289636,
-34.5804924934159));
#17216=CARTESIAN_POINT('Ctrl Pts',(-33.7536016859333,-11.2004506097536,
-34.5764834878312));
#17217=CARTESIAN_POINT('Ctrl Pts',(-33.7597726891855,-11.1686071890505,
-34.5704585666387));
#17218=CARTESIAN_POINT('Ctrl Pts',(-33.767882341873,-11.137638677352,-34.56253360839));
#17219=CARTESIAN_POINT('Ctrl Pts',(-33.7732201625828,-11.1172550222851,
-34.5573173546374));
#17220=CARTESIAN_POINT('Ctrl Pts',(-33.7793970738421,-11.0972501995398,
-34.5512787192884));
#17221=CARTESIAN_POINT('Ctrl Pts',(-33.7863693688805,-11.0776955263552,
-34.5444588488597));
#17222=CARTESIAN_POINT('Ctrl Pts',(-33.7864893126861,-11.0773591289561,
-34.544341527202));
#17223=CARTESIAN_POINT('Ctrl Pts',(-33.7866094630912,-11.0770229370417,
-34.5442240023173));
#17224=CARTESIAN_POINT('Ctrl Pts',(-33.786729819816,-11.0766869507352,-34.5441062744646));
#17225=CARTESIAN_POINT('Ctrl Pts',(-33.8022773598336,-11.0332846351901,
-34.5288983290528));
#17226=CARTESIAN_POINT('Ctrl Pts',(-33.8213000908315,-10.9932074809924,
-34.5102718127948));
#17227=CARTESIAN_POINT('Ctrl Pts',(-33.843357849581,-10.9565169212052,-34.4886249102596));
#17228=CARTESIAN_POINT('Ctrl Pts',(-33.8609994737114,-10.9271720964544,
-34.4713118857385));
#17229=CARTESIAN_POINT('Ctrl Pts',(-33.8805833998321,-10.8999941023351,
-34.4520659626183));
#17230=CARTESIAN_POINT('Ctrl Pts',(-33.9018981598468,-10.8750283402102,
-34.431077335514));
#17231=CARTESIAN_POINT('Ctrl Pts',(-33.9021320889446,-10.8747543414317,
-34.4308469857189));
#17232=CARTESIAN_POINT('Ctrl Pts',(-33.9023661565204,-10.8744806828913,
-34.4306164948919));
#17233=CARTESIAN_POINT('Ctrl Pts',(-33.9026003625033,-10.8742073644076,
-34.4303858630855));
#17234=CARTESIAN_POINT('Ctrl Pts',(-33.9358541806131,-10.8354001442444,
-34.3976395256663));
#17235=CARTESIAN_POINT('Ctrl Pts',(-33.9718287747473,-10.8035158666488,
-34.3621194921614));
#17236=CARTESIAN_POINT('Ctrl Pts',(-34.0102669183332,-10.77801326275,-34.3240306104592));
#17237=CARTESIAN_POINT('Ctrl Pts',(-34.0274350180743,-10.7666227218303,
-34.307018505839));
#17238=CARTESIAN_POINT('Ctrl Pts',(-34.0450948202377,-10.7565058951319,
-34.2894936964469));
#17239=CARTESIAN_POINT('Ctrl Pts',(-34.0632245195362,-10.7476174402576,
-34.2714733192354));
#17240=CARTESIAN_POINT('Ctrl Pts',(-34.1063603392022,-10.726469224821,-34.2285976085627));
#17241=CARTESIAN_POINT('Ctrl Pts',(-34.1503947118412,-10.7131720597996,
-34.1846669431258));
#17242=CARTESIAN_POINT('Ctrl Pts',(-34.1952401964989,-10.7075299711974,
-34.1397474070344));
#17243=CARTESIAN_POINT('Ctrl Pts',(-34.2118228995322,-10.7054436724208,
-34.1231373216918));
#17244=CARTESIAN_POINT('Ctrl Pts',(-34.2285165562592,-10.7044045890775,
-34.1063919661939));
#17245=CARTESIAN_POINT('Ctrl Pts',(-34.2453168949582,-10.7044045823054,
-34.0895144903673));
#17246=CARTESIAN_POINT('',(-33.7434406426353,-12.8919045823054,-34.5863970829463));
#17247=CARTESIAN_POINT('',(-33.7434406426353,-14.7669045823054,-34.5863970829463));
#17248=CARTESIAN_POINT('',(-32.6993142077795,-12.8919045823054,-35.5753409497245));
#17249=CARTESIAN_POINT('Origin',(0.0835265683620477,-12.8919045823054,0.0824317919394229));
#17250=CARTESIAN_POINT('',(-32.6993142077795,-7.07886995352309,-35.5753409497245));
#17251=CARTESIAN_POINT('',(-32.6993142077795,-14.7669045823054,-35.5753409497245));
#17252=CARTESIAN_POINT('',(-31.9785029491318,-5.88746284406389,-36.2248356550794));
#17253=CARTESIAN_POINT('Ctrl Pts',(-32.6993142077795,-7.07886995352308,
-35.5753409497245));
#17254=CARTESIAN_POINT('Ctrl Pts',(-32.6993141890216,-7.03750286914987,
-35.57534096697));
#17255=CARTESIAN_POINT('Ctrl Pts',(-32.6974037000232,-6.99633891590311,
-35.5770991970757));
#17256=CARTESIAN_POINT('Ctrl Pts',(-32.6938255771434,-6.95552189492887,
-35.5803886267239));
#17257=CARTESIAN_POINT('Ctrl Pts',(-32.6900544424132,-6.91250311369896,
-35.5838554954721));
#17258=CARTESIAN_POINT('Ctrl Pts',(-32.6844305168472,-6.86986888735245,
-35.5890235854372));
#17259=CARTESIAN_POINT('Ctrl Pts',(-32.6771941549931,-6.82778372079203,
-35.595667622039));
#17260=CARTESIAN_POINT('Ctrl Pts',(-32.6694234763069,-6.78259107932476,
-35.6028022394964));
#17261=CARTESIAN_POINT('Ctrl Pts',(-32.6597929251584,-6.7380302650182,-35.6116393169474));
#17262=CARTESIAN_POINT('Ctrl Pts',(-32.6485578657088,-6.6943175445256,-35.6219386076638));
#17263=CARTESIAN_POINT('Ctrl Pts',(-32.6464297722183,-6.68603768126831,
-35.6238894521278));
#17264=CARTESIAN_POINT('Ctrl Pts',(-32.6442440128163,-6.67778831508655,
-35.6258928482889));
#17265=CARTESIAN_POINT('Ctrl Pts',(-32.642002195744,-6.66957102631483,-35.6279472788522));
#17266=CARTESIAN_POINT('Ctrl Pts',(-32.6419067978027,-6.66922134906346,
-35.6280347027766));
#17267=CARTESIAN_POINT('Ctrl Pts',(-32.6418113005124,-6.66887173803703,
-35.6281222171344));
#17268=CARTESIAN_POINT('Ctrl Pts',(-32.6417157040268,-6.66852219341255,
-35.6282098217813));
#17269=CARTESIAN_POINT('Ctrl Pts',(-32.6143370871273,-6.56841340481339,
-35.6532995941997));
#17270=CARTESIAN_POINT('Ctrl Pts',(-32.5786451116525,-6.47280389957943,
-35.6859556615968));
#17271=CARTESIAN_POINT('Ctrl Pts',(-32.5352999968674,-6.38345299073607,
-35.725439138337));
#17272=CARTESIAN_POINT('Ctrl Pts',(-32.5223872637832,-6.35683489449971,
-35.7372014695457));
#17273=CARTESIAN_POINT('Ctrl Pts',(-32.5087951312509,-6.33077245175437,
-35.7495698920825));
#17274=CARTESIAN_POINT('Ctrl Pts',(-32.4945405618258,-6.30531282539085,
-35.7625252919));
#17275=CARTESIAN_POINT('Ctrl Pts',(-32.4942862754435,-6.30485865269096,
-35.762756402476));
#17276=CARTESIAN_POINT('Ctrl Pts',(-32.4940317788724,-6.30440467367563,
-35.7629876992832));
#17277=CARTESIAN_POINT('Ctrl Pts',(-32.4937770722144,-6.30395088860745,
-35.7632191822082));
#17278=CARTESIAN_POINT('Ctrl Pts',(-32.4546918357289,-6.23431667942218,
-35.7987406912838));
#17279=CARTESIAN_POINT('Ctrl Pts',(-32.4115439325377,-6.17022875447443,
-35.8378479719379));
#17280=CARTESIAN_POINT('Ctrl Pts',(-32.3632288549189,-6.11310220460954,
-35.8814360911247));
#17281=CARTESIAN_POINT('Ctrl Pts',(-32.3347554894498,-6.0794360032401,-35.9071237337589));
#17282=CARTESIAN_POINT('Ctrl Pts',(-32.3044870505616,-6.04818794008861,
-35.9343680232496));
#17283=CARTESIAN_POINT('Ctrl Pts',(-32.2721921797993,-6.01965292485617,
-35.9633567363832));
#17284=CARTESIAN_POINT('Ctrl Pts',(-32.2718739291876,-6.01937172583479,
-35.9636424063819));
#17285=CARTESIAN_POINT('Ctrl Pts',(-32.2715554768813,-6.01909078646788,
-35.9639282501853));
#17286=CARTESIAN_POINT('Ctrl Pts',(-32.2712368226893,-6.01881010710782,
-35.9642142679451));
#17287=CARTESIAN_POINT('Ctrl Pts',(-32.2363099186584,-5.98804553121875,
-35.9955639727344));
#17288=CARTESIAN_POINT('Ctrl Pts',(-32.1993811541001,-5.9608315182235,-36.0286153970774));
#17289=CARTESIAN_POINT('Ctrl Pts',(-32.1608601743171,-5.93928082324375,
-36.0629780580403));
#17290=CARTESIAN_POINT('Ctrl Pts',(-32.1292685256388,-5.92160676644647,
-36.0911594054232));
#17291=CARTESIAN_POINT('Ctrl Pts',(-32.096606812592,-5.90774301107131,-36.120221920952));
#17292=CARTESIAN_POINT('Ctrl Pts',(-32.0631128848336,-5.89882514867459,
-36.1499402460543));
#17293=CARTESIAN_POINT('Ctrl Pts',(-32.0354319125146,-5.89145500373582,
-36.1745008810583));
#17294=CARTESIAN_POINT('Ctrl Pts',(-32.0071827930371,-5.88746290319435,
-36.1995092103617));
#17295=CARTESIAN_POINT('Ctrl Pts',(-31.9785029491318,-5.88746284406389,
-36.2248356550794));
#17296=CARTESIAN_POINT('',(-4.12926308943377,-5.88746284406389,-48.1715194405676));
#17297=CARTESIAN_POINT('Origin',(0.0835265683620477,-5.88746284406389,0.0824317919394229));
#17298=CARTESIAN_POINT('',(0.0835265683620358,-5.88746284406389,-48.3550682080606));
#17299=CARTESIAN_POINT('Origin',(0.0835265683620358,-5.88746284406389,0.0824317919239981));
#17300=CARTESIAN_POINT('',(4.29631622615797,-5.88746284406389,-48.1715194405676));
#17301=CARTESIAN_POINT('Origin',(0.0835265683614989,-5.88746284406448,0.0824317919478901));
#17302=CARTESIAN_POINT('',(27.4089435087152,-5.88746284406389,-39.9114801858336));
#17303=CARTESIAN_POINT('Origin',(0.0835265683620477,-5.88746284406389,0.0824317919394229));
#17304=CARTESIAN_POINT('',(27.83708867484,-6.59535043767467,-39.6155681155102));
#17305=CARTESIAN_POINT('Ctrl Pts',(27.83708867484,-6.59535043767467,-39.6155681155102));
#17306=CARTESIAN_POINT('Ctrl Pts',(27.83708867484,-6.57489151419422,-39.6155681155102));
#17307=CARTESIAN_POINT('Ctrl Pts',(27.836655176211,-6.55450357765523,-39.6158724587832));
#17308=CARTESIAN_POINT('Ctrl Pts',(27.8357664522595,-6.53419088775619,-39.6164954665305));
#17309=CARTESIAN_POINT('Ctrl Pts',(27.8345585192379,-6.50658234986769,-39.6173422442385));
#17310=CARTESIAN_POINT('Ctrl Pts',(27.832487993333,-6.47911098113413,-39.6187928339203));
#17311=CARTESIAN_POINT('Ctrl Pts',(27.8295120078771,-6.45179259387858,-39.6208751943986));
#17312=CARTESIAN_POINT('Ctrl Pts',(27.8266817262854,-6.42581171133972,-39.6228556027764));
#17313=CARTESIAN_POINT('Ctrl Pts',(27.823032742518,-6.39996806269036,-39.6254072593775));
#17314=CARTESIAN_POINT('Ctrl Pts',(27.8184901647979,-6.37426951908824,-39.6285807536621));
#17315=CARTESIAN_POINT('Ctrl Pts',(27.8172665474591,-6.36734719756233,-39.6294355860658));
#17316=CARTESIAN_POINT('Ctrl Pts',(27.815977857445,-6.36043542154902,-39.6303357016121));
#17317=CARTESIAN_POINT('Ctrl Pts',(27.8146220855601,-6.35353442314532,-39.631282468793));
#17318=CARTESIAN_POINT('Ctrl Pts',(27.8126752083534,-6.34362464654871,-39.6326420186297));
#17319=CARTESIAN_POINT('Ctrl Pts',(27.8105950238881,-6.33375626741062,-39.6340942599238));
#17320=CARTESIAN_POINT('Ctrl Pts',(27.808376485745,-6.32393813773167,-39.6356426218902));
#17321=CARTESIAN_POINT('Ctrl Pts',(27.7998397081135,-6.28615867016339,-39.6416006090639));
#17322=CARTESIAN_POINT('Ctrl Pts',(27.7892605760959,-6.24912973384469,-39.6489775177705));
#17323=CARTESIAN_POINT('Ctrl Pts',(27.7763383872198,-6.21334185675317,-39.6579779000859));
#17324=CARTESIAN_POINT('Ctrl Pts',(27.7657530430359,-6.18402584843166,-39.6653506560106));
#17325=CARTESIAN_POINT('Ctrl Pts',(27.7535956624506,-6.15554336971148,-39.6738126409832));
#17326=CARTESIAN_POINT('Ctrl Pts',(27.7397173972946,-6.1281808765288,-39.6834645905917));
#17327=CARTESIAN_POINT('Ctrl Pts',(27.7396495265103,-6.1280470619739,-39.6835117928452));
#17328=CARTESIAN_POINT('Ctrl Pts',(27.739581615123,-6.12791327327708,-39.6835590231725));
#17329=CARTESIAN_POINT('Ctrl Pts',(27.7395136631173,-6.12777951046932,-39.683606281584));
#17330=CARTESIAN_POINT('Ctrl Pts',(27.7155971091982,-6.08070002589822,-39.7002394675499));
#17331=CARTESIAN_POINT('Ctrl Pts',(27.6861774164157,-6.03703191459323,-39.7206691077616));
#17332=CARTESIAN_POINT('Ctrl Pts',(27.6519797918984,-6.00042962266881,-39.7443407878068));
#17333=CARTESIAN_POINT('Ctrl Pts',(27.6358495743922,-5.98316517993923,-39.7555061641526));
#17334=CARTESIAN_POINT('Ctrl Pts',(27.6186563757994,-5.96747341994242,-39.7673928114367));
#17335=CARTESIAN_POINT('Ctrl Pts',(27.6004764305224,-5.95374197151959,-39.7799424039819));
#17336=CARTESIAN_POINT('Ctrl Pts',(27.6003465988456,-5.95364390868456,-39.7800320266193));
#17337=CARTESIAN_POINT('Ctrl Pts',(27.6002167198624,-5.95354594807974,-39.7801216809836));
#17338=CARTESIAN_POINT('Ctrl Pts',(27.6000867935882,-5.95344808981843,-39.7802113670623));
#17339=CARTESIAN_POINT('Ctrl Pts',(27.5821256937692,-5.93992009472884,-39.7926096338564));
#17340=CARTESIAN_POINT('Ctrl Pts',(27.5631805548778,-5.92838288344823,-39.8056670967633));
#17341=CARTESIAN_POINT('Ctrl Pts',(27.5435280911194,-5.91890173045397,-39.819190609827));
#17342=CARTESIAN_POINT('Ctrl Pts',(27.5238684671156,-5.90941712306419,-39.8327190500933));
#17343=CARTESIAN_POINT('Ctrl Pts',(27.5034997509027,-5.90198963168597,-39.8467147528884));
#17344=CARTESIAN_POINT('Ctrl Pts',(27.4826836363497,-5.89673275177528,-39.8609944159974));
#17345=CARTESIAN_POINT('Ctrl Pts',(27.4627720720246,-5.89170430603802,-39.8746535659704));
#17346=CARTESIAN_POINT('Ctrl Pts',(27.4424500848554,-5.88866186034975,-39.8885732709138));
#17347=CARTESIAN_POINT('Ctrl Pts',(27.421949512218,-5.88775186306162,-39.9025906103224));
#17348=CARTESIAN_POINT('Ctrl Pts',(27.4176213409719,-5.88755974042358,-39.905550012796));
#17349=CARTESIAN_POINT('Ctrl Pts',(27.4132852513333,-5.88746284473744,-39.9085137361562));
#17350=CARTESIAN_POINT('Ctrl Pts',(27.4089435087152,-5.8874628440639,-39.9114801858336));
#17351=CARTESIAN_POINT('',(27.83708867484,-12.8919045823054,-39.6155681155102));
#17352=CARTESIAN_POINT('',(27.83708867484,-14.7669045823054,-39.6155681155102));
#17353=CARTESIAN_POINT('',(29.326104774044,-12.8919045823054,-38.5318534679819));
#17354=CARTESIAN_POINT('Origin',(0.0835265683620477,-12.8919045823054,0.0824317919394229));
#17355=CARTESIAN_POINT('',(29.326104774044,-11.3294045823054,-38.5318534679819));
#17356=CARTESIAN_POINT('',(29.326104774044,-14.7669045823054,-38.5318534679819));
#17357=CARTESIAN_POINT('',(29.8546073333508,-10.7044045823054,-38.1258677820342));
#17358=CARTESIAN_POINT('Ctrl Pts',(29.8546073333508,-10.7044045823054,-38.1258677820342));
#17359=CARTESIAN_POINT('Ctrl Pts',(29.8254288587611,-10.7044045890531,-38.1486030184435));
#17360=CARTESIAN_POINT('Ctrl Pts',(29.7962751522468,-10.7074293129569,-38.171256149822));
#17361=CARTESIAN_POINT('Ctrl Pts',(29.7675037506096,-10.7132787489605,-38.1935614172609));
#17362=CARTESIAN_POINT('Ctrl Pts',(29.7367847659283,-10.7195241428156,-38.2173765645869));
#17363=CARTESIAN_POINT('Ctrl Pts',(29.7065005896978,-10.728989449479,-38.240795924131));
#17364=CARTESIAN_POINT('Ctrl Pts',(29.6770705336955,-10.7414871419714,-38.2635069321427));
#17365=CARTESIAN_POINT('Ctrl Pts',(29.6474093552607,-10.7540829823262,-38.2863962960303));
#17366=CARTESIAN_POINT('Ctrl Pts',(29.6186144690049,-10.7697593965676,-38.3085671131521));
#17367=CARTESIAN_POINT('Ctrl Pts',(29.5911176088584,-10.7883769193641,-38.3296964868852));
#17368=CARTESIAN_POINT('Ctrl Pts',(29.5647514636682,-10.8062288597864,-38.349956986908));
#17369=CARTESIAN_POINT('Ctrl Pts',(29.5395777912734,-10.8267856372365,-38.3692606745751));
#17370=CARTESIAN_POINT('Ctrl Pts',(29.515996018308,-10.8499643578382,-38.3873078411977));
#17371=CARTESIAN_POINT('Ctrl Pts',(29.5061376996133,-10.8596541812013,-38.3948524274492));
#17372=CARTESIAN_POINT('Ctrl Pts',(29.4965579033399,-10.8698026687045,-38.4021771711327));
#17373=CARTESIAN_POINT('Ctrl Pts',(29.4872874594866,-10.8804055842375,-38.4092588912199));
#17374=CARTESIAN_POINT('Ctrl Pts',(29.4871625415619,-10.8805484570304,-38.4093543164003));
#17375=CARTESIAN_POINT('Ctrl Pts',(29.4870376818136,-10.8806914099898,-38.4094496959213));
#17376=CARTESIAN_POINT('Ctrl Pts',(29.48691288032,-10.8808344430918,-38.4095450297241));
#17377=CARTESIAN_POINT('Ctrl Pts',(29.46464681133,-10.9063532475959,-38.426553712628));
#17378=CARTESIAN_POINT('Ctrl Pts',(29.4442636446832,-10.9345143821536,-38.4420972625752));
#17379=CARTESIAN_POINT('Ctrl Pts',(29.4260425219237,-10.9647671393854,-38.4559745126752));
#17380=CARTESIAN_POINT('Ctrl Pts',(29.4033891538499,-11.0023788087573,-38.4732273712679));
#17381=CARTESIAN_POINT('Ctrl Pts',(29.3840737190552,-11.0432205203968,-38.4879076348992));
#17382=CARTESIAN_POINT('Ctrl Pts',(29.3686257364766,-11.08627305062,-38.4996339100558));
#17383=CARTESIAN_POINT('Ctrl Pts',(29.3549562604386,-11.1243689979234,-38.5100101541028));
#17384=CARTESIAN_POINT('Ctrl Pts',(29.3443133887266,-11.1641988556518,-38.5180746303382));
#17385=CARTESIAN_POINT('Ctrl Pts',(29.3370892507806,-11.2050768636209,-38.5235439733073));
#17386=CARTESIAN_POINT('Ctrl Pts',(29.3299080068013,-11.2457121547532,-38.5289808415623));
#17387=CARTESIAN_POINT('Ctrl Pts',(29.3261047905288,-11.287384929945,-38.5318534554979));
#17388=CARTESIAN_POINT('Ctrl Pts',(29.326104774044,-11.3294045823054,-38.5318534679819));
#17389=CARTESIAN_POINT('',(34.2554728506688,-10.7044045823054,-34.2464116713807));
#17390=CARTESIAN_POINT('Origin',(0.0835265683620477,-10.7044045823054,0.0824317919394229));
#17391=CARTESIAN_POINT('Ctrl Pts',(34.7523554432478,-11.3294045823054,-33.7445354190578));
#17392=CARTESIAN_POINT('Ctrl Pts',(34.7523554432478,-11.2968266539615,-33.7445354190578));
#17393=CARTESIAN_POINT('Ctrl Pts',(34.7503631038632,-11.2645751883046,-33.7465795541709));
#17394=CARTESIAN_POINT('Ctrl Pts',(34.7464508537183,-11.2329045289702,-33.750588435629));
#17395=CARTESIAN_POINT('Ctrl Pts',(34.7424418481339,-11.2004506097603,-33.7546964623547));
#17396=CARTESIAN_POINT('Ctrl Pts',(34.7364169269417,-11.1686071890573,-33.7608674656065));
#17397=CARTESIAN_POINT('Ctrl Pts',(34.7284919686934,-11.1376386773589,-33.7689771182937));
#17398=CARTESIAN_POINT('Ctrl Pts',(34.7232757149404,-11.1172550222896,-33.7743149390039));
#17399=CARTESIAN_POINT('Ctrl Pts',(34.7172370795908,-11.097250199542,-33.7804918502638));
#17400=CARTESIAN_POINT('Ctrl Pts',(34.7104172091613,-11.0776955263552,-33.7874641453031));
#17401=CARTESIAN_POINT('Ctrl Pts',(34.7102998875036,-11.0773591289561,-33.7875840891086));
#17402=CARTESIAN_POINT('Ctrl Pts',(34.7101823626189,-11.0770229370417,-33.7877042395138));
#17403=CARTESIAN_POINT('Ctrl Pts',(34.7100646347662,-11.0766869507352,-33.7878245962385));
#17404=CARTESIAN_POINT('Ctrl Pts',(34.6948566893518,-11.0332846351828,-33.8033721362587));
#17405=CARTESIAN_POINT('Ctrl Pts',(34.6762301730901,-10.993207480979,-33.8223948672603));
#17406=CARTESIAN_POINT('Ctrl Pts',(34.6545832705503,-10.9565169211867,-33.8444526260146));
#17407=CARTESIAN_POINT('Ctrl Pts',(34.637270246032,-10.927172096443,-33.8620942501421));
#17408=CARTESIAN_POINT('Ctrl Pts',(34.6180243229155,-10.8999941023299,-33.8816781762591));
#17409=CARTESIAN_POINT('Ctrl Pts',(34.5970356958156,-10.8750283402102,-33.9029929362693));
#17410=CARTESIAN_POINT('Ctrl Pts',(34.5968053460205,-10.8747543414317,-33.9032268653671));
#17411=CARTESIAN_POINT('Ctrl Pts',(34.5965748551935,-10.8744806828913,-33.9034609329429));
#17412=CARTESIAN_POINT('Ctrl Pts',(34.5963442233871,-10.8742073644076,-33.9036951389258));
#17413=CARTESIAN_POINT('Ctrl Pts',(34.5635978859542,-10.8354001442282,-33.9369489570494));
#17414=CARTESIAN_POINT('Ctrl Pts',(34.5280778524334,-10.8035158666223,-33.9729235511997));
#17415=CARTESIAN_POINT('Ctrl Pts',(34.4899889707131,-10.7780132627181,-34.0113616948038));
#17416=CARTESIAN_POINT('Ctrl Pts',(34.4729768661079,-10.7666227218115,-34.0285297945297));
#17417=CARTESIAN_POINT('Ctrl Pts',(34.4554520567317,-10.7565058951237,-34.0461895966771));
#17418=CARTESIAN_POINT('Ctrl Pts',(34.437431679537,-10.7476174402577,-34.0643192959587));
#17419=CARTESIAN_POINT('Ctrl Pts',(34.3945559688426,-10.7264692248103,-34.1074551156465));
#17420=CARTESIAN_POINT('Ctrl Pts',(34.3506253033834,-10.7131720597862,-34.1514894883078));
#17421=CARTESIAN_POINT('Ctrl Pts',(34.3057057672688,-10.707529971189,-34.1963349729886));
#17422=CARTESIAN_POINT('Ctrl Pts',(34.2890956819482,-10.705443672418,-34.2129176759997));
#17423=CARTESIAN_POINT('Ctrl Pts',(34.2723503264727,-10.7044045890775,-34.2296113327044));
#17424=CARTESIAN_POINT('Ctrl Pts',(34.2554728506688,-10.7044045823054,-34.2464116713807));
#17425=CARTESIAN_POINT('',(35.7412993100261,-12.8919045823054,-32.700408984202));
#17426=CARTESIAN_POINT('Origin',(0.0835265683620477,-12.8919045823054,0.0824317919394229));
#17427=CARTESIAN_POINT('',(35.7412993100261,-7.07886995352309,-32.700408984202));
#17428=CARTESIAN_POINT('',(35.7412993100261,-14.7669045823054,-32.700408984202));
#17429=CARTESIAN_POINT('',(36.390794015381,-5.88746284406389,-31.9795977255543));
#17430=CARTESIAN_POINT('Ctrl Pts',(35.7412993100261,-7.0788699535231,-32.700408984202));
#17431=CARTESIAN_POINT('Ctrl Pts',(35.7412993272714,-7.03750286915156,-32.7004089654444));
#17432=CARTESIAN_POINT('Ctrl Pts',(35.7430575573768,-6.99633891590645,-32.6984984764463));
#17433=CARTESIAN_POINT('Ctrl Pts',(35.7463469870247,-6.95552189493383,-32.6949203535668));
#17434=CARTESIAN_POINT('Ctrl Pts',(35.7498138557726,-6.91250311370568,-32.6911492188369));
#17435=CARTESIAN_POINT('Ctrl Pts',(35.7549819457374,-6.8698688873609,-32.6855252932712));
#17436=CARTESIAN_POINT('Ctrl Pts',(35.7616259823388,-6.82778372080215,-32.6782889314176));
#17437=CARTESIAN_POINT('Ctrl Pts',(35.7687605997959,-6.78259107933578,-32.6705182527317));
#17438=CARTESIAN_POINT('Ctrl Pts',(35.7775976772465,-6.73803026503009,-32.6608877015835));
#17439=CARTESIAN_POINT('Ctrl Pts',(35.7878969679625,-6.69431754453829,-32.6496526421344));
#17440=CARTESIAN_POINT('Ctrl Pts',(35.7898478124275,-6.68603768127677,-32.6475245486429));
#17441=CARTESIAN_POINT('Ctrl Pts',(35.7918512085896,-6.6777883150908,-32.6453387892399));
#17442=CARTESIAN_POINT('Ctrl Pts',(35.7939056391539,-6.6695710263149,-32.6430969721664));
#17443=CARTESIAN_POINT('Ctrl Pts',(35.7939930630783,-6.66922134906352,-32.6430015742251));
#17444=CARTESIAN_POINT('Ctrl Pts',(35.7940805774361,-6.66887173803709,-32.6429060769348));
#17445=CARTESIAN_POINT('Ctrl Pts',(35.794168182083,-6.66852219341261,-32.6428104804492));
#17446=CARTESIAN_POINT('Ctrl Pts',(35.8192579545976,-6.56841340442999,-32.6154318634447));
#17447=CARTESIAN_POINT('Ctrl Pts',(35.8519140221486,-6.47280389884689,-32.5797398878015));
#17448=CARTESIAN_POINT('Ctrl Pts',(35.8913974990923,-6.38345298970913,-32.5363947727917));
#17449=CARTESIAN_POINT('Ctrl Pts',(35.9031598301653,-6.35683489382933,-32.5234820398561));
#17450=CARTESIAN_POINT('Ctrl Pts',(35.9155282525506,-6.33077245142688,-32.5098899074902));
#17451=CARTESIAN_POINT('Ctrl Pts',(35.9284836522014,-6.30531282539074,-32.4956353382484));
#17452=CARTESIAN_POINT('Ctrl Pts',(35.9287147627774,-6.30485865269084,-32.4953810518661));
#17453=CARTESIAN_POINT('Ctrl Pts',(35.9289460595847,-6.30440467367551,-32.495126555295));
#17454=CARTESIAN_POINT('Ctrl Pts',(35.9291775425096,-6.30395088860734,-32.4948718486371));
#17455=CARTESIAN_POINT('Ctrl Pts',(35.9646990516115,-6.23431667937041,-32.4557866121226));
#17456=CARTESIAN_POINT('Ctrl Pts',(36.0038063322973,-6.17022875437937,-32.4126387088964));
#17457=CARTESIAN_POINT('Ctrl Pts',(36.047394451523,-6.1131022044825,-32.3643236312342));
#17458=CARTESIAN_POINT('Ctrl Pts',(36.0730820941289,-6.07943600316146,-32.3358502657963));
#17459=CARTESIAN_POINT('Ctrl Pts',(36.1003263835876,-6.04818794005264,-32.3055818269435));
#17460=CARTESIAN_POINT('Ctrl Pts',(36.1293150966848,-6.019652924856,-32.2732869562219));
#17461=CARTESIAN_POINT('Ctrl Pts',(36.1296007666834,-6.01937172583463,-32.2729687056102));
#17462=CARTESIAN_POINT('Ctrl Pts',(36.1298866104868,-6.01909078646772,-32.2726502533039));
#17463=CARTESIAN_POINT('Ctrl Pts',(36.1301726282466,-6.01881010710765,-32.2723315991119));
#17464=CARTESIAN_POINT('Ctrl Pts',(36.1615223330518,-5.98804553120297,-32.2374046950633));
#17465=CARTESIAN_POINT('Ctrl Pts',(36.1945737574123,-5.96083151819561,-32.2004759304853));
#17466=CARTESIAN_POINT('Ctrl Pts',(36.228936418394,-5.93928082321056,-32.1619549506812));
#17467=CARTESIAN_POINT('Ctrl Pts',(36.2571177657912,-5.92160676640953,-32.1303633019867));
#17468=CARTESIAN_POINT('Ctrl Pts',(36.2861802813351,-5.90774301103496,-32.0977015889228));
#17469=CARTESIAN_POINT('Ctrl Pts',(36.3158986064529,-5.89882514864486,-32.0642076611468));
#17470=CARTESIAN_POINT('Ctrl Pts',(36.3404592414257,-5.89145500372474,-32.0365266888627));
#17471=CARTESIAN_POINT('Ctrl Pts',(36.3654675706966,-5.88746290319394,-32.0082775694218));
#17472=CARTESIAN_POINT('Ctrl Pts',(36.390794015381,-5.88746284406389,-31.9795977255543));
#17473=CARTESIAN_POINT('',(48.3374778008691,-5.88746284406389,-4.1303578658561));
#17474=CARTESIAN_POINT('Origin',(0.0835265683620477,-5.88746284406389,0.0824317919394229));
#17475=CARTESIAN_POINT('',(48.5210265683621,-5.88746284406389,0.082431791939678));
#17476=CARTESIAN_POINT('Origin',(0.0835265683666275,-5.88746284406447,0.082431791939678));
#17477=CARTESIAN_POINT('',(48.3374778008691,-5.88746284406389,4.29522144973544));
#17478=CARTESIAN_POINT('Origin',(0.0835265683722142,-5.88746284406447,0.0824317919400358));
#17479=CARTESIAN_POINT('',(40.0774385461352,-5.88746284406389,27.4078487322925));
#17480=CARTESIAN_POINT('Origin',(0.0835265683620477,-5.88746284406389,0.0824317919394229));
#17481=CARTESIAN_POINT('Ctrl Pts',(39.7815264758118,-6.59535043767467,27.8359938984173));
#17482=CARTESIAN_POINT('Ctrl Pts',(39.7815264758118,-6.57489151419421,27.8359938984173));
#17483=CARTESIAN_POINT('Ctrl Pts',(39.7818308190845,-6.5545035776552,27.8355603997887));
#17484=CARTESIAN_POINT('Ctrl Pts',(39.7824538268318,-6.53419088775616,27.8346716758371));
#17485=CARTESIAN_POINT('Ctrl Pts',(39.78330060454,-6.50658234986543,27.8334637428152));
#17486=CARTESIAN_POINT('Ctrl Pts',(39.7847511942221,-6.47911098112967,27.83139321691));
#17487=CARTESIAN_POINT('Ctrl Pts',(39.7868335547006,-6.45179259387194,27.8284172314537));
#17488=CARTESIAN_POINT('Ctrl Pts',(39.7888139630787,-6.42581171133136,27.8255869498616));
#17489=CARTESIAN_POINT('Ctrl Pts',(39.7913656196801,-6.39996806268029,27.8219379660937));
#17490=CARTESIAN_POINT('Ctrl Pts',(39.7945391139651,-6.37426951907649,27.8173953883731));
#17491=CARTESIAN_POINT('Ctrl Pts',(39.7953939463684,-6.3673471975545,27.8161717710348));
#17492=CARTESIAN_POINT('Ctrl Pts',(39.7962940619142,-6.36043542154511,27.8148830810215));
#17493=CARTESIAN_POINT('Ctrl Pts',(39.7972408290946,-6.35353442314531,27.8135273091373));
#17494=CARTESIAN_POINT('Ctrl Pts',(39.7986003789312,-6.34362464654871,27.8115804319307));
#17495=CARTESIAN_POINT('Ctrl Pts',(39.8000526202253,-6.33375626741061,27.8095002474653));
#17496=CARTESIAN_POINT('Ctrl Pts',(39.8016009821918,-6.32393813773167,27.8072817093222));
#17497=CARTESIAN_POINT('Ctrl Pts',(39.8075589693638,-6.28615867017362,27.798744931693));
#17498=CARTESIAN_POINT('Ctrl Pts',(39.814935878068,-6.24912973386477,27.7881657996788));
#17499=CARTESIAN_POINT('Ctrl Pts',(39.8239362603802,-6.21334185678225,27.7752436108075));
#17500=CARTESIAN_POINT('Ctrl Pts',(39.8313090163065,-6.18402584845048,27.7646582666212));
#17501=CARTESIAN_POINT('Ctrl Pts',(39.8397710012815,-6.15554336972048,27.7525008860325));
#17502=CARTESIAN_POINT('Ctrl Pts',(39.8494229508932,-6.12818087652871,27.738622620872));
#17503=CARTESIAN_POINT('Ctrl Pts',(39.8494701531467,-6.12804706197381,27.7385547500876));
#17504=CARTESIAN_POINT('Ctrl Pts',(39.849517383474,-6.12791327327699,27.7384868387004));
#17505=CARTESIAN_POINT('Ctrl Pts',(39.8495646418855,-6.12777951046923,27.7384188866947));
#17506=CARTESIAN_POINT('Ctrl Pts',(39.8661978278375,-6.08070002593731,27.7145023327956));
#17507=CARTESIAN_POINT('Ctrl Pts',(39.886627468029,-6.03703191466581,27.6850826400422));
#17508=CARTESIAN_POINT('Ctrl Pts',(39.9102991480491,-6.0004296227601,27.6508850155614));
#17509=CARTESIAN_POINT('Ctrl Pts',(39.921464524412,-5.98316517999444,27.6347547980304));
#17510=CARTESIAN_POINT('Ctrl Pts',(39.9333511717159,-5.96747341996643,27.617561599409));
#17511=CARTESIAN_POINT('Ctrl Pts',(39.9459007642834,-5.95374197151939,27.5993816540998));
#17512=CARTESIAN_POINT('Ctrl Pts',(39.9459903869208,-5.95364390868437,27.5992518224229));
#17513=CARTESIAN_POINT('Ctrl Pts',(39.9460800412851,-5.95354594807955,27.5991219434397));
#17514=CARTESIAN_POINT('Ctrl Pts',(39.9461697273638,-5.95344808981824,27.5989920171655));
#17515=CARTESIAN_POINT('Ctrl Pts',(39.9585679941583,-5.93992009472827,27.5810309173459));
#17516=CARTESIAN_POINT('Ctrl Pts',(39.9716254570657,-5.92838288344757,27.5620857784538));
#17517=CARTESIAN_POINT('Ctrl Pts',(39.9851489701298,-5.91890173045338,27.5424333146948));
#17518=CARTESIAN_POINT('Ctrl Pts',(39.9986774103974,-5.90941712306312,27.5227736906891));
#17519=CARTESIAN_POINT('Ctrl Pts',(40.0126731131938,-5.9019896316848,27.5024049744744));
#17520=CARTESIAN_POINT('Ctrl Pts',(40.0269527763041,-5.89673275177423,27.4815888599194));
#17521=CARTESIAN_POINT('Ctrl Pts',(40.0406119262791,-5.89170430603683,27.4616772955916));
#17522=CARTESIAN_POINT('Ctrl Pts',(40.0545316312244,-5.88866186034882,27.4413553084195));
#17523=CARTESIAN_POINT('Ctrl Pts',(40.0685489706349,-5.88775186306124,27.4208547357792));
#17524=CARTESIAN_POINT('Ctrl Pts',(40.0715083731049,-5.88755974042358,27.4165265645385));
#17525=CARTESIAN_POINT('Ctrl Pts',(40.0744720964614,-5.88746284473756,27.4121904749052));
#17526=CARTESIAN_POINT('Ctrl Pts',(40.0774385461352,-5.88746284406389,27.4078487322925));
#17527=CARTESIAN_POINT('',(38.6978118282835,-12.8919045823054,29.3250099976212));
#17528=CARTESIAN_POINT('Origin',(0.0835265683620477,-12.8919045823054,0.0824317919394229));
#17529=CARTESIAN_POINT('',(38.6978118282835,-11.3294045823054,29.3250099976212));
#17530=CARTESIAN_POINT('',(38.6978118282835,-14.7669045823054,29.3250099976212));
#17531=CARTESIAN_POINT('',(38.2918261423358,-10.7044045823054,29.8535125569281));
#17532=CARTESIAN_POINT('Ctrl Pts',(38.2918261423358,-10.7044045823054,29.8535125569281));
#17533=CARTESIAN_POINT('Ctrl Pts',(38.3145613787425,-10.7044045890531,29.8243340823417));
#17534=CARTESIAN_POINT('Ctrl Pts',(38.3372145101185,-10.7074293129562,29.7951803758307));
#17535=CARTESIAN_POINT('Ctrl Pts',(38.3595197775548,-10.7132787489585,29.7664089741967));
#17536=CARTESIAN_POINT('Ctrl Pts',(38.3833349248782,-10.7195241428123,29.7356899895188));
#17537=CARTESIAN_POINT('Ctrl Pts',(38.4067542844197,-10.7289894494735,29.7054058132917));
#17538=CARTESIAN_POINT('Ctrl Pts',(38.4294652924291,-10.7414871419631,29.6759757572924));
#17539=CARTESIAN_POINT('Ctrl Pts',(38.4523546563143,-10.754082982315,29.6463145788608));
#17540=CARTESIAN_POINT('Ctrl Pts',(38.4745254734339,-10.7697593965528,29.6175196926078));
#17541=CARTESIAN_POINT('Ctrl Pts',(38.4956548471652,-10.7883769193451,29.5900228324637));
#17542=CARTESIAN_POINT('Ctrl Pts',(38.5159153471861,-10.8062288597631,29.563656687276));
#17543=CARTESIAN_POINT('Ctrl Pts',(38.5352190348517,-10.8267856372083,29.5384830148832));
#17544=CARTESIAN_POINT('Ctrl Pts',(38.5532662014732,-10.8499643578046,29.5149012419193));
#17545=CARTESIAN_POINT('Ctrl Pts',(38.5608107877339,-10.8596541811778,29.5050429232126));
#17546=CARTESIAN_POINT('Ctrl Pts',(38.5681355314262,-10.8698026686923,29.4954631269277));
#17547=CARTESIAN_POINT('Ctrl Pts',(38.5752172515215,-10.8804055842374,29.4861926830638));
#17548=CARTESIAN_POINT('Ctrl Pts',(38.5753126767019,-10.8805484570303,29.4860677651391));
#17549=CARTESIAN_POINT('Ctrl Pts',(38.5754080562229,-10.8806914099898,29.4859429053908));
#17550=CARTESIAN_POINT('Ctrl Pts',(38.5755033900257,-10.8808344430917,29.4858181038972));
#17551=CARTESIAN_POINT('Ctrl Pts',(38.5925120729296,-10.9063532475959,29.4635520349072));
#17552=CARTESIAN_POINT('Ctrl Pts',(38.6080556228767,-10.9345143821538,29.4431688682605));
#17553=CARTESIAN_POINT('Ctrl Pts',(38.6219328729767,-10.9647671393856,29.4249477455011));
#17554=CARTESIAN_POINT('Ctrl Pts',(38.6391857315655,-11.0023788087495,29.4022943774324));
#17555=CARTESIAN_POINT('Ctrl Pts',(38.653865995194,-11.0432205203795,29.3829789426412));
#17556=CARTESIAN_POINT('Ctrl Pts',(38.6655922703494,-11.0862730505925,29.3675309600644));
#17557=CARTESIAN_POINT('Ctrl Pts',(38.6759685143952,-11.124368997887,29.353861484028));
#17558=CARTESIAN_POINT('Ctrl Pts',(38.6840329906305,-11.1641988556059,29.3432186123161));
#17559=CARTESIAN_POINT('Ctrl Pts',(38.689502333601,-11.2050768635654,29.3359944743684));
#17560=CARTESIAN_POINT('Ctrl Pts',(38.6949392018608,-11.2457121547152,29.3288132303826));
#17561=CARTESIAN_POINT('Ctrl Pts',(38.6978118157992,-11.2873849299258,29.3250100141064));
#17562=CARTESIAN_POINT('Ctrl Pts',(38.6978118282835,-11.3294045823054,29.3250099976212));
#17563=CARTESIAN_POINT('',(34.4123700316823,-10.7044045823054,34.2543780742461));
#17564=CARTESIAN_POINT('Origin',(0.0835265683620477,-10.7044045823054,0.0824317919394229));
#17565=CARTESIAN_POINT('',(33.9104937793594,-11.3294045823054,34.7512606668251));
#17566=CARTESIAN_POINT('Ctrl Pts',(33.9104937793594,-11.3294045823054,34.7512606668251));
#17567=CARTESIAN_POINT('Ctrl Pts',(33.9104937793594,-11.2968266539584,34.7512606668251));
#17568=CARTESIAN_POINT('Ctrl Pts',(33.9125379144729,-11.2645751882985,34.7492683274401));
#17569=CARTESIAN_POINT('Ctrl Pts',(33.9165467959317,-11.2329045289611,34.7453560772944));
#17570=CARTESIAN_POINT('Ctrl Pts',(33.9206548226578,-11.2004506097504,34.7413470717096));
#17571=CARTESIAN_POINT('Ctrl Pts',(33.9268258259103,-11.1686071890466,34.7353221505169));
#17572=CARTESIAN_POINT('Ctrl Pts',(33.9349354785982,-11.1376386773475,34.7273971922678));
#17573=CARTESIAN_POINT('Ctrl Pts',(33.9402732993077,-11.1172550222821,34.7221809385155));
#17574=CARTESIAN_POINT('Ctrl Pts',(33.9464502105666,-11.0972501995383,34.7161423031669));
#17575=CARTESIAN_POINT('Ctrl Pts',(33.9534225056046,-11.0776955263552,34.7093224327386));
#17576=CARTESIAN_POINT('Ctrl Pts',(33.9535424494101,-11.077359128956,34.7092051110809));
#17577=CARTESIAN_POINT('Ctrl Pts',(33.9536625998153,-11.0770229370416,34.7090875861962));
#17578=CARTESIAN_POINT('Ctrl Pts',(33.95378295654,-11.0766869507352,34.7089698583435));
#17579=CARTESIAN_POINT('Ctrl Pts',(33.9693304965678,-11.033284635162,34.6937619129218));
#17580=CARTESIAN_POINT('Ctrl Pts',(33.9883532275802,-10.9932074809405,34.6751353966495));
#17581=CARTESIAN_POINT('Ctrl Pts',(34.0104109863479,-10.9565169211339,34.6534884940964));
#17582=CARTESIAN_POINT('Ctrl Pts',(34.0280526104672,-10.9271720964104,34.6361754695862));
#17583=CARTESIAN_POINT('Ctrl Pts',(34.0476365365734,-10.8999941023149,34.6169295464802));
#17584=CARTESIAN_POINT('Ctrl Pts',(34.0689512965709,-10.8750283402102,34.5959409193929));
#17585=CARTESIAN_POINT('Ctrl Pts',(34.0691852256687,-10.8747543414317,34.5957105695978));
#17586=CARTESIAN_POINT('Ctrl Pts',(34.0694192932445,-10.8744806828913,34.5954800787707));
#17587=CARTESIAN_POINT('Ctrl Pts',(34.0696534992273,-10.8742073644076,34.5952494469643));
#17588=CARTESIAN_POINT('Ctrl Pts',(34.1029073173621,-10.8354001442153,34.5625031095206));
#17589=CARTESIAN_POINT('Ctrl Pts',(34.1388819115252,-10.8035158666011,34.5269830759871));
#17590=CARTESIAN_POINT('Ctrl Pts',(34.1773200551437,-10.7780132626927,34.4888941942524));
#17591=CARTESIAN_POINT('Ctrl Pts',(34.1944881548576,-10.7666227217964,34.4718820896591));
#17592=CARTESIAN_POINT('Ctrl Pts',(34.2121479569922,-10.7565058951171,34.4543572802956));
#17593=CARTESIAN_POINT('Ctrl Pts',(34.2302776562603,-10.7476174402577,34.4363369031143));
#17594=CARTESIAN_POINT('Ctrl Pts',(34.2734134759625,-10.7264692248033,34.3934611924055));
#17595=CARTESIAN_POINT('Ctrl Pts',(34.3174478486389,-10.7131720597773,34.3495305269313));
#17596=CARTESIAN_POINT('Ctrl Pts',(34.3622933333352,-10.7075299711833,34.3046109908009));
#17597=CARTESIAN_POINT('Ctrl Pts',(34.3788760363315,-10.7054436724162,34.2880009054952));
#17598=CARTESIAN_POINT('Ctrl Pts',(34.3955696930212,-10.7044045890775,34.2712555500347));
#17599=CARTESIAN_POINT('Ctrl Pts',(34.4123700316823,-10.7044045823054,34.2543780742461));
#17600=CARTESIAN_POINT('',(33.9104937793594,-12.8919045823054,34.7512606668251));
#17601=CARTESIAN_POINT('',(33.9104937793594,-14.7669045823054,34.7512606668251));
#17602=CARTESIAN_POINT('',(32.8663673445036,-12.8919045823054,35.7402045336033));
#17603=CARTESIAN_POINT('Origin',(0.0835265683620477,-12.8919045823054,0.0824317919394229));
#17604=CARTESIAN_POINT('',(32.8663673445036,-7.07886995352309,35.7402045336033));
#17605=CARTESIAN_POINT('',(32.8663673445036,-14.7669045823054,35.7402045336033));
#17606=CARTESIAN_POINT('',(32.1455560858559,-5.88746284406389,36.3896992389582));
#17607=CARTESIAN_POINT('Ctrl Pts',(32.8663673445036,-7.07886995352308,35.7402045336033));
#17608=CARTESIAN_POINT('Ctrl Pts',(32.8663673257456,-7.03750286914797,35.740204550849));
#17609=CARTESIAN_POINT('Ctrl Pts',(32.8644568367469,-6.99633891589931,35.7419627809549));
#17610=CARTESIAN_POINT('Ctrl Pts',(32.8608787138668,-6.95552189492322,35.7452522106034));
#17611=CARTESIAN_POINT('Ctrl Pts',(32.8571075791363,-6.91250311369205,35.7487190793519));
#17612=CARTESIAN_POINT('Ctrl Pts',(32.8514836535699,-6.86986888734432,35.7538871693173));
#17613=CARTESIAN_POINT('Ctrl Pts',(32.8442472917155,-6.82778372078273,35.7605312059195));
#17614=CARTESIAN_POINT('Ctrl Pts',(32.836476613029,-6.78259107931536,35.7676658233771));
#17615=CARTESIAN_POINT('Ctrl Pts',(32.8268460618802,-6.73803026500875,35.7765029008283));
#17616=CARTESIAN_POINT('Ctrl Pts',(32.8156110024303,-6.69431754451611,35.786802191545));
#17617=CARTESIAN_POINT('Ctrl Pts',(32.8134829089406,-6.68603768126203,35.7887530360083));
#17618=CARTESIAN_POINT('Ctrl Pts',(32.8112971495395,-6.67778831508346,35.7907564321687));
#17619=CARTESIAN_POINT('Ctrl Pts',(32.809055332468,-6.66957102631489,35.7928108627312));
#17620=CARTESIAN_POINT('Ctrl Pts',(32.8089599345267,-6.66922134906352,35.7928982866556));
#17621=CARTESIAN_POINT('Ctrl Pts',(32.8088644372364,-6.66887173803708,35.7929858010134));
#17622=CARTESIAN_POINT('Ctrl Pts',(32.8087688407508,-6.6685221934126,35.7930734056603));
#17623=CARTESIAN_POINT('Ctrl Pts',(32.7813902237688,-6.56841340451216,35.8181631781542));
#17624=CARTESIAN_POINT('Ctrl Pts',(32.7456982481617,-6.47280389900386,35.8508192456723));
#17625=CARTESIAN_POINT('Ctrl Pts',(32.7023531332,-6.38345298992926,35.8903027225724));
#17626=CARTESIAN_POINT('Ctrl Pts',(32.6894404002325,-6.35683489397307,35.9020650536745));
#17627=CARTESIAN_POINT('Ctrl Pts',(32.6758482678309,-6.33077245149717,35.9144334760923));
#17628=CARTESIAN_POINT('Ctrl Pts',(32.6615936985498,-6.30531282539089,35.9273888757788));
#17629=CARTESIAN_POINT('Ctrl Pts',(32.6613394121676,-6.304858652691,35.9276199863548));
#17630=CARTESIAN_POINT('Ctrl Pts',(32.6610849155965,-6.30440467367567,35.9278512831621));
#17631=CARTESIAN_POINT('Ctrl Pts',(32.6608302089385,-6.3039508886075,35.9280827660871));
#17632=CARTESIAN_POINT('Ctrl Pts',(32.6217449724213,-6.23431667936603,35.9636042751914));
#17633=CARTESIAN_POINT('Ctrl Pts',(32.5785970691921,-6.170228754371,36.0027115558799));
#17634=CARTESIAN_POINT('Ctrl Pts',(32.530281991526,-6.11310220447119,36.0462996751091));
#17635=CARTESIAN_POINT('Ctrl Pts',(32.501808626091,-6.07943600315446,36.0719873177124));
#17636=CARTESIAN_POINT('Ctrl Pts',(32.4715401872415,-6.04818794004946,36.0992316071682));
#17637=CARTESIAN_POINT('Ctrl Pts',(32.4392453165235,-6.01965292485606,36.1282203202621));
#17638=CARTESIAN_POINT('Ctrl Pts',(32.4389270659117,-6.01937172583469,36.1285059902607));
#17639=CARTESIAN_POINT('Ctrl Pts',(32.4386086136055,-6.01909078646778,36.1287918340641));
#17640=CARTESIAN_POINT('Ctrl Pts',(32.4382899594135,-6.01881010710771,36.1290778518239));
#17641=CARTESIAN_POINT('Ctrl Pts',(32.4033630553722,-5.98804553120947,36.1604275566225));
#17642=CARTESIAN_POINT('Ctrl Pts',(32.3664342908023,-5.96083151820698,36.1934789809758));
#17643=CARTESIAN_POINT('Ctrl Pts',(32.3279133110069,-5.93928082322402,36.2278416419498));
#17644=CARTESIAN_POINT('Ctrl Pts',(32.2963216623196,-5.92160676642473,36.2560229893406));
#17645=CARTESIAN_POINT('Ctrl Pts',(32.2636599492633,-5.90774301105001,36.2850855048778));
#17646=CARTESIAN_POINT('Ctrl Pts',(32.2301660214951,-5.8988251486572,36.3148038299887));
#17647=CARTESIAN_POINT('Ctrl Pts',(32.2024850491961,-5.89145500372915,36.3393644649749));
#17648=CARTESIAN_POINT('Ctrl Pts',(32.1742359297396,-5.8874629031939,36.3643727942596));
#17649=CARTESIAN_POINT('Ctrl Pts',(32.1455560858559,-5.8874628440639,36.3896992389582));
#17650=CARTESIAN_POINT('',(4.29631622615791,-5.88746284406389,48.3363830244465));
#17651=CARTESIAN_POINT('Origin',(0.0835265683620477,-5.88746284406389,0.0824317919394229));
#17652=CARTESIAN_POINT('Origin',(0.0835265683623214,-5.88746284406272,0.0824317919373119));
#17653=CARTESIAN_POINT('',(4.29631622615776,11.353653679453,48.3363830244465));
#17654=CARTESIAN_POINT('Origin',(0.0835265683614805,11.3536536794601,0.0824317919346118));
#17655=CARTESIAN_POINT('',(48.3374778008691,11.353653679453,4.29522144973533));
#17656=CARTESIAN_POINT('Origin',(0.0835265683620477,11.353653679453,0.0824317919394229));
#17657=CARTESIAN_POINT('',(48.5210265683621,11.353653679453,0.0824317919395275));
#17658=CARTESIAN_POINT('Origin',(0.0835265683614939,11.3536536794601,0.0824317919395275));
#17659=CARTESIAN_POINT('',(48.3374778008691,11.3536536794531,-4.13035786585629));
#17660=CARTESIAN_POINT('Origin',(0.0835265683752606,11.3536536794495,0.0824317919385903));
#17661=CARTESIAN_POINT('',(4.29631622615795,11.3536536794531,-48.1715194405676));
#17662=CARTESIAN_POINT('Origin',(0.0835265683620477,11.3536536794531,0.0824317919394229));
#17663=CARTESIAN_POINT('Origin',(0.0835265683620358,11.3536536794531,0.0824317919406425));
#17664=CARTESIAN_POINT('Origin',(-44.291473431638,16.4830954176946,-44.2925682080606));
#17665=CARTESIAN_POINT('',(-44.291473431638,16.4830954176946,-41.4800682080606));
#17666=CARTESIAN_POINT('Origin',(-44.291473431638,16.4830954176946,-44.2925682080606));
#17667=CARTESIAN_POINT('',(-44.291473431638,16.4830954176946,-41.4800682080606));
#17668=CARTESIAN_POINT('Origin',(0.0835265683620477,-8.56135981233827,0.0824317919394229));
#17669=CARTESIAN_POINT('',(-34.2245838299083,-3.84038894321748,-35.9856330592973));
#17670=CARTESIAN_POINT('',(34.3916369666325,-3.84038894321748,-35.9856330592972));
#17671=CARTESIAN_POINT('Origin',(0.0835265683620477,-3.84038894321748,0.0824317919394229));
#17672=CARTESIAN_POINT('',(37.6657443451358,-8.46983068145907,-39.2604024894786));
#17673=CARTESIAN_POINT('Ctrl Pts',(34.3916369666325,-3.84038894321748,-35.9856330592972));
#17674=CARTESIAN_POINT('Ctrl Pts',(34.4958082618834,-3.98768003220409,-36.0898273687807));
#17675=CARTESIAN_POINT('Ctrl Pts',(34.5999795168213,-4.13497132206384,-36.1940214346108));
#17676=CARTESIAN_POINT('Ctrl Pts',(35.120835595128,-4.87142874967365,-36.7149905771548));
#17677=CARTESIAN_POINT('Ctrl Pts',(35.5375198299908,-5.46059781902367,-37.1317620980747));
#17678=CARTESIAN_POINT('Ctrl Pts',(36.5247181312096,-6.85645163869056,-38.1191604328652));
#17679=CARTESIAN_POINT('Ctrl Pts',(37.0952317024764,-7.66313885272879,-38.6897842589155));
#17680=CARTESIAN_POINT('Ctrl Pts',(37.6657443451358,-8.46983068145907,-39.2604024894786));
#17681=CARTESIAN_POINT('',(21.7919948253829,-8.46983068145907,-49.8076885551783));
#17682=CARTESIAN_POINT('Origin',(0.0835265683620477,-8.46983068145906,0.0824317919394229));
#17683=CARTESIAN_POINT('',(0.0835265683748736,-3.96983068145906,-49.8260390771814));
#17684=CARTESIAN_POINT('Ctrl Pts',(21.7919948253829,-8.46983068145907,-49.8076885551783));
#17685=CARTESIAN_POINT('Ctrl Pts',(18.3176422503578,-7.08833344112081,-49.812854312048));
#17686=CARTESIAN_POINT('Ctrl Pts',(14.7835076505935,-5.9615388332069,-49.8174729109528));
#17687=CARTESIAN_POINT('Ctrl Pts',(9.36046138845711,-4.79046405132309,-49.8224360560758));
#17688=CARTESIAN_POINT('Ctrl Pts',(7.53242010945153,-4.48684598729498,-49.8237597865973));
#17689=CARTESIAN_POINT('Ctrl Pts',(4.75579089154249,-4.17869234558141,-49.825113184365));
#17690=CARTESIAN_POINT('Ctrl Pts',(3.82399411154456,-4.10048196518639,-49.8254593234283));
#17691=CARTESIAN_POINT('Ctrl Pts',(1.950298450602,-3.99585474310376,-49.8259231591874));
#17692=CARTESIAN_POINT('Ctrl Pts',(1.0157663414152,-3.9698306814593,-49.8260390771814));
#17693=CARTESIAN_POINT('Ctrl Pts',(0.0835265683748736,-3.96983068145906,
-49.8260390771814));
#17694=CARTESIAN_POINT('',(-21.6249416886588,-8.46983068145907,-49.8076885551783));
#17695=CARTESIAN_POINT('Ctrl Pts',(0.0835265683748736,-3.96983068145906,
-49.8260390771814));
#17696=CARTESIAN_POINT('Ctrl Pts',(-3.6278126578305,-3.96983068145811,-49.8260390771814));
#17697=CARTESIAN_POINT('Ctrl Pts',(-7.30249637963826,-4.38596719587718,
-49.8241519497213));
#17698=CARTESIAN_POINT('Ctrl Pts',(-11.8554848249969,-5.36440184532962,
-49.8200032614064));
#17699=CARTESIAN_POINT('Ctrl Pts',(-12.7640306839956,-5.58285881740927,
-49.8190865644975));
#17700=CARTESIAN_POINT('Ctrl Pts',(-14.5677356401152,-6.06008817135185,
-49.8171139830856));
#17701=CARTESIAN_POINT('Ctrl Pts',(-15.4645089261327,-6.31922781225809,
-49.8160565954838));
#17702=CARTESIAN_POINT('Ctrl Pts',(-18.1357164005855,-7.15188128916168,
-49.8127161593677));
#17703=CARTESIAN_POINT('Ctrl Pts',(-19.8909577469063,-7.78035142493754,
-49.8102666871513));
#17704=CARTESIAN_POINT('Ctrl Pts',(-21.6249416886588,-8.46983068145907,
-49.8076885551783));
#17705=CARTESIAN_POINT('',(-37.4986912084115,-8.46983068145907,-39.2604024894787));
#17706=CARTESIAN_POINT('Origin',(0.0835265683620477,-8.46983068145906,0.0824317919394229));
#17707=CARTESIAN_POINT('Ctrl Pts',(-37.4986912084115,-8.46983068145907,
-39.2604024894787));
#17708=CARTESIAN_POINT('Ctrl Pts',(-37.3945206549071,-8.32253590125116,
-39.1562126565586));
#17709=CARTESIAN_POINT('Ctrl Pts',(-37.2903500703809,-8.17524127521396,
-39.0520226367007));
#17710=CARTESIAN_POINT('Ctrl Pts',(-36.7694969888621,-7.43876893481716,
-38.5310715797203));
#17711=CARTESIAN_POINT('Ctrl Pts',(-36.3528140157447,-6.84959358714928,
-38.1143076728));
#17712=CARTESIAN_POINT('Ctrl Pts',(-35.3656160331638,-5.45373818194082,
-37.1269112608724));
#17713=CARTESIAN_POINT('Ctrl Pts',(-34.795100534904,-4.64706055617428,-36.5562758067325));
#17714=CARTESIAN_POINT('Ctrl Pts',(-34.2245838299083,-3.84038894321748,
-35.9856330592973));
#17715=CARTESIAN_POINT('Origin',(-39.6912298733813,13.1261401876617,-39.6923246498039));
#17716=CARTESIAN_POINT('',(-40.3541424807436,12.8136401876617,-39.0294120424415));
#17717=CARTESIAN_POINT('',(-39.0283172660189,12.8136401876617,-40.3552372571663));
#17718=CARTESIAN_POINT('Origin',(-39.6912298733813,12.8136401876617,-39.6923246498039));
#17719=CARTESIAN_POINT('',(-39.0283172660189,16.4855954176946,-40.3552372571663));
#17720=CARTESIAN_POINT('',(-40.3541424807436,16.4855954176946,-39.0294120424415));
#17721=CARTESIAN_POINT('Origin',(16.7670594440865,-17.1192738307565,25.3269308122136));
#17722=CARTESIAN_POINT('',(16.3756046859818,-11.3294045823054,26.5140547199659));
#17723=CARTESIAN_POINT('',(17.9541833518389,-11.3294045823054,25.7183855703182));
#17724=CARTESIAN_POINT('Origin',(16.7670594440865,-11.3294045823054,25.3269308122136));
#17725=CARTESIAN_POINT('',(16.3756046859818,-11.0169045823054,26.5140547199659));
#17726=CARTESIAN_POINT('',(16.3756046859818,-17.1192738307565,26.5140547199659));
#17727=CARTESIAN_POINT('',(17.9541833518389,-11.0169045823054,25.7183855703182));
#17728=CARTESIAN_POINT('Origin',(16.7670594440865,-11.0169045823054,25.3269308122136));
#17729=CARTESIAN_POINT('',(17.9541833518389,-17.1192738307565,25.7183855703182));
#17730=CARTESIAN_POINT('Origin',(-44.291473431638,16.4830954176946,-44.2925682080606));
#17731=CARTESIAN_POINT('',(49.7710265683621,16.4830954176946,44.4574317919394));
#17732=CARTESIAN_POINT('',(49.7710265683619,16.4830954176946,37.6072170232579));
#17733=CARTESIAN_POINT('',(49.7710265683622,16.4830954176946,-44.2925682080604));
#17734=CARTESIAN_POINT('',(48.8335265683621,16.4830954176946,37.6072170232579));
#17735=CARTESIAN_POINT('',(0.0835265683620477,16.4830954176946,37.6072170232579));
#17736=CARTESIAN_POINT('',(48.8335265683621,16.4830954176946,38.3884670232579));
#17737=CARTESIAN_POINT('',(48.8335265683619,16.4830954176946,0.0824317919392537));
#17738=CARTESIAN_POINT('',(48.8335265683621,16.4830954176946,40.1612670779183));
#17739=CARTESIAN_POINT('',(41.173224139993,16.4830954176946,46.8471376742924));
#17740=CARTESIAN_POINT('Origin',(44.4585265683621,16.4830954176946,44.4574317919394));
#17741=CARTESIAN_POINT('',(40.162361854341,16.4830954176946,48.8324317919394));
#17742=CARTESIAN_POINT('Origin',(40.162361854341,16.4830954176946,47.5824317919394));
#17743=CARTESIAN_POINT('',(29.625935174466,16.4830954176946,48.8324317919394));
#17744=CARTESIAN_POINT('',(29.625935174466,16.4830954176946,48.8324317919394));
#17745=CARTESIAN_POINT('',(28.9657696190223,16.4830954176946,46.5209792779729));
#17746=CARTESIAN_POINT('Origin',(29.625935174466,16.4830954176946,47.5824317919394));
#17747=CARTESIAN_POINT('',(46.5220740543956,16.4830954176946,28.9646748425997));
#17748=CARTESIAN_POINT('Origin',(0.0835265683620477,16.4830954176946,0.0824317919394229));
#17749=CARTESIAN_POINT('',(48.8335265683621,16.4830954176946,29.6248403980433));
#17750=CARTESIAN_POINT('Origin',(47.583526568362,16.4830954176946,29.6248403980433));
#17751=CARTESIAN_POINT('',(48.8335265683621,16.4830954176946,35.8884670232579));
#17752=CARTESIAN_POINT('',(48.8335265683621,16.4830954176946,40.1612670779183));
#17753=CARTESIAN_POINT('',(48.8335265683621,16.4830954176946,36.6697170232579));
#17754=CARTESIAN_POINT('',(48.8335265683619,16.4830954176946,0.0824317919392537));
#17755=CARTESIAN_POINT('',(49.7710265683619,16.4830954176946,36.6697170232579));
#17756=CARTESIAN_POINT('',(0.0835265683620477,16.4830954176946,36.6697170232579));
#17757=CARTESIAN_POINT('',(49.7710265683622,16.4830954176946,-44.2925682080604));
#17758=CARTESIAN_POINT('',(49.7710265683622,16.4830954176946,-44.2925682080604));
#17759=CARTESIAN_POINT('',(44.4585265683622,16.4830954176946,-49.6050682080606));
#17760=CARTESIAN_POINT('Origin',(44.4585265683622,16.4830954176946,-44.2925682080604));
#17761=CARTESIAN_POINT('',(-44.2914734316379,16.4830954176946,-49.6050682080606));
#17762=CARTESIAN_POINT('',(-44.2914734316379,16.4830954176946,-49.6050682080606));
#17763=CARTESIAN_POINT('',(-49.603973431638,16.4830954176946,-44.2925682080605));
#17764=CARTESIAN_POINT('Origin',(-44.291473431638,16.4830954176946,-44.2925682080606));
#17765=CARTESIAN_POINT('',(-49.6039734316384,16.4830954176946,44.4574317919389));
#17766=CARTESIAN_POINT('',(-49.603973431638,16.4830954176946,44.4574317919389));
#17767=CARTESIAN_POINT('',(-44.2914734316384,16.4830954176946,49.7699317919394));
#17768=CARTESIAN_POINT('Origin',(-44.2914734316384,16.4830954176946,44.457431791939));
#17769=CARTESIAN_POINT('',(44.458526568362,16.4830954176946,49.7699317919394));
#17770=CARTESIAN_POINT('',(44.458526568362,16.4830954176946,49.7699317919394));
#17771=CARTESIAN_POINT('Origin',(44.4585265683621,16.4830954176946,44.4574317919394));
#17772=CARTESIAN_POINT('',(-46.3550209176718,16.4830954176946,28.9646748425992));
#17773=CARTESIAN_POINT('',(-28.7987164822987,16.4830954176946,46.5209792779726));
#17774=CARTESIAN_POINT('Origin',(0.0835265683620477,16.4830954176946,0.0824317919394229));
#17775=CARTESIAN_POINT('',(-29.4588820377424,16.4830954176946,48.8324317919391));
#17776=CARTESIAN_POINT('Origin',(-29.4588820377423,16.4830954176946,47.5824317919391));
#17777=CARTESIAN_POINT('',(-39.9953087176173,16.4830954176946,48.832431791939));
#17778=CARTESIAN_POINT('',(-39.9953087176173,16.4830954176946,48.832431791939));
#17779=CARTESIAN_POINT('',(-41.0061710032694,16.4830954176946,46.8471376742919));
#17780=CARTESIAN_POINT('Origin',(-39.9953087176173,16.4830954176946,47.582431791939));
#17781=CARTESIAN_POINT('Origin',(-44.2914734316384,16.4830954176946,44.457431791939));
#17782=CARTESIAN_POINT('',(-48.6664734316382,16.4830954176946,29.6248403980428));
#17783=CARTESIAN_POINT('',(-48.6664734316382,16.4830954176946,29.6248403980428));
#17784=CARTESIAN_POINT('Origin',(-47.4164734316383,16.4830954176946,29.6248403980429));
#17785=CARTESIAN_POINT('',(28.9657696190224,16.4830954176946,-46.356115694094));
#17786=CARTESIAN_POINT('Origin',(0.0835265683620477,16.4830954176946,0.0824317919394229));
#17787=CARTESIAN_POINT('',(29.6259351744661,16.4830954176946,-48.6675682080605));
#17788=CARTESIAN_POINT('Origin',(29.6259351744661,16.4830954176946,-47.4175682080605));
#17789=CARTESIAN_POINT('',(40.1623618543411,16.4830954176946,-48.6675682080604));
#17790=CARTESIAN_POINT('',(40.1623618543411,16.4830954176946,-48.6675682080604));
#17791=CARTESIAN_POINT('Origin',(40.1623618543411,16.4830954176946,-47.4175682080604));
#17792=CARTESIAN_POINT('',(48.8335265683622,16.4830954176946,-39.9964034940393));
#17793=CARTESIAN_POINT('Origin',(47.5835265683622,16.4830954176946,-39.9964034940393));
#17794=CARTESIAN_POINT('',(48.8335265683621,16.4830954176946,-29.4599768141643));
#17795=CARTESIAN_POINT('',(-28.7987164822982,16.4830954176946,-46.3561156940941));
#17796=CARTESIAN_POINT('Origin',(0.0835265683620477,16.4830954176946,0.0824317919394229));
#17797=CARTESIAN_POINT('',(-48.6664734316379,16.4830954176946,-39.9964034940395));
#17798=CARTESIAN_POINT('',(-48.6664734316379,16.4830954176946,-39.9964034940395));
#17799=CARTESIAN_POINT('Origin',(-47.4164734316379,16.4830954176946,-39.9964034940395));
#17800=CARTESIAN_POINT('',(-39.9953087176169,16.4830954176946,-48.6675682080606));
#17801=CARTESIAN_POINT('Origin',(-39.9953087176169,16.4830954176946,-47.4175682080606));
#17802=CARTESIAN_POINT('',(-29.4588820377419,16.4830954176946,-48.6675682080606));
#17803=CARTESIAN_POINT('',(-29.4588820377419,16.4830954176946,-48.6675682080606));
#17804=CARTESIAN_POINT('Origin',(-29.4588820377419,16.4830954176946,-47.4175682080606));
#17805=CARTESIAN_POINT('',(48.6088737900632,16.4830954176946,22.7696071163714));
#17806=CARTESIAN_POINT('',(48.833526568362,16.4830954176946,21.5181263879131));
#17807=CARTESIAN_POINT('Ctrl Pts',(48.6088737900632,16.4830954176946,22.7696071163714));
#17808=CARTESIAN_POINT('Ctrl Pts',(48.6546862755533,16.4830954176946,22.6716193001842));
#17809=CARTESIAN_POINT('Ctrl Pts',(48.6897381335915,16.4830954176946,22.5688627245672));
#17810=CARTESIAN_POINT('Ctrl Pts',(48.746344156916,16.4830954176946,22.3629081987095));
#17811=CARTESIAN_POINT('Ctrl Pts',(48.7679585435476,16.4830954176946,22.258923921387));
#17812=CARTESIAN_POINT('Ctrl Pts',(48.8185384277345,16.4830954176946,21.9448236639213));
#17813=CARTESIAN_POINT('Ctrl Pts',(48.8335265683619,16.4830954176946,21.7326033051433));
#17814=CARTESIAN_POINT('Ctrl Pts',(48.833526568362,16.4830954176946,21.5181263879131));
#17815=CARTESIAN_POINT('',(22.7707018927938,16.4830954176946,48.6077790136406));
#17816=CARTESIAN_POINT('Origin',(0.0835265683620477,16.4830954176946,0.0824317919394229));
#17817=CARTESIAN_POINT('',(21.5192211643356,16.4830954176946,48.8324317919394));
#17818=CARTESIAN_POINT('Ctrl Pts',(21.5192211643356,16.4830954176946,48.8324317919394));
#17819=CARTESIAN_POINT('Ctrl Pts',(21.7332984919314,16.4830954176946,48.8324317919394));
#17820=CARTESIAN_POINT('Ctrl Pts',(21.9465891291831,16.4830954176946,48.8173905539921));
#17821=CARTESIAN_POINT('Ctrl Pts',(22.2609747321794,16.4830954176946,48.7666821942729));
#17822=CARTESIAN_POINT('Ctrl Pts',(22.3650002683796,16.4830954176946,48.745019785418));
#17823=CARTESIAN_POINT('Ctrl Pts',(22.570892003613,16.4830954176946,48.6883415841153));
#17824=CARTESIAN_POINT('Ctrl Pts',(22.6731778206313,16.4830954176946,48.6533746837426));
#17825=CARTESIAN_POINT('Ctrl Pts',(22.7707018927938,16.4830954176946,48.6077790136406));
#17826=CARTESIAN_POINT('',(-21.3521680276115,16.4830954176946,48.8324317919394));
#17827=CARTESIAN_POINT('',(-44.291473431638,16.4830954176946,48.8324317919394));
#17828=CARTESIAN_POINT('',(-22.6036487560697,16.4830954176946,48.6077790136406));
#17829=CARTESIAN_POINT('Ctrl Pts',(-22.6036487560697,16.4830954176946,48.6077790136407));
#17830=CARTESIAN_POINT('Ctrl Pts',(-22.5442911026821,16.4830954176946,48.6355306057096));
#17831=CARTESIAN_POINT('Ctrl Pts',(-22.483475353007,16.4830954176946,48.6595286545756));
#17832=CARTESIAN_POINT('Ctrl Pts',(-22.4216836912354,16.4830954176946,48.680466078412));
#17833=CARTESIAN_POINT('Ctrl Pts',(-22.3548812712597,16.4830954176946,48.7031013424626));
#17834=CARTESIAN_POINT('Ctrl Pts',(-22.2869375438441,16.4830954176946,48.7221589140917));
#17835=CARTESIAN_POINT('Ctrl Pts',(-22.2184316516974,16.4830954176945,48.7384583526655));
#17836=CARTESIAN_POINT('Ctrl Pts',(-22.1424085678882,16.4830954176944,48.756546338179));
#17837=CARTESIAN_POINT('Ctrl Pts',(-22.0656917788855,16.4830954176943,48.7712365700779));
#17838=CARTESIAN_POINT('Ctrl Pts',(-21.9890537694626,16.483095417693,48.783595693684));
#17839=CARTESIAN_POINT('Ctrl Pts',(-21.988813152617,16.483095417693,48.7836344970579));
#17840=CARTESIAN_POINT('Ctrl Pts',(-21.9885725320674,16.483095417693,48.7836732756889));
#17841=CARTESIAN_POINT('Ctrl Pts',(-21.9883319078107,16.483095417693,48.7837120295832));
#17842=CARTESIAN_POINT('Ctrl Pts',(-21.7932700913188,16.4830954176898,48.8151278358004));
#17843=CARTESIAN_POINT('Ctrl Pts',(-21.5961370769475,16.4830954176946,48.8302373326079));
#17844=CARTESIAN_POINT('Ctrl Pts',(-21.3973353133493,16.4830954176946,48.8322086727425));
#17845=CARTESIAN_POINT('Ctrl Pts',(-21.3822890539765,16.4830954176946,48.8323578731039));
#17846=CARTESIAN_POINT('Ctrl Pts',(-21.3672332341099,16.4830954176946,48.8324317919394));
#17847=CARTESIAN_POINT('Ctrl Pts',(-21.3521680276115,16.4830954176946,48.8324317919394));
#17848=CARTESIAN_POINT('',(-48.4418206533391,16.4830954176946,22.7696071163712));
#17849=CARTESIAN_POINT('Origin',(0.0835265683620477,16.4830954176946,0.0824317919394229));
#17850=CARTESIAN_POINT('',(-48.6664734316379,16.4830954176946,21.5181263879129));
#17851=CARTESIAN_POINT('Ctrl Pts',(-48.6664734316379,16.4830954176946,21.5181263879129));
#17852=CARTESIAN_POINT('Ctrl Pts',(-48.6664734316379,16.4830954176946,21.6670631867632));
#17853=CARTESIAN_POINT('Ctrl Pts',(-48.6591650713411,16.4830954176948,21.8157113579154));
#17854=CARTESIAN_POINT('Ctrl Pts',(-48.6433862740522,16.4830954176944,21.9626800039502));
#17855=CARTESIAN_POINT('Ctrl Pts',(-48.6364163282529,16.4830954176942,22.0276002560013));
#17856=CARTESIAN_POINT('Ctrl Pts',(-48.6277942051812,16.4830954176938,22.0921928653205));
#17857=CARTESIAN_POINT('Ctrl Pts',(-48.6174230355526,16.4830954176928,22.1563387307969));
#17858=CARTESIAN_POINT('Ctrl Pts',(-48.617413607667,16.4830954176928,22.1563970424342));
#17859=CARTESIAN_POINT('Ctrl Pts',(-48.6174041785652,16.4830954176928,22.1564553538403));
#17860=CARTESIAN_POINT('Ctrl Pts',(-48.6173947482465,16.4830954176928,22.1565136650151));
#17861=CARTESIAN_POINT('Ctrl Pts',(-48.6004607795326,16.4830954176911,22.2612227048913));
#17862=CARTESIAN_POINT('Ctrl Pts',(-48.5796176356208,16.4830954176926,22.3651301096173));
#17863=CARTESIAN_POINT('Ctrl Pts',(-48.5514944830101,16.4830954176936,22.4675457567853));
#17864=CARTESIAN_POINT('Ctrl Pts',(-48.5306835096382,16.4830954176943,22.5433327546222));
#17865=CARTESIAN_POINT('Ctrl Pts',(-48.5058864570286,16.4830954176946,22.6183030588211));
#17866=CARTESIAN_POINT('Ctrl Pts',(-48.4756998063479,16.4830954176946,22.6921687122293));
#17867=CARTESIAN_POINT('Ctrl Pts',(-48.4650933730757,16.4830954176946,22.7181222746919));
#17868=CARTESIAN_POINT('Ctrl Pts',(-48.4538211421634,16.4830954176946,22.7439393637239));
#17869=CARTESIAN_POINT('Ctrl Pts',(-48.4418206533392,16.4830954176946,22.7696071163711));
#17870=CARTESIAN_POINT('',(-48.6664734316379,16.4830954176946,-21.3532628040342));
#17871=CARTESIAN_POINT('',(-48.6664734316379,16.4830954176946,-44.2925682080606));
#17872=CARTESIAN_POINT('',(-48.4418206533391,16.4830954176946,-22.6047435324924));
#17873=CARTESIAN_POINT('Ctrl Pts',(-48.4418206533392,16.4830954176946,-22.6047435324923));
#17874=CARTESIAN_POINT('Ctrl Pts',(-48.4698886928407,16.4830954176946,-22.5447090321936));
#17875=CARTESIAN_POINT('Ctrl Pts',(-48.4941170616729,16.4830954176946,-22.4831875953525));
#17876=CARTESIAN_POINT('Ctrl Pts',(-48.5152210475791,16.4830954176946,-22.4206776899558));
#17877=CARTESIAN_POINT('Ctrl Pts',(-48.5380549774177,16.4830954176946,-22.3530436988988));
#17878=CARTESIAN_POINT('Ctrl Pts',(-48.5572307441801,16.4830954176946,-22.2842518491799));
#17879=CARTESIAN_POINT('Ctrl Pts',(-48.5735983779025,16.4830954176945,-22.2149034817008));
#17880=CARTESIAN_POINT('Ctrl Pts',(-48.5911862340032,16.4830954176944,-22.1403851286675));
#17881=CARTESIAN_POINT('Ctrl Pts',(-48.6055304232494,16.4830954176942,-22.0652228656951));
#17882=CARTESIAN_POINT('Ctrl Pts',(-48.6176377678211,16.4830954176929,-21.9901456057825));
#17883=CARTESIAN_POINT('Ctrl Pts',(-48.6176781949277,16.4830954176929,-21.9898949185755));
#17884=CARTESIAN_POINT('Ctrl Pts',(-48.6177185951685,16.4830954176929,-21.9896442273897));
#17885=CARTESIAN_POINT('Ctrl Pts',(-48.6177589685505,16.4830954176929,-21.9893935322219));
#17886=CARTESIAN_POINT('Ctrl Pts',(-48.6490360664948,16.4830954176895,-21.7951809860257));
#17887=CARTESIAN_POINT('Ctrl Pts',(-48.6641532259573,16.4830954176946,-21.5988820000785));
#17888=CARTESIAN_POINT('Ctrl Pts',(-48.6662251385255,16.4830954176946,-21.4008987475353));
#17889=CARTESIAN_POINT('Ctrl Pts',(-48.6663911974825,16.4830954176946,-21.3850308518833));
#17890=CARTESIAN_POINT('Ctrl Pts',(-48.6664734316364,16.4830954176946,-21.369152135278));
#17891=CARTESIAN_POINT('Ctrl Pts',(-48.6664734316379,16.4830954176946,-21.3532628040342));
#17892=CARTESIAN_POINT('',(-22.6036487560697,16.4830954176946,-48.4429154297618));
#17893=CARTESIAN_POINT('Origin',(0.0835265683620477,16.4830954176946,0.0824317919394229));
#17894=CARTESIAN_POINT('',(-21.3521680276115,16.4830954176946,-48.6675682080606));
#17895=CARTESIAN_POINT('Ctrl Pts',(-21.3521680276115,16.4830954176946,-48.6675682080606));
#17896=CARTESIAN_POINT('Ctrl Pts',(-21.5662453552073,16.4830954176946,-48.6675682080605));
#17897=CARTESIAN_POINT('Ctrl Pts',(-21.779535992459,16.4830954176946,-48.6525269701133));
#17898=CARTESIAN_POINT('Ctrl Pts',(-22.0939215954554,16.4830954176946,-48.601818610394));
#17899=CARTESIAN_POINT('Ctrl Pts',(-22.1979471316555,16.4830954176946,-48.5801562015391));
#17900=CARTESIAN_POINT('Ctrl Pts',(-22.4038388668889,16.4830954176946,-48.5234780002364));
#17901=CARTESIAN_POINT('Ctrl Pts',(-22.5061246839072,16.4830954176946,-48.4885110998637));
#17902=CARTESIAN_POINT('Ctrl Pts',(-22.6036487560697,16.4830954176946,-48.4429154297618));
#17903=CARTESIAN_POINT('',(21.5192211643356,16.4830954176946,-48.6675682080606));
#17904=CARTESIAN_POINT('',(-44.291473431638,16.4830954176946,-48.6675682080606));
#17905=CARTESIAN_POINT('',(22.7707018927938,16.4830954176946,-48.4429154297618));
#17906=CARTESIAN_POINT('Ctrl Pts',(22.7707018927938,16.4830954176946,-48.4429154297618));
#17907=CARTESIAN_POINT('Ctrl Pts',(22.7113442394013,16.4830954176946,-48.4706670218339));
#17908=CARTESIAN_POINT('Ctrl Pts',(22.6505284897208,16.4830954176946,-48.4946650707021));
#17909=CARTESIAN_POINT('Ctrl Pts',(22.5887368279435,16.4830954176946,-48.5156024945398));
#17910=CARTESIAN_POINT('Ctrl Pts',(22.5219344079612,16.4830954176946,-48.5382377585921));
#17911=CARTESIAN_POINT('Ctrl Pts',(22.4539906805388,16.4830954176946,-48.5572953302219));
#17912=CARTESIAN_POINT('Ctrl Pts',(22.3854847883852,16.4830954176945,-48.573594768796));
#17913=CARTESIAN_POINT('Ctrl Pts',(22.3094617045878,16.4830954176944,-48.5916827543053));
#17914=CARTESIAN_POINT('Ctrl Pts',(22.2327449155974,16.4830954176943,-48.6063729862011));
#17915=CARTESIAN_POINT('Ctrl Pts',(22.1561069061867,16.483095417693,-48.6187321098052));
#17916=CARTESIAN_POINT('Ctrl Pts',(22.1558662893411,16.483095417693,-48.6187709131791));
#17917=CARTESIAN_POINT('Ctrl Pts',(22.1556256687915,16.483095417693,-48.6188096918101));
#17918=CARTESIAN_POINT('Ctrl Pts',(22.1553850445348,16.483095417693,-48.6188484457044));
#17919=CARTESIAN_POINT('Ctrl Pts',(21.960323227055,16.4830954176898,-48.6502642520806));
#17920=CARTESIAN_POINT('Ctrl Pts',(21.763190211675,16.4830954176946,-48.6653737488822));
#17921=CARTESIAN_POINT('Ctrl Pts',(21.5643884470531,16.4830954176946,-48.6673450888936));
#17922=CARTESIAN_POINT('Ctrl Pts',(21.5493421886858,16.4830954176946,-48.667494289235));
#17923=CARTESIAN_POINT('Ctrl Pts',(21.534286369826,16.4830954176946,-48.6675682080606));
#17924=CARTESIAN_POINT('Ctrl Pts',(21.5192211643356,16.4830954176946,-48.6675682080606));
#17925=CARTESIAN_POINT('',(48.6088737900633,16.4830954176946,-22.6047435324922));
#17926=CARTESIAN_POINT('Origin',(0.0835265683620477,16.4830954176946,0.0824317919394229));
#17927=CARTESIAN_POINT('',(48.8335265683621,16.4830954176946,-21.353262804034));
#17928=CARTESIAN_POINT('Ctrl Pts',(48.8335265683621,16.4830954176946,-21.353262804034));
#17929=CARTESIAN_POINT('Ctrl Pts',(48.8335265683621,16.4830954176946,-21.5205271356));
#17930=CARTESIAN_POINT('Ctrl Pts',(48.8242872408348,16.4830954176954,-21.6876151718335));
#17931=CARTESIAN_POINT('Ctrl Pts',(48.8041808326122,16.4830954176937,-21.8523364174683));
#17932=CARTESIAN_POINT('Ctrl Pts',(48.798489466322,16.4830954176932,-21.8989627932144));
#17933=CARTESIAN_POINT('Ctrl Pts',(48.7919270859958,16.4830954176924,-21.9453996267745));
#17934=CARTESIAN_POINT('Ctrl Pts',(48.7844559810354,16.483095417691,-21.9915973363727));
#17935=CARTESIAN_POINT('Ctrl Pts',(48.7844427023226,16.483095417691,-21.9916794455283));
#17936=CARTESIAN_POINT('Ctrl Pts',(48.7844294211923,16.483095417691,-21.991761554233));
#17937=CARTESIAN_POINT('Ctrl Pts',(48.7844161376429,16.483095417691,-21.9918436624863));
#17938=CARTESIAN_POINT('Ctrl Pts',(48.7674708494511,16.4830954176877,-22.0965858496438));
#17939=CARTESIAN_POINT('Ctrl Pts',(48.7466093475409,16.4830954176906,-22.2005030769087));
#17940=CARTESIAN_POINT('Ctrl Pts',(48.7184834265343,16.4830954176926,-22.3028911433133));
#17941=CARTESIAN_POINT('Ctrl Pts',(48.6974913278267,16.4830954176941,-22.3793096327179));
#17942=CARTESIAN_POINT('Ctrl Pts',(48.672452993622,16.4830954176945,-22.454876484413));
#17943=CARTESIAN_POINT('Ctrl Pts',(48.6419388604506,16.4830954176946,-22.5292903869264));
#17944=CARTESIAN_POINT('Ctrl Pts',(48.6315691300731,16.4830954176946,-22.5545787377723));
#17945=CARTESIAN_POINT('Ctrl Pts',(48.6205666139332,16.4830954176946,-22.5797338420621));
#17946=CARTESIAN_POINT('Ctrl Pts',(48.6088737900634,16.4830954176946,-22.6047435324921));
#17947=CARTESIAN_POINT('',(48.8335265683622,16.4830954176946,-44.2925682080603));
#17948=CARTESIAN_POINT('Origin',(50.0835265683621,16.4830954176946,0.0824317919395974));
#17949=CARTESIAN_POINT('',(50.0835265683619,-8.87385981233827,37.6072170232579));
#17950=CARTESIAN_POINT('',(50.0835265683619,-14.4544045823054,37.6072170232579));
#17951=CARTESIAN_POINT('',(50.0835265683619,16.4830954176946,37.6072170232579));
#17952=CARTESIAN_POINT('',(50.0835265683621,-8.87385981233827,44.4574317919394));
#17953=CARTESIAN_POINT('',(50.0835265683621,-8.87385981233827,0.0824317919395974));
#17954=CARTESIAN_POINT('',(50.0835265683621,-14.4544045823054,44.4574317919394));
#17955=CARTESIAN_POINT('',(50.0835265683621,16.4830954176946,44.4574317919394));
#17956=CARTESIAN_POINT('',(50.0835265683621,-14.4544045823054,0.0824317919395974));
#17957=CARTESIAN_POINT('Origin',(50.0835265683621,16.4830954176946,0.0824317919395974));
#17958=CARTESIAN_POINT('',(50.0835265683619,16.1705954176946,37.6072170232579));
#17959=CARTESIAN_POINT('',(50.0835265683619,13.4386401876617,37.6072170232579));
#17960=CARTESIAN_POINT('',(50.0835265683619,16.4830954176946,37.6072170232579));
#17961=CARTESIAN_POINT('',(50.0835265683621,16.1705954176946,44.4574317919394));
#17962=CARTESIAN_POINT('',(50.0835265683619,16.1705954176946,44.4574317919394));
#17963=CARTESIAN_POINT('',(50.0835265683621,13.4386401876617,44.4574317919394));
#17964=CARTESIAN_POINT('',(50.0835265683621,16.4830954176946,44.4574317919394));
#17965=CARTESIAN_POINT('',(50.0835265683621,13.4386401876617,0.0824317919395974));
#17966=CARTESIAN_POINT('Origin',(68.5210265683621,-8.56135981233827,0.0824317919394229));
#17967=CARTESIAN_POINT('',(46.9585265683621,-8.56135981233827,38.3884670232579));
#17968=CARTESIAN_POINT('',(46.9585265683621,-8.56135981233827,36.5987899438301));
#17969=CARTESIAN_POINT('',(46.9585265683619,-8.56135981233827,0.0824317919394977));
#17970=CARTESIAN_POINT('',(44.4818701996542,-8.56135981233827,35.7821111511702));
#17971=CARTESIAN_POINT('',(46.9585265683621,-8.56135981233827,36.5987899438301));
#17972=CARTESIAN_POINT('',(45.272154845105,-8.56135981233827,33.3854975524836));
#17973=CARTESIAN_POINT('',(44.4818701996542,-8.56135981233827,35.7821111511702));
#17974=CARTESIAN_POINT('',(48.8335265683621,-8.56135981233827,34.5598618267976));
#17975=CARTESIAN_POINT('',(45.272154845105,-8.56135981233827,33.3854975524836));
#17976=CARTESIAN_POINT('',(48.8335265683621,-8.56135981233827,36.6697170232579));
#17977=CARTESIAN_POINT('',(48.8335265683619,-8.56135981233827,0.0824317919394912));
#17978=CARTESIAN_POINT('',(49.7710265683619,-8.56135981233827,36.6697170232579));
#17979=CARTESIAN_POINT('',(68.5210265683621,-8.56135981233827,36.6697170232579));
#17980=CARTESIAN_POINT('',(49.771026568362,-8.56135981233827,22.7876789472104));
#17981=CARTESIAN_POINT('',(49.7710265683621,-8.56135981233827,0.0824317919393611));
#17982=CARTESIAN_POINT('',(39.5861451654569,-8.56135981233827,37.8172834360679));
#17983=CARTESIAN_POINT('Origin',(0.0835265683620477,-8.56135981233827,0.0824317919394229));
#17984=CARTESIAN_POINT('',(40.7421664865885,-8.56135981233827,38.9733047571995));
#17985=CARTESIAN_POINT('',(40.7421664865885,-8.56135981233827,38.9733047571995));
#17986=CARTESIAN_POINT('',(38.9743995336222,-8.56135981233827,40.7410717101659));
#17987=CARTESIAN_POINT('Origin',(39.8582830101054,-8.56135981233827,39.8571882336827));
#17988=CARTESIAN_POINT('',(37.8183782124906,-8.56135981233827,39.5850503890343));
#17989=CARTESIAN_POINT('',(37.7312605880988,-8.56135981233827,39.4979327646425));
#17990=CARTESIAN_POINT('',(22.7887737236329,-8.56135981233827,49.7699317919394));
#17991=CARTESIAN_POINT('Origin',(0.0835265683620477,-8.56135981233827,0.0824317919394229));
#17992=CARTESIAN_POINT('',(44.458526568362,-8.56135981233827,49.7699317919394));
#17993=CARTESIAN_POINT('',(68.5210265683621,-8.56135981233827,49.7699317919394));
#17994=CARTESIAN_POINT('',(49.7710265683619,-8.56135981233827,44.4574317919394));
#17995=CARTESIAN_POINT('Origin',(44.4585265683621,-8.56135981233827,44.4574317919394));
#17996=CARTESIAN_POINT('',(49.7710265683619,-8.56135981233827,37.6072170232579));
#17997=CARTESIAN_POINT('',(49.7710265683621,-8.56135981233827,0.0824317919393611));
#17998=CARTESIAN_POINT('',(48.8335265683621,-8.56135981233827,37.6072170232579));
#17999=CARTESIAN_POINT('',(68.5210265683621,-8.56135981233827,37.6072170232579));
#18000=CARTESIAN_POINT('',(48.8335265683621,-8.56135981233827,38.3884670232579));
#18001=CARTESIAN_POINT('',(48.8335265683619,-8.56135981233827,0.0824317919394912));
#18002=CARTESIAN_POINT('',(68.5210265683621,-8.56135981233827,38.3884670232579));
#18003=CARTESIAN_POINT('Origin',(50.833526568362,13.1261401876617,0.0824317919394229));
#18004=CARTESIAN_POINT('',(49.771026568362,13.1261401876617,37.6072170232579));
#18005=CARTESIAN_POINT('',(48.8335265683621,13.1261401876617,37.6072170232579));
#18006=CARTESIAN_POINT('',(50.833526568362,13.1261401876617,37.6072170232579));
#18007=CARTESIAN_POINT('',(49.7710265683619,13.1261401876617,44.4574317919394));
#18008=CARTESIAN_POINT('',(49.7710265683621,13.1261401876617,0.0824317919394194));
#18009=CARTESIAN_POINT('',(44.458526568362,13.1261401876617,49.7699317919394));
#18010=CARTESIAN_POINT('Origin',(44.4585265683621,13.1261401876617,44.4574317919394));
#18011=CARTESIAN_POINT('',(11.0320394968433,13.1261401876617,49.7699317919394));
#18012=CARTESIAN_POINT('',(50.8335265683621,13.1261401876617,49.7699317919394));
#18013=CARTESIAN_POINT('',(35.1659821576993,13.1261401876617,36.932654334243));
#18014=CARTESIAN_POINT('Origin',(0.0835265683620477,13.1261401876617,0.0824317919394229));
#18015=CARTESIAN_POINT('',(38.9743995336222,13.1261401876617,40.7410717101659));
#18016=CARTESIAN_POINT('',(36.9337491106657,13.1261401876617,35.1648873812767));
#18017=CARTESIAN_POINT('',(36.846955706336,13.1261401876617,35.078093976947));
#18018=CARTESIAN_POINT('',(49.771026568362,13.1261401876617,11.0309447204208));
#18019=CARTESIAN_POINT('Origin',(0.0835265683620477,13.1261401876617,0.0824317919394229));
#18020=CARTESIAN_POINT('',(49.771026568362,13.1261401876617,36.6697170232579));
#18021=CARTESIAN_POINT('',(49.7710265683621,13.1261401876617,0.0824317919394194));
#18022=CARTESIAN_POINT('',(48.8335265683621,13.1261401876617,36.6697170232579));
#18023=CARTESIAN_POINT('',(50.833526568362,13.1261401876617,36.6697170232579));
#18024=CARTESIAN_POINT('',(48.8335265683621,13.1261401876617,35.8884670232579));
#18025=CARTESIAN_POINT('',(48.8335265683619,13.1261401876617,0.0824317919394298));
#18026=CARTESIAN_POINT('',(46.958526568362,13.1261401876617,35.8884670232579));
#18027=CARTESIAN_POINT('',(50.833526568362,13.1261401876617,35.8884670232579));
#18028=CARTESIAN_POINT('',(46.9585265683621,13.1261401876617,38.3884670232579));
#18029=CARTESIAN_POINT('',(46.9585265683619,13.1261401876617,0.0824317919394363));
#18030=CARTESIAN_POINT('',(48.8335265683621,13.1261401876617,38.3884670232579));
#18031=CARTESIAN_POINT('',(50.833526568362,13.1261401876617,38.3884670232579));
#18032=CARTESIAN_POINT('',(48.8335265683619,13.1261401876617,0.0824317919394298));
#18033=CARTESIAN_POINT('Origin',(48.5210265683621,15.5455954176946,42.8336341598436));
#18034=CARTESIAN_POINT('',(48.5210265683621,15.8580954176946,38.3884670232579));
#18035=CARTESIAN_POINT('',(48.5210265683621,16.1705954176946,38.3884670232579));
#18036=CARTESIAN_POINT('',(48.5210265683621,15.5455954176946,38.3884670232579));
#18037=CARTESIAN_POINT('',(48.5210265683621,15.8580954176946,42.8336341598436));
#18038=CARTESIAN_POINT('',(48.5210265683621,16.4830954176946,40.1612670779183));
#18039=CARTESIAN_POINT('',(48.5210265683621,16.1705954176946,29.6248403980433));
#18040=CARTESIAN_POINT('Origin',(49.7710265683621,13.4386401876617,0.0824317919395964));
#18041=CARTESIAN_POINT('Origin',(49.7710265683619,13.4386401876617,37.6072170232579));
#18042=CARTESIAN_POINT('Origin',(49.7710265683619,13.4386401876617,44.4574317919394));
#18043=CARTESIAN_POINT('Origin',(49.7710265683621,-8.87385981233827,0.0824317919395964));
#18044=CARTESIAN_POINT('Origin',(49.7710265683619,-8.87385981233827,37.6072170232579));
#18045=CARTESIAN_POINT('Origin',(49.7710265683619,-8.87385981233827,44.4574317919394));
#18046=CARTESIAN_POINT('Origin',(49.7710265683621,-14.4544045823054,0.0824317919395964));
#18047=CARTESIAN_POINT('',(49.7710265683619,-14.7669045823054,37.6072170232579));
#18048=CARTESIAN_POINT('',(49.7710265683619,-14.7669045823054,44.4574317919394));
#18049=CARTESIAN_POINT('',(49.7710265683622,-14.7669045823054,-44.2925682080603));
#18050=CARTESIAN_POINT('Origin',(49.7710265683619,-14.4544045823054,37.6072170232579));
#18051=CARTESIAN_POINT('Origin',(49.7710265683619,-14.4544045823054,44.4574317919394));
#18052=CARTESIAN_POINT('Origin',(49.7710265683622,16.1705954176946,-44.2925682080603));
#18053=CARTESIAN_POINT('Origin',(49.7710265683619,16.1705954176946,37.6072170232579));
#18054=CARTESIAN_POINT('Origin',(49.7710265683619,16.1705954176946,44.4574317919394));
#18055=CARTESIAN_POINT('Origin',(48.8335265683621,16.1705954176946,42.8336341598436));
#18056=CARTESIAN_POINT('Origin',(48.8335265683621,16.1705954176946,38.3884670232579));
#18057=CARTESIAN_POINT('Origin',(48.2085265683621,15.8580954176946,0.0824317919394229));
#18058=CARTESIAN_POINT('',(48.2085265683621,15.5455954176946,38.3884670232579));
#18059=CARTESIAN_POINT('Origin',(48.2085265683621,15.8580954176946,38.3884670232579));
#18060=CARTESIAN_POINT('',(48.2085265683621,15.5455954176946,0.0824317919394229));
#18061=CARTESIAN_POINT('Origin',(-4.89277133898972,-11.0169045823054,15.1735300494181));
#18062=CARTESIAN_POINT('',(10.111699809421,-11.3294045823054,20.1212626201575));
#18063=CARTESIAN_POINT('',(15.8818970466764,-11.3294045823054,22.02398831625));
#18064=CARTESIAN_POINT('',(-4.89277133898972,-11.3294045823054,15.1735300494181));
#18065=CARTESIAN_POINT('',(15.8818970466764,-14.4544045823054,22.02398831625));
#18066=CARTESIAN_POINT('',(15.8818970466764,-11.0169045823054,22.02398831625));
#18067=CARTESIAN_POINT('',(10.111699809421,-14.4544045823054,20.1212626201575));
#18068=CARTESIAN_POINT('',(-4.89277133898972,-14.4544045823054,15.1735300494181));
#18069=CARTESIAN_POINT('',(10.111699809421,-11.0169045823054,20.1212626201575));
#18070=CARTESIAN_POINT('Origin',(-4.99063502851588,-14.4544045823054,15.4703110263562));
#18071=CARTESIAN_POINT('',(15.7840333571502,-14.7669045823054,22.3207692931881));
#18072=CARTESIAN_POINT('Origin',(15.7840333571502,-14.4544045823054,22.3207692931881));
#18073=CARTESIAN_POINT('',(10.0138361198949,-14.7669045823054,20.4180435970956));
#18074=CARTESIAN_POINT('',(-58.2113397045057,-14.7669045823054,-2.07924545974433));
#18075=CARTESIAN_POINT('Origin',(10.0138361198949,-14.4544045823054,20.4180435970956));
#18076=CARTESIAN_POINT('Origin',(-4.99063502851588,-11.3294045823054,15.4703110263562));
#18077=CARTESIAN_POINT('',(15.7840333571502,-11.0169045823054,22.3207692931881));
#18078=CARTESIAN_POINT('Origin',(15.7840333571502,-11.3294045823054,22.3207692931881));
#18079=CARTESIAN_POINT('',(10.0138361198949,-11.0169045823054,20.4180435970956));
#18080=CARTESIAN_POINT('Origin',(10.0138361198949,-11.3294045823054,20.4180435970956));
#18081=CARTESIAN_POINT('',(-4.99063502851588,-11.0169045823054,15.4703110263562));
#18082=CARTESIAN_POINT('Origin',(0.0835265683620477,-12.5794045823054,0.0824317919394229));
#18083=CARTESIAN_POINT('',(15.3925785990455,-12.5794045823054,23.5078932009404));
#18084=CARTESIAN_POINT('',(7.67510093260532,-12.5794045823054,20.9630507178886));
#18085=CARTESIAN_POINT('',(-5.38208978662056,-12.5794045823054,16.6574349341085));
#18086=CARTESIAN_POINT('',(7.59696574233659,-12.5794045823054,18.6174859267129));
#18087=CARTESIAN_POINT('Origin',(8.06655569071,-12.5794045823054,19.7759268101363));
#18088=CARTESIAN_POINT('',(-6.17974956131282,-12.5794045823054,19.076414315977));
#18089=CARTESIAN_POINT('Origin',(0.0835265683620477,-12.5794045823054,0.0824317919394229));
#18090=CARTESIAN_POINT('',(14.5949188243533,-12.5794045823054,25.9268725828089));
#18091=CARTESIAN_POINT('',(-6.17974956131282,-12.5794045823054,19.076414315977));
#18092=CARTESIAN_POINT('',(20.8581949540281,-12.5794045823054,6.93289005877128));
#18093=CARTESIAN_POINT('Origin',(0.083526568362047,-85.4775827009602,-48.3550682080606));
#18094=CARTESIAN_POINT('',(0.0835265683620966,-6.14692278878557,-48.3550682080606));
#18095=CARTESIAN_POINT('',(4.28505819640517,-6.32940458230551,-48.3550682080606));
#18096=CARTESIAN_POINT('Origin',(0.0819794890372154,-78.8840761885053,-48.3550682139743));
#18097=CARTESIAN_POINT('',(-4.11800505968097,-6.32940458230551,-48.3550682080606));
#18098=CARTESIAN_POINT('Origin',(0.0850736528295037,-78.8840761674478,-48.3550682141158));
#18099=CARTESIAN_POINT('',(-29.3897661934246,-14.4544067125512,-48.3550682080518));
#18100=CARTESIAN_POINT('Ctrl Pts',(-4.11800505968098,-6.32940458230551,
-48.3550682080575));
#18101=CARTESIAN_POINT('Ctrl Pts',(-7.23028203564418,-6.60009089469845,
-48.355068207831));
#18102=CARTESIAN_POINT('Ctrl Pts',(-10.2832623655178,-7.16548762139643,
-48.3550682009245));
#18103=CARTESIAN_POINT('Ctrl Pts',(-13.2881929703542,-7.96970396804477,
-48.3550682035663));
#18104=CARTESIAN_POINT('Ctrl Pts',(-14.5634332304672,-8.310999391452,-48.3550682046874));
#18105=CARTESIAN_POINT('Ctrl Pts',(-15.8300197329982,-8.69530573227847,
-48.3550682067606));
#18106=CARTESIAN_POINT('Ctrl Pts',(-17.0888126926591,-9.1183486423787,-48.3550682076745));
#18107=CARTESIAN_POINT('Ctrl Pts',(-17.2519209468127,-9.17316448001821,
-48.3550682077929));
#18108=CARTESIAN_POINT('Ctrl Pts',(-17.4148784256617,-9.22862227451152,
-48.3550682078197));
#18109=CARTESIAN_POINT('Ctrl Pts',(-17.5776977494185,-9.28471651645609,
-48.3550682078142));
#18110=CARTESIAN_POINT('Ctrl Pts',(-18.1582353086448,-9.48472234840386,
-48.3550682077949));
#18111=CARTESIAN_POINT('Ctrl Pts',(-18.7377862785179,-9.69311870418431,
-48.3550682069701));
#18112=CARTESIAN_POINT('Ctrl Pts',(-19.3151335384121,-9.9089582081689,-48.3550682065996));
#18113=CARTESIAN_POINT('Ctrl Pts',(-19.6244384053913,-10.0245908849067,
-48.3550682064011));
#18114=CARTESIAN_POINT('Ctrl Pts',(-19.9331105403827,-10.1423607380609,
-48.3550682065513));
#18115=CARTESIAN_POINT('Ctrl Pts',(-20.2409594146601,-10.2621272193483,
-48.3550682071088));
#18116=CARTESIAN_POINT('Ctrl Pts',(-20.4551588435133,-10.3454600297986,
-48.3550682074966));
#18117=CARTESIAN_POINT('Ctrl Pts',(-20.6689790522681,-10.4297627624244,
-48.3550682076939));
#18118=CARTESIAN_POINT('Ctrl Pts',(-20.8823303370506,-10.5149781806565,
-48.355068207817));
#18119=CARTESIAN_POINT('Ctrl Pts',(-21.7084873705318,-10.8449565878889,
-48.3550682082937));
#18120=CARTESIAN_POINT('Ctrl Pts',(-22.5282779369094,-11.1887405793905,
-48.3550682080817));
#18121=CARTESIAN_POINT('Ctrl Pts',(-23.3424573486984,-11.5450903892485,
-48.3550682080254));
#18122=CARTESIAN_POINT('Ctrl Pts',(-23.6003183388764,-11.6579509129724,
-48.3550682080076));
#18123=CARTESIAN_POINT('Ctrl Pts',(-23.8576082226002,-11.7720687209439,
-48.3550682079892));
#18124=CARTESIAN_POINT('Ctrl Pts',(-24.1143473570555,-11.8874012527357,
-48.355068207977));
#18125=CARTESIAN_POINT('Ctrl Pts',(-25.0059583796815,-12.2879313738297,
-48.3550682079346));
#18126=CARTESIAN_POINT('Ctrl Pts',(-25.8909652612289,-12.70304390055,-48.3550682079832));
#18127=CARTESIAN_POINT('Ctrl Pts',(-26.7699903573938,-13.1313454185227,
-48.3550682080198));
#18128=CARTESIAN_POINT('Ctrl Pts',(-27.6490154535586,-13.5596469364954,
-48.3550682080564));
#18129=CARTESIAN_POINT('Ctrl Pts',(-28.5220589757606,-14.0011371004764,
-48.3550682080606));
#18130=CARTESIAN_POINT('Ctrl Pts',(-29.3897729325326,-14.4543739218821,
-48.3550682080606));
#18131=CARTESIAN_POINT('',(29.5568215162337,-14.4544045823054,-48.3550682080606));
#18132=CARTESIAN_POINT('',(30.4844928359005,-14.4544045823054,-48.3550682080606));
#18133=CARTESIAN_POINT('Ctrl Pts',(29.5568262308554,-14.4543736123985,-48.3550682080606));
#18134=CARTESIAN_POINT('Ctrl Pts',(28.6887755859948,-14.0009603589244,-48.3550682080606));
#18135=CARTESIAN_POINT('Ctrl Pts',(27.8153643667776,-13.5592886344723,-48.3550682080563));
#18136=CARTESIAN_POINT('Ctrl Pts',(26.9359347762758,-13.1308037218343,-48.3550682080188));
#18137=CARTESIAN_POINT('Ctrl Pts',(26.056505185774,-12.7023188091962,-48.3550682079813));
#18138=CARTESIAN_POINT('Ctrl Pts',(25.1710570057786,-12.2870210611749,-48.3550682079315));
#18139=CARTESIAN_POINT('Ctrl Pts',(24.2789629867541,-11.8863062114338,-48.3550682079749));
#18140=CARTESIAN_POINT('Ctrl Pts',(24.0216212267556,-11.7707122689897,-48.3550682079874));
#18141=CARTESIAN_POINT('Ctrl Pts',(23.7637232181357,-11.6563375248582,-48.3550682080063));
#18142=CARTESIAN_POINT('Ctrl Pts',(23.5052482767864,-11.5432249100067,-48.3550682080246));
#18143=CARTESIAN_POINT('Ctrl Pts',(22.7812340028694,-11.2263851139127,-48.3550682080758));
#18144=CARTESIAN_POINT('Ctrl Pts',(22.0529935081657,-10.9195690669471,-48.3550682081345));
#18145=CARTESIAN_POINT('Ctrl Pts',(21.3194160810682,-10.6234156296954,-48.3550682079765));
#18146=CARTESIAN_POINT('Ctrl Pts',(21.2279594902917,-10.5864935779565,-48.3550682079568));
#18147=CARTESIAN_POINT('Ctrl Pts',(21.1364199114277,-10.5497373133991,-48.3550682079309));
#18148=CARTESIAN_POINT('Ctrl Pts',(21.044795160316,-10.5131481250887,-48.3550682078952));
#18149=CARTESIAN_POINT('Ctrl Pts',(20.8306342211836,-10.4276256561536,-48.3550682078117));
#18150=CARTESIAN_POINT('Ctrl Pts',(20.6160433656434,-10.343038687593,-48.3550682076774));
#18151=CARTESIAN_POINT('Ctrl Pts',(20.4010822779403,-10.2594333452067,-48.3550682074127));
#18152=CARTESIAN_POINT('Ctrl Pts',(19.8668935038345,-10.0516699968013,-48.355068206755));
#18153=CARTESIAN_POINT('Ctrl Pts',(19.3307765011361,-9.85012639361532,-48.3550682071424));
#18154=CARTESIAN_POINT('Ctrl Pts',(18.7933371416024,-9.6553764716246,-48.3550682075041));
#18155=CARTESIAN_POINT('Ctrl Pts',(18.4431914865909,-9.52849547977083,-48.3550682077397));
#18156=CARTESIAN_POINT('Ctrl Pts',(18.092483769791,-9.4044988724651,-48.3550682078824));
#18157=CARTESIAN_POINT('Ctrl Pts',(17.741376829569,-9.28355639505756,-48.3550682078902));
#18158=CARTESIAN_POINT('Ctrl Pts',(17.5775565924851,-9.2271267918435,-48.3550682078938));
#18159=CARTESIAN_POINT('Ctrl Pts',(17.4135884308508,-9.17133865071493,-48.3550682078751));
#18160=CARTESIAN_POINT('Ctrl Pts',(17.2494553456226,-9.11619658428714,-48.3550682077922));
#18161=CARTESIAN_POINT('Ctrl Pts',(15.6417454071451,-8.57607118482318,-48.3550682069807));
#18162=CARTESIAN_POINT('Ctrl Pts',(14.0213893603513,-8.09914440993566,-48.3550682048256));
#18163=CARTESIAN_POINT('Ctrl Pts',(12.386600966108,-7.69433778621075,-48.3550682041081));
#18164=CARTESIAN_POINT('Ctrl Pts',(10.8104759197869,-7.30405739223667,-48.3550682034163));
#18165=CARTESIAN_POINT('Ctrl Pts',(9.22093586202024,-6.98081413681076,-48.3550682041519));
#18166=CARTESIAN_POINT('Ctrl Pts',(7.61638998568351,-6.73255660071286,-48.3550682056399));
#18167=CARTESIAN_POINT('Ctrl Pts',(6.51321047809351,-6.56187115602289,-48.355068206663));
#18168=CARTESIAN_POINT('Ctrl Pts',(5.40293781007535,-6.42663073301706,-48.3550682079868));
#18169=CARTESIAN_POINT('Ctrl Pts',(4.28505819640523,-6.32940458230469,-48.3550682080579));
#18170=CARTESIAN_POINT('Origin',(48.5210265683621,-85.4775827009602,0.0824317919395913));
#18171=CARTESIAN_POINT('',(48.5210265683621,-6.14692278878556,0.0824317919396692));
#18172=CARTESIAN_POINT('',(48.521026568362,-6.32940458230551,4.28396341998264));
#18173=CARTESIAN_POINT('Origin',(48.5210265743607,-78.8840761814646,0.0808847117366288));
#18174=CARTESIAN_POINT('',(48.5210265683621,-6.32940458230548,-4.1190998361033));
#18175=CARTESIAN_POINT('Origin',(48.5210265744032,-78.8840761438039,0.0839788755104842));
#18176=CARTESIAN_POINT('',(48.5210265683534,-14.454406712551,-29.390860969846));
#18177=CARTESIAN_POINT('Ctrl Pts',(48.5210265683589,-6.32940458230548,-4.1190998361033));
#18178=CARTESIAN_POINT('Ctrl Pts',(48.5210265681324,-6.60009087956923,-7.23137663811504));
#18179=CARTESIAN_POINT('Ctrl Pts',(48.521026561226,-7.16548755819356,-10.2843568006686));
#18180=CARTESIAN_POINT('Ctrl Pts',(48.5210265638678,-7.96970383319668,-13.2892872429231));
#18181=CARTESIAN_POINT('Ctrl Pts',(48.5210265649889,-8.31099929022391,-14.5645276732667));
#18182=CARTESIAN_POINT('Ctrl Pts',(48.5210265670621,-8.69530567656249,-15.8311143436352));
#18183=CARTESIAN_POINT('Ctrl Pts',(48.521026567976,-9.11834864237817,-17.0899074690816));
#18184=CARTESIAN_POINT('Ctrl Pts',(48.5210265680944,-9.17316448001765,-17.2530157232352));
#18185=CARTESIAN_POINT('Ctrl Pts',(48.5210265681212,-9.22862227451093,-17.4159732020842));
#18186=CARTESIAN_POINT('Ctrl Pts',(48.5210265681158,-9.28471651645553,-17.578792525841));
#18187=CARTESIAN_POINT('Ctrl Pts',(48.5210265680965,-9.48472234837756,-18.1593300849925));
#18188=CARTESIAN_POINT('Ctrl Pts',(48.5210265672717,-9.69311870413019,-18.7388810547907));
#18189=CARTESIAN_POINT('Ctrl Pts',(48.5210265669012,-9.90895820808511,-19.3162283146108));
#18190=CARTESIAN_POINT('Ctrl Pts',(48.5210265667027,-10.0245908848499,-19.6255331816648));
#18191=CARTESIAN_POINT('Ctrl Pts',(48.5210265668528,-10.1423607380321,-19.9342053167309));
#18192=CARTESIAN_POINT('Ctrl Pts',(48.5210265674103,-10.2621272193483,-20.2420541910824));
#18193=CARTESIAN_POINT('Ctrl Pts',(48.5210265677982,-10.3454600297987,-20.4562536199356));
#18194=CARTESIAN_POINT('Ctrl Pts',(48.5210265679954,-10.4297627624243,-20.6700738286905));
#18195=CARTESIAN_POINT('Ctrl Pts',(48.5210265681185,-10.5149781806561,-20.8834251134732));
#18196=CARTESIAN_POINT('Ctrl Pts',(48.5210265685952,-10.8449565878873,-21.7095821469555));
#18197=CARTESIAN_POINT('Ctrl Pts',(48.5210265683833,-11.1887405793895,-22.5293727133321));
#18198=CARTESIAN_POINT('Ctrl Pts',(48.521026568327,-11.5450903892478,-23.3435521251211));
#18199=CARTESIAN_POINT('Ctrl Pts',(48.5210265683092,-11.6579509129718,-23.6014131152991));
#18200=CARTESIAN_POINT('Ctrl Pts',(48.5210265682908,-11.7720687209433,-23.8587029990229));
#18201=CARTESIAN_POINT('Ctrl Pts',(48.5210265682786,-11.8874012527351,-24.1154421334782));
#18202=CARTESIAN_POINT('Ctrl Pts',(48.5210265682361,-12.287931373829,-25.0070531561044));
#18203=CARTESIAN_POINT('Ctrl Pts',(48.5210265682847,-12.7030439005514,-25.8920600376509));
#18204=CARTESIAN_POINT('Ctrl Pts',(48.5210265683213,-13.1313454185256,-26.7710851338149));
#18205=CARTESIAN_POINT('Ctrl Pts',(48.521026568358,-13.5596469364998,-27.6501102299789));
#18206=CARTESIAN_POINT('Ctrl Pts',(48.5210265683622,-14.0011371004819,-28.5231537521802));
#18207=CARTESIAN_POINT('Ctrl Pts',(48.5210265683622,-14.4543739218857,-29.3908677089532));
#18208=CARTESIAN_POINT('',(48.5210265683619,-14.4544045823054,29.5557267398091));
#18209=CARTESIAN_POINT('',(48.5210265683619,-14.4544045823054,30.4833980594777));
#18210=CARTESIAN_POINT('Ctrl Pts',(48.5210265683619,-14.4543736124042,29.55573145443));
#18211=CARTESIAN_POINT('Ctrl Pts',(48.5210265683619,-14.0009603589333,28.687680809568));
#18212=CARTESIAN_POINT('Ctrl Pts',(48.5210265683577,-13.5592886344784,27.8142695903511));
#18213=CARTESIAN_POINT('Ctrl Pts',(48.5210265683202,-13.1308037218372,26.9348399998503));
#18214=CARTESIAN_POINT('Ctrl Pts',(48.5210265682827,-12.702318809196,26.0554104093494));
#18215=CARTESIAN_POINT('Ctrl Pts',(48.5210265682328,-12.2870210611714,25.1699622293556));
#18216=CARTESIAN_POINT('Ctrl Pts',(48.5210265682762,-11.8863062114323,24.2778682103323));
#18217=CARTESIAN_POINT('Ctrl Pts',(48.5210265682888,-11.7707122689886,24.0205264503339));
#18218=CARTESIAN_POINT('Ctrl Pts',(48.5210265683076,-11.656337524857,23.762628441714));
#18219=CARTESIAN_POINT('Ctrl Pts',(48.5210265683259,-11.5432249100052,23.5041535003646));
#18220=CARTESIAN_POINT('Ctrl Pts',(48.5210265683772,-11.2263851140862,22.7801392268488));
#18221=CARTESIAN_POINT('Ctrl Pts',(48.5210265684358,-10.9195690672826,22.051898732552));
#18222=CARTESIAN_POINT('Ctrl Pts',(48.5210265682779,-10.6234156301853,21.3183213058656));
#18223=CARTESIAN_POINT('Ctrl Pts',(48.5210265682582,-10.5864935782812,21.2268647146834));
#18224=CARTESIAN_POINT('Ctrl Pts',(48.5210265682323,-10.54973731356,21.135325135413));
#18225=CARTESIAN_POINT('Ctrl Pts',(48.5210265681966,-10.5131481250875,21.043700383894));
#18226=CARTESIAN_POINT('Ctrl Pts',(48.5210265681131,-10.4276256561534,20.8295394447612));
#18227=CARTESIAN_POINT('Ctrl Pts',(48.5210265679788,-10.3430386875933,20.6149485892208));
#18228=CARTESIAN_POINT('Ctrl Pts',(48.5210265677141,-10.2594333452069,20.3999875015178));
#18229=CARTESIAN_POINT('Ctrl Pts',(48.5210265670564,-10.0516699968362,19.8657987275014));
#18230=CARTESIAN_POINT('Ctrl Pts',(48.5210265674438,-9.85012639368244,19.3296817248934));
#18231=CARTESIAN_POINT('Ctrl Pts',(48.5210265678055,-9.65537647172188,18.7922423654503));
#18232=CARTESIAN_POINT('Ctrl Pts',(48.5210265680411,-9.52849547983389,18.4420967103491));
#18233=CARTESIAN_POINT('Ctrl Pts',(48.5210265681838,-9.40449887249552,18.0913889934592));
#18234=CARTESIAN_POINT('Ctrl Pts',(48.5210265681916,-9.2835563950572,17.7402820531467));
#18235=CARTESIAN_POINT('Ctrl Pts',(48.5210265681952,-9.2271267918433,17.5764618160627));
#18236=CARTESIAN_POINT('Ctrl Pts',(48.5210265681765,-9.17133865071483,17.4124936544283));
#18237=CARTESIAN_POINT('Ctrl Pts',(48.5210265680936,-9.11619658428705,17.2483605692001));
#18238=CARTESIAN_POINT('Ctrl Pts',(48.5210265672821,-8.57607118524294,15.6406506319723));
#18239=CARTESIAN_POINT('Ctrl Pts',(48.521026565127,-8.09914441067713,14.020294586448));
#18240=CARTESIAN_POINT('Ctrl Pts',(48.5210265644095,-7.69433778715491,12.3855061934978));
#18241=CARTESIAN_POINT('Ctrl Pts',(48.5210265637178,-7.30405739322943,10.8093811478304));
#18242=CARTESIAN_POINT('Ctrl Pts',(48.5210265644534,-6.98081413779193,9.21984109072944));
#18243=CARTESIAN_POINT('Ctrl Pts',(48.5210265659414,-6.73255660161266,7.6152952150723));
#18244=CARTESIAN_POINT('Ctrl Pts',(48.5210265669644,-6.56187115649859,6.51211570557005));
#18245=CARTESIAN_POINT('Ctrl Pts',(48.5210265682882,-6.42663073318859,5.40184303561563));
#18246=CARTESIAN_POINT('Ctrl Pts',(48.5210265683593,-6.32940458230551,4.28396341998264));
#18247=CARTESIAN_POINT('Origin',(-48.3539734316379,-85.4775827009602,-44.2925682080605));
#18248=CARTESIAN_POINT('',(-48.3539734316379,11.6131136241746,0.0824317919394229));
#18249=CARTESIAN_POINT('',(-48.3539734316379,11.7955954176947,4.28396341998245));
#18250=CARTESIAN_POINT('Origin',(-48.3539734376649,84.3502670064654,0.0808847007703356));
#18251=CARTESIAN_POINT('',(-48.3539734316379,11.7955954176947,-4.11909983610361));
#18252=CARTESIAN_POINT('Origin',(-48.3539734316379,84.3502670509921,0.0839788788605111));
#18253=CARTESIAN_POINT('',(-48.3539734315249,16.1706033824528,-21.353305195093));
#18254=CARTESIAN_POINT('Ctrl Pts',(-48.3539734316379,11.7955954176947,-4.11909983610361));
#18255=CARTESIAN_POINT('Ctrl Pts',(-48.353973431634,11.9012754521151,-5.3341798859156));
#18256=CARTESIAN_POINT('Ctrl Pts',(-48.3539734314967,12.0520583764943,-6.54394408577816));
#18257=CARTESIAN_POINT('Ctrl Pts',(-48.3539734315406,12.2455340422119,-7.74867686713406));
#18258=CARTESIAN_POINT('Ctrl Pts',(-48.3539734315501,12.2874241550106,-8.00951789805218));
#18259=CARTESIAN_POINT('Ctrl Pts',(-48.3539734315666,12.3313158172651,-8.27012304299333));
#18260=CARTESIAN_POINT('Ctrl Pts',(-48.3539734315853,12.3771848834513,-8.53049515220305));
#18261=CARTESIAN_POINT('Ctrl Pts',(-48.3539734315909,12.3910255799847,-8.60906076622044));
#18262=CARTESIAN_POINT('Ctrl Pts',(-48.3539734315881,12.4050450140598,-8.68760078593728));
#18263=CARTESIAN_POINT('Ctrl Pts',(-48.3539734315757,12.4192427232385,-8.7661163838354));
#18264=CARTESIAN_POINT('Ctrl Pts',(-48.3539734314889,12.5191317203699,-9.31851848156123));
#18265=CARTESIAN_POINT('Ctrl Pts',(-48.3539734306321,12.6280707956224,-9.8704261542129));
#18266=CARTESIAN_POINT('Ctrl Pts',(-48.3539734253286,12.7454889374165,-10.4210002063411));
#18267=CARTESIAN_POINT('Ctrl Pts',(-48.3539734198873,12.8659559514451,-10.9858704303805));
#18268=CARTESIAN_POINT('Ctrl Pts',(-48.3539734095596,12.9953485174401,-11.5493381718557));
#18269=CARTESIAN_POINT('Ctrl Pts',(-48.3539734075923,13.1331031833232,-12.1104878242374));
#18270=CARTESIAN_POINT('Ctrl Pts',(-48.3539734066747,13.1973553945651,-12.3722220150321));
#18271=CARTESIAN_POINT('Ctrl Pts',(-48.3539734078578,13.2634275010588,-12.6334516466247));
#18272=CARTESIAN_POINT('Ctrl Pts',(-48.3539734114491,13.3312657045535,-12.8940818979516));
#18273=CARTESIAN_POINT('Ctrl Pts',(-48.3539734141449,13.3821877700732,-13.089721376163));
#18274=CARTESIAN_POINT('Ctrl Pts',(-48.353973416395,13.4341067575185,-13.2850480331676));
#18275=CARTESIAN_POINT('Ctrl Pts',(-48.3539734183061,13.4869947668895,-13.4800014094153));
#18276=CARTESIAN_POINT('Ctrl Pts',(-48.3539734261861,13.7050584674933,-14.2838179110258));
#18277=CARTESIAN_POINT('Ctrl Pts',(-48.3539734286587,13.9395350033133,-15.0824829261137));
#18278=CARTESIAN_POINT('Ctrl Pts',(-48.3539734300256,14.1892982822773,-15.8762917931586));
#18279=CARTESIAN_POINT('Ctrl Pts',(-48.3539734314172,14.4435598427712,-16.6843973005252));
#18280=CARTESIAN_POINT('Ctrl Pts',(-48.3539734315029,14.7136635661991,-17.487470208706));
#18281=CARTESIAN_POINT('Ctrl Pts',(-48.3539734315848,14.9983707523295,-18.2858425197307));
#18282=CARTESIAN_POINT('Ctrl Pts',(-48.3539734316691,15.2915959446077,-19.108100916477));
#18283=CARTESIAN_POINT('Ctrl Pts',(-48.3539734316379,15.6003113763674,-19.9253732888144));
#18284=CARTESIAN_POINT('Ctrl Pts',(-48.353973431638,15.9231126704198,-20.738043122766));
#18285=CARTESIAN_POINT('Ctrl Pts',(-48.353973431638,16.0046899473676,-20.9434183592749));
#18286=CARTESIAN_POINT('Ctrl Pts',(-48.353973431638,16.0871665857534,-21.1484997497311));
#18287=CARTESIAN_POINT('Ctrl Pts',(-48.353973431638,16.1705194395641,-21.3532936780839));
#18288=CARTESIAN_POINT('',(-48.3539734315243,16.1706033612909,21.5181686663419));
#18289=CARTESIAN_POINT('',(-48.3539734316379,16.1705954176946,-44.2925682080605));
#18290=CARTESIAN_POINT('Ctrl Pts',(-48.3539734316379,16.1705196413371,21.5181571799855));
#18291=CARTESIAN_POINT('Ctrl Pts',(-48.3539734316379,15.8435202227306,20.7147347555301));
#18292=CARTESIAN_POINT('Ctrl Pts',(-48.3539734316511,15.5300086685144,19.9068834941557));
#18293=CARTESIAN_POINT('Ctrl Pts',(-48.3539734316247,15.231367963442,19.0942317333251));
#18294=CARTESIAN_POINT('Ctrl Pts',(-48.3539734315988,14.9390610385349,18.2988152572923));
#18295=CARTESIAN_POINT('Ctrl Pts',(-48.3539734316217,14.661001060423,17.498799666427));
#18296=CARTESIAN_POINT('Ctrl Pts',(-48.3539734308659,14.3984390229057,16.6938550497342));
#18297=CARTESIAN_POINT('Ctrl Pts',(-48.3539734301297,14.1426624799502,15.9097129350739));
#18298=CARTESIAN_POINT('Ctrl Pts',(-48.3539734287875,13.9015932981126,15.1208932392611));
#18299=CARTESIAN_POINT('Ctrl Pts',(-48.3539734237001,13.6763418781396,14.327109601817));
#18300=CARTESIAN_POINT('Ctrl Pts',(-48.3539734222457,13.611948351827,14.100187491624));
#18301=CARTESIAN_POINT('Ctrl Pts',(-48.3539734204628,13.5488472152034,13.8728598288434));
#18302=CARTESIAN_POINT('Ctrl Pts',(-48.3539734182148,13.4870636734944,13.6451202163981));
#18303=CARTESIAN_POINT('Ctrl Pts',(-48.3539734162904,13.4341751304698,13.4501683577308));
#18304=CARTESIAN_POINT('Ctrl Pts',(-48.3539734140247,13.3822549873807,13.2548408272286));
#18305=CARTESIAN_POINT('Ctrl Pts',(-48.3539734113102,13.3313312754875,13.0591984279295));
#18306=CARTESIAN_POINT('Ctrl Pts',(-48.3539734035448,13.1856558716878,12.4995321259522));
#18307=CARTESIAN_POINT('Ctrl Pts',(-48.3539734087768,13.0481153498403,11.9370799621826));
#18308=CARTESIAN_POINT('Ctrl Pts',(-48.3539734159749,12.9192577967628,11.3727821628695));
#18309=CARTESIAN_POINT('Ctrl Pts',(-48.3539734230251,12.7930466643237,10.8200736674549));
#18310=CARTESIAN_POINT('Ctrl Pts',(-48.3539734290975,12.675165032771,10.2655932894663));
#18311=CARTESIAN_POINT('Ctrl Pts',(-48.3539734306761,12.5661734819508,9.71020714836219));
#18312=CARTESIAN_POINT('Ctrl Pts',(-48.3539734314138,12.515246017069,9.45069704887183));
#18313=CARTESIAN_POINT('Ctrl Pts',(-48.3539734315343,12.4662602455005,9.19098905945248));
#18314=CARTESIAN_POINT('Ctrl Pts',(-48.3539734315754,12.4192773203286,8.9311713748959));
#18315=CARTESIAN_POINT('Ctrl Pts',(-48.3539734315878,12.4050773744282,8.85264503684491));
#18316=CARTESIAN_POINT('Ctrl Pts',(-48.3539734315907,12.3910557938715,8.77409450616072));
#18317=CARTESIAN_POINT('Ctrl Pts',(-48.353973431585,12.3772130393338,8.695518620036));
#18318=CARTESIAN_POINT('Ctrl Pts',(-48.3539734314988,12.1658567957286,7.49579322693565));
#18319=CARTESIAN_POINT('Ctrl Pts',(-48.3539734315723,11.9964818470948,6.29113564323276));
#18320=CARTESIAN_POINT('Ctrl Pts',(-48.3539734316199,11.8714667021317,5.08126600825786));
#18321=CARTESIAN_POINT('Ctrl Pts',(-48.3539734316303,11.8440311371517,4.81575052213465));
#18322=CARTESIAN_POINT('Ctrl Pts',(-48.353973431637,11.8187322169269,4.54998399158691));
#18323=CARTESIAN_POINT('Ctrl Pts',(-48.3539734316379,11.7955954176945,4.28396341998246));
#18324=CARTESIAN_POINT('Origin',(0.0835265683620484,-85.4775827009602,48.5199317919394));
#18325=CARTESIAN_POINT('',(0.0835265683620147,-6.14692278878557,48.5199317919394));
#18326=CARTESIAN_POINT('',(-4.11800505968107,-6.32940458230551,48.5199317919394));
#18327=CARTESIAN_POINT('Origin',(0.0850736476760322,-78.8840761880214,48.5199317979381));
#18328=CARTESIAN_POINT('',(4.2850581964051,-6.32940458230551,48.5199317919394));
#18329=CARTESIAN_POINT('Origin',(0.0819794837711729,-78.8840761734555,48.5199317979947));
#18330=CARTESIAN_POINT('',(29.5568193301503,-14.4544067125516,48.5199317919306));
#18331=CARTESIAN_POINT('Ctrl Pts',(4.2850581964051,-6.3294045823055,48.5199317919363));
#18332=CARTESIAN_POINT('Ctrl Pts',(7.39733506399622,-6.60009088527294,48.5199317917098));
#18333=CARTESIAN_POINT('Ctrl Pts',(10.450315289629,-7.16548758202087,48.5199317848033));
#18334=CARTESIAN_POINT('Ctrl Pts',(13.4552457931766,-7.96970388403428,48.5199317874451));
#18335=CARTESIAN_POINT('Ctrl Pts',(14.7304861593436,-8.3109993283869,48.5199317885663));
#18336=CARTESIAN_POINT('Ctrl Pts',(15.9970727664377,-8.69530569756759,48.5199317906394));
#18337=CARTESIAN_POINT('Ctrl Pts',(17.2558658293831,-9.11834864237876,48.5199317915533));
#18338=CARTESIAN_POINT('Ctrl Pts',(17.4189740835368,-9.17316448001826,48.5199317916717));
#18339=CARTESIAN_POINT('Ctrl Pts',(17.5819315623858,-9.2286222745116,48.5199317916985));
#18340=CARTESIAN_POINT('Ctrl Pts',(17.7447508861427,-9.28471651645626,48.5199317916931));
#18341=CARTESIAN_POINT('Ctrl Pts',(18.3252884455851,-9.48472234847866,48.5199317916738));
#18342=CARTESIAN_POINT('Ctrl Pts',(18.9048394156729,-9.69311870433946,48.519931790849));
#18343=CARTESIAN_POINT('Ctrl Pts',(19.4821866757799,-9.90895820840961,48.5199317904785));
#18344=CARTESIAN_POINT('Ctrl Pts',(19.7914915425436,-10.0245908850701,48.51993179028));
#18345=CARTESIAN_POINT('Ctrl Pts',(20.1001636773203,-10.142360738144,48.5199317904301));
#18346=CARTESIAN_POINT('Ctrl Pts',(20.4080125513842,-10.2621272193482,48.5199317909876));
#18347=CARTESIAN_POINT('Ctrl Pts',(20.6222119802371,-10.3454600297985,48.5199317913755));
#18348=CARTESIAN_POINT('Ctrl Pts',(20.836032188992,-10.4297627624242,48.5199317915727));
#18349=CARTESIAN_POINT('Ctrl Pts',(21.049383473775,-10.5149781806563,48.5199317916958));
#18350=CARTESIAN_POINT('Ctrl Pts',(21.8755405072593,-10.8449565878891,48.5199317921725));
#18351=CARTESIAN_POINT('Ctrl Pts',(22.6953310736331,-11.1887405793906,48.5199317919606));
#18352=CARTESIAN_POINT('Ctrl Pts',(23.5095104854225,-11.5450903892486,48.5199317919043));
#18353=CARTESIAN_POINT('Ctrl Pts',(23.7673714756,-11.6579509129722,48.5199317918865));
#18354=CARTESIAN_POINT('Ctrl Pts',(24.0246613593238,-11.7720687209435,48.5199317918681));
#18355=CARTESIAN_POINT('Ctrl Pts',(24.2814004937799,-11.8874012527353,48.5199317918559));
#18356=CARTESIAN_POINT('Ctrl Pts',(25.1730115164114,-12.2879313738302,48.5199317918134));
#18357=CARTESIAN_POINT('Ctrl Pts',(26.0580183979601,-12.7030439005477,48.519931791862));
#18358=CARTESIAN_POINT('Ctrl Pts',(26.9370434941245,-13.1313454185182,48.5199317918986));
#18359=CARTESIAN_POINT('Ctrl Pts',(27.8160685902889,-13.5596469364886,48.5199317919352));
#18360=CARTESIAN_POINT('Ctrl Pts',(28.6891121124888,-14.001137100468,48.5199317919394));
#18361=CARTESIAN_POINT('Ctrl Pts',(29.5568260692594,-14.4543739218769,48.5199317919394));
#18362=CARTESIAN_POINT('',(-29.3897683795096,-14.4544045823054,48.5199317919394));
#18363=CARTESIAN_POINT('',(-30.3174396991767,-14.4544045823054,48.5199317919394));
#18364=CARTESIAN_POINT('Ctrl Pts',(-29.3897730941313,-14.4543736123985,
48.5199317919394));
#18365=CARTESIAN_POINT('Ctrl Pts',(-28.5217224492708,-14.0009603589245,
48.5199317919394));
#18366=CARTESIAN_POINT('Ctrl Pts',(-27.6483112300529,-13.5592886344715,
48.5199317919352));
#18367=CARTESIAN_POINT('Ctrl Pts',(-26.7688816395507,-13.1308037218328,
48.5199317918976));
#18368=CARTESIAN_POINT('Ctrl Pts',(-25.8894520490486,-12.702318809194,48.5199317918601));
#18369=CARTESIAN_POINT('Ctrl Pts',(-25.0040038690532,-12.2870210611724,
48.5199317918103));
#18370=CARTESIAN_POINT('Ctrl Pts',(-24.1119098500306,-11.8863062114326,
48.5199317918537));
#18371=CARTESIAN_POINT('Ctrl Pts',(-23.8545680900323,-11.7707122689887,
48.5199317918662));
#18372=CARTESIAN_POINT('Ctrl Pts',(-23.5966700814124,-11.656337524857,48.5199317918851));
#18373=CARTESIAN_POINT('Ctrl Pts',(-23.338195140063,-11.5432249100053,48.5199317919034));
#18374=CARTESIAN_POINT('Ctrl Pts',(-22.614180866145,-11.2263851139103,48.5199317919547));
#18375=CARTESIAN_POINT('Ctrl Pts',(-21.8859403714393,-10.9195690669419,
48.5199317920133));
#18376=CARTESIAN_POINT('Ctrl Pts',(-21.1523629443404,-10.6234156296919,
48.5199317918553));
#18377=CARTESIAN_POINT('Ctrl Pts',(-21.0609063535652,-10.5864935779538,
48.5199317918356));
#18378=CARTESIAN_POINT('Ctrl Pts',(-20.9693667747026,-10.5497373133972,
48.5199317918098));
#18379=CARTESIAN_POINT('Ctrl Pts',(-20.8777420235922,-10.5131481250878,
48.5199317917741));
#18380=CARTESIAN_POINT('Ctrl Pts',(-20.6635810844597,-10.4276256561535,
48.5199317916905));
#18381=CARTESIAN_POINT('Ctrl Pts',(-20.4489902289193,-10.3430386875933,
48.5199317915563));
#18382=CARTESIAN_POINT('Ctrl Pts',(-20.2340291412162,-10.2594333452069,
48.5199317912916));
#18383=CARTESIAN_POINT('Ctrl Pts',(-19.6998403673666,-10.051669996901,48.5199317906338));
#18384=CARTESIAN_POINT('Ctrl Pts',(-19.1637233649263,-9.85012639380828,
48.5199317910213));
#18385=CARTESIAN_POINT('Ctrl Pts',(-18.6262840056516,-9.6553764719043,48.5199317913829));
#18386=CARTESIAN_POINT('Ctrl Pts',(-18.2761383503831,-9.52849547995278,
48.5199317916186));
#18387=CARTESIAN_POINT('Ctrl Pts',(-17.9254306333254,-9.40449887255358,
48.5199317917613));
#18388=CARTESIAN_POINT('Ctrl Pts',(-17.574323692845,-9.28355639505737,48.519931791769));
#18389=CARTESIAN_POINT('Ctrl Pts',(-17.410503455761,-9.22712679184346,48.5199317917726));
#18390=CARTESIAN_POINT('Ctrl Pts',(-17.2465352941267,-9.17133865071499,
48.5199317917539));
#18391=CARTESIAN_POINT('Ctrl Pts',(-17.0824022088985,-9.11619658428719,
48.5199317916711));
#18392=CARTESIAN_POINT('Ctrl Pts',(-15.4746922696518,-8.57607118456477,
48.5199317908595));
#18393=CARTESIAN_POINT('Ctrl Pts',(-13.8543362220765,-8.09914440947939,
48.5199317887045));
#18394=CARTESIAN_POINT('Ctrl Pts',(-12.219547827037,-7.69433778562994,48.519931787987));
#18395=CARTESIAN_POINT('Ctrl Pts',(-10.6434227803378,-7.30405739163223,
48.5199317872952));
#18396=CARTESIAN_POINT('Ctrl Pts',(-9.0538827221862,-6.98081413621769,48.5199317880308));
#18397=CARTESIAN_POINT('Ctrl Pts',(-7.44933684545642,-6.73255660017158,
48.5199317895188));
#18398=CARTESIAN_POINT('Ctrl Pts',(-6.34615733901905,-6.56187115573737,
48.5199317905419));
#18399=CARTESIAN_POINT('Ctrl Pts',(-5.23588467216803,-6.42663073291497,
48.5199317918656));
#18400=CARTESIAN_POINT('Ctrl Pts',(-4.11800505968107,-6.3294045823055,48.5199317919367));
#18401=CARTESIAN_POINT('Origin',(0.0835265683620477,-6.01690458230549,0.0824317919394229));
#18402=CARTESIAN_POINT('',(-45.805095386722,-13.2959337131846,-31.5176630410747));
#18403=CARTESIAN_POINT('',(-46.7085547781037,-13.2959337131846,-30.163770311099));
#18404=CARTESIAN_POINT('Origin',(0.0835265683620477,-13.2959337131846,0.0824317919394229));
#18405=CARTESIAN_POINT('',(-46.4447277393149,-12.6709337131846,-29.4166890942607));
#18406=CARTESIAN_POINT('Ctrl Pts',(-46.7085547781037,-13.2959337131846,
-30.163770311099));
#18407=CARTESIAN_POINT('Ctrl Pts',(-46.7308018048241,-13.2959337131846,
-30.129353273202));
#18408=CARTESIAN_POINT('Ctrl Pts',(-46.7494092222397,-13.2919430659168,
-30.0931246196562));
#18409=CARTESIAN_POINT('Ctrl Pts',(-46.7639937886785,-13.2842290832231,
-30.0561954407828));
#18410=CARTESIAN_POINT('Ctrl Pts',(-46.7786223726414,-13.2764918190406,
-30.0191548063493));
#18411=CARTESIAN_POINT('Ctrl Pts',(-46.7892044314641,-13.2650083398592,
-29.9814076918208));
#18412=CARTESIAN_POINT('Ctrl Pts',(-46.7953183242711,-13.2500137812566,
-29.9440648720613));
#18413=CARTESIAN_POINT('Ctrl Pts',(-46.7975557030175,-13.2445265233364,
-29.9303992691638));
#18414=CARTESIAN_POINT('Ctrl Pts',(-46.7991943226864,-13.2385687578685,
-29.9167878375396));
#18415=CARTESIAN_POINT('Ctrl Pts',(-46.800212090454,-13.2321510039651,-29.9032853674899));
#18416=CARTESIAN_POINT('Ctrl Pts',(-46.8002328818205,-13.2320198995248,
-29.9030095336383));
#18417=CARTESIAN_POINT('Ctrl Pts',(-46.8002534141945,-13.2318886036913,
-29.9027337461559));
#18418=CARTESIAN_POINT('Ctrl Pts',(-46.8002736873875,-13.2317571165657,
-29.9024580055318));
#18419=CARTESIAN_POINT('Ctrl Pts',(-46.8037330656023,-13.2093204091686,
-29.855406161685));
#18420=CARTESIAN_POINT('Ctrl Pts',(-46.7999626260835,-13.182136836623,-29.8107688763396));
#18421=CARTESIAN_POINT('Ctrl Pts',(-46.7906793329817,-13.1520894283718,
-29.7694085048952));
#18422=CARTESIAN_POINT('Ctrl Pts',(-46.7828212048694,-13.1266548782729,
-29.7343977501966));
#18423=CARTESIAN_POINT('Ctrl Pts',(-46.7710141350354,-13.0991694705396,
-29.7017353456062));
#18424=CARTESIAN_POINT('Ctrl Pts',(-46.7563177878289,-13.0707895719797,
-29.6719424887082));
#18425=CARTESIAN_POINT('Ctrl Pts',(-46.7561779609415,-13.0705195543472,
-29.6716590276285));
#18426=CARTESIAN_POINT('Ctrl Pts',(-46.7560378601023,-13.0702494422352,
-29.6713758206481));
#18427=CARTESIAN_POINT('Ctrl Pts',(-46.7558974863178,-13.0699792367999,
-29.6710928683671));
#18428=CARTESIAN_POINT('Ctrl Pts',(-46.7457918813678,-13.0505269623226,
-29.6507229397278));
#18429=CARTESIAN_POINT('Ctrl Pts',(-46.73431142011,-13.0305367697067,-29.6315119049251));
#18430=CARTESIAN_POINT('Ctrl Pts',(-46.7216707893827,-13.0101903794928,
-29.6134615953136));
#18431=CARTESIAN_POINT('Ctrl Pts',(-46.7142947412409,-12.9983178743173,
-29.6029288967844));
#18432=CARTESIAN_POINT('Ctrl Pts',(-46.7065242359664,-12.9863240855344,
-29.5927905109074));
#18433=CARTESIAN_POINT('Ctrl Pts',(-46.6984056317191,-12.9742444051773,
-29.5830396522533));
#18434=CARTESIAN_POINT('Ctrl Pts',(-46.6872931082818,-12.9577100691025,
-29.5696929436287));
#18435=CARTESIAN_POINT('Ctrl Pts',(-46.6755261223313,-12.9410147689399,
-29.5570758028062));
#18436=CARTESIAN_POINT('Ctrl Pts',(-46.6632182383888,-12.9242496162066,
-29.5451798612475));
#18437=CARTESIAN_POINT('Ctrl Pts',(-46.6570642964176,-12.9158670398399,
-29.5392318904681));
#18438=CARTESIAN_POINT('Ctrl Pts',(-46.6507751298663,-12.9074670004228,
-29.5334642194506));
#18439=CARTESIAN_POINT('Ctrl Pts',(-46.6443649334478,-12.8990608878296,
-29.5278758016581));
#18440=CARTESIAN_POINT('Ctrl Pts',(-46.6379547370293,-12.8906547752363,
-29.5222873838655));
#18441=CARTESIAN_POINT('Ctrl Pts',(-46.6314235107303,-12.8822425894822,
-29.5168782192877));
#18442=CARTESIAN_POINT('Ctrl Pts',(-46.6247854486351,-12.8738357211132,
-29.5116472610983));
#18443=CARTESIAN_POINT('Ctrl Pts',(-46.6039049055347,-12.8473912596424,
-29.4951928733019));
#18444=CARTESIAN_POINT('Ctrl Pts',(-46.58177099161,-12.8207472740161,-29.4803404238949));
#18445=CARTESIAN_POINT('Ctrl Pts',(-46.5586011720367,-12.7940681980357,
-29.467056051049));
#18446=CARTESIAN_POINT('Ctrl Pts',(-46.5523076389907,-12.7868214585527,
-29.4634476656131));
#18447=CARTESIAN_POINT('Ctrl Pts',(-46.5459376589846,-12.7795722581759,
-29.4599552418543));
#18448=CARTESIAN_POINT('Ctrl Pts',(-46.5394956075852,-12.7723242153339,
-29.4565786810166));
#18449=CARTESIAN_POINT('Ctrl Pts',(-46.5160864719647,-12.7459862668529,
-29.4443089293986));
#18450=CARTESIAN_POINT('Ctrl Pts',(-46.4917263584107,-12.7196622748126,
-29.433565514209));
#18451=CARTESIAN_POINT('Ctrl Pts',(-46.4666223821401,-12.6935087390694,
-29.4243162909518));
#18452=CARTESIAN_POINT('Ctrl Pts',(-46.4593842022175,-12.6859679417358,
-29.4216494806681));
#18453=CARTESIAN_POINT('Ctrl Pts',(-46.4520842494196,-12.6784415052693,
-29.4191071382984));
#18454=CARTESIAN_POINT('Ctrl Pts',(-46.4447277393149,-12.6709337131846,
-29.4166890942607));
#18455=CARTESIAN_POINT('',(-39.9859592520698,-6.10843371318466,-27.2946201763046));
#18456=CARTESIAN_POINT('Origin',(-197.331032377167,-177.510314406253,-79.3434317434775));
#18457=CARTESIAN_POINT('',(-48.261606955145,-6.10843371318471,-4.13831849444347));
#18458=CARTESIAN_POINT('Origin',(0.0835265683620477,-6.10843371318469,0.0824317919394229));
#18459=CARTESIAN_POINT('',(-48.2284487824326,-14.6753754514266,-30.3462212704581));
#18460=CARTESIAN_POINT('Ctrl Pts',(-48.2616069550931,-6.10843371318472,
-4.13831849503754));
#18461=CARTESIAN_POINT('Ctrl Pts',(-48.2597772986175,-6.50994980321316,
-8.77579754148006));
#18462=CARTESIAN_POINT('Ctrl Pts',(-48.2550176567395,-7.55645913600449,
-13.2581019939041));
#18463=CARTESIAN_POINT('Ctrl Pts',(-48.2459144235836,-9.80534906153842,
-19.8181734642193));
#18464=CARTESIAN_POINT('Ctrl Pts',(-48.2425547211608,-10.6692546575742,
-21.9792831240841));
#18465=CARTESIAN_POINT('Ctrl Pts',(-48.2356129829617,-12.5596572871779,
-26.217495153478));
#18466=CARTESIAN_POINT('Ctrl Pts',(-48.2320290688777,-13.58630787804,-28.2970230681186));
#18467=CARTESIAN_POINT('Ctrl Pts',(-48.2284487824325,-14.6753754514262,
-30.3462212704574));
#18468=CARTESIAN_POINT('',(-47.1694990908375,-14.6753754514262,-31.9659918126394));
#18469=CARTESIAN_POINT('Origin',(0.0835265683620477,-14.6753754514262,0.0824317919394229));
#18470=CARTESIAN_POINT('Origin',(1241.62995219148,-1402.95413115888,321.769152191711));
#18471=CARTESIAN_POINT('Origin',(0.0835265683620477,-11.0169045823054,0.0824317919394229));
#18472=CARTESIAN_POINT('',(15.3925785990456,-11.0169045823054,23.5078932009404));
#18473=CARTESIAN_POINT('',(7.67510093260532,-11.0169045823054,20.9630507178886));
#18474=CARTESIAN_POINT('',(-5.38208978662056,-11.0169045823054,16.6574349341085));
#18475=CARTESIAN_POINT('',(14.5949188243533,-11.0169045823054,25.9268725828089));
#18476=CARTESIAN_POINT('',(9.92432302202933,-11.0169045823054,19.2683675629017));
#18477=CARTESIAN_POINT('Origin',(10.2095634989472,-11.0169045823054,19.8244816432194));
#18478=CARTESIAN_POINT('',(20.56141397709,-11.0169045823054,6.83502636924522));
#18479=CARTESIAN_POINT('Origin',(0.0835265683620477,-11.0169045823054,0.0824317919394229));
#18480=CARTESIAN_POINT('',(34.0350086811056,-11.0169045823054,-34.02493526194));
#18481=CARTESIAN_POINT('',(34.0952935222086,-11.0169045823054,-34.2077547951474));
#18482=CARTESIAN_POINT('',(29.6625358445444,-11.0169045823054,-37.8793626234925));
#18483=CARTESIAN_POINT('Origin',(0.0835265683620477,-11.0169045823054,0.0824317919394229));
#18484=CARTESIAN_POINT('',(20.4191383735183,-11.0169045823054,-9.84787775959334));
#18485=CARTESIAN_POINT('',(15.4714058027788,-11.0169045823054,5.15659338881741));
#18486=CARTESIAN_POINT('',(19.2694623393243,-11.0169045823054,-9.75836466172779));
#18487=CARTESIAN_POINT('Origin',(19.8255764196421,-11.0169045823054,-10.0436051386457));
#18488=CARTESIAN_POINT('',(6.83612114566777,-11.0169045823054,-20.3954556167886));
#18489=CARTESIAN_POINT('Origin',(0.0835265683620477,-11.0169045823054,0.0824317919394229));
#18490=CARTESIAN_POINT('',(-34.0238404855175,-11.0169045823054,-33.869050320804));
#18491=CARTESIAN_POINT('',(-34.2066600187249,-11.0169045823054,-33.9293351619071));
#18492=CARTESIAN_POINT('',(-37.87826784707,-11.0169045823054,-29.4965774842428));
#18493=CARTESIAN_POINT('Origin',(0.0835265683620477,-11.0169045823054,0.0824317919394229));
#18494=CARTESIAN_POINT('',(-9.84678298317079,-11.0169045823054,-20.2531800132168));
#18495=CARTESIAN_POINT('',(5.15768816523998,-11.0169045823054,-15.3054474424773));
#18496=CARTESIAN_POINT('',(-9.75726988530523,-11.0169045823054,-19.1035039790228));
#18497=CARTESIAN_POINT('Origin',(-10.0425103622231,-11.0169045823054,-19.6596180593406));
#18498=CARTESIAN_POINT('',(-20.394360840366,-11.0169045823054,-6.6701627853663));
#18499=CARTESIAN_POINT('Origin',(0.0835265683620477,-11.0169045823054,0.0824317919394229));
#18500=CARTESIAN_POINT('',(-33.8679555443817,-11.0169045823054,34.1897988458186));
#18501=CARTESIAN_POINT('',(-33.9282403854848,-11.0169045823054,34.372618379026));
#18502=CARTESIAN_POINT('',(-29.4954827078206,-11.0169045823054,38.0442262073711));
#18503=CARTESIAN_POINT('Origin',(0.0835265683620477,-11.0169045823054,0.0824317919394229));
#18504=CARTESIAN_POINT('',(-15.3043526660546,-11.0169045823054,-4.99172980493867));
#18505=CARTESIAN_POINT('',(-6.66906800894368,-11.0169045823054,20.5603192006674));
#18506=CARTESIAN_POINT('Origin',(0.0835265683620477,-11.0169045823054,0.0824317919394229));
#18507=CARTESIAN_POINT('',(34.1908936222416,-11.0169045823054,34.0339139046828));
#18508=CARTESIAN_POINT('',(34.373713155449,-11.0169045823054,34.0941987457859));
#18509=CARTESIAN_POINT('',(38.0453209837941,-11.0169045823054,29.6614410681217));
#18510=CARTESIAN_POINT('Origin',(0.0835265683620477,-11.0169045823054,0.0824317919394229));
#18511=CARTESIAN_POINT('',(18.7518431265311,-11.0169045823054,23.2994061884498));
#18512=CARTESIAN_POINT('',(-4.99063502851588,-11.0169045823054,15.4703110263562));
#18513=CARTESIAN_POINT('',(17.9541833518389,-11.0169045823054,25.7183855703182));
#18514=CARTESIAN_POINT('',(-6.17974956131282,-11.0169045823054,19.076414315977));
#18515=CARTESIAN_POINT('',(-6.17974956131282,-11.0169045823054,19.076414315977));
#18516=CARTESIAN_POINT('',(7.59696574233659,-11.0169045823054,18.6174859267129));
#18517=CARTESIAN_POINT('Origin',(0.0835265683620477,-11.0169045823054,0.0824317919394229));
#18518=CARTESIAN_POINT('Origin',(8.06655569071,-11.0169045823054,19.7759268101363));
#18519=CARTESIAN_POINT('Origin',(5.05982447571381,-11.0169045823054,-15.0086664655392));
#18520=CARTESIAN_POINT('',(-9.94464667269696,-14.4544045823054,-19.9563990362787));
#18521=CARTESIAN_POINT('',(-9.94464667269696,-11.3294045823054,-19.9563990362787));
#18522=CARTESIAN_POINT('',(-9.94464667269695,-11.0169045823054,-19.9563990362787));
#18523=CARTESIAN_POINT('',(5.05982447571381,-11.3294045823054,-15.0086664655392));
#18524=CARTESIAN_POINT('',(-38.8106378122313,-13.5169045823054,-29.4749754082874));
#18525=CARTESIAN_POINT('Ctrl Pts',(-38.8106378122313,-13.5169045823054,
-29.4749754082875));
#18526=CARTESIAN_POINT('Ctrl Pts',(-38.7753398292788,-13.516904574972,-29.4633358790959));
#18527=CARTESIAN_POINT('Ctrl Pts',(-38.740120224442,-13.5137764691087,-29.4517221951311));
#18528=CARTESIAN_POINT('Ctrl Pts',(-38.7054177666676,-13.5077394335821,
-29.4402790406912));
#18529=CARTESIAN_POINT('Ctrl Pts',(-38.6681956028728,-13.5012640557669,
-29.4280050118123));
#18530=CARTESIAN_POINT('Ctrl Pts',(-38.6315672874808,-13.4914421681932,
-29.4159268047662));
#18531=CARTESIAN_POINT('Ctrl Pts',(-38.5960538527439,-13.4784883891798,
-29.4042162302247));
#18532=CARTESIAN_POINT('Ctrl Pts',(-38.5599884642765,-13.4653332811001,
-29.3923236486385));
#18533=CARTESIAN_POINT('Ctrl Pts',(-38.5250713397532,-13.4489478321153,
-29.3808097077152));
#18534=CARTESIAN_POINT('Ctrl Pts',(-38.4918489021924,-13.4295031815242,
-29.3698545907503));
#18535=CARTESIAN_POINT('Ctrl Pts',(-38.4597058287231,-13.4106902683721,
-29.3592553946852));
#18536=CARTESIAN_POINT('Ctrl Pts',(-38.4291478346119,-13.3890130654893,
-29.3491788794119));
#18537=CARTESIAN_POINT('Ctrl Pts',(-38.4006911147723,-13.3645846069462,
-29.3397952604838));
#18538=CARTESIAN_POINT('Ctrl Pts',(-38.3914518672752,-13.3566532439598,
-29.3367486135694));
#18539=CARTESIAN_POINT('Ctrl Pts',(-38.3824343769285,-13.3484315569496,
-29.3337750911969));
#18540=CARTESIAN_POINT('Ctrl Pts',(-38.3736571535326,-13.3399225829037,
-29.3308807969828));
#18541=CARTESIAN_POINT('Ctrl Pts',(-38.3735625124312,-13.3398308342221,
-29.3308495890278));
#18542=CARTESIAN_POINT('Ctrl Pts',(-38.3734678995551,-13.3397390509054,
-29.3308183903802));
#18543=CARTESIAN_POINT('Ctrl Pts',(-38.3733733149185,-13.3396472329757,
-29.3307872010446));
#18544=CARTESIAN_POINT('Ctrl Pts',(-38.3385278839172,-13.3058210699866,
-29.3192969011185));
#18545=CARTESIAN_POINT('Ctrl Pts',(-38.3076591439821,-13.2674403223333,
-29.3091179172323));
#18546=CARTESIAN_POINT('Ctrl Pts',(-38.2814620639506,-13.2257618864376,
-29.3004794157585));
#18547=CARTESIAN_POINT('Ctrl Pts',(-38.267671485342,-13.2038216646339,-29.295931964917));
#18548=CARTESIAN_POINT('Ctrl Pts',(-38.2551759277532,-13.1809667714821,
-29.2918115479652));
#18549=CARTESIAN_POINT('Ctrl Pts',(-38.244080552279,-13.1573764603981,-29.2881528418319));
#18550=CARTESIAN_POINT('Ctrl Pts',(-38.2261880905563,-13.1193345988063,
-29.2822527927891));
#18551=CARTESIAN_POINT('Ctrl Pts',(-38.2119311974999,-13.0793753611319,
-29.2775515745033));
#18552=CARTESIAN_POINT('Ctrl Pts',(-38.2017729510058,-13.0382175960144,
-29.2742018871638));
#18553=CARTESIAN_POINT('Ctrl Pts',(-38.1918154952388,-12.9978733667359,
-29.2709184106765));
#18554=CARTESIAN_POINT('Ctrl Pts',(-38.1857967255739,-12.9563778844919,
-29.2689337180864));
#18555=CARTESIAN_POINT('Ctrl Pts',(-38.1841997911564,-12.9144212113995,
-29.2684071280885));
#18556=CARTESIAN_POINT('Ctrl Pts',(-38.1839146266109,-12.9069290091652,
-29.2683130949236));
#18557=CARTESIAN_POINT('Ctrl Pts',(-38.1837705844942,-12.8994221374466,
-29.2682655969568));
#18558=CARTESIAN_POINT('Ctrl Pts',(-38.1837705810014,-12.8919045823054,
-29.2682655958051));
#18559=CARTESIAN_POINT('',(-45.5252381517553,-13.5169045823054,-31.689118544074));
#18560=CARTESIAN_POINT('',(5.05982447571381,-13.5169045823054,-15.0086664655392));
#18561=CARTESIAN_POINT('',(-46.4522196376124,-14.4544045724558,-31.9947911962243));
#18562=CARTESIAN_POINT('Origin',(1220.3812882873,-1402.30169205975,385.744251110796));
#18563=CARTESIAN_POINT('',(5.05982447571381,-14.4544045823054,-15.0086664655392));
#18564=CARTESIAN_POINT('Origin',(6.93398483519394,-11.0169045823054,-20.6922365937267));
#18565=CARTESIAN_POINT('',(-33.623065834026,-12.8919045823054,-34.0659462422992));
#18566=CARTESIAN_POINT('',(-33.623065834026,-11.3294045823054,-34.0659462422992));
#18567=CARTESIAN_POINT('',(-33.623065834026,-11.0169045823054,-34.0659462422992));
#18568=CARTESIAN_POINT('',(6.93398483519395,-11.3294045823054,-20.6922365937267));
#18569=CARTESIAN_POINT('',(6.93398483519401,-11.3294045823054,-20.6922365937267));
#18570=CARTESIAN_POINT('',(6.93398483519395,-14.4544045823054,-20.6922365937267));
#18571=CARTESIAN_POINT('',(6.93398483519395,-11.0169045823054,-20.6922365937267));
#18572=CARTESIAN_POINT('',(-42.3443728514905,-14.4544045474394,-36.9418020030986));
#18573=CARTESIAN_POINT('',(-43.2465796510443,-14.4544045823054,-37.2393051888733));
#18574=CARTESIAN_POINT('',(-41.3745486405956,-13.5169045823054,-36.6220019389143));
#18575=CARTESIAN_POINT('Origin',(530.074081345601,-669.972711183026,151.813496477798));
#18576=CARTESIAN_POINT('',(-34.2908051207842,-13.5169045823054,-34.2861336374548));
#18577=CARTESIAN_POINT('',(-34.1087963291987,-13.5169045823054,-34.2261161388451));
#18578=CARTESIAN_POINT('Ctrl Pts',(-33.6230658340261,-12.8919045823054,
-34.0659462422992));
#18579=CARTESIAN_POINT('Ctrl Pts',(-33.6230658340261,-12.9240089539717,
-34.0659462422992));
#18580=CARTESIAN_POINT('Ctrl Pts',(-33.6256783091265,-12.9558011838052,
-34.066807707393));
#18581=CARTESIAN_POINT('Ctrl Pts',(-33.630814373568,-12.987039082263,-34.0685013274527));
#18582=CARTESIAN_POINT('Ctrl Pts',(-33.6360742275513,-13.019029877259,-34.0702357671816));
#18583=CARTESIAN_POINT('Ctrl Pts',(-33.6439806080066,-13.0504387215005,
-34.0728429004626));
#18584=CARTESIAN_POINT('Ctrl Pts',(-33.6543863713838,-13.0810143824775,
-34.0762742066298));
#18585=CARTESIAN_POINT('Ctrl Pts',(-33.6616724148322,-13.1024232485325,
-34.0786767834434));
#18586=CARTESIAN_POINT('Ctrl Pts',(-33.6701827293343,-13.1234238076968,
-34.0814830643069));
#18587=CARTESIAN_POINT('Ctrl Pts',(-33.6798531673154,-13.1439346499851,
-34.0846718965225));
#18588=CARTESIAN_POINT('Ctrl Pts',(-33.6798967429698,-13.1440270732421,
-34.0846862656184));
#18589=CARTESIAN_POINT('Ctrl Pts',(-33.6799403391956,-13.1441194808469,
-34.0847006414977));
#18590=CARTESIAN_POINT('Ctrl Pts',(-33.6799839559855,-13.1442118727969,
-34.084715024158));
#18591=CARTESIAN_POINT('Ctrl Pts',(-33.7146023119914,-13.2175427490685,
-34.0961304459929));
#18592=CARTESIAN_POINT('Ctrl Pts',(-33.7623907865948,-13.2814833076131,
-34.1118887216388));
#18593=CARTESIAN_POINT('Ctrl Pts',(-33.8207273804618,-13.3355724234755,
-34.1311252453856));
#18594=CARTESIAN_POINT('Ctrl Pts',(-33.8247694769424,-13.3393202155624,
-34.1324581289117));
#18595=CARTESIAN_POINT('Ctrl Pts',(-33.8288622293082,-13.3430206975035,
-34.1338077162437));
#18596=CARTESIAN_POINT('Ctrl Pts',(-33.8330047712751,-13.3466737099125,
-34.135173721724));
#18597=CARTESIAN_POINT('Ctrl Pts',(-33.8330549933399,-13.3467179971708,
-34.1351902824773));
#18598=CARTESIAN_POINT('Ctrl Pts',(-33.8331052202197,-13.3467622754629,
-34.1352068448184));
#18599=CARTESIAN_POINT('Ctrl Pts',(-33.833155451914,-13.3468065447896,-34.1352234087471));
#18600=CARTESIAN_POINT('Ctrl Pts',(-33.8971289942698,-13.4031865990188,
-34.156318719343));
#18601=CARTESIAN_POINT('Ctrl Pts',(-33.9688832036395,-13.4450083105498,
-34.179979709142));
#18602=CARTESIAN_POINT('Ctrl Pts',(-34.0475696763434,-13.4738659092279,
-34.2059266165677));
#18603=CARTESIAN_POINT('Ctrl Pts',(-34.1262997844951,-13.5027395108376,
-34.2318879128062));
#18604=CARTESIAN_POINT('Ctrl Pts',(-34.2074475252744,-13.5169045582356,
-34.2586464247271));
#18605=CARTESIAN_POINT('Ctrl Pts',(-34.2908051207842,-13.5169045823054,
-34.2861336374548));
#18606=CARTESIAN_POINT('Origin',(0.0835265683620477,-6.01690458230549,0.0824317919394229));
#18607=CARTESIAN_POINT('',(-4.13722357323051,-6.1084342262812,-48.2627019018071));
#18608=CARTESIAN_POINT('',(-32.0390884399918,-6.10843371299758,-36.2934430895344));
#18609=CARTESIAN_POINT('Origin',(0.0835265683620477,-6.10843371318469,0.0824317919394229));
#18610=CARTESIAN_POINT('',(-39.1269295149477,-12.6709337131846,-38.6166213711206));
#18611=CARTESIAN_POINT('Ctrl Pts',(-32.0390884396323,-6.10843371318765,
-36.2934430901055));
#18612=CARTESIAN_POINT('Ctrl Pts',(-32.5225298437675,-6.54712953976947,
-36.4517920085165));
#18613=CARTESIAN_POINT('Ctrl Pts',(-33.0050570127847,-6.98698298247917,
-36.609758923213));
#18614=CARTESIAN_POINT('Ctrl Pts',(-33.4866867369723,-7.42790908709951,
-36.7674553177767));
#18615=CARTESIAN_POINT('Ctrl Pts',(-33.9664335523027,-7.86711141175758,
-36.924535205669));
#18616=CARTESIAN_POINT('Ctrl Pts',(-34.4452900133375,-8.30737802767764,
-37.0813467433358));
#18617=CARTESIAN_POINT('Ctrl Pts',(-34.9232986528203,-8.74862497312586,
-37.2379554426264));
#18618=CARTESIAN_POINT('Ctrl Pts',(-35.4003758146033,-9.18901207702346,
-37.3942589643555));
#18619=CARTESIAN_POINT('Ctrl Pts',(-35.8766085225511,-9.63037569350826,
-37.5503604966855));
#18620=CARTESIAN_POINT('Ctrl Pts',(-36.3520638137852,-10.0726323507299,
-37.7062796845329));
#18621=CARTESIAN_POINT('Ctrl Pts',(-36.826174045008,-10.5136378666659,-37.8617577779841));
#18622=CARTESIAN_POINT('Ctrl Pts',(-37.2995113121353,-10.9555313776728,
-38.0170545978434));
#18623=CARTESIAN_POINT('Ctrl Pts',(-37.7721657694013,-11.3982301183219,
-38.1721436168242));
#18624=CARTESIAN_POINT('Ctrl Pts',(-38.2243455601687,-11.8217518281934,
-38.3205144172578));
#18625=CARTESIAN_POINT('Ctrl Pts',(-38.675900600911,-12.2460105160849,-38.4686947735073));
#18626=CARTESIAN_POINT('Ctrl Pts',(-39.1269295149477,-12.6709337131846,
-38.6166213711206));
#18627=CARTESIAN_POINT('',(-40.2726585348436,-13.2959337131846,-38.3325384971017));
#18628=CARTESIAN_POINT('Ctrl Pts',(-40.2726585348435,-13.2959337131846,
-38.3325384971018));
#18629=CARTESIAN_POINT('Ctrl Pts',(-40.2396336815792,-13.2959336603245,
-38.3672321109749));
#18630=CARTESIAN_POINT('Ctrl Pts',(-40.203931177053,-13.2916605128733,-38.3984485109642));
#18631=CARTESIAN_POINT('Ctrl Pts',(-40.1665336587125,-13.2840750781675,
-38.4265635639867));
#18632=CARTESIAN_POINT('Ctrl Pts',(-40.1233293436535,-13.2753118359676,
-38.4590441044767));
#18633=CARTESIAN_POINT('Ctrl Pts',(-40.0778617899977,-13.262127307608,-38.487385683028));
#18634=CARTESIAN_POINT('Ctrl Pts',(-40.0316115052285,-13.2459526170016,
-38.512130144461));
#18635=CARTESIAN_POINT('Ctrl Pts',(-40.0180845510295,-13.2412219585828,
-38.5193672284736));
#18636=CARTESIAN_POINT('Ctrl Pts',(-40.0044905078433,-13.2362352705449,
-38.5262963859028));
#18637=CARTESIAN_POINT('Ctrl Pts',(-39.9908662064094,-13.2310278528739,
-38.5329306481798));
#18638=CARTESIAN_POINT('Ctrl Pts',(-39.9908210967496,-13.2310106112677,
-38.5329526140264));
#18639=CARTESIAN_POINT('Ctrl Pts',(-39.9907759867598,-13.230993367242,-38.5329745766387));
#18640=CARTESIAN_POINT('Ctrl Pts',(-39.9907308764414,-13.2309761207982,
-38.5329965360173));
#18641=CARTESIAN_POINT('Ctrl Pts',(-39.9008654396959,-13.1966190321654,
-38.5767423843686));
#18642=CARTESIAN_POINT('Ctrl Pts',(-39.8096589826388,-13.1525556483329,
-38.6075525746423));
#18643=CARTESIAN_POINT('Ctrl Pts',(-39.7201449624174,-13.1028429779769,
-38.6282896284184));
#18644=CARTESIAN_POINT('Ctrl Pts',(-39.7095659381455,-13.0969677916652,
-38.6307403930549));
#18645=CARTESIAN_POINT('Ctrl Pts',(-39.6990105689488,-13.091013739855,-38.6330505050437));
#18646=CARTESIAN_POINT('Ctrl Pts',(-39.6884838737899,-13.0849875486837,
-38.6352247206687));
#18647=CARTESIAN_POINT('Ctrl Pts',(-39.6883620970893,-13.0849178354768,
-38.6352498727987));
#18648=CARTESIAN_POINT('Ctrl Pts',(-39.6882403231401,-13.0848481114876,
-38.6352750062405));
#18649=CARTESIAN_POINT('Ctrl Pts',(-39.6881185519542,-13.0847783767298,
-38.6353001210018));
#18650=CARTESIAN_POINT('Ctrl Pts',(-39.6633307896687,-13.0705831581647,
-38.6404124858695));
#18651=CARTESIAN_POINT('Ctrl Pts',(-39.6385397905417,-13.0558793142743,
-38.6447819668785));
#18652=CARTESIAN_POINT('Ctrl Pts',(-39.6138315388079,-13.0407301262923,
-38.6484136767956));
#18653=CARTESIAN_POINT('Ctrl Pts',(-39.576587090328,-13.0178947125452,-38.6538880031203));
#18654=CARTESIAN_POINT('Ctrl Pts',(-39.5395279799376,-12.9940463246918,
-38.6576871593004));
#18655=CARTESIAN_POINT('Ctrl Pts',(-39.5029368702493,-12.9693962501975,
-38.6598334969272));
#18656=CARTESIAN_POINT('Ctrl Pts',(-39.4663457605609,-12.9447461757032,
-38.6619798345541));
#18657=CARTESIAN_POINT('Ctrl Pts',(-39.4302226608903,-12.9192944015675,
-38.662473362689));
#18658=CARTESIAN_POINT('Ctrl Pts',(-39.3948503116026,-12.8932521061511,
-38.6613365091335));
#18659=CARTESIAN_POINT('Ctrl Pts',(-39.3647901092163,-12.8711207892725,
-38.6603703859144));
#18660=CARTESIAN_POINT('Ctrl Pts',(-39.3352090913624,-12.8485482515871,
-38.6582701011378));
#18661=CARTESIAN_POINT('Ctrl Pts',(-39.3061311012479,-12.8255048446002,
-38.6549739360498));
#18662=CARTESIAN_POINT('Ctrl Pts',(-39.2895870067339,-12.8123941618599,
-38.6530985634214));
#18663=CARTESIAN_POINT('Ctrl Pts',(-39.2732062544516,-12.7991308725972,
-38.6508352926566));
#18664=CARTESIAN_POINT('Ctrl Pts',(-39.2569980022231,-12.7857088195892,
-38.6481669486584));
#18665=CARTESIAN_POINT('Ctrl Pts',(-39.2280783717813,-12.7617604748022,
-38.6434059465941));
#18666=CARTESIAN_POINT('Ctrl Pts',(-39.1997054209728,-12.7373067239667,
-38.637357958912));
#18667=CARTESIAN_POINT('Ctrl Pts',(-39.1719053122653,-12.7123167139494,
-38.6299576805737));
#18668=CARTESIAN_POINT('Ctrl Pts',(-39.1567397038309,-12.6986840799665,
-38.6259206559431));
#18669=CARTESIAN_POINT('Ctrl Pts',(-39.1417450242042,-12.684891691096,-38.62148049444));
#18670=CARTESIAN_POINT('Ctrl Pts',(-39.1269295149477,-12.6709337131846,
-38.6166213711206));
#18671=CARTESIAN_POINT('',(-41.4413720390587,-13.2959337131846,-37.0661134559641));
#18672=CARTESIAN_POINT('Origin',(0.0835265683620477,-13.2959337131846,0.0824317919394229));
#18673=CARTESIAN_POINT('',(-42.868890621412,-14.6753754514262,-37.5345822714215));
#18674=CARTESIAN_POINT('Origin',(537.351619142406,-671.736419815441,133.622883040623));
#18675=CARTESIAN_POINT('',(-30.3451265715159,-14.675375306047,-48.2295436818698));
#18676=CARTESIAN_POINT('Origin',(0.0835265683620477,-14.6753754514262,0.0824317919394229));
#18677=CARTESIAN_POINT('Ctrl Pts',(-30.3451268039573,-14.6753748699083,
-48.2295440509134));
#18678=CARTESIAN_POINT('Ctrl Pts',(-29.4817793367662,-14.2165313285487,
-48.2310581461111));
#18679=CARTESIAN_POINT('Ctrl Pts',(-28.6133029132634,-13.7688961381484,
-48.2325674328801));
#18680=CARTESIAN_POINT('Ctrl Pts',(-27.7390368044124,-13.3339028932971,
-48.2340665432468));
#18681=CARTESIAN_POINT('Ctrl Pts',(-26.8896562709457,-12.9112915274605,
-48.2355229821389));
#18682=CARTESIAN_POINT('Ctrl Pts',(-26.0348108991148,-12.5006127526482,
-48.2369698132499));
#18683=CARTESIAN_POINT('Ctrl Pts',(-25.1739206375199,-12.103139198304,-48.2384019171115));
#18684=CARTESIAN_POINT('Ctrl Pts',(-24.8546574836089,-11.9557352070903,
-48.2389330161563));
#18685=CARTESIAN_POINT('Ctrl Pts',(-24.5345632331656,-11.8101469176186,
-48.239462087945));
#18686=CARTESIAN_POINT('Ctrl Pts',(-24.2136092696096,-11.6664376689277,
-48.2399888653929));
#18687=CARTESIAN_POINT('Ctrl Pts',(-24.1814220403843,-11.6520256252871,
-48.2400416938617));
#18688=CARTESIAN_POINT('Ctrl Pts',(-24.1492261126984,-11.6376325718391,
-48.240094498393));
#18689=CARTESIAN_POINT('Ctrl Pts',(-24.1170214462916,-11.6232585917442,
-48.240147278535));
#18690=CARTESIAN_POINT('Ctrl Pts',(-23.3441962477099,-11.2783218089513,
-48.2414138596948));
#18691=CARTESIAN_POINT('Ctrl Pts',(-22.566326590449,-10.9443666876212,-48.242664919568));
#18692=CARTESIAN_POINT('Ctrl Pts',(-21.7829239437866,-10.6225428072345,
-48.2438912877425));
#18693=CARTESIAN_POINT('Ctrl Pts',(-21.51280683996,-10.511577986165,-48.2443141392875));
#18694=CARTESIAN_POINT('Ctrl Pts',(-21.2420321676512,-10.4020550272744,
-48.2447340583014));
#18695=CARTESIAN_POINT('Ctrl Pts',(-20.9705806532939,-10.2940198074422,
-48.2451506784524));
#18696=CARTESIAN_POINT('Ctrl Pts',(-20.9543075471883,-10.2875432600572,
-48.2451756541979));
#18697=CARTESIAN_POINT('Ctrl Pts',(-20.9380317506347,-10.2810720136179,
-48.2452006183239));
#18698=CARTESIAN_POINT('Ctrl Pts',(-20.9217533048638,-10.274606093873,-48.2452255706762));
#18699=CARTESIAN_POINT('Ctrl Pts',(-20.4658680493351,-10.0935250793455,
-48.2459243726188));
#18700=CARTESIAN_POINT('Ctrl Pts',(-20.0079420683559,-9.91663263844885,
-48.2466145458997));
#18701=CARTESIAN_POINT('Ctrl Pts',(-19.5482069672317,-9.74425107317444,
-48.2472938116465));
#18702=CARTESIAN_POINT('Ctrl Pts',(-19.1078591483264,-9.57913893337382,
-48.2479444323828));
#18703=CARTESIAN_POINT('Ctrl Pts',(-18.6658501180235,-9.41816464536872,
-48.2485850503878));
#18704=CARTESIAN_POINT('Ctrl Pts',(-18.2223680178153,-9.26165511807674,
-48.2492135577687));
#18705=CARTESIAN_POINT('Ctrl Pts',(-18.0367076056395,-9.19613359345863,
-48.249476677609));
#18706=CARTESIAN_POINT('Ctrl Pts',(-17.8507889517602,-9.1313951604908,-48.2497376732635));
#18707=CARTESIAN_POINT('Ctrl Pts',(-17.6646259020658,-9.06746659619127,
-48.2499963816089));
#18708=CARTESIAN_POINT('Ctrl Pts',(-17.6610247716672,-9.0662299646652,-48.2500013860525));
#18709=CARTESIAN_POINT('Ctrl Pts',(-17.6574235801825,-9.06499364665118,
-48.2500063895844));
#18710=CARTESIAN_POINT('Ctrl Pts',(-17.6538223280036,-9.06375764243259,
-48.2500113922032));
#18711=CARTESIAN_POINT('Ctrl Pts',(-16.7856068602355,-8.76577296168996,
-48.2512174590869));
#18712=CARTESIAN_POINT('Ctrl Pts',(-15.912148956512,-8.48534970224392,-48.2523723989392));
#18713=CARTESIAN_POINT('Ctrl Pts',(-15.0330164282587,-8.22405492508236,
-48.2534642885946));
#18714=CARTESIAN_POINT('Ctrl Pts',(-14.806881310249,-8.15684330070286,-48.253745150226));
#18715=CARTESIAN_POINT('Ctrl Pts',(-14.5803706794578,-8.09089757133394,
-48.2540218379708));
#18716=CARTESIAN_POINT('Ctrl Pts',(-14.3534770702195,-8.02624496071179,
-48.2542941443476));
#18717=CARTESIAN_POINT('Ctrl Pts',(-13.8350297076525,-7.87851503754358,
-48.2549163589764));
#18718=CARTESIAN_POINT('Ctrl Pts',(-13.3142751741925,-7.73745329658206,
-48.2555159228595));
#18719=CARTESIAN_POINT('Ctrl Pts',(-12.791639486122,-7.60353311379642,-48.2560895730586));
#18720=CARTESIAN_POINT('Ctrl Pts',(-12.289610378971,-7.47489316186051,-48.2566406052667));
#18721=CARTESIAN_POINT('Ctrl Pts',(-11.7858455328013,-7.35284273127803,
-48.2571677252085));
#18722=CARTESIAN_POINT('Ctrl Pts',(-11.2807318563516,-7.2377561198086,-48.2576681937696));
#18723=CARTESIAN_POINT('Ctrl Pts',(-11.1005031779102,-7.19669227842297,
-48.257846765033));
#18724=CARTESIAN_POINT('Ctrl Pts',(-10.9201009710423,-7.15651419448117,
-48.2580219465406));
#18725=CARTESIAN_POINT('Ctrl Pts',(-10.7395560300484,-7.1172401230684,-48.2581936074901));
#18726=CARTESIAN_POINT('Ctrl Pts',(-9.65047242716134,-6.88033098034299,
-48.2592291010593));
#18727=CARTESIAN_POINT('Ctrl Pts',(-8.5559911237925,-6.67627260249923,-48.2601366679466));
#18728=CARTESIAN_POINT('Ctrl Pts',(-7.45572847150844,-6.50737682460517,
-48.2608950409414));
#18729=CARTESIAN_POINT('Ctrl Pts',(-6.35546581922438,-6.33848104671112,
-48.2616534139363));
#18730=CARTESIAN_POINT('Ctrl Pts',(-5.24942178111159,-6.20474805617039,
-48.2622625913705));
#18731=CARTESIAN_POINT('Ctrl Pts',(-4.13722359825051,-6.10843510301128,
-48.262701707337));
#18732=CARTESIAN_POINT('Origin',(0.0835265683620477,-8.56135981233827,0.0824317919394229));
#18733=CARTESIAN_POINT('',(-39.2593077130565,-8.46983068145907,37.6646495687126));
#18734=CARTESIAN_POINT('',(-35.984538282875,-3.84038894321748,34.3905421902094));
#18735=CARTESIAN_POINT('Ctrl Pts',(-39.2593077130565,-8.46983068145907,
37.6646495687126));
#18736=CARTESIAN_POINT('Ctrl Pts',(-39.1551178801364,-8.32253590125116,
37.5604790152082));
#18737=CARTESIAN_POINT('Ctrl Pts',(-39.0509278602785,-8.17524127521395,
37.4563084306819));
#18738=CARTESIAN_POINT('Ctrl Pts',(-38.5299768032981,-7.43876893481715,
36.9354553491631));
#18739=CARTESIAN_POINT('Ctrl Pts',(-38.1132128963777,-6.84959358714927,
36.5187723760457));
#18740=CARTESIAN_POINT('Ctrl Pts',(-37.1258164844502,-5.45373818194081,
35.5315743934649));
#18741=CARTESIAN_POINT('Ctrl Pts',(-36.5551810303102,-4.64706055617428,
34.961058895205));
#18742=CARTESIAN_POINT('Ctrl Pts',(-35.984538282875,-3.84038894321748,34.3905421902094));
#18743=CARTESIAN_POINT('',(-35.9845382828747,-3.84038894321748,-34.2256786063309));
#18744=CARTESIAN_POINT('Origin',(0.0835265683620477,-3.84038894321747,0.0824317919394229));
#18745=CARTESIAN_POINT('',(-39.2593077130561,-8.46983068145907,-37.4997859848342));
#18746=CARTESIAN_POINT('Ctrl Pts',(-35.9845382828747,-3.84038894321748,
-34.2256786063309));
#18747=CARTESIAN_POINT('Ctrl Pts',(-36.0887325923582,-3.98768003220409,
-34.3298499015818));
#18748=CARTESIAN_POINT('Ctrl Pts',(-36.1929266581883,-4.13497132206384,
-34.4340211565197));
#18749=CARTESIAN_POINT('Ctrl Pts',(-36.7138958007323,-4.87142874967365,
-34.9548772348263));
#18750=CARTESIAN_POINT('Ctrl Pts',(-37.1306673216522,-5.46059781902367,
-35.3715614696892));
#18751=CARTESIAN_POINT('Ctrl Pts',(-38.1180656564427,-6.85645163869055,
-36.358759770908));
#18752=CARTESIAN_POINT('Ctrl Pts',(-38.688689482493,-7.66313885272879,-36.9292733421747));
#18753=CARTESIAN_POINT('Ctrl Pts',(-39.2593077130561,-8.46983068145907,
-37.4997859848342));
#18754=CARTESIAN_POINT('',(-49.8065937787556,-8.46983068145906,-21.6260364650814));
#18755=CARTESIAN_POINT('Origin',(0.0835265683620477,-8.46983068145906,0.0824317919394229));
#18756=CARTESIAN_POINT('',(-49.8065937787556,-8.46983068145906,21.7909000489602));
#18757=CARTESIAN_POINT('Ctrl Pts',(-49.8065937787556,-8.46983068145906,
-21.6260364650814));
#18758=CARTESIAN_POINT('Ctrl Pts',(-49.8091724689568,-7.78020213595473,
-19.8916770737466));
#18759=CARTESIAN_POINT('Ctrl Pts',(-49.8116222102493,-7.15174092367616,
-18.13538723326));
#18760=CARTESIAN_POINT('Ctrl Pts',(-49.8160494956856,-6.04804272442583,
-14.5965921523776));
#18761=CARTESIAN_POINT('Ctrl Pts',(-49.8180308842616,-5.57158091815884,
-12.8110043255947));
#18762=CARTESIAN_POINT('Ctrl Pts',(-49.8213344689701,-4.79205582539579,
-9.20258923968633));
#18763=CARTESIAN_POINT('Ctrl Pts',(-49.8226553391186,-4.48906686350367,
-7.3797460175301));
#18764=CARTESIAN_POINT('Ctrl Pts',(-49.8240081829567,-4.18101117599353,
-4.61403398685641));
#18765=CARTESIAN_POINT('Ctrl Pts',(-49.8243546591215,-4.10271637230149,
-3.68689182696108));
#18766=CARTESIAN_POINT('Ctrl Pts',(-49.8248218054713,-3.99733451725048,
-1.82160999461689));
#18767=CARTESIAN_POINT('Ctrl Pts',(-49.8249413755347,-3.97048844752839,
-0.88414976855677));
#18768=CARTESIAN_POINT('Ctrl Pts',(-49.8249557340184,-3.96725979794587,
3.77506613399273));
#18769=CARTESIAN_POINT('Ctrl Pts',(-49.8230647514948,-4.38426661992436,
7.45640245004576));
#18770=CARTESIAN_POINT('Ctrl Pts',(-49.818921517886,-5.36130666529405,12.0080656973011));
#18771=CARTESIAN_POINT('Ctrl Pts',(-49.8180052418649,-5.57963087290763,
12.9171167524008));
#18772=CARTESIAN_POINT('Ctrl Pts',(-49.8160296339025,-6.05753886911523,
14.7247229136368));
#18773=CARTESIAN_POINT('Ctrl Pts',(-49.8149721493814,-6.31667893722832,
15.6219036997713));
#18774=CARTESIAN_POINT('Ctrl Pts',(-49.8116301976253,-7.14963222024195,
18.2952277610572));
#18775=CARTESIAN_POINT('Ctrl Pts',(-49.8091774529085,-7.77886925953041,
20.0531885824263));
#18776=CARTESIAN_POINT('Ctrl Pts',(-49.8065937787556,-8.46983068145906,
21.7909000489602));
#18777=CARTESIAN_POINT('Origin',(0.0835265683620477,-8.46983068145906,0.0824317919394229));
#18778=CARTESIAN_POINT('Origin',(0.0835265683620477,11.4830954176946,0.0824317919394229));
#18779=CARTESIAN_POINT('',(-35.918219620459,-3.61941807409668,34.3274595712494));
#18780=CARTESIAN_POINT('',(-35.918219620459,11.9341984494201,34.3274595712494));
#18781=CARTESIAN_POINT('',(-35.918219620459,11.4830954176946,34.3274595712494));
#18782=CARTESIAN_POINT('',(-35.9182196204586,11.9341984494201,-34.1625959873709));
#18783=CARTESIAN_POINT('Origin',(0.0835265683620477,11.9341984494201,0.0824317919394229));
#18784=CARTESIAN_POINT('',(-35.9182196204586,-3.61941807409668,-34.1625959873709));
#18785=CARTESIAN_POINT('',(-35.9182196204586,11.4830954176946,-34.1625959873709));
#18786=CARTESIAN_POINT('Origin',(0.0835265683620477,-3.61941807409668,0.0824317919394229));
#18787=CARTESIAN_POINT('Origin',(0.0835265683620477,11.4830954176946,0.0824317919394229));
#18788=CARTESIAN_POINT('Origin',(0.0835265683620477,11.9341984494201,0.0824317919394229));
#18789=CARTESIAN_POINT('Origin',(0.0835265683620477,-3.61941807409668,0.0824317919394229));
#18790=CARTESIAN_POINT('Origin',(0.0835265683620477,12.0636401876617,0.0824317919394229));
#18791=CARTESIAN_POINT('',(-36.6066544046101,13.0346110567823,-34.8476596904499));
#18792=CARTESIAN_POINT('',(-35.9845382828753,12.1551693185412,-34.2256786063306));
#18793=CARTESIAN_POINT('',(-36.6066544046107,13.0346110567825,-34.8476596904497));
#18794=CARTESIAN_POINT('',(-35.9845382828754,12.1551693185417,34.3905421902101));
#18795=CARTESIAN_POINT('Origin',(0.0835265683620477,12.1551693185409,0.0824317919394229));
#18796=CARTESIAN_POINT('',(-36.6066544046109,13.0346110567825,35.0125232743281));
#18797=CARTESIAN_POINT('',(-35.984538282875,12.1551693185409,34.3905421902094));
#18798=CARTESIAN_POINT('',(-49.8216584885785,13.0346110567825,8.78606179499423));
#18799=CARTESIAN_POINT('Origin',(0.0835265683620477,13.0346110567825,0.0824317919394229));
#18800=CARTESIAN_POINT('',(-49.8216584885785,13.0346110567825,-8.6211982111154));
#18801=CARTESIAN_POINT('Ctrl Pts',(-49.8216584885785,13.0346110567825,8.78606179499423));
#18802=CARTESIAN_POINT('Ctrl Pts',(-49.8223976721169,12.8633426645386,7.78497558757201));
#18803=CARTESIAN_POINT('Ctrl Pts',(-49.8230202078243,12.7204977856027,6.78145983735361));
#18804=CARTESIAN_POINT('Ctrl Pts',(-49.8235176993747,12.607033826209,5.77542487233127));
#18805=CARTESIAN_POINT('Ctrl Pts',(-49.8240131775891,12.4940290526656,4.77346130604461));
#18806=CARTESIAN_POINT('Ctrl Pts',(-49.8243846217383,12.4101678841265,3.76899887262193));
#18807=CARTESIAN_POINT('Ctrl Pts',(-49.8246240837851,12.3563452055187,2.76195712956022));
#18808=CARTESIAN_POINT('Ctrl Pts',(-49.8248351469452,12.308905601697,1.87434501959917));
#18809=CARTESIAN_POINT('Ctrl Pts',(-49.8249436813649,12.2848014527005,0.984729221390203));
#18810=CARTESIAN_POINT('Ctrl Pts',(-49.824944469213,12.2846123568863,0.0930599517194889));
#18811=CARTESIAN_POINT('Ctrl Pts',(-49.8249444697293,12.2846122329701,0.0924756330936691));
#18812=CARTESIAN_POINT('Ctrl Pts',(-49.8249444701992,12.284612119341,0.0918913167795029));
#18813=CARTESIAN_POINT('Ctrl Pts',(-49.8249444706228,12.2846120159986,0.0913070027769935));
#18814=CARTESIAN_POINT('Ctrl Pts',(-49.8249449290864,12.284500162369,-0.541130544723481));
#18815=CARTESIAN_POINT('Ctrl Pts',(-49.8248910995487,12.2964431061466,-1.17335603026734));
#18816=CARTESIAN_POINT('Ctrl Pts',(-49.8247846280076,12.3202812996977,-1.80503154627235));
#18817=CARTESIAN_POINT('Ctrl Pts',(-49.8246764726378,12.3444964900669,-2.44669689892658));
#18818=CARTESIAN_POINT('Ctrl Pts',(-49.8245139977477,12.3809861187555,-3.08779471686519));
#18819=CARTESIAN_POINT('Ctrl Pts',(-49.8242991879303,12.4295292879082,-3.72797704193668));
#18820=CARTESIAN_POINT('Ctrl Pts',(-49.8240822089778,12.4785626427164,-4.37462388504563));
#18821=CARTESIAN_POINT('Ctrl Pts',(-49.8238118339164,12.5398940970328,-5.02033662533801));
#18822=CARTESIAN_POINT('Ctrl Pts',(-49.8234903564628,12.6132427399653,-5.66476341594209));
#18823=CARTESIAN_POINT('Ctrl Pts',(-49.8231633549434,12.6878517597083,-6.32026363000007));
#18824=CARTESIAN_POINT('Ctrl Pts',(-49.8227834807396,12.774894442269,-6.97443328341991));
#18825=CARTESIAN_POINT('Ctrl Pts',(-49.8223533878003,12.8740215067224,-7.62690954257758));
#18826=CARTESIAN_POINT('Ctrl Pts',(-49.8221346202543,12.9244426660921,-7.95879276366675));
#18827=CARTESIAN_POINT('Ctrl Pts',(-49.8219028634911,12.9779895328919,-8.29023798040707));
#18828=CARTESIAN_POINT('Ctrl Pts',(-49.8216584885785,13.0346110567825,-8.62119821111539));
#18829=CARTESIAN_POINT('Origin',(0.0835265683620477,13.0346110567825,0.0824317919394229));
#18830=CARTESIAN_POINT('Origin',(0.0835265683620477,12.0636401876617,0.0824317919394229));
#18831=CARTESIAN_POINT('',(35.0136180507514,13.0346110567824,-36.6077491810329));
#18832=CARTESIAN_POINT('',(34.3916369666323,12.155169318541,-35.9856330592975));
#18833=CARTESIAN_POINT('',(35.0136180507513,13.0346110567825,-36.6077491810332));
#18834=CARTESIAN_POINT('',(-34.224583829909,12.1551693185417,-35.9856330592976));
#18835=CARTESIAN_POINT('Origin',(0.0835265683620477,12.1551693185409,0.0824317919394229));
#18836=CARTESIAN_POINT('',(-34.8465649140271,13.0346110567825,-36.6077491810333));
#18837=CARTESIAN_POINT('',(-34.2245838299083,12.1551693185409,-35.9856330592973));
#18838=CARTESIAN_POINT('',(-8.62010343469281,13.0346110567825,-49.8227532650011));
#18839=CARTESIAN_POINT('Origin',(0.0835265683620477,13.0346110567825,0.0824317919394229));
#18840=CARTESIAN_POINT('',(8.78715657141686,13.0346110567825,-49.8227532650011));
#18841=CARTESIAN_POINT('Ctrl Pts',(-8.62010343469281,13.0346110567825,-49.8227532650012));
#18842=CARTESIAN_POINT('Ctrl Pts',(-7.75844751180745,12.8871967547116,-49.8233894957965));
#18843=CARTESIAN_POINT('Ctrl Pts',(-6.89456295486043,12.7606786215472,-49.8239416754741));
#18844=CARTESIAN_POINT('Ctrl Pts',(-6.02838145460376,12.6558408127419,-49.824401445282));
#18845=CARTESIAN_POINT('Ctrl Pts',(-5.45188904034233,12.5860653655796,-49.8247074478998));
#18846=CARTESIAN_POINT('Ctrl Pts',(-4.87437937103337,12.5258925149287,-49.8249725252371));
#18847=CARTESIAN_POINT('Ctrl Pts',(-4.29583487440298,12.4755408811181,-49.8251943106573));
#18848=CARTESIAN_POINT('Ctrl Pts',(-4.29265435629997,12.4752640756454,-49.825195529911));
#18849=CARTESIAN_POINT('Ctrl Pts',(-4.28947377822589,12.4749875690291,-49.825196747846));
#18850=CARTESIAN_POINT('Ctrl Pts',(-4.28629314051264,12.4747113612835,-49.8251979644619));
#18851=CARTESIAN_POINT('Ctrl Pts',(-3.86378044609719,12.438020203936,-49.8253595784886));
#18852=CARTESIAN_POINT('Ctrl Pts',(-3.44050667647658,12.4066244502033,-49.8254981885894));
#18853=CARTESIAN_POINT('Ctrl Pts',(-3.01673651081865,12.3805167222789,-49.8256136721586));
#18854=CARTESIAN_POINT('Ctrl Pts',(-2.58887894632784,12.3541571769655,-49.8257302696038));
#18855=CARTESIAN_POINT('Ctrl Pts',(-2.1605141706406,12.3331879704997,-49.8258232933164));
#18856=CARTESIAN_POINT('Ctrl Pts',(-1.73189789250613,12.3176520559965,-49.8258923976071));
#18857=CARTESIAN_POINT('Ctrl Pts',(-1.31087896549224,12.3023915202026,-49.8259602770036));
#18858=CARTESIAN_POINT('Ctrl Pts',(-0.889616220769264,12.2923733967901,
-49.8260050775384));
#18859=CARTESIAN_POINT('Ctrl Pts',(-0.468353474323579,12.2876877721295,
-49.826026253509));
#18860=CARTESIAN_POINT('Ctrl Pts',(-0.284460199973243,12.2856423625402,
-49.8260354974277));
#18861=CARTESIAN_POINT('Ctrl Pts',(-0.100567045923406,12.2846137392999,
-49.8260402366669));
#18862=CARTESIAN_POINT('Ctrl Pts',(0.0833047732558613,12.2846124143579,
-49.8260404123309));
#18863=CARTESIAN_POINT('Ctrl Pts',(0.0872263894601545,12.2846123860995,
-49.8260404160775));
#18864=CARTESIAN_POINT('Ctrl Pts',(0.0911479501779279,12.2846128251744,
-49.8260404177092));
#18865=CARTESIAN_POINT('Ctrl Pts',(0.0950694548097551,12.2846137316609,
-49.8260404172258));
#18866=CARTESIAN_POINT('Ctrl Pts',(1.25176284833155,12.2848811103974,-49.8260402746341));
#18867=CARTESIAN_POINT('Ctrl Pts',(2.40624585563398,12.3254286614646,-49.8258561458821));
#18868=CARTESIAN_POINT('Ctrl Pts',(3.55854196309821,12.4051717612045,-49.8255020546121));
#18869=CARTESIAN_POINT('Ctrl Pts',(3.85537063385761,12.4257133894758,-49.8254108415634));
#18870=CARTESIAN_POINT('Ctrl Pts',(4.15205421108766,12.4488556287928,-49.825308352493));
#18871=CARTESIAN_POINT('Ctrl Pts',(4.44859314096187,12.4745793828298,-49.825194832241));
#18872=CARTESIAN_POINT('Ctrl Pts',(4.99533228329415,12.5220071631409,-49.8249855310028));
#18873=CARTESIAN_POINT('Ctrl Pts',(5.54164564607858,12.578220119787,-49.8247383049551));
#18874=CARTESIAN_POINT('Ctrl Pts',(6.08714324293855,12.643043269177,-49.8244545700796));
#18875=CARTESIAN_POINT('Ctrl Pts',(6.64034176769106,12.7087815434036,-49.824166829647));
#18876=CARTESIAN_POINT('Ctrl Pts',(7.19270133263586,12.7833747882158,-49.823841543167));
#18877=CARTESIAN_POINT('Ctrl Pts',(7.74382117374416,12.8665869343007,-49.8234804167539));
#18878=CARTESIAN_POINT('Ctrl Pts',(8.09212801691555,12.9191768752799,-49.8232521854481));
#18879=CARTESIAN_POINT('Ctrl Pts',(8.43993980678189,12.9752083234332,-49.8230096434377));
#18880=CARTESIAN_POINT('Ctrl Pts',(8.78715657141686,13.0346110567825,-49.8227532650012));
#18881=CARTESIAN_POINT('Origin',(0.0835265683620477,13.0346110567825,0.0824317919394229));
#18882=CARTESIAN_POINT('Origin',(-68.3539734316379,-8.56135981233827,0.0824317919394229));
#18883=CARTESIAN_POINT('',(-22.6217205869088,-8.56135981233827,-49.6050682080606));
#18884=CARTESIAN_POINT('',(-44.2914734316379,-8.56135981233827,-49.6050682080606));
#18885=CARTESIAN_POINT('',(-68.353973431638,-8.56135981233827,-49.6050682080606));
#18886=CARTESIAN_POINT('',(-49.603973431638,-8.56135981233827,-44.2925682080605));
#18887=CARTESIAN_POINT('Origin',(-44.291473431638,-8.56135981233827,-44.2925682080606));
#18888=CARTESIAN_POINT('',(-49.6039734316379,-8.56135981233827,-22.6228153633314));
#18889=CARTESIAN_POINT('',(-49.603973431638,-8.56135981233827,0.0824317919394229));
#18890=CARTESIAN_POINT('',(-39.4190920287328,-8.56135981233827,-37.6524198521891));
#18891=CARTESIAN_POINT('Origin',(0.0835265683620477,-8.56135981233827,0.0824317919394229));
#18892=CARTESIAN_POINT('',(-40.5751133498644,-8.56135981233827,-38.8084411733207));
#18893=CARTESIAN_POINT('',(-37.6513250757665,-8.56135981233827,-39.4201868051554));
#18894=CARTESIAN_POINT('',(-37.5642074513747,-8.56135981233827,-39.3330691807637));
#18895=CARTESIAN_POINT('Origin',(0.0835265683620477,-8.56135981233827,0.0824317919394229));
#18896=CARTESIAN_POINT('Origin',(-50.666473431638,13.1261401876617,0.0824317919394229));
#18897=CARTESIAN_POINT('',(-49.603973431638,13.1261401876617,-10.8660811365418));
#18898=CARTESIAN_POINT('',(-49.603973431638,13.1261401876617,-44.2925682080605));
#18899=CARTESIAN_POINT('',(-49.603973431638,13.1261401876617,0.0824317919394229));
#18900=CARTESIAN_POINT('',(-44.2914734316379,13.1261401876617,-49.6050682080606));
#18901=CARTESIAN_POINT('Origin',(-44.291473431638,13.1261401876617,-44.2925682080606));
#18902=CARTESIAN_POINT('',(-10.8649863601192,13.1261401876617,-49.6050682080606));
#18903=CARTESIAN_POINT('',(-50.666473431638,13.1261401876617,-49.6050682080606));
#18904=CARTESIAN_POINT('',(-34.9989290209752,13.1261401876617,-36.7677907503642));
#18905=CARTESIAN_POINT('Origin',(0.0835265683620477,13.1261401876617,0.0824317919394229));
#18906=CARTESIAN_POINT('',(-38.8073463968981,13.1261401876617,-40.576208126287));
#18907=CARTESIAN_POINT('',(-38.8073463968981,13.1261401876617,-40.576208126287));
#18908=CARTESIAN_POINT('',(-40.5751133498644,13.1261401876617,-38.8084411733207));
#18909=CARTESIAN_POINT('Origin',(-39.6912298733813,13.1261401876617,-39.6923246498039));
#18910=CARTESIAN_POINT('',(-36.7666959739416,13.1261401876617,-35.0000237973978));
#18911=CARTESIAN_POINT('',(-36.6799025696119,13.1261401876617,-34.9132303930681));
#18912=CARTESIAN_POINT('Origin',(0.0835265683620477,13.1261401876617,0.0824317919394229));
#18913=CARTESIAN_POINT('Origin',(0.0835265683620477,16.4830954176946,-49.9175682080606));
#18914=CARTESIAN_POINT('',(22.7887737236329,-8.87385981233827,-49.9175682080606));
#18915=CARTESIAN_POINT('',(21.7038295264614,-8.69080155057986,-49.9175682080606));
#18916=CARTESIAN_POINT('Ctrl Pts',(22.7887737236329,-8.87385981233827,-49.9175682080606));
#18917=CARTESIAN_POINT('Ctrl Pts',(22.7188372925805,-8.87385981188611,-49.9175682080606));
#18918=CARTESIAN_POINT('Ctrl Pts',(22.6488692798012,-8.87185808464265,-49.9175682080607));
#18919=CARTESIAN_POINT('Ctrl Pts',(22.5790744235432,-8.86782837150082,-49.9175682080605));
#18920=CARTESIAN_POINT('Ctrl Pts',(22.5081988311883,-8.8637362604018,-49.9175682080604));
#18921=CARTESIAN_POINT('Ctrl Pts',(22.4375001565979,-8.85755327620009,-49.9175682080604));
#18922=CARTESIAN_POINT('Ctrl Pts',(22.3671724444924,-8.84920383564249,-49.9175682080574));
#18923=CARTESIAN_POINT('Ctrl Pts',(22.3238948570106,-8.8440658376423,-49.9175682080556));
#18924=CARTESIAN_POINT('Ctrl Pts',(22.2807574487412,-8.83810648050698,-49.9175682080525));
#18925=CARTESIAN_POINT('Ctrl Pts',(22.2378058279894,-8.83129827231295,-49.9175682080462));
#18926=CARTESIAN_POINT('Ctrl Pts',(22.2374771383617,-8.83124617212726,-49.9175682080461));
#18927=CARTESIAN_POINT('Ctrl Pts',(22.2371484567731,-8.83119402657727,-49.9175682080461));
#18928=CARTESIAN_POINT('Ctrl Pts',(22.2368197832205,-8.83114183558492,-49.917568208046));
#18929=CARTESIAN_POINT('Ctrl Pts',(22.124266225982,-8.81326914154663,-49.9175682080295));
#18930=CARTESIAN_POINT('Ctrl Pts',(22.0129325594699,-8.79011900697469,-49.9175682080505));
#18931=CARTESIAN_POINT('Ctrl Pts',(21.9034992420944,-8.75874571241589,-49.917568208057));
#18932=CARTESIAN_POINT('Ctrl Pts',(21.8361694326296,-8.73944301744522,-49.917568208061));
#18933=CARTESIAN_POINT('Ctrl Pts',(21.7695591263239,-8.71702701269534,-49.9175682080606));
#18934=CARTESIAN_POINT('Ctrl Pts',(21.7038295264635,-8.69080155058071,-49.9175682080606));
#18935=CARTESIAN_POINT('',(44.4585265683622,-8.87385981233827,-49.9175682080604));
#18936=CARTESIAN_POINT('',(0.0835265683620477,-8.87385981233827,-49.9175682080606));
#18937=CARTESIAN_POINT('',(44.4585265683622,-14.4544045823054,-49.9175682080604));
#18938=CARTESIAN_POINT('',(44.4585265683622,16.4830954176946,-49.9175682080604));
#18939=CARTESIAN_POINT('',(-44.2914734316379,-14.4544045823054,-49.9175682080606));
#18940=CARTESIAN_POINT('',(0.0835265683620477,-14.4544045823054,-49.9175682080606));
#18941=CARTESIAN_POINT('',(-44.2914734316379,-8.87385981233827,-49.9175682080606));
#18942=CARTESIAN_POINT('',(-44.2914734316379,16.4830954176946,-49.9175682080606));
#18943=CARTESIAN_POINT('',(-22.6217205869088,-8.87385981233827,-49.9175682080606));
#18944=CARTESIAN_POINT('',(0.0835265683620477,-8.87385981233827,-49.9175682080606));
#18945=CARTESIAN_POINT('',(-21.5367763897373,-8.69080155057986,-49.9175682080606));
#18946=CARTESIAN_POINT('Ctrl Pts',(-21.5367763897373,-8.69080155057986,
-49.9175682080606));
#18947=CARTESIAN_POINT('Ctrl Pts',(-21.6469419836331,-8.73475654612936,
-49.9175682080606));
#18948=CARTESIAN_POINT('Ctrl Pts',(-21.7605113768685,-8.76821292000271,
-49.9175682080606));
#18949=CARTESIAN_POINT('Ctrl Pts',(-21.8753760693094,-8.79411643469424,
-49.9175682080606));
#18950=CARTESIAN_POINT('Ctrl Pts',(-21.9404607776001,-8.80879390138636,
-49.9175682080605));
#18951=CARTESIAN_POINT('Ctrl Pts',(-22.0059610421381,-8.8210476068981,-49.9175682080605));
#18952=CARTESIAN_POINT('Ctrl Pts',(-22.0714936521756,-8.83141832822413,
-49.9175682080604));
#18953=CARTESIAN_POINT('Ctrl Pts',(-22.0715976486236,-8.83143478595685,
-49.9175682080604));
#18954=CARTESIAN_POINT('Ctrl Pts',(-22.0717016456503,-8.83145123875071,
-49.9175682080604));
#18955=CARTESIAN_POINT('Ctrl Pts',(-22.0718056432557,-8.83146768660594,
-49.9175682080604));
#18956=CARTESIAN_POINT('Ctrl Pts',(-22.253099438842,-8.86014040550798,-49.91756820806));
#18957=CARTESIAN_POINT('Ctrl Pts',(-22.4364613235644,-8.87385980853305,
-49.9175682080606));
#18958=CARTESIAN_POINT('Ctrl Pts',(-22.6217205869088,-8.87385981233827,
-49.9175682080606));
#18959=CARTESIAN_POINT('Ctrl Pts',(-21.5367763897373,-8.69080155057986,
-49.9175682080606));
#18960=CARTESIAN_POINT('Ctrl Pts',(-20.6768191353961,-8.34768669239856,
-49.9175682080606));
#18961=CARTESIAN_POINT('Ctrl Pts',(-19.8120276459033,-8.01980178776443,
-49.9175682080606));
#18962=CARTESIAN_POINT('Ctrl Pts',(-18.9419176465726,-7.70866381791265,
-49.9175682080605));
#18963=CARTESIAN_POINT('Ctrl Pts',(-18.0718076472418,-7.39752584806087,
-49.9175682080604));
#18964=CARTESIAN_POINT('Ctrl Pts',(-17.1963790130006,-7.10313511035513,
-49.9175682080604));
#18965=CARTESIAN_POINT('Ctrl Pts',(-16.3151693873186,-6.82695644195446,
-49.9175682080605));
#18966=CARTESIAN_POINT('Ctrl Pts',(-16.3042756711398,-6.82354225770076,
-49.9175682080605));
#18967=CARTESIAN_POINT('Ctrl Pts',(-16.2933810694345,-6.8201308617252,-49.9175682080605));
#18968=CARTESIAN_POINT('Ctrl Pts',(-16.2824855811758,-6.81672225716408,
-49.9175682080605));
#18969=CARTESIAN_POINT('Ctrl Pts',(-15.5378838660857,-6.58377695521956,
-49.9175682080606));
#18970=CARTESIAN_POINT('Ctrl Pts',(-14.7891028645241,-6.3638606691259,-49.917568208062));
#18971=CARTESIAN_POINT('Ctrl Pts',(-14.0359286423201,-6.15798672782537,
-49.9175682080591));
#18972=CARTESIAN_POINT('Ctrl Pts',(-13.9037503637057,-6.1218568891102,-49.9175682080586));
#18973=CARTESIAN_POINT('Ctrl Pts',(-13.7714368304336,-6.08615941360799,
-49.9175682080578));
#18974=CARTESIAN_POINT('Ctrl Pts',(-13.6389869509882,-6.05089962282532,
-49.9175682080567));
#18975=CARTESIAN_POINT('Ctrl Pts',(-13.6273051545214,-6.04778978458984,
-49.9175682080566));
#18976=CARTESIAN_POINT('Ctrl Pts',(-13.6156219114651,-6.0446832728291,-49.9175682080565));
#18977=CARTESIAN_POINT('Ctrl Pts',(-13.6039372399092,-6.04158009539289,
-49.9175682080564));
#18978=CARTESIAN_POINT('Ctrl Pts',(-13.0752254251082,-5.90116651456622,
-49.9175682080514));
#18979=CARTESIAN_POINT('Ctrl Pts',(-12.5437410638479,-5.76761845979613,
-49.9175682080552));
#18980=CARTESIAN_POINT('Ctrl Pts',(-12.0106327436219,-5.6415312830481,-49.9175682080555));
#18981=CARTESIAN_POINT('Ctrl Pts',(-11.6460490610781,-5.55530241458691,
-49.9175682080557));
#18982=CARTESIAN_POINT('Ctrl Pts',(-11.2807047388469,-5.47256360694476,
-49.9175682080568));
#18983=CARTESIAN_POINT('Ctrl Pts',(-10.9149590454957,-5.39351662111492,
-49.9175682080423));
#18984=CARTESIAN_POINT('Ctrl Pts',(-10.9060718037445,-5.39159586118379,
-49.9175682080419));
#18985=CARTESIAN_POINT('Ctrl Pts',(-10.8971843893216,-5.38967730441873,
-49.9175682080416));
#18986=CARTESIAN_POINT('Ctrl Pts',(-10.8882968000924,-5.38776095106793,
-49.9175682080412));
#18987=CARTESIAN_POINT('Ctrl Pts',(-7.25039299962549,-4.60335148320457,
-49.9175682078867));
#18988=CARTESIAN_POINT('Ctrl Pts',(-3.57988304581191,-4.18752460344888,
-49.9175682079243));
#18989=CARTESIAN_POINT('Ctrl Pts',(0.127706037135239,-4.19081815795041,
-49.9175682080454));
#18990=CARTESIAN_POINT('Ctrl Pts',(0.134604712366228,-4.19082428623549,
-49.9175682080457));
#18991=CARTESIAN_POINT('Ctrl Pts',(0.14150351591446,-4.19083186535562,-49.9175682080459));
#18992=CARTESIAN_POINT('Ctrl Pts',(0.148402447809441,-4.19084089563809,
-49.9175682080461));
#18993=CARTESIAN_POINT('Ctrl Pts',(1.06843527170032,-4.19204516267696,-49.917568208075));
#18994=CARTESIAN_POINT('Ctrl Pts',(1.99072993137287,-4.2188222636332,-49.9175682080603));
#18995=CARTESIAN_POINT('Ctrl Pts',(2.91531018987283,-4.27143022964227,-49.9175682080605));
#18996=CARTESIAN_POINT('Ctrl Pts',(2.92625210297229,-4.27205281679694,-49.9175682080605));
#18997=CARTESIAN_POINT('Ctrl Pts',(2.93719445465181,-4.27267902824778,-49.9175682080605));
#18998=CARTESIAN_POINT('Ctrl Pts',(2.94813724502557,-4.27330886465573,-49.9175682080605));
#18999=CARTESIAN_POINT('Ctrl Pts',(3.86878242893392,-4.32629862648307,-49.9175682080607));
#19000=CARTESIAN_POINT('Ctrl Pts',(4.78362256361209,-4.40442769523306,-49.9175682080604));
#19001=CARTESIAN_POINT('Ctrl Pts',(5.69278120066898,-4.50641515619369,-49.9175682080605));
#19002=CARTESIAN_POINT('Ctrl Pts',(5.70666065356689,-4.50797212337509,-49.9175682080605));
#19003=CARTESIAN_POINT('Ctrl Pts',(5.72053877758951,-4.50953465011834,-49.9175682080605));
#19004=CARTESIAN_POINT('Ctrl Pts',(5.73441557288183,-4.51110273180188,-49.9175682080605));
#19005=CARTESIAN_POINT('Ctrl Pts',(6.81408656211051,-4.63310585044643,-49.9175682080606));
#19006=CARTESIAN_POINT('Ctrl Pts',(7.88583325609898,-4.78875206541689,-49.9175682080605));
#19007=CARTESIAN_POINT('Ctrl Pts',(8.95019649950668,-4.97573014441061,-49.9175682080605));
#19008=CARTESIAN_POINT('Ctrl Pts',(9.68564887908743,-5.10492802302684,-49.9175682080605));
#19009=CARTESIAN_POINT('Ctrl Pts',(10.4175763192467,-5.24908423889634,-49.9175682080604));
#19010=CARTESIAN_POINT('Ctrl Pts',(11.1461610317702,-5.40742232363211,-49.9175682080605));
#19011=CARTESIAN_POINT('Ctrl Pts',(11.1607824021305,-5.41059988107913,-49.9175682080605));
#19012=CARTESIAN_POINT('Ctrl Pts',(11.1754024252444,-5.41378314936595,-49.9175682080605));
#19013=CARTESIAN_POINT('Ctrl Pts',(11.1900211026185,-5.41697212217341,-49.9175682080605));
#19014=CARTESIAN_POINT('Ctrl Pts',(12.2995504913854,-5.65900900138633,-49.9175682080606));
#19015=CARTESIAN_POINT('Ctrl Pts',(13.4013634194074,-5.93379674455541,-49.9175682080606));
#19016=CARTESIAN_POINT('Ctrl Pts',(14.4960809935799,-6.23869144821723,-49.9175682080606));
#19017=CARTESIAN_POINT('Ctrl Pts',(15.6085307003123,-6.54852480768373,-49.9175682080606));
#19018=CARTESIAN_POINT('Ctrl Pts',(16.7136533733802,-6.88944821124417,-49.9175682080606));
#19019=CARTESIAN_POINT('Ctrl Pts',(17.8121149578433,-7.25863482928546,-49.9175682080606));
#19020=CARTESIAN_POINT('Ctrl Pts',(18.938442146212,-7.63718691646206,-49.9175682080606));
#19021=CARTESIAN_POINT('Ctrl Pts',(20.0577660356483,-8.04545424377254,-49.9175682080606));
#19022=CARTESIAN_POINT('Ctrl Pts',(21.1708187939427,-8.4803367087649,-49.9175682080606));
#19023=CARTESIAN_POINT('Ctrl Pts',(21.3486480781158,-8.54981664749443,-49.9175682080606));
#19024=CARTESIAN_POINT('Ctrl Pts',(21.526317316444,-8.61997584795984,-49.9175682080606));
#19025=CARTESIAN_POINT('Ctrl Pts',(21.7038295264614,-8.69080155057986,-49.9175682080606));
#19026=CARTESIAN_POINT('Origin',(-49.916473431638,16.4830954176946,0.0824317919394229));
#19027=CARTESIAN_POINT('',(-49.9164734316384,-8.87385981233827,44.4574317919389));
#19028=CARTESIAN_POINT('',(-49.9164734316384,-14.4544045823054,44.4574317919389));
#19029=CARTESIAN_POINT('',(-49.9164734316384,16.4830954176946,44.4574317919389));
#19030=CARTESIAN_POINT('',(-49.916473431638,-8.87385981233827,22.7876789472102));
#19031=CARTESIAN_POINT('',(-49.916473431638,-8.87385981233827,0.0824317919394229));
#19032=CARTESIAN_POINT('',(-49.916473431638,-8.69080155057986,21.7027347500388));
#19033=CARTESIAN_POINT('Ctrl Pts',(-49.916473431638,-8.69080155057985,21.7027347500388));
#19034=CARTESIAN_POINT('Ctrl Pts',(-49.916473431638,-8.73475654611729,21.8129003439043));
#19035=CARTESIAN_POINT('Ctrl Pts',(-49.916473431638,-8.76821291998423,21.9264697371077));
#19036=CARTESIAN_POINT('Ctrl Pts',(-49.916473431638,-8.79411643467275,22.0413344295164));
#19037=CARTESIAN_POINT('Ctrl Pts',(-49.9164734316379,-8.8087939013743,22.1064191378382));
#19038=CARTESIAN_POINT('Ctrl Pts',(-49.9164734316379,-8.82104760689287,
22.1719194024078));
#19039=CARTESIAN_POINT('Ctrl Pts',(-49.9164734316378,-8.83141832822398,
22.2374520124771));
#19040=CARTESIAN_POINT('Ctrl Pts',(-49.9164734316378,-8.8314347859567,22.2375560089251));
#19041=CARTESIAN_POINT('Ctrl Pts',(-49.9164734316378,-8.83145123875055,
22.2376600059518));
#19042=CARTESIAN_POINT('Ctrl Pts',(-49.9164734316378,-8.83146768660578,
22.2377640035571));
#19043=CARTESIAN_POINT('Ctrl Pts',(-49.9164734316374,-8.86014040550796,
22.4190577991434));
#19044=CARTESIAN_POINT('Ctrl Pts',(-49.916473431638,-8.87385980853305,22.6024196838659));
#19045=CARTESIAN_POINT('Ctrl Pts',(-49.916473431638,-8.87385981233827,22.7876789472102));
#19046=CARTESIAN_POINT('',(-49.916473431638,-8.69080155057987,-21.5378711661599));
#19047=CARTESIAN_POINT('Ctrl Pts',(-49.916473431638,-8.69080155057986,21.7027347500388));
#19048=CARTESIAN_POINT('Ctrl Pts',(-49.916473431638,-8.34822820653461,20.8441347059753));
#19049=CARTESIAN_POINT('Ctrl Pts',(-49.9164734316379,-8.02077061917538,
19.9805588353482));
#19050=CARTESIAN_POINT('Ctrl Pts',(-49.9164734316377,-7.70995711777993,
19.1115008037841));
#19051=CARTESIAN_POINT('Ctrl Pts',(-49.9164734316375,-7.4148561321092,18.2863761532518));
#19052=CARTESIAN_POINT('Ctrl Pts',(-49.9164734316374,-7.13475881039956,
17.4563096733183));
#19053=CARTESIAN_POINT('Ctrl Pts',(-49.9164734316377,-6.87092633632312,
16.6208886788675));
#19054=CARTESIAN_POINT('Ctrl Pts',(-49.9164734316377,-6.85687869806059,
16.5764070737578));
#19055=CARTESIAN_POINT('Ctrl Pts',(-49.9164734316378,-6.84287715903063,
16.5319102936858));
#19056=CARTESIAN_POINT('Ctrl Pts',(-49.9164734316378,-6.82892190575843,
16.4873982780546));
#19057=CARTESIAN_POINT('Ctrl Pts',(-49.9164734316378,-6.8242227389863,16.472409701299));
#19058=CARTESIAN_POINT('Ctrl Pts',(-49.9164734316378,-6.81952883192422,
16.4574193922089));
#19059=CARTESIAN_POINT('Ctrl Pts',(-49.9164734316378,-6.81484019286318,
16.4424273479626));
#19060=CARTESIAN_POINT('Ctrl Pts',(-49.9164734316381,-6.54248035969403,
15.571549761391));
#19061=CARTESIAN_POINT('Ctrl Pts',(-49.9164734316437,-6.28791975259315,
14.6948819543752));
#19062=CARTESIAN_POINT('Ctrl Pts',(-49.9164734316321,-6.05269948554821,
13.8117061511833));
#19063=CARTESIAN_POINT('Ctrl Pts',(-49.9164734316319,-6.04801972917164,
13.794135183985));
#19064=CARTESIAN_POINT('Ctrl Pts',(-49.9164734316317,-6.04334784544025,
13.7765622827464));
#19065=CARTESIAN_POINT('Ctrl Pts',(-49.9164734316314,-6.03868385436031,
13.758987494549));
#19066=CARTESIAN_POINT('Ctrl Pts',(-49.9164734316237,-5.8954927971015,13.2194168864696));
#19067=CARTESIAN_POINT('Ctrl Pts',(-49.9164734316301,-5.75970470970634,
12.6779353473642));
#19068=CARTESIAN_POINT('Ctrl Pts',(-49.9164734316267,-5.63181003590257,
12.135443265805));
#19069=CARTESIAN_POINT('Ctrl Pts',(-49.9164734316245,-5.55024150573681,
11.7894532382044));
#19070=CARTESIAN_POINT('Ctrl Pts',(-49.916473431624,-5.47188458180954,11.4430515684158));
#19071=CARTESIAN_POINT('Ctrl Pts',(-49.9164734315809,-5.39687731108541,
11.0964691595927));
#19072=CARTESIAN_POINT('Ctrl Pts',(-49.9164734315788,-5.39311846273983,
11.0791008338099));
#19073=CARTESIAN_POINT('Ctrl Pts',(-49.9164734315765,-5.38936791684796,
11.0617313708499));
#19074=CARTESIAN_POINT('Ctrl Pts',(-49.916473431574,-5.38562567685748,11.044360755025));
#19075=CARTESIAN_POINT('Ctrl Pts',(-49.9164734313206,-4.99630199552335,
9.23720992632475));
#19076=CARTESIAN_POINT('Ctrl Pts',(-49.9164734311946,-4.69745652901532,
7.41999756265195));
#19077=CARTESIAN_POINT('Ctrl Pts',(-49.9164734313608,-4.49601810718718,
5.59209844177902));
#19078=CARTESIAN_POINT('Ctrl Pts',(-49.9164734315186,-4.30470355970131,
3.85606571283916));
#19079=CARTESIAN_POINT('Ctrl Pts',(-49.9164734316221,-4.20125131727341,
2.11039336761343));
#19080=CARTESIAN_POINT('Ctrl Pts',(-49.9164734315923,-4.19154830182168,
0.35454703990375));
#19081=CARTESIAN_POINT('Ctrl Pts',(-49.9164734315908,-4.19103484317222,
0.261632163227361));
#19082=CARTESIAN_POINT('Ctrl Pts',(-49.9164734315888,-4.19078389395497,
0.168688797219065));
#19083=CARTESIAN_POINT('Ctrl Pts',(-49.9164734315863,-4.19079632233919,
0.0757168628223127));
#19084=CARTESIAN_POINT('Ctrl Pts',(-49.9164734315859,-4.19079846573759,
0.0596829285896319));
#19085=CARTESIAN_POINT('Ctrl Pts',(-49.9164734315854,-4.19080843354687,
0.0436473284827703));
#19086=CARTESIAN_POINT('Ctrl Pts',(-49.916473431585,-4.19082622399388,0.0276101156591523));
#19087=CARTESIAN_POINT('Ctrl Pts',(-49.9164734315646,-4.19162018413241,
-0.688105892081282));
#19088=CARTESIAN_POINT('Ctrl Pts',(-49.9164734316302,-4.20800554127586,
-1.40723120732015));
#19089=CARTESIAN_POINT('Ctrl Pts',(-49.9164734316362,-4.23981712342223,
-2.12474644065311));
#19090=CARTESIAN_POINT('Ctrl Pts',(-49.9164734316379,-4.24861125979728,
-2.32309956826786));
#19091=CARTESIAN_POINT('Ctrl Pts',(-49.9164734316379,-4.25858398530448,
-2.52132964566887));
#19092=CARTESIAN_POINT('Ctrl Pts',(-49.9164734316379,-4.26973111075349,
-2.71933074008867));
#19093=CARTESIAN_POINT('Ctrl Pts',(-49.9164734316379,-4.2706085974261,-2.73491711904427));
#19094=CARTESIAN_POINT('Ctrl Pts',(-49.9164734316379,-4.27149329106795,
-2.75050184046942));
#19095=CARTESIAN_POINT('Ctrl Pts',(-49.9164734316379,-4.27238518534672,
-2.76608490257921));
#19096=CARTESIAN_POINT('Ctrl Pts',(-49.9164734316378,-4.32475213351491,
-3.68103348474944));
#19097=CARTESIAN_POINT('Ctrl Pts',(-49.9164734316383,-4.40195367207473,
-4.59033598105189));
#19098=CARTESIAN_POINT('Ctrl Pts',(-49.9164734316376,-4.50277353999861,
-5.49426913991013));
#19099=CARTESIAN_POINT('Ctrl Pts',(-49.9164734316375,-4.50439146708877,
-5.5087751889213));
#19100=CARTESIAN_POINT('Ctrl Pts',(-49.9164734316375,-4.50601548028131,
-5.52327985438146));
#19101=CARTESIAN_POINT('Ctrl Pts',(-49.9164734316375,-4.50764557399692,
-5.53778313755417));
#19102=CARTESIAN_POINT('Ctrl Pts',(-49.9164734316361,-4.67191819991777,
-6.99935089187925));
#19103=CARTESIAN_POINT('Ctrl Pts',(-49.9164734316377,-4.89794158359744,
-8.4468800578816));
#19104=CARTESIAN_POINT('Ctrl Pts',(-49.9164734316379,-5.18003634705726,
-9.88166170717016));
#19105=CARTESIAN_POINT('Ctrl Pts',(-49.916473431638,-5.25026828473809,-10.2388732134829));
#19106=CARTESIAN_POINT('Ctrl Pts',(-49.916473431638,-5.32397599704584,-10.5952945281149));
#19107=CARTESIAN_POINT('Ctrl Pts',(-49.916473431638,-5.40107232558369,-10.9509454768652));
#19108=CARTESIAN_POINT('Ctrl Pts',(-49.916473431638,-5.4034198965424,-10.9617749917663));
#19109=CARTESIAN_POINT('Ctrl Pts',(-49.916473431638,-5.40577060663127,-10.9726037929874));
#19110=CARTESIAN_POINT('Ctrl Pts',(-49.916473431638,-5.40812445329306,-10.9834318811089));
#19111=CARTESIAN_POINT('Ctrl Pts',(-49.916473431638,-5.56766845157895,-11.7173609431609));
#19112=CARTESIAN_POINT('Ctrl Pts',(-49.916473431638,-5.74152740039569,-12.4475970185755));
#19113=CARTESIAN_POINT('Ctrl Pts',(-49.916473431638,-5.9289461269564,-13.1746186103254));
#19114=CARTESIAN_POINT('Ctrl Pts',(-49.916473431638,-6.12360434445706,-13.9297231280625));
#19115=CARTESIAN_POINT('Ctrl Pts',(-49.916473431638,-6.33289027977071,-14.681359999281));
#19116=CARTESIAN_POINT('Ctrl Pts',(-49.916473431638,-6.55601304252968,-15.4300534395904));
#19117=CARTESIAN_POINT('Ctrl Pts',(-49.916473431638,-6.64209054281505,-15.7188884245332));
#19118=CARTESIAN_POINT('Ctrl Pts',(-49.916473431638,-6.73022793651285,-16.0072852182616));
#19119=CARTESIAN_POINT('Ctrl Pts',(-49.916473431638,-6.82038180282843,-16.2952734904535));
#19120=CARTESIAN_POINT('Ctrl Pts',(-49.916473431638,-7.06758554760755,-17.0849432211904));
#19121=CARTESIAN_POINT('Ctrl Pts',(-49.916473431638,-7.33017880636613,-17.872095719996));
#19122=CARTESIAN_POINT('Ctrl Pts',(-49.916473431638,-7.60687660982169,-18.6562161182093));
#19123=CARTESIAN_POINT('Ctrl Pts',(-49.916473431638,-7.8961442096356,-19.4759574487281));
#19124=CARTESIAN_POINT('Ctrl Pts',(-49.916473431638,-8.20082770029567,-20.2923858276412));
#19125=CARTESIAN_POINT('Ctrl Pts',(-49.916473431638,-8.5195083391632,-21.1048868783802));
#19126=CARTESIAN_POINT('Ctrl Pts',(-49.916473431638,-8.57616615668215,-21.249340386539));
#19127=CARTESIAN_POINT('Ctrl Pts',(-49.916473431638,-8.63326651034672,-21.3936696719873));
#19128=CARTESIAN_POINT('Ctrl Pts',(-49.916473431638,-8.69080155057986,-21.5378711661599));
#19129=CARTESIAN_POINT('',(-49.916473431638,-8.87385981233827,-22.6228153633314));
#19130=CARTESIAN_POINT('Ctrl Pts',(-49.916473431638,-8.87385981233827,-22.6228153633314));
#19131=CARTESIAN_POINT('Ctrl Pts',(-49.916473431638,-8.87385981188611,-22.5528789322874));
#19132=CARTESIAN_POINT('Ctrl Pts',(-49.916473431638,-8.87185808464313,-22.4829109195166));
#19133=CARTESIAN_POINT('Ctrl Pts',(-49.9164734316379,-8.86782837150228,
-22.413116063267));
#19134=CARTESIAN_POINT('Ctrl Pts',(-49.9164734316378,-8.86373626040425,
-22.3422404709206));
#19135=CARTESIAN_POINT('Ctrl Pts',(-49.9164734316378,-8.85755327620405,
-22.2715417963385));
#19136=CARTESIAN_POINT('Ctrl Pts',(-49.9164734316348,-8.84920383564849,
-22.2012140842413));
#19137=CARTESIAN_POINT('Ctrl Pts',(-49.9164734316329,-8.84406583764695,
-22.1579364967426));
#19138=CARTESIAN_POINT('Ctrl Pts',(-49.9164734316298,-8.83810648050965,
-22.1147990884564));
#19139=CARTESIAN_POINT('Ctrl Pts',(-49.9164734316236,-8.83129827231297,
-22.0718474676879));
#19140=CARTESIAN_POINT('Ctrl Pts',(-49.9164734316235,-8.83124617212729,
-22.0715187780602));
#19141=CARTESIAN_POINT('Ctrl Pts',(-49.9164734316235,-8.83119402657729,
-22.0711900964716));
#19142=CARTESIAN_POINT('Ctrl Pts',(-49.9164734316234,-8.83114183558494,
-22.070861422919));
#19143=CARTESIAN_POINT('Ctrl Pts',(-49.9164734316069,-8.81326914156542,
-21.9583078657989));
#19144=CARTESIAN_POINT('Ctrl Pts',(-49.9164734316278,-8.79011900702328,
-21.8469741994026));
#19145=CARTESIAN_POINT('Ctrl Pts',(-49.9164734316343,-8.75874571251476,
-21.7375408821381));
#19146=CARTESIAN_POINT('Ctrl Pts',(-49.9164734316383,-8.73944301752175,
-21.6702110725558));
#19147=CARTESIAN_POINT('Ctrl Pts',(-49.916473431638,-8.71702701274011,-21.6036007661347));
#19148=CARTESIAN_POINT('Ctrl Pts',(-49.916473431638,-8.69080155058072,-21.5378711661621));
#19149=CARTESIAN_POINT('',(-49.916473431638,-8.87385981233827,-44.2925682080605));
#19150=CARTESIAN_POINT('',(-49.916473431638,-8.87385981233827,0.0824317919394229));
#19151=CARTESIAN_POINT('',(-49.916473431638,-14.4544045823054,-44.2925682080605));
#19152=CARTESIAN_POINT('',(-49.916473431638,16.4830954176946,-44.2925682080605));
#19153=CARTESIAN_POINT('',(-49.916473431638,-14.4544045823054,0.0824317919394229));
#19154=CARTESIAN_POINT('Origin',(-44.291473431638,16.4830954176946,-44.2925682080606));
#19155=CARTESIAN_POINT('Origin',(-44.291473431638,-8.87385981233827,-44.2925682080606));
#19156=CARTESIAN_POINT('Origin',(-44.291473431638,-14.4544045823054,-44.2925682080606));
#19157=CARTESIAN_POINT('Origin',(0.0835265683620477,16.4830954176946,-49.9175682080606));
#19158=CARTESIAN_POINT('',(44.4585265683622,16.1705954176946,-49.9175682080604));
#19159=CARTESIAN_POINT('',(44.4585265683622,13.4386401876617,-49.9175682080604));
#19160=CARTESIAN_POINT('',(44.4585265683622,16.4830954176946,-49.9175682080604));
#19161=CARTESIAN_POINT('',(11.0320394968432,13.4386401876617,-49.9175682080606));
#19162=CARTESIAN_POINT('',(0.0835265683620477,13.4386401876617,-49.9175682080606));
#19163=CARTESIAN_POINT('',(8.7491915745805,13.2555819259033,-49.9175682080606));
#19164=CARTESIAN_POINT('Ctrl Pts',(8.7491915745807,13.2555819259034,-49.9175682080606));
#19165=CARTESIAN_POINT('Ctrl Pts',(8.99003448998826,13.2969611280011,-49.9175682080606));
#19166=CARTESIAN_POINT('Ctrl Pts',(9.23206419125339,13.3294628821321,-49.9175682080606));
#19167=CARTESIAN_POINT('Ctrl Pts',(9.47484465594503,13.3553162053599,-49.9175682080606));
#19168=CARTESIAN_POINT('Ctrl Pts',(9.61194028432273,13.3699153107618,-49.9175682080606));
#19169=CARTESIAN_POINT('Ctrl Pts',(9.7492755379265,13.3823932020189,-49.9175682080606));
#19170=CARTESIAN_POINT('Ctrl Pts',(9.88677297754905,13.3931443825075,-49.9175682080606));
#19171=CARTESIAN_POINT('Ctrl Pts',(9.88683951929583,13.3931495855305,-49.9175682080606));
#19172=CARTESIAN_POINT('Ctrl Pts',(9.88690606106421,13.3931547881236,-49.9175682080606));
#19173=CARTESIAN_POINT('Ctrl Pts',(9.88697260285417,13.3931599902869,-49.9175682080606));
#19174=CARTESIAN_POINT('Ctrl Pts',(10.268028857282,13.4229505456848,-49.9175682080605));
#19175=CARTESIAN_POINT('Ctrl Pts',(10.6496949233627,13.4386401851025,-49.9175682080606));
#19176=CARTESIAN_POINT('Ctrl Pts',(11.0320394968432,13.4386401876617,-49.9175682080606));
#19177=CARTESIAN_POINT('',(-8.58213843785645,13.2555819259033,-49.9175682080606));
#19178=CARTESIAN_POINT('Ctrl Pts',(8.7491915745805,13.2555819259033,-49.9175682080606));
#19179=CARTESIAN_POINT('Ctrl Pts',(7.5422194222208,13.0482120850067,-49.9175682080606));
#19180=CARTESIAN_POINT('Ctrl Pts',(6.33247425101392,12.8826695784009,-49.9175682080606));
#19181=CARTESIAN_POINT('Ctrl Pts',(5.11985609192787,12.760436563551,-49.9175682080606));
#19182=CARTESIAN_POINT('Ctrl Pts',(3.91790295807075,12.6392785929576,-49.9175682080606));
#19183=CARTESIAN_POINT('Ctrl Pts',(2.7131271460502,12.5606716819903,-49.9175682080606));
#19184=CARTESIAN_POINT('Ctrl Pts',(1.50543703120817,12.5260083291905,-49.9175682080606));
#19185=CARTESIAN_POINT('Ctrl Pts',(1.03589406416592,12.5125314170909,-49.9175682080606));
#19186=CARTESIAN_POINT('Ctrl Pts',(0.565910630292547,12.5056965050877,-49.9175682080606));
#19187=CARTESIAN_POINT('Ctrl Pts',(0.0954815837620025,12.5055833090051,
-49.9175682080606));
#19188=CARTESIAN_POINT('Ctrl Pts',(0.0953271721160354,12.5055832718501,
-49.9175682080606));
#19189=CARTESIAN_POINT('Ctrl Pts',(0.0951727604441331,12.5055832354192,
-49.9175682080606));
#19190=CARTESIAN_POINT('Ctrl Pts',(0.0950183487462883,12.5055831997124,
-49.9175682080606));
#19191=CARTESIAN_POINT('Ctrl Pts',(-0.368415625222207,12.5054760332808,
-49.9175682080606));
#19192=CARTESIAN_POINT('Ctrl Pts',(-0.83251289115487,12.5119501585721,-49.9175682080609));
#19193=CARTESIAN_POINT('Ctrl Pts',(-1.29674624812002,12.5248910213237,-49.9175682080556));
#19194=CARTESIAN_POINT('Ctrl Pts',(-1.76348911659495,12.5379018386435,-49.9175682080503));
#19195=CARTESIAN_POINT('Ctrl Pts',(-2.23037087262208,12.5574495854659,-49.9175682080378));
#19196=CARTESIAN_POINT('Ctrl Pts',(-2.69685756803722,12.5834701483509,-49.9175682080287));
#19197=CARTESIAN_POINT('Ctrl Pts',(-3.15176140393925,12.6088446209459,-49.9175682080198));
#19198=CARTESIAN_POINT('Ctrl Pts',(-3.6062907130313,12.640374766738,-49.9175682080177));
#19199=CARTESIAN_POINT('Ctrl Pts',(-4.05993384799849,12.6780474220078,-49.9175682080302));
#19200=CARTESIAN_POINT('Ctrl Pts',(-4.12648203001281,12.6835738954108,-49.917568208032));
#19201=CARTESIAN_POINT('Ctrl Pts',(-4.19301109425748,12.689232634644,-49.9175682080341));
#19202=CARTESIAN_POINT('Ctrl Pts',(-4.25951937176003,12.6950236788102,-49.9175682080363));
#19203=CARTESIAN_POINT('Ctrl Pts',(-4.26518626359148,12.6955171094344,-49.9175682080365));
#19204=CARTESIAN_POINT('Ctrl Pts',(-4.27085296587595,12.6960114970058,-49.9175682080367));
#19205=CARTESIAN_POINT('Ctrl Pts',(-4.27651947671762,12.6965068414395,-49.9175682080369));
#19206=CARTESIAN_POINT('Ctrl Pts',(-5.12417205630176,12.7706053473349,-49.9175682080647));
#19207=CARTESIAN_POINT('Ctrl Pts',(-5.96958723650869,12.8659719414249,-49.9175682080601));
#19208=CARTESIAN_POINT('Ctrl Pts',(-6.81281170710773,12.9818931835264,-49.9175682080605));
#19209=CARTESIAN_POINT('Ctrl Pts',(-7.403656226973,13.0631188037732,-49.9175682080607));
#19210=CARTESIAN_POINT('Ctrl Pts',(-7.99342539485118,13.1544351597103,-49.9175682080606));
#19211=CARTESIAN_POINT('Ctrl Pts',(-8.58213843785645,13.2555819259033,-49.9175682080606));
#19212=CARTESIAN_POINT('',(-10.8649863601192,13.4386401876617,-49.9175682080606));
#19213=CARTESIAN_POINT('Ctrl Pts',(-10.8649863601192,13.4386401876617,-49.9175682080606));
#19214=CARTESIAN_POINT('Ctrl Pts',(-10.623898890525,13.4386401861139,-49.9175682080606));
#19215=CARTESIAN_POINT('Ctrl Pts',(-10.382962818652,13.4323889945158,-49.9175682080607));
#19216=CARTESIAN_POINT('Ctrl Pts',(-10.1423122637659,13.4203066131622,-49.9175682080605));
#19217=CARTESIAN_POINT('Ctrl Pts',(-10.0015635238242,13.4132400183986,-49.9175682080604));
#19218=CARTESIAN_POINT('Ctrl Pts',(-9.86091228790643,13.4041776979187,-49.9175682080602));
#19219=CARTESIAN_POINT('Ctrl Pts',(-9.72038472080964,13.3931955538157,-49.9175682080593));
#19220=CARTESIAN_POINT('Ctrl Pts',(-9.72013673011797,13.3931761734936,-49.9175682080593));
#19221=CARTESIAN_POINT('Ctrl Pts',(-9.71988874014172,13.3931567875853,-49.9175682080593));
#19222=CARTESIAN_POINT('Ctrl Pts',(-9.71964075088092,13.3931373960886,-49.9175682080593));
#19223=CARTESIAN_POINT('Ctrl Pts',(-9.33859499556313,13.363341559395,-49.917568208057));
#19224=CARTESIAN_POINT('Ctrl Pts',(-8.95909331010943,13.3203465159016,-49.9175682080606));
#19225=CARTESIAN_POINT('Ctrl Pts',(-8.58213843785645,13.2555819259033,-49.9175682080606));
#19226=CARTESIAN_POINT('',(-44.2914734316379,13.4386401876617,-49.9175682080606));
#19227=CARTESIAN_POINT('',(0.0835265683620477,13.4386401876617,-49.9175682080606));
#19228=CARTESIAN_POINT('',(-44.2914734316379,16.1705954176946,-49.9175682080606));
#19229=CARTESIAN_POINT('',(-44.2914734316379,16.4830954176946,-49.9175682080606));
#19230=CARTESIAN_POINT('',(44.4585265683622,16.1705954176946,-49.9175682080606));
#19231=CARTESIAN_POINT('Origin',(-49.916473431638,16.4830954176946,0.0824317919394229));
#19232=CARTESIAN_POINT('',(-49.916473431638,13.4386401876617,11.0309447204206));
#19233=CARTESIAN_POINT('',(-49.916473431638,13.2555819259033,8.74809679815787));
#19234=CARTESIAN_POINT('Ctrl Pts',(-49.916473431638,13.4386401876617,11.0309447204206));
#19235=CARTESIAN_POINT('Ctrl Pts',(-49.916473431638,13.4386401861139,10.7898572509304));
#19236=CARTESIAN_POINT('Ctrl Pts',(-49.916473431638,13.4323889945212,10.548921179161));
#19237=CARTESIAN_POINT('Ctrl Pts',(-49.9164734316379,13.4203066131778,10.3082706243783));
#19238=CARTESIAN_POINT('Ctrl Pts',(-49.9164734316378,13.413240018412,10.1675218843328));
#19239=CARTESIAN_POINT('Ctrl Pts',(-49.9164734316375,13.4041776979268,10.0268706483114));
#19240=CARTESIAN_POINT('Ctrl Pts',(-49.9164734316367,13.3931955538157,9.88634308111107));
#19241=CARTESIAN_POINT('Ctrl Pts',(-49.9164734316367,13.3931761734936,9.8860950904194));
#19242=CARTESIAN_POINT('Ctrl Pts',(-49.9164734316367,13.3931567875854,9.88584710044315));
#19243=CARTESIAN_POINT('Ctrl Pts',(-49.9164734316367,13.3931373960886,9.88559911118235));
#19244=CARTESIAN_POINT('Ctrl Pts',(-49.9164734316343,13.363341559395,9.50455335586456));
#19245=CARTESIAN_POINT('Ctrl Pts',(-49.9164734316379,13.3203465158881,9.12505167041318));
#19246=CARTESIAN_POINT('Ctrl Pts',(-49.9164734316379,13.2555819259033,8.74809679815787));
#19247=CARTESIAN_POINT('',(-49.9164734316384,13.4386401876617,44.4574317919389));
#19248=CARTESIAN_POINT('',(-49.916473431638,13.4386401876617,0.0824317919394229));
#19249=CARTESIAN_POINT('',(-49.9164734316384,16.1705954176946,44.4574317919389));
#19250=CARTESIAN_POINT('',(-49.9164734316384,16.4830954176946,44.4574317919389));
#19251=CARTESIAN_POINT('',(-49.916473431638,16.1705954176946,-44.2925682080605));
#19252=CARTESIAN_POINT('',(-49.916473431638,16.1705954176946,-44.2925682080605));
#19253=CARTESIAN_POINT('',(-49.916473431638,13.4386401876617,-44.2925682080605));
#19254=CARTESIAN_POINT('',(-49.916473431638,16.4830954176946,-44.2925682080605));
#19255=CARTESIAN_POINT('',(-49.916473431638,13.4386401876617,-10.8660811365418));
#19256=CARTESIAN_POINT('',(-49.916473431638,13.4386401876617,0.0824317919394229));
#19257=CARTESIAN_POINT('',(-49.916473431638,13.2555819259033,-8.58323321427904));
#19258=CARTESIAN_POINT('Ctrl Pts',(-49.916473431638,13.2555819259034,-8.58323321427923));
#19259=CARTESIAN_POINT('Ctrl Pts',(-49.916473431638,13.2969611279791,-8.82407612955931));
#19260=CARTESIAN_POINT('Ctrl Pts',(-49.916473431638,13.3294628820976,-9.06610583069568));
#19261=CARTESIAN_POINT('Ctrl Pts',(-49.916473431638,13.3553162053187,-9.308886295258));
#19262=CARTESIAN_POINT('Ctrl Pts',(-49.916473431638,13.3699153107383,-9.44598192376377));
#19263=CARTESIAN_POINT('Ctrl Pts',(-49.9164734316379,13.3823932020088,-9.58331717749613));
#19264=CARTESIAN_POINT('Ctrl Pts',(-49.9164734316379,13.3931443825075,-9.72081461724757));
#19265=CARTESIAN_POINT('Ctrl Pts',(-49.9164734316379,13.3931495855304,-9.72088115899436));
#19266=CARTESIAN_POINT('Ctrl Pts',(-49.9164734316379,13.3931547881236,-9.72094770076274));
#19267=CARTESIAN_POINT('Ctrl Pts',(-49.9164734316379,13.3931599902869,-9.7210142425527));
#19268=CARTESIAN_POINT('Ctrl Pts',(-49.9164734316379,13.4229505456848,-10.1020704969805));
#19269=CARTESIAN_POINT('Ctrl Pts',(-49.916473431638,13.4386401851025,-10.4837365630612));
#19270=CARTESIAN_POINT('Ctrl Pts',(-49.916473431638,13.4386401876617,-10.8660811365418));
#19271=CARTESIAN_POINT('Ctrl Pts',(-49.916473431638,13.2555819259033,-8.58323321427904));
#19272=CARTESIAN_POINT('Ctrl Pts',(-49.916473431638,12.96000054605,-6.86283601154779));
#19273=CARTESIAN_POINT('Ctrl Pts',(-49.9164734316353,12.7491268966531,-5.13488457809543));
#19274=CARTESIAN_POINT('Ctrl Pts',(-49.91647343163,12.627713447568,-3.39929723711238));
#19275=CARTESIAN_POINT('Ctrl Pts',(-49.9164734316266,12.5467548468234,-2.24200598433218));
#19276=CARTESIAN_POINT('Ctrl Pts',(-49.9164734316258,12.5055720509986,-1.08131859955897));
#19277=CARTESIAN_POINT('Ctrl Pts',(-49.9164734316312,12.5055798807548,0.0828009301210683));
#19278=CARTESIAN_POINT('Ctrl Pts',(-49.9164734316312,12.5055799036492,0.0862048405726741));
#19279=CARTESIAN_POINT('Ctrl Pts',(-49.9164734316312,12.5055802787149,0.0896088291256518));
#19280=CARTESIAN_POINT('Ctrl Pts',(-49.9164734316313,12.5055810060177,0.0930128957784022));
#19281=CARTESIAN_POINT('Ctrl Pts',(-49.9164734316359,12.5057958374954,1.09850968428123));
#19282=CARTESIAN_POINT('Ctrl Pts',(-49.9164734316369,12.5366929761477,2.10132408426752));
#19283=CARTESIAN_POINT('Ctrl Pts',(-49.9164734316374,12.5974162153564,3.1015486275048));
#19284=CARTESIAN_POINT('Ctrl Pts',(-49.916473431638,12.658429061564,4.10654353595992));
#19285=CARTESIAN_POINT('Ctrl Pts',(-49.9164734316379,12.7495531744451,5.10892382670438));
#19286=CARTESIAN_POINT('Ctrl Pts',(-49.916473431638,12.8698680207488,6.10879232242438));
#19287=CARTESIAN_POINT('Ctrl Pts',(-49.916473431638,12.9759630639947,6.99048809441394));
#19288=CARTESIAN_POINT('Ctrl Pts',(-49.916473431638,13.1047558095398,7.87023084868606));
#19289=CARTESIAN_POINT('Ctrl Pts',(-49.916473431638,13.2555819259033,8.74809679815787));
#19290=CARTESIAN_POINT('Origin',(-44.291473431638,-14.7669045823054,-44.2925682080606));
#19291=CARTESIAN_POINT('',(49.7710265683622,-14.7669045823054,-44.2925682080604));
#19292=CARTESIAN_POINT('',(49.7710265683619,-14.7669045823054,36.6697170232579));
#19293=CARTESIAN_POINT('',(49.7710265683622,-14.7669045823054,-44.2925682080603));
#19294=CARTESIAN_POINT('',(48.8335265683621,-14.7669045823054,36.6697170232579));
#19295=CARTESIAN_POINT('',(0.0835265683620477,-14.7669045823054,36.6697170232579));
#19296=CARTESIAN_POINT('',(48.8335265683621,-14.7669045823054,34.5598618267976));
#19297=CARTESIAN_POINT('',(48.8335265683621,-14.7669045823054,37.2170722197182));
#19298=CARTESIAN_POINT('',(18.353013239185,-14.7669045823054,24.508895879384));
#19299=CARTESIAN_POINT('',(48.8335265683621,-14.7669045823054,34.5598618267976));
#19300=CARTESIAN_POINT('',(18.7518431265311,-14.7669045823054,23.2994061884498));
#19301=CARTESIAN_POINT('',(32.6717093993989,-14.7669045823054,-18.9139165598666));
#19302=CARTESIAN_POINT('',(46.5214090713319,-14.7669045823054,32.4564357525968));
#19303=CARTESIAN_POINT('',(-58.2113397045057,-14.7669045823054,-2.07924545974433));
#19304=CARTESIAN_POINT('',(47.5194292675621,-14.7669045823054,32.2548881068839));
#19305=CARTESIAN_POINT('Ctrl Pts',(47.5194292675621,-14.7669045823054,32.2548881068839));
#19306=CARTESIAN_POINT('Ctrl Pts',(47.5162066872753,-14.7669045823054,32.2596395478179));
#19307=CARTESIAN_POINT('Ctrl Pts',(47.5129007460645,-14.7669045824339,32.2643216222363));
#19308=CARTESIAN_POINT('Ctrl Pts',(47.5095148041896,-14.7669045818319,32.2689345284333));
#19309=CARTESIAN_POINT('Ctrl Pts',(47.4966520226391,-14.7669045795448,32.2864583982804));
#19310=CARTESIAN_POINT('Ctrl Pts',(47.4826382204761,-14.766904560918,32.302996393618));
#19311=CARTESIAN_POINT('Ctrl Pts',(47.4676517348738,-14.7669044772679,32.3185353475));
#19312=CARTESIAN_POINT('Ctrl Pts',(47.4530508977656,-14.7669043957704,32.3336744361751));
#19313=CARTESIAN_POINT('Ctrl Pts',(47.4375274264405,-14.7669042476547,32.3478657656707));
#19314=CARTESIAN_POINT('Ctrl Pts',(47.4212585314406,-14.7669041441791,32.3611431655407));
#19315=CARTESIAN_POINT('Ctrl Pts',(47.4130166573114,-14.7669040917581,32.3678695386897));
#19316=CARTESIAN_POINT('Ctrl Pts',(47.40458270289,-14.7669040484303,32.3743583583499));
#19317=CARTESIAN_POINT('Ctrl Pts',(47.3959789550955,-14.7669040210232,32.3806110243808));
#19318=CARTESIAN_POINT('Ctrl Pts',(47.3927525496726,-14.7669040107455,32.3829557741424));
#19319=CARTESIAN_POINT('Ctrl Pts',(47.3895022670568,-14.7669040026344,32.3852673148));
#19320=CARTESIAN_POINT('Ctrl Pts',(47.3862292825356,-14.7669039967743,32.3875457201751));
#19321=CARTESIAN_POINT('Ctrl Pts',(47.3833654210796,-14.7669039916467,32.3895393248782));
#19322=CARTESIAN_POINT('Ctrl Pts',(47.3804841784773,-14.7669039882399,32.3915075603807));
#19323=CARTESIAN_POINT('Ctrl Pts',(47.3775863420797,-14.7669039865145,32.3934504761374));
#19324=CARTESIAN_POINT('Ctrl Pts',(47.357301487297,-14.7669039744365,32.4070508864343));
#19325=CARTESIAN_POINT('Ctrl Pts',(47.3362035365451,-14.7669040526285,32.4194106291601));
#19326=CARTESIAN_POINT('Ctrl Pts',(47.3145625513543,-14.7669041305354,32.430546667658));
#19327=CARTESIAN_POINT('Ctrl Pts',(47.2859543315849,-14.7669042335241,32.4452679122732));
#19328=CARTESIAN_POINT('Ctrl Pts',(47.2562626252597,-14.7669043748298,32.4579595038599));
#19329=CARTESIAN_POINT('Ctrl Pts',(47.2258539195548,-14.7669044578905,32.4687823727686));
#19330=CARTESIAN_POINT('Ctrl Pts',(47.2135323703003,-14.7669044915466,32.4731677785016));
#19331=CARTESIAN_POINT('Ctrl Pts',(47.2010930296491,-14.7669045170158,32.4772457401317));
#19332=CARTESIAN_POINT('Ctrl Pts',(47.188560256884,-14.7669045346655,32.4810246061808));
#19333=CARTESIAN_POINT('Ctrl Pts',(47.15181324702,-14.7669045864155,32.4921045188691));
#19334=CARTESIAN_POINT('Ctrl Pts',(47.1142633116265,-14.7669045820527,32.5006221872233));
#19335=CARTESIAN_POINT('Ctrl Pts',(47.0765238293988,-14.7669045822747,32.5068345296263));
#19336=CARTESIAN_POINT('Ctrl Pts',(47.0696355872449,-14.7669045823153,32.5079684116059));
#19337=CARTESIAN_POINT('Ctrl Pts',(47.0627410460591,-14.7669045823054,32.5090253551335));
#19338=CARTESIAN_POINT('Ctrl Pts',(47.0558439863807,-14.7669045823054,32.51000674472));
#19339=CARTESIAN_POINT('Ctrl Pts',(47.0558350832418,-14.7669045823054,32.5100080115567));
#19340=CARTESIAN_POINT('Ctrl Pts',(47.0558261800784,-14.7669045823054,32.5100092782722));
#19341=CARTESIAN_POINT('Ctrl Pts',(47.0558172768906,-14.7669045823054,32.5100105448667));
#19342=CARTESIAN_POINT('Ctrl Pts',(47.0334702770518,-14.7669045823054,32.5131896967335));
#19343=CARTESIAN_POINT('Ctrl Pts',(47.0109580530394,-14.7669045826373,32.5155957537189));
#19344=CARTESIAN_POINT('Ctrl Pts',(46.988364088111,-14.7669045772469,32.5172682730289));
#19345=CARTESIAN_POINT('Ctrl Pts',(46.9544731407184,-14.7669045691613,32.5197770519939));
#19346=CARTESIAN_POINT('Ctrl Pts',(46.9203982755575,-14.766904546284,32.5206353717701));
#19347=CARTESIAN_POINT('Ctrl Pts',(46.8864212383181,-14.7669045319054,32.5199766904459));
#19348=CARTESIAN_POINT('Ctrl Pts',(46.8524442010786,-14.7669045175269,32.5193180091216));
#19349=CARTESIAN_POINT('Ctrl Pts',(46.8185649917614,-14.7669045165844,32.5171423266874));
#19350=CARTESIAN_POINT('Ctrl Pts',(46.7850653560599,-14.7669045221653,32.5135831012478));
#19351=CARTESIAN_POINT('Ctrl Pts',(46.7521381651874,-14.7669045276508,32.510084696177));
#19352=CARTESIAN_POINT('Ctrl Pts',(46.7194212193199,-14.766904544103,32.505250427923));
#19353=CARTESIAN_POINT('Ctrl Pts',(46.6868943696421,-14.7669045570257,32.4991343892605));
#19354=CARTESIAN_POINT('Ctrl Pts',(46.6540025802383,-14.7669045700934,32.4929497308117));
#19355=CARTESIAN_POINT('Ctrl Pts',(46.6213042457889,-14.7669045784001,32.4854538238257));
#19356=CARTESIAN_POINT('Ctrl Pts',(46.5887987004027,-14.7669045808678,32.4766539405727));
#19357=CARTESIAN_POINT('Ctrl Pts',(46.566239175518,-14.7669045825804,32.4705466384841));
#19358=CARTESIAN_POINT('Ctrl Pts',(46.5437729059787,-14.7669045823054,32.4638102368474));
#19359=CARTESIAN_POINT('Ctrl Pts',(46.5214090713319,-14.7669045823054,32.4564357525968));
#19360=CARTESIAN_POINT('',(48.582477269951,-14.7669045823054,30.6288487842779));
#19361=CARTESIAN_POINT('Origin',(0.0835265683620477,-14.7669045823054,0.0824317919394229));
#19362=CARTESIAN_POINT('',(48.833526568362,-14.7669045823054,29.5557152835192));
#19363=CARTESIAN_POINT('Ctrl Pts',(48.833526568362,-14.7669045823054,29.5557152835192));
#19364=CARTESIAN_POINT('Ctrl Pts',(48.8335265671902,-14.7669045823054,29.6860166606407));
#19365=CARTESIAN_POINT('Ctrl Pts',(48.8252222740679,-14.7669045823192,29.8150666965999));
#19366=CARTESIAN_POINT('Ctrl Pts',(48.8072820544696,-14.7669045822898,29.9426399241485));
#19367=CARTESIAN_POINT('Ctrl Pts',(48.7995859656251,-14.7669045822772,29.9973669517645));
#19368=CARTESIAN_POINT('Ctrl Pts',(48.7901172263589,-14.7669045822536,30.0518222752217));
#19369=CARTESIAN_POINT('Ctrl Pts',(48.7787736637774,-14.7669045821918,30.1059884300764));
#19370=CARTESIAN_POINT('Ctrl Pts',(48.7786594332202,-14.7669045821911,30.1065338874674));
#19371=CARTESIAN_POINT('Ctrl Pts',(48.7785450210994,-14.7669045821905,30.1070793522221));
#19372=CARTESIAN_POINT('Ctrl Pts',(48.7784304268186,-14.7669045821899,30.1076248236673));
#19373=CARTESIAN_POINT('Ctrl Pts',(48.7628103615851,-14.7669045821038,30.1819766979346));
#19374=CARTESIAN_POINT('Ctrl Pts',(48.7438390541929,-14.7669045821474,30.2563336460274));
#19375=CARTESIAN_POINT('Ctrl Pts',(48.7199833467506,-14.7669045822053,30.3291843404247));
#19376=CARTESIAN_POINT('Ctrl Pts',(48.701498823388,-14.7669045822502,30.3856324824816));
#19377=CARTESIAN_POINT('Ctrl Pts',(48.6800822715329,-14.7669045822859,30.4411782859976));
#19378=CARTESIAN_POINT('Ctrl Pts',(48.6549907210206,-14.7669045822974,30.4951150676414));
#19379=CARTESIAN_POINT('Ctrl Pts',(48.6336414604553,-14.7669045823072,30.5410074251026));
#19380=CARTESIAN_POINT('Ctrl Pts',(48.609631649145,-14.7669045823054,30.5857353283516));
#19381=CARTESIAN_POINT('Ctrl Pts',(48.582477269951,-14.7669045823054,30.6288487842779));
#19382=CARTESIAN_POINT('',(48.8335265683622,-14.7669045823054,-29.39085169964));
#19383=CARTESIAN_POINT('',(48.8335265683622,-14.7669045823054,-30.3185344755987));
#19384=CARTESIAN_POINT('',(48.5824772699512,-14.7669045823054,-30.4639852003988));
#19385=CARTESIAN_POINT('Ctrl Pts',(48.5824772699512,-14.7669045823054,-30.4639852003988));
#19386=CARTESIAN_POINT('Ctrl Pts',(48.6324063391242,-14.7669045823054,-30.3847121561984));
#19387=CARTESIAN_POINT('Ctrl Pts',(48.6712567149129,-14.7669045823054,-30.2991109807002));
#19388=CARTESIAN_POINT('Ctrl Pts',(48.7346346019905,-14.7669045823054,-30.1242144446989));
#19389=CARTESIAN_POINT('Ctrl Pts',(48.7589711993479,-14.7669045823054,-30.0350331364586));
#19390=CARTESIAN_POINT('Ctrl Pts',(48.8162053854519,-14.7669045823054,-29.7637707034856));
#19391=CARTESIAN_POINT('Ctrl Pts',(48.8335265683622,-14.7669045823054,-29.5772266964482));
#19392=CARTESIAN_POINT('Ctrl Pts',(48.8335265683622,-14.7669045823054,-29.39085169964));
#19393=CARTESIAN_POINT('',(37.8461247099825,-14.7669045823054,-43.0362183703681));
#19394=CARTESIAN_POINT('Origin',(0.0835265683620477,-14.7669045823054,0.0824317919394229));
#19395=CARTESIAN_POINT('',(36.8109793750892,-14.7669045823054,-42.4433312829855));
#19396=CARTESIAN_POINT('Ctrl Pts',(37.8461247099825,-14.7669045823054,-43.0362183703681));
#19397=CARTESIAN_POINT('Ctrl Pts',(37.8298309202723,-14.7669045823054,-43.0504882009569));
#19398=CARTESIAN_POINT('Ctrl Pts',(37.812621196783,-14.7669045823054,-43.0635470401069));
#19399=CARTESIAN_POINT('Ctrl Pts',(37.7946352381859,-14.7669045823054,-43.0752957980133));
#19400=CARTESIAN_POINT('Ctrl Pts',(37.7769014109269,-14.7669045823054,-43.0868798591073));
#19401=CARTESIAN_POINT('Ctrl Pts',(37.7584118543307,-14.7669045823054,-43.0971912466976));
#19402=CARTESIAN_POINT('Ctrl Pts',(37.7392652539178,-14.7669045823054,-43.1061009232293));
#19403=CARTESIAN_POINT('Ctrl Pts',(37.7246902092306,-14.7669045823054,-43.1128832726176));
#19404=CARTESIAN_POINT('Ctrl Pts',(37.7097336127022,-14.7669045823054,-43.1188527973872));
#19405=CARTESIAN_POINT('Ctrl Pts',(37.6944306958395,-14.7669045823054,-43.123933952747));
#19406=CARTESIAN_POINT('Ctrl Pts',(37.6944288513635,-14.7669045823054,-43.1239345651839));
#19407=CARTESIAN_POINT('Ctrl Pts',(37.694427006883,-14.7669045823054,-43.1239351776075));
#19408=CARTESIAN_POINT('Ctrl Pts',(37.6944251623982,-14.7669045823054,-43.123935790018));
#19409=CARTESIAN_POINT('Ctrl Pts',(37.6386324644014,-14.7669045823054,-43.1424602224209));
#19410=CARTESIAN_POINT('Ctrl Pts',(37.5790647273354,-14.7669045823054,-43.1489383928368));
#19411=CARTESIAN_POINT('Ctrl Pts',(37.5205875226989,-14.7669045823054,-43.1443560209437));
#19412=CARTESIAN_POINT('Ctrl Pts',(37.5205836562294,-14.7669045823054,-43.1443557179606));
#19413=CARTESIAN_POINT('Ctrl Pts',(37.5205797897646,-14.7669045823054,-43.1443554149293));
#19414=CARTESIAN_POINT('Ctrl Pts',(37.5205759233047,-14.7669045823054,-43.1443551118495));
#19415=CARTESIAN_POINT('Ctrl Pts',(37.4036218025329,-14.7669045823054,-43.1351874428476));
#19416=CARTESIAN_POINT('Ctrl Pts',(37.2925576207558,-14.7669045823054,-43.0833778715053));
#19417=CARTESIAN_POINT('Ctrl Pts',(37.1988710917299,-14.7669045823054,-43.0132402586517));
#19418=CARTESIAN_POINT('Ctrl Pts',(37.1988648972462,-14.7669045823054,-43.0132356212048));
#19419=CARTESIAN_POINT('Ctrl Pts',(37.1988587028394,-14.7669045823054,-43.013230983672));
#19420=CARTESIAN_POINT('Ctrl Pts',(37.1988525085094,-14.7669045823054,-43.0132263460532));
#19421=CARTESIAN_POINT('Ctrl Pts',(37.1871477901788,-14.7669045823054,-43.0044631670982));
#19422=CARTESIAN_POINT('Ctrl Pts',(37.1756777312701,-14.7669045833006,-42.9954067949474));
#19423=CARTESIAN_POINT('Ctrl Pts',(37.1644411183454,-14.7669045783028,-42.9860779934194));
#19424=CARTESIAN_POINT('Ctrl Pts',(37.1375020351172,-14.7669045663207,-42.9637127698001));
#19425=CARTESIAN_POINT('Ctrl Pts',(37.1118996431171,-14.766904502036,-42.9397826144006));
#19426=CARTESIAN_POINT('Ctrl Pts',(37.0876273944267,-14.7669043153494,-42.9145720776327));
#19427=CARTESIAN_POINT('Ctrl Pts',(37.076446034899,-14.7669042293495,-42.902958482243));
#19428=CARTESIAN_POINT('Ctrl Pts',(37.0655462087051,-14.766904120834,-42.8910733513313));
#19429=CARTESIAN_POINT('Ctrl Pts',(37.0549236503131,-14.7669040086953,-42.8789450456804));
#19430=CARTESIAN_POINT('Ctrl Pts',(37.0380827633631,-14.7669038309118,-42.8597169636288));
#19431=CARTESIAN_POINT('Ctrl Pts',(37.0219431169162,-14.7669036396173,-42.8398770152339));
#19432=CARTESIAN_POINT('Ctrl Pts',(37.0064975538102,-14.7669035207875,-42.8195368438202));
#19433=CARTESIAN_POINT('Ctrl Pts',(36.9987747722572,-14.7669034613726,-42.8093667581133));
#19434=CARTESIAN_POINT('Ctrl Pts',(36.9912255115448,-14.7669034201738,-42.7990716166501));
#19435=CARTESIAN_POINT('Ctrl Pts',(36.9838488770277,-14.7669034045806,-42.7886653748589));
#19436=CARTESIAN_POINT('Ctrl Pts',(36.9764722425106,-14.7669033889875,-42.7782591330677));
#19437=CARTESIAN_POINT('Ctrl Pts',(36.9692682341903,-14.7669033991487,-42.7677417909482));
#19438=CARTESIAN_POINT('Ctrl Pts',(36.9622359573889,-14.7669034367692,-42.7571273039553));
#19439=CARTESIAN_POINT('Ctrl Pts',(36.9439833349958,-14.766903534415,-42.7295768777632));
#19440=CARTESIAN_POINT('Ctrl Pts',(36.9268780766106,-14.7669038199043,-42.7013696444846));
#19441=CARTESIAN_POINT('Ctrl Pts',(36.9108834785333,-14.7669040506412,-42.6725488010595));
#19442=CARTESIAN_POINT('Ctrl Pts',(36.8987074856777,-14.7669042262912,-42.6506087446767));
#19443=CARTESIAN_POINT('Ctrl Pts',(36.8871762981436,-14.7669043666507,-42.6283125394509));
#19444=CARTESIAN_POINT('Ctrl Pts',(36.8762936044956,-14.766904445574,-42.6056762745794));
#19445=CARTESIAN_POINT('Ctrl Pts',(36.8605909997264,-14.7669045594521,-42.5730144784999));
#19446=CARTESIAN_POINT('Ctrl Pts',(36.8462324067551,-14.7669045735796,-42.5396467674435));
#19447=CARTESIAN_POINT('Ctrl Pts',(36.8331795428374,-14.7669045795915,-42.5056252356918));
#19448=CARTESIAN_POINT('Ctrl Pts',(36.8253027509148,-14.7669045832193,-42.4850948349931));
#19449=CARTESIAN_POINT('Ctrl Pts',(36.8179024354812,-14.7669045823054,-42.4643261242436));
#19450=CARTESIAN_POINT('Ctrl Pts',(36.8109793750892,-14.7669045823054,-42.4433312829855));
#19451=CARTESIAN_POINT('',(20.56141397709,-14.7669045823054,6.83502636924522));
#19452=CARTESIAN_POINT('',(20.56141397709,-14.7669045823054,6.83502636924521));
#19453=CARTESIAN_POINT('',(9.92432302202933,-14.7669045823054,19.2683675629017));
#19454=CARTESIAN_POINT('Origin',(0.0835265683620477,-14.7669045823054,0.0824317919394229));
#19455=CARTESIAN_POINT('Origin',(10.2095634989472,-14.7669045823054,19.8244816432194));
#19456=CARTESIAN_POINT('',(14.5949188243533,-14.7669045823054,25.9268725828089));
#19457=CARTESIAN_POINT('',(29.703899630018,-14.7669045823054,-19.8925534551282));
#19458=CARTESIAN_POINT('',(46.9585265683621,-14.7669045823054,36.5987899438301));
#19459=CARTESIAN_POINT('',(-59.4004542373026,-14.7669045823054,1.52685782987659));
#19460=CARTESIAN_POINT('',(46.9585265683621,-14.7669045823054,38.3884670232579));
#19461=CARTESIAN_POINT('',(46.9585265683619,-14.7669045823054,0.0824317919392602));
#19462=CARTESIAN_POINT('',(48.8335265683621,-14.7669045823054,38.3884670232579));
#19463=CARTESIAN_POINT('',(0.0835265683620477,-14.7669045823054,38.3884670232579));
#19464=CARTESIAN_POINT('',(48.8335265683621,-14.7669045823054,37.6072170232579));
#19465=CARTESIAN_POINT('',(48.8335265683619,-14.7669045823054,0.0824317919392537));
#19466=CARTESIAN_POINT('',(0.0835265683620477,-14.7669045823054,37.6072170232579));
#19467=CARTESIAN_POINT('',(44.458526568362,-14.7669045823054,49.7699317919394));
#19468=CARTESIAN_POINT('Origin',(44.4585265683621,-14.7669045823054,44.4574317919394));
#19469=CARTESIAN_POINT('',(-44.2914734316384,-14.7669045823054,49.7699317919394));
#19470=CARTESIAN_POINT('',(-44.2914734316379,-14.7669045823054,49.7699317919394));
#19471=CARTESIAN_POINT('',(-49.603973431638,-14.7669045823054,44.4574317919389));
#19472=CARTESIAN_POINT('Origin',(-44.2914734316384,-14.7669045823054,44.457431791939));
#19473=CARTESIAN_POINT('',(-49.603973431638,-14.7669045823054,-44.2925682080605));
#19474=CARTESIAN_POINT('',(-49.603973431638,-14.7669045823054,-44.2925682080606));
#19475=CARTESIAN_POINT('',(-44.2914734316379,-14.7669045823054,-49.6050682080606));
#19476=CARTESIAN_POINT('Origin',(-44.291473431638,-14.7669045823054,-44.2925682080606));
#19477=CARTESIAN_POINT('',(44.4585265683622,-14.7669045823054,-49.6050682080606));
#19478=CARTESIAN_POINT('',(-44.291473431638,-14.7669045823054,-49.6050682080606));
#19479=CARTESIAN_POINT('Origin',(44.4585265683622,-14.7669045823054,-44.2925682080604));
#19480=CARTESIAN_POINT('',(30.6299435607004,-14.7669045823054,48.5813824935285));
#19481=CARTESIAN_POINT('',(43.2021767306697,-14.7669045823054,37.8450299335598));
#19482=CARTESIAN_POINT('Origin',(0.0835265683620477,-14.7669045823054,0.0824317919394229));
#19483=CARTESIAN_POINT('',(42.6092896432871,-14.7669045823054,36.8098845986664));
#19484=CARTESIAN_POINT('Ctrl Pts',(43.2021767306697,-14.7669045823054,37.8450299335598));
#19485=CARTESIAN_POINT('Ctrl Pts',(43.2164465612568,-14.7669045823054,37.8287361438515));
#19486=CARTESIAN_POINT('Ctrl Pts',(43.2295054004053,-14.7669045823054,37.8115264203645));
#19487=CARTESIAN_POINT('Ctrl Pts',(43.2412541583107,-14.7669045823054,37.7935404617698));
#19488=CARTESIAN_POINT('Ctrl Pts',(43.2528382194038,-14.7669045823054,37.7758066345126));
#19489=CARTESIAN_POINT('Ctrl Pts',(43.2631496069936,-14.7669045823054,37.7573170779186));
#19490=CARTESIAN_POINT('Ctrl Pts',(43.2720592835251,-14.7669045823054,37.7381704775078));
#19491=CARTESIAN_POINT('Ctrl Pts',(43.2788416329158,-14.7669045823054,37.7235954328166));
#19492=CARTESIAN_POINT('Ctrl Pts',(43.2848111576874,-14.7669045823054,37.708638836284));
#19493=CARTESIAN_POINT('Ctrl Pts',(43.2898923130487,-14.7669045823054,37.6933359194168));
#19494=CARTESIAN_POINT('Ctrl Pts',(43.2898929254855,-14.7669045823054,37.6933340749407));
#19495=CARTESIAN_POINT('Ctrl Pts',(43.2898935379092,-14.7669045823054,37.6933322304602));
#19496=CARTESIAN_POINT('Ctrl Pts',(43.2898941503197,-14.7669045823054,37.6933303859754));
#19497=CARTESIAN_POINT('Ctrl Pts',(43.3084185827225,-14.7669045823054,37.6375376879786));
#19498=CARTESIAN_POINT('Ctrl Pts',(43.3148967531382,-14.7669045823054,37.5779699509127));
#19499=CARTESIAN_POINT('Ctrl Pts',(43.3103143812451,-14.7669045823054,37.5194927462761));
#19500=CARTESIAN_POINT('Ctrl Pts',(43.3103140782621,-14.7669045823054,37.5194888798066));
#19501=CARTESIAN_POINT('Ctrl Pts',(43.3103137752307,-14.7669045823054,37.5194850133419));
#19502=CARTESIAN_POINT('Ctrl Pts',(43.310313472151,-14.7669045823054,37.5194811468819));
#19503=CARTESIAN_POINT('Ctrl Pts',(43.3011458031491,-14.7669045823054,37.4025270261101));
#19504=CARTESIAN_POINT('Ctrl Pts',(43.2493362318067,-14.7669045823054,37.2914628443332));
#19505=CARTESIAN_POINT('Ctrl Pts',(43.1791986189533,-14.7669045823054,37.1977763153071));
#19506=CARTESIAN_POINT('Ctrl Pts',(43.1791939815064,-14.7669045823054,37.1977701208234));
#19507=CARTESIAN_POINT('Ctrl Pts',(43.1791893439736,-14.7669045823054,37.1977639264166));
#19508=CARTESIAN_POINT('Ctrl Pts',(43.1791847063548,-14.7669045823054,37.1977577320866));
#19509=CARTESIAN_POINT('Ctrl Pts',(43.1704215273998,-14.7669045823054,37.186053013756));
#19510=CARTESIAN_POINT('Ctrl Pts',(43.1613651552491,-14.7669045833006,37.1745829548473));
#19511=CARTESIAN_POINT('Ctrl Pts',(43.152036353721,-14.7669045783028,37.1633463419226));
#19512=CARTESIAN_POINT('Ctrl Pts',(43.129671130102,-14.7669045663207,37.1364072586948));
#19513=CARTESIAN_POINT('Ctrl Pts',(43.1057409747029,-14.766904502036,37.110804866695));
#19514=CARTESIAN_POINT('Ctrl Pts',(43.0805304379353,-14.7669043153494,37.0865326180049));
#19515=CARTESIAN_POINT('Ctrl Pts',(43.0689168425453,-14.7669042293495,37.0753512584769));
#19516=CARTESIAN_POINT('Ctrl Pts',(43.0570317116333,-14.766904120834,37.0644514322827));
#19517=CARTESIAN_POINT('Ctrl Pts',(43.0449034059821,-14.7669040086953,37.0538288738903));
#19518=CARTESIAN_POINT('Ctrl Pts',(43.0256753239304,-14.7669038309118,37.0369879869403));
#19519=CARTESIAN_POINT('Ctrl Pts',(43.0058353755356,-14.7669036396173,37.0208483404934));
#19520=CARTESIAN_POINT('Ctrl Pts',(42.9854952041218,-14.7669035207875,37.0054027773874));
#19521=CARTESIAN_POINT('Ctrl Pts',(42.975325118415,-14.7669034613726,36.9976799958344));
#19522=CARTESIAN_POINT('Ctrl Pts',(42.9650299769516,-14.7669034201738,36.990130735122));
#19523=CARTESIAN_POINT('Ctrl Pts',(42.9546237351605,-14.7669034045806,36.982754100605));
#19524=CARTESIAN_POINT('Ctrl Pts',(42.9442174933693,-14.7669033889875,36.9753774660879));
#19525=CARTESIAN_POINT('Ctrl Pts',(42.9337001512499,-14.7669033991487,36.9681734577675));
#19526=CARTESIAN_POINT('Ctrl Pts',(42.9230856642569,-14.7669034367692,36.9611411809661));
#19527=CARTESIAN_POINT('Ctrl Pts',(42.8955352380647,-14.766903534415,36.9428885585729));
#19528=CARTESIAN_POINT('Ctrl Pts',(42.8673280047859,-14.7669038199043,36.9257833001877));
#19529=CARTESIAN_POINT('Ctrl Pts',(42.8385071613608,-14.7669040506412,36.9097887021103));
#19530=CARTESIAN_POINT('Ctrl Pts',(42.8165671049781,-14.7669042262912,36.8976127092548));
#19531=CARTESIAN_POINT('Ctrl Pts',(42.7942708997524,-14.7669043666507,36.8860815217207));
#19532=CARTESIAN_POINT('Ctrl Pts',(42.771634634881,-14.766904445574,36.8751988280728));
#19533=CARTESIAN_POINT('Ctrl Pts',(42.7389728388023,-14.7669045594521,36.859496223304));
#19534=CARTESIAN_POINT('Ctrl Pts',(42.7056051277468,-14.7669045735796,36.845137630333));
#19535=CARTESIAN_POINT('Ctrl Pts',(42.6715835959959,-14.7669045795915,36.8320847664156));
#19536=CARTESIAN_POINT('Ctrl Pts',(42.6510531952964,-14.7669045832193,36.8242079744926));
#19537=CARTESIAN_POINT('Ctrl Pts',(42.6302844845461,-14.7669045823054,36.8168076590587));
#19538=CARTESIAN_POINT('Ctrl Pts',(42.6092896432871,-14.7669045823054,36.8098845986664));
#19539=CARTESIAN_POINT('',(-6.66906800894368,-14.7669045823054,20.5603192006674));
#19540=CARTESIAN_POINT('',(-6.66906800894368,-14.7669045823054,20.5603192006674));
#19541=CARTESIAN_POINT('',(-19.1024092026003,-14.7669045823054,9.9232282456065));
#19542=CARTESIAN_POINT('Origin',(0.0835265683620477,-14.7669045823054,0.0824317919394229));
#19543=CARTESIAN_POINT('',(-20.2520852367942,-14.7669045823054,10.012741343472));
#19544=CARTESIAN_POINT('Origin',(-19.6585232829181,-14.7669045823054,10.2084687225244));
#19545=CARTESIAN_POINT('',(-32.2904773922958,-14.7669045823054,46.520314294909));
#19546=CARTESIAN_POINT('',(-6.45864799006472,-14.7669045823054,-31.8171733188375));
#19547=CARTESIAN_POINT('',(-32.0889297465829,-14.7669045823054,47.5183344911391));
#19548=CARTESIAN_POINT('Ctrl Pts',(-32.0889297465829,-14.7669045823054,
47.5183344911391));
#19549=CARTESIAN_POINT('Ctrl Pts',(-32.093681187517,-14.7669045823054,47.5151119108524));
#19550=CARTESIAN_POINT('Ctrl Pts',(-32.0983632619353,-14.7669045824339,
47.5118059696416));
#19551=CARTESIAN_POINT('Ctrl Pts',(-32.1029761681324,-14.7669045818319,
47.5084200277666));
#19552=CARTESIAN_POINT('Ctrl Pts',(-32.1205000379794,-14.7669045795448,
47.4955572462162));
#19553=CARTESIAN_POINT('Ctrl Pts',(-32.137038033317,-14.7669045609181,47.4815434440533));
#19554=CARTESIAN_POINT('Ctrl Pts',(-32.1525769871989,-14.7669044772679,
47.466556958451));
#19555=CARTESIAN_POINT('Ctrl Pts',(-32.1677160758741,-14.7669043957704,
47.4519561213427));
#19556=CARTESIAN_POINT('Ctrl Pts',(-32.1819074053697,-14.7669042476547,
47.4364326500176));
#19557=CARTESIAN_POINT('Ctrl Pts',(-32.1951848052397,-14.7669041441791,
47.4201637550177));
#19558=CARTESIAN_POINT('Ctrl Pts',(-32.2019111783887,-14.7669040917581,
47.4119218808885));
#19559=CARTESIAN_POINT('Ctrl Pts',(-32.208399998049,-14.7669040484303,47.4034879264671));
#19560=CARTESIAN_POINT('Ctrl Pts',(-32.2146526640799,-14.7669040210232,
47.3948841786726));
#19561=CARTESIAN_POINT('Ctrl Pts',(-32.2169974138415,-14.7669040107455,
47.3916577732497));
#19562=CARTESIAN_POINT('Ctrl Pts',(-32.2193089544991,-14.7669040026344,
47.3884074906338));
#19563=CARTESIAN_POINT('Ctrl Pts',(-32.2215873598741,-14.7669039967743,
47.3851345061127));
#19564=CARTESIAN_POINT('Ctrl Pts',(-32.2235809645773,-14.7669039916468,
47.3822706446566));
#19565=CARTESIAN_POINT('Ctrl Pts',(-32.2255492000797,-14.7669039882399,
47.3793894020543));
#19566=CARTESIAN_POINT('Ctrl Pts',(-32.2274921158364,-14.7669039865145,
47.3764915656568));
#19567=CARTESIAN_POINT('Ctrl Pts',(-32.2410925261333,-14.7669039744365,
47.3562067108741));
#19568=CARTESIAN_POINT('Ctrl Pts',(-32.2534522688591,-14.7669040526285,
47.3351087601222));
#19569=CARTESIAN_POINT('Ctrl Pts',(-32.264588307357,-14.7669041305354,47.3134677749313));
#19570=CARTESIAN_POINT('Ctrl Pts',(-32.2793095519727,-14.7669042335241,
47.2848595551612));
#19571=CARTESIAN_POINT('Ctrl Pts',(-32.2920011435596,-14.7669043748298,
47.2551678488351));
#19572=CARTESIAN_POINT('Ctrl Pts',(-32.3028240124684,-14.7669044578905,
47.2247591431293));
#19573=CARTESIAN_POINT('Ctrl Pts',(-32.3072094182012,-14.7669044915466,
47.2124375938757));
#19574=CARTESIAN_POINT('Ctrl Pts',(-32.311287379831,-14.7669045170158,47.1999982532253));
#19575=CARTESIAN_POINT('Ctrl Pts',(-32.3150662458798,-14.7669045346655,
47.187465480461));
#19576=CARTESIAN_POINT('Ctrl Pts',(-32.3261461585685,-14.7669045864155,
47.1507184705958));
#19577=CARTESIAN_POINT('Ctrl Pts',(-32.3346638269229,-14.7669045820527,
47.1131685352009));
#19578=CARTESIAN_POINT('Ctrl Pts',(-32.340876169326,-14.7669045822747,47.0754290529718));
#19579=CARTESIAN_POINT('Ctrl Pts',(-32.3420100513053,-14.7669045823153,
47.0685408108192));
#19580=CARTESIAN_POINT('Ctrl Pts',(-32.3430669948327,-14.7669045823054,
47.0616462696348));
#19581=CARTESIAN_POINT('Ctrl Pts',(-32.3440483844191,-14.7669045823054,
47.0547492099578));
#19582=CARTESIAN_POINT('Ctrl Pts',(-32.3440496512557,-14.7669045823054,
47.0547403068188));
#19583=CARTESIAN_POINT('Ctrl Pts',(-32.3440509179712,-14.7669045823054,
47.0547314036554));
#19584=CARTESIAN_POINT('Ctrl Pts',(-32.3440521845657,-14.7669045823054,
47.0547225004677));
#19585=CARTESIAN_POINT('Ctrl Pts',(-32.3472313364325,-14.7669045823054,
47.0323755006289));
#19586=CARTESIAN_POINT('Ctrl Pts',(-32.3496373934179,-14.7669045826373,
47.0098632766164));
#19587=CARTESIAN_POINT('Ctrl Pts',(-32.3513099127279,-14.7669045772469,
46.987269311688));
#19588=CARTESIAN_POINT('Ctrl Pts',(-32.353818691693,-14.7669045691613,46.9533783642954));
#19589=CARTESIAN_POINT('Ctrl Pts',(-32.3546770114691,-14.766904546284,46.9193034991345));
#19590=CARTESIAN_POINT('Ctrl Pts',(-32.3540183301449,-14.7669045319054,
46.8853264618951));
#19591=CARTESIAN_POINT('Ctrl Pts',(-32.3533596488207,-14.7669045175269,
46.8513494246557));
#19592=CARTESIAN_POINT('Ctrl Pts',(-32.3511839663865,-14.7669045165844,
46.8174702153385));
#19593=CARTESIAN_POINT('Ctrl Pts',(-32.3476247409469,-14.7669045221653,
46.783970579637));
#19594=CARTESIAN_POINT('Ctrl Pts',(-32.3441263358758,-14.7669045276508,
46.7510433887625));
#19595=CARTESIAN_POINT('Ctrl Pts',(-32.3392920676214,-14.766904544103,46.718326442893));
#19596=CARTESIAN_POINT('Ctrl Pts',(-32.3331760289583,-14.7669045570257,
46.6857995932133));
#19597=CARTESIAN_POINT('Ctrl Pts',(-32.3269913705088,-14.7669045700934,
46.6529078038072));
#19598=CARTESIAN_POINT('Ctrl Pts',(-32.319495463522,-14.7669045784001,46.6202094693554));
#19599=CARTESIAN_POINT('Ctrl Pts',(-32.310695580268,-14.7669045808678,46.5877039239669));
#19600=CARTESIAN_POINT('Ctrl Pts',(-32.3045882781803,-14.7669045825804,
46.5651443990865));
#19601=CARTESIAN_POINT('Ctrl Pts',(-32.2978518765448,-14.7669045823054,
46.5426781295515));
#19602=CARTESIAN_POINT('Ctrl Pts',(-32.2904773922958,-14.7669045823054,
46.520314294909));
#19603=CARTESIAN_POINT('',(-30.4628904239763,-14.7669045823054,48.5813824935285));
#19604=CARTESIAN_POINT('Origin',(0.0835265683620477,-14.7669045823054,0.0824317919394229));
#19605=CARTESIAN_POINT('',(-29.3897569232175,-14.7669045823054,48.8324317919394));
#19606=CARTESIAN_POINT('Ctrl Pts',(-29.3897569232175,-14.7669045823054,
48.8324317919394));
#19607=CARTESIAN_POINT('Ctrl Pts',(-29.5200807466481,-14.7669045823054,
48.8324317908));
#19608=CARTESIAN_POINT('Ctrl Pts',(-29.6491709400179,-14.7669045823184,
48.8241256340683));
#19609=CARTESIAN_POINT('Ctrl Pts',(-29.7768043956785,-14.7669045822907,
48.8061704983924));
#19610=CARTESIAN_POINT('Ctrl Pts',(-29.8315190134296,-14.7669045822788,
48.7984733912343));
#19611=CARTESIAN_POINT('Ctrl Pts',(-29.8859659940187,-14.7669045822566,
48.7890037111312));
#19612=CARTESIAN_POINT('Ctrl Pts',(-29.9401280908703,-14.7669045821984,
48.7776586172617));
#19613=CARTESIAN_POINT('Ctrl Pts',(-29.9406641464146,-14.7669045821978,
48.7775463320877));
#19614=CARTESIAN_POINT('Ctrl Pts',(-29.9412002084696,-14.7669045821972,
48.7774338713268));
#19615=CARTESIAN_POINT('Ctrl Pts',(-29.9417362763945,-14.7669045821967,
48.7773212344192));
#19616=CARTESIAN_POINT('Ctrl Pts',(-30.0123701479919,-14.7669045821198,
48.7624798673106));
#19617=CARTESIAN_POINT('Ctrl Pts',(-30.0829795903623,-14.7669045821514,
48.7446144797856));
#19618=CARTESIAN_POINT('Ctrl Pts',(-30.1522892880597,-14.766904582203,48.7224220884003));
#19619=CARTESIAN_POINT('Ctrl Pts',(-30.2064608535874,-14.7669045822433,
48.7050768016066));
#19620=CARTESIAN_POINT('Ctrl Pts',(-30.2598402837736,-14.7669045822799,
48.6850886651948));
#19621=CARTESIAN_POINT('Ctrl Pts',(-30.3118149289063,-14.7669045822938,
48.6618061992418));
#19622=CARTESIAN_POINT('Ctrl Pts',(-30.360916740954,-14.7669045823069,48.639810642287));
#19623=CARTESIAN_POINT('Ctrl Pts',(-30.408765698194,-14.7669045823054,48.6148755124272));
#19624=CARTESIAN_POINT('Ctrl Pts',(-30.4548245533698,-14.7669045823054,
48.5864144376838));
#19625=CARTESIAN_POINT('Ctrl Pts',(-30.4575193501094,-14.7669045823054,
48.5847492462428));
#19626=CARTESIAN_POINT('Ctrl Pts',(-30.4602080106262,-14.7669045823054,
48.5830719723037));
#19627=CARTESIAN_POINT('Ctrl Pts',(-30.4628904239763,-14.7669045823054,
48.5813824935285));
#19628=CARTESIAN_POINT('',(29.5568100599416,-14.7669045823054,48.8324317919394));
#19629=CARTESIAN_POINT('',(30.4844928359003,-14.7669045823054,48.8324317919394));
#19630=CARTESIAN_POINT('Ctrl Pts',(30.6299435607004,-14.7669045823054,48.5813824935285));
#19631=CARTESIAN_POINT('Ctrl Pts',(30.5506705165001,-14.7669045823054,48.6313115627014));
#19632=CARTESIAN_POINT('Ctrl Pts',(30.4650693410018,-14.7669045823054,48.6701619384902));
#19633=CARTESIAN_POINT('Ctrl Pts',(30.2901728050006,-14.7669045823054,48.7335398255678));
#19634=CARTESIAN_POINT('Ctrl Pts',(30.2009914967602,-14.7669045823054,48.7578764229251));
#19635=CARTESIAN_POINT('Ctrl Pts',(29.9297290637873,-14.7669045823054,48.8151106090292));
#19636=CARTESIAN_POINT('Ctrl Pts',(29.7431850567499,-14.7669045823054,48.8324317919394));
#19637=CARTESIAN_POINT('Ctrl Pts',(29.5568100599416,-14.7669045823054,48.8324317919394));
#19638=CARTESIAN_POINT('',(-30.4628904239763,-14.7669045823054,-48.4165189096496));
#19639=CARTESIAN_POINT('',(-43.0351235939456,-14.7669045823054,-37.6801663496809));
#19640=CARTESIAN_POINT('Origin',(0.0835265683620477,-14.7669045823054,0.0824317919394229));
#19641=CARTESIAN_POINT('',(-42.442236506563,-14.7669045823054,-36.6450210147876));
#19642=CARTESIAN_POINT('Ctrl Pts',(-43.0351235939456,-14.7669045823054,
-37.6801663496809));
#19643=CARTESIAN_POINT('Ctrl Pts',(-43.0493934245332,-14.7669045823054,
-37.663872559972));
#19644=CARTESIAN_POINT('Ctrl Pts',(-43.0624522636822,-14.7669045823054,
-37.6466628364843));
#19645=CARTESIAN_POINT('Ctrl Pts',(-43.0742010215879,-14.7669045823054,
-37.6286768778889));
#19646=CARTESIAN_POINT('Ctrl Pts',(-43.085785082681,-14.7669045823054,-37.6109430506316));
#19647=CARTESIAN_POINT('Ctrl Pts',(-43.0960964702708,-14.7669045823054,
-37.5924534940372));
#19648=CARTESIAN_POINT('Ctrl Pts',(-43.1050061468023,-14.7669045823054,
-37.5733068936262));
#19649=CARTESIAN_POINT('Ctrl Pts',(-43.1117884961925,-14.7669045823054,
-37.5587318489358));
#19650=CARTESIAN_POINT('Ctrl Pts',(-43.1177580209636,-14.7669045823054,
-37.5437752524041));
#19651=CARTESIAN_POINT('Ctrl Pts',(-43.1228391763247,-14.7669045823054,
-37.5284723355379));
#19652=CARTESIAN_POINT('Ctrl Pts',(-43.1228397887615,-14.7669045823054,
-37.5284704910619));
#19653=CARTESIAN_POINT('Ctrl Pts',(-43.1228404011851,-14.7669045823054,
-37.5284686465814));
#19654=CARTESIAN_POINT('Ctrl Pts',(-43.1228410135956,-14.7669045823054,
-37.5284668020966));
#19655=CARTESIAN_POINT('Ctrl Pts',(-43.1413654459984,-14.7669045823054,
-37.4726741040998));
#19656=CARTESIAN_POINT('Ctrl Pts',(-43.1478436164141,-14.7669045823054,
-37.4131063670338));
#19657=CARTESIAN_POINT('Ctrl Pts',(-43.1432612445211,-14.7669045823054,
-37.3546291623973));
#19658=CARTESIAN_POINT('Ctrl Pts',(-43.143260941538,-14.7669045823054,-37.3546252959278));
#19659=CARTESIAN_POINT('Ctrl Pts',(-43.1432606385066,-14.7669045823054,
-37.354621429463));
#19660=CARTESIAN_POINT('Ctrl Pts',(-43.1432603354269,-14.7669045823054,
-37.354617563003));
#19661=CARTESIAN_POINT('Ctrl Pts',(-43.134092666425,-14.7669045823054,-37.2376634422313));
#19662=CARTESIAN_POINT('Ctrl Pts',(-43.0822830950826,-14.7669045823054,
-37.1265992604543));
#19663=CARTESIAN_POINT('Ctrl Pts',(-43.0121454822292,-14.7669045823054,
-37.0329127314283));
#19664=CARTESIAN_POINT('Ctrl Pts',(-43.0121408447823,-14.7669045823054,
-37.0329065369446));
#19665=CARTESIAN_POINT('Ctrl Pts',(-43.0121362072495,-14.7669045823054,
-37.0329003425378));
#19666=CARTESIAN_POINT('Ctrl Pts',(-43.0121315696307,-14.7669045823054,
-37.0328941482078));
#19667=CARTESIAN_POINT('Ctrl Pts',(-43.0033683906757,-14.7669045823054,
-37.0211894298772));
#19668=CARTESIAN_POINT('Ctrl Pts',(-42.994312018525,-14.7669045833006,-37.0097193709685));
#19669=CARTESIAN_POINT('Ctrl Pts',(-42.9849832169969,-14.7669045783028,
-36.9984827580438));
#19670=CARTESIAN_POINT('Ctrl Pts',(-42.9626179933785,-14.7669045663207,
-36.9715436748167));
#19671=CARTESIAN_POINT('Ctrl Pts',(-42.9386878379802,-14.766904502036,-36.9459412828177));
#19672=CARTESIAN_POINT('Ctrl Pts',(-42.9134773012134,-14.7669043153494,
-36.9216690341282));
#19673=CARTESIAN_POINT('Ctrl Pts',(-42.9018637058227,-14.7669042293495,
-36.9104876745995));
#19674=CARTESIAN_POINT('Ctrl Pts',(-42.8899785749099,-14.766904120834,-36.8995878484045));
#19675=CARTESIAN_POINT('Ctrl Pts',(-42.877850269258,-14.7669040086953,-36.8889652900115));
#19676=CARTESIAN_POINT('Ctrl Pts',(-42.8586221872063,-14.7669038309118,
-36.8721244030615));
#19677=CARTESIAN_POINT('Ctrl Pts',(-42.8387822388114,-14.7669036396173,
-36.8559847566146));
#19678=CARTESIAN_POINT('Ctrl Pts',(-42.8184420673977,-14.7669035207875,
-36.8405391935086));
#19679=CARTESIAN_POINT('Ctrl Pts',(-42.8082719816908,-14.7669034613726,
-36.8328164119555));
#19680=CARTESIAN_POINT('Ctrl Pts',(-42.7979768402275,-14.7669034201738,
-36.8252671512432));
#19681=CARTESIAN_POINT('Ctrl Pts',(-42.7875705984364,-14.7669034045806,
-36.8178905167261));
#19682=CARTESIAN_POINT('Ctrl Pts',(-42.7771643566452,-14.7669033889875,
-36.810513882209));
#19683=CARTESIAN_POINT('Ctrl Pts',(-42.7666470145257,-14.7669033991487,
-36.8033098738887));
#19684=CARTESIAN_POINT('Ctrl Pts',(-42.7560325275328,-14.7669034367692,
-36.7962775970873));
#19685=CARTESIAN_POINT('Ctrl Pts',(-42.7284821013409,-14.766903534415,-36.7780249746943));
#19686=CARTESIAN_POINT('Ctrl Pts',(-42.7002748680626,-14.7669038199043,
-36.7609197163093));
#19687=CARTESIAN_POINT('Ctrl Pts',(-42.6714540246378,-14.7669040506412,
-36.7449251182321));
#19688=CARTESIAN_POINT('Ctrl Pts',(-42.6495139682548,-14.7669042262912,
-36.7327491253764));
#19689=CARTESIAN_POINT('Ctrl Pts',(-42.6272177630288,-14.7669043666507,
-36.7212179378421));
#19690=CARTESIAN_POINT('Ctrl Pts',(-42.6045814981569,-14.766904445574,-36.7103352441939));
#19691=CARTESIAN_POINT('Ctrl Pts',(-42.5719197020778,-14.7669045594521,
-36.694632639425));
#19692=CARTESIAN_POINT('Ctrl Pts',(-42.5385519910219,-14.7669045735796,
-36.6802740464539));
#19693=CARTESIAN_POINT('Ctrl Pts',(-42.5045304592707,-14.7669045795915,
-36.6672211825363));
#19694=CARTESIAN_POINT('Ctrl Pts',(-42.4840000585715,-14.7669045832193,
-36.6593443906135));
#19695=CARTESIAN_POINT('Ctrl Pts',(-42.4632313478216,-14.7669045823054,
-36.6519440751797));
#19696=CARTESIAN_POINT('Ctrl Pts',(-42.442236506563,-14.7669045823054,-36.6450210147876));
#19697=CARTESIAN_POINT('',(6.83612114566778,-14.7669045823054,-20.3954556167886));
#19698=CARTESIAN_POINT('',(6.83612114566778,-14.7669045823054,-20.3954556167886));
#19699=CARTESIAN_POINT('Origin',(0.0835265683620477,-14.7669045823054,0.0824317919394229));
#19700=CARTESIAN_POINT('',(32.4575305290195,-14.7669045823054,-46.3554507110303));
#19701=CARTESIAN_POINT('',(24.3171104787687,-14.7669045823054,-21.6688501250819));
#19702=CARTESIAN_POINT('',(32.2559828833067,-14.7669045823054,-47.3534709072605));
#19703=CARTESIAN_POINT('Ctrl Pts',(32.2559828833067,-14.7669045823054,-47.3534709072605));
#19704=CARTESIAN_POINT('Ctrl Pts',(32.2607343242407,-14.7669045823054,-47.3502483269737));
#19705=CARTESIAN_POINT('Ctrl Pts',(32.2654163986591,-14.7669045824339,-47.3469423857629));
#19706=CARTESIAN_POINT('Ctrl Pts',(32.2700293048561,-14.7669045818318,-47.343556443888));
#19707=CARTESIAN_POINT('Ctrl Pts',(32.2875531747034,-14.7669045795448,-47.3306936623373));
#19708=CARTESIAN_POINT('Ctrl Pts',(32.3040911700412,-14.766904560918,-47.3166798601742));
#19709=CARTESIAN_POINT('Ctrl Pts',(32.3196301239233,-14.7669044772679,-47.3016933745717));
#19710=CARTESIAN_POINT('Ctrl Pts',(32.3347692125982,-14.7669043957704,-47.2870925374637));
#19711=CARTESIAN_POINT('Ctrl Pts',(32.3489605420936,-14.7669042476547,-47.2715690661388));
#19712=CARTESIAN_POINT('Ctrl Pts',(32.3622379419634,-14.7669041441791,-47.255300171139));
#19713=CARTESIAN_POINT('Ctrl Pts',(32.3689643151124,-14.7669040917581,-47.2470582970099));
#19714=CARTESIAN_POINT('Ctrl Pts',(32.3754531347727,-14.7669040484303,-47.2386243425884));
#19715=CARTESIAN_POINT('Ctrl Pts',(32.3817058008036,-14.7669040210232,-47.2300205947939));
#19716=CARTESIAN_POINT('Ctrl Pts',(32.3840505505652,-14.7669040107455,-47.226794189371));
#19717=CARTESIAN_POINT('Ctrl Pts',(32.3863620912228,-14.7669040026344,-47.2235439067552));
#19718=CARTESIAN_POINT('Ctrl Pts',(32.3886404965979,-14.7669039967743,-47.220270922234));
#19719=CARTESIAN_POINT('Ctrl Pts',(32.390634101301,-14.7669039916468,-47.217407060778));
#19720=CARTESIAN_POINT('Ctrl Pts',(32.3926023368035,-14.7669039882399,-47.2145258181757));
#19721=CARTESIAN_POINT('Ctrl Pts',(32.3945452525602,-14.7669039865145,-47.2116279817781));
#19722=CARTESIAN_POINT('Ctrl Pts',(32.4081456628571,-14.7669039744365,-47.1913431269954));
#19723=CARTESIAN_POINT('Ctrl Pts',(32.4205054055829,-14.7669040526285,-47.1702451762436));
#19724=CARTESIAN_POINT('Ctrl Pts',(32.4316414440808,-14.7669041305354,-47.1486041910527));
#19725=CARTESIAN_POINT('Ctrl Pts',(32.4463626886987,-14.7669042335241,-47.1199959712781));
#19726=CARTESIAN_POINT('Ctrl Pts',(32.4590542802873,-14.7669043748298,-47.0903042649473));
#19727=CARTESIAN_POINT('Ctrl Pts',(32.4698771491973,-14.7669044578905,-47.0598955592365));
#19728=CARTESIAN_POINT('Ctrl Pts',(32.4742625549281,-14.7669044915466,-47.0475740099875));
#19729=CARTESIAN_POINT('Ctrl Pts',(32.4783405165562,-14.7669045170158,-47.0351346693419));
#19730=CARTESIAN_POINT('Ctrl Pts',(32.4821193826036,-14.7669045346655,-47.0226018965824));
#19731=CARTESIAN_POINT('Ctrl Pts',(32.4931992952929,-14.7669045864155,-46.9858548867149));
#19732=CARTESIAN_POINT('Ctrl Pts',(32.5017169636477,-14.7669045820527,-46.9483049513178));
#19733=CARTESIAN_POINT('Ctrl Pts',(32.5079293060509,-14.7669045822747,-46.9105654690864));
#19734=CARTESIAN_POINT('Ctrl Pts',(32.5090631880298,-14.7669045823153,-46.9036772269361));
#19735=CARTESIAN_POINT('Ctrl Pts',(32.5101201315568,-14.7669045823054,-46.8967826857539));
#19736=CARTESIAN_POINT('Ctrl Pts',(32.5111015211428,-14.7669045823054,-46.8898856260792));
#19737=CARTESIAN_POINT('Ctrl Pts',(32.5111027879795,-14.7669045823054,-46.8898767229402));
#19738=CARTESIAN_POINT('Ctrl Pts',(32.511104054695,-14.7669045823054,-46.8898678197768));
#19739=CARTESIAN_POINT('Ctrl Pts',(32.5111053212894,-14.7669045823054,-46.889858916589));
#19740=CARTESIAN_POINT('Ctrl Pts',(32.5142844731562,-14.7669045823054,-46.8675119167502));
#19741=CARTESIAN_POINT('Ctrl Pts',(32.5166905301417,-14.7669045826373,-46.8449996927378));
#19742=CARTESIAN_POINT('Ctrl Pts',(32.5183630494517,-14.7669045772469,-46.8224057278094));
#19743=CARTESIAN_POINT('Ctrl Pts',(32.5208718284167,-14.7669045691613,-46.7885147804168));
#19744=CARTESIAN_POINT('Ctrl Pts',(32.5217301481929,-14.766904546284,-46.7544399152559));
#19745=CARTESIAN_POINT('Ctrl Pts',(32.5210714668687,-14.7669045319054,-46.7204628780165));
#19746=CARTESIAN_POINT('Ctrl Pts',(32.5204127855445,-14.7669045175269,-46.6864858407771));
#19747=CARTESIAN_POINT('Ctrl Pts',(32.5182371031102,-14.7669045165844,-46.6526066314599));
#19748=CARTESIAN_POINT('Ctrl Pts',(32.5146778776706,-14.7669045221653,-46.6191069957584));
#19749=CARTESIAN_POINT('Ctrl Pts',(32.5111794725999,-14.7669045276508,-46.5861798048872));
#19750=CARTESIAN_POINT('Ctrl Pts',(32.5063452043462,-14.766904544103,-46.553462859021));
#19751=CARTESIAN_POINT('Ctrl Pts',(32.5002291656841,-14.7669045570257,-46.5209360093445));
#19752=CARTESIAN_POINT('Ctrl Pts',(32.4940445072357,-14.7669045700934,-46.4880442199424));
#19753=CARTESIAN_POINT('Ctrl Pts',(32.4865486002504,-14.7669045784001,-46.4553458854947));
#19754=CARTESIAN_POINT('Ctrl Pts',(32.4777487169981,-14.7669045808678,-46.4228403401102));
#19755=CARTESIAN_POINT('Ctrl Pts',(32.4716414149088,-14.7669045825804,-46.4002808152224));
#19756=CARTESIAN_POINT('Ctrl Pts',(32.4649050132712,-14.7669045823054,-46.3778145456801));
#19757=CARTESIAN_POINT('Ctrl Pts',(32.4575305290195,-14.7669045823054,-46.3554507110304));
#19758=CARTESIAN_POINT('',(30.6299435607004,-14.7669045823054,-48.4165189096496));
#19759=CARTESIAN_POINT('Origin',(0.0835265683620477,-14.7669045823054,0.0824317919394229));
#19760=CARTESIAN_POINT('',(29.5568100599416,-14.7669045823054,-48.6675682080606));
#19761=CARTESIAN_POINT('Ctrl Pts',(29.5568100599416,-14.7669045823054,-48.6675682080606));
#19762=CARTESIAN_POINT('Ctrl Pts',(29.687226059415,-14.7669045823054,-48.6675682069665));
#19763=CARTESIAN_POINT('Ctrl Pts',(29.8164312767719,-14.7669045823175,-48.6592516832571));
#19764=CARTESIAN_POINT('Ctrl Pts',(29.9442057515289,-14.7669045822917,-48.6412585834828));
#19765=CARTESIAN_POINT('Ctrl Pts',(29.9988450488462,-14.7669045822807,-48.6335643211499));
#19766=CARTESIAN_POINT('Ctrl Pts',(30.0532227864462,-14.7669045822601,-48.6241012172608));
#19767=CARTESIAN_POINT('Ctrl Pts',(30.1073220850124,-14.7669045822063,-48.6127658445173));
#19768=CARTESIAN_POINT('Ctrl Pts',(30.1078450912829,-14.7669045822058,-48.6126562595285));
#19769=CARTESIAN_POINT('Ctrl Pts',(30.1083681026981,-14.7669045822053,-48.6125465072483));
#19770=CARTESIAN_POINT('Ctrl Pts',(30.1088911186622,-14.7669045822047,-48.6124365871634));
#19771=CARTESIAN_POINT('Ctrl Pts',(30.1758594224764,-14.7669045821373,-48.5983621379247));
#19772=CARTESIAN_POINT('Ctrl Pts',(30.2427679718073,-14.7669045821586,-48.5815717818007));
#19773=CARTESIAN_POINT('Ctrl Pts',(30.3085555596271,-14.7669045822031,-48.5609664254967));
#19774=CARTESIAN_POINT('Ctrl Pts',(30.3646336248817,-14.7669045822411,-48.5434021925814));
#19775=CARTESIAN_POINT('Ctrl Pts',(30.4198994743272,-14.766904582279,-48.5230669892512));
#19776=CARTESIAN_POINT('Ctrl Pts',(30.473690093401,-14.7669045822933,-48.4992416030476));
#19777=CARTESIAN_POINT('Ctrl Pts',(30.5206443189021,-14.7669045823058,-48.4784442488673));
#19778=CARTESIAN_POINT('Ctrl Pts',(30.5664751505883,-14.7669045823054,-48.454987627778));
#19779=CARTESIAN_POINT('Ctrl Pts',(30.6107202044109,-14.7669045823054,-48.4283554531363));
#19780=CARTESIAN_POINT('Ctrl Pts',(30.6171621507609,-14.7669045823054,-48.4244778888573));
#19781=CARTESIAN_POINT('Ctrl Pts',(30.6235704304707,-14.7669045823054,-48.4205329323747));
#19782=CARTESIAN_POINT('Ctrl Pts',(30.6299435607004,-14.7669045823054,-48.4165189096496));
#19783=CARTESIAN_POINT('',(-29.3897569232175,-14.7669045823054,-48.6675682080606));
#19784=CARTESIAN_POINT('',(-30.3174396991762,-14.7669045823054,-48.6675682080606));
#19785=CARTESIAN_POINT('Ctrl Pts',(-30.4628904239763,-14.7669045823054,
-48.4165189096496));
#19786=CARTESIAN_POINT('Ctrl Pts',(-30.383617379776,-14.7669045823054,-48.4664479788226));
#19787=CARTESIAN_POINT('Ctrl Pts',(-30.2980162042778,-14.7669045823054,
-48.5052983546113));
#19788=CARTESIAN_POINT('Ctrl Pts',(-30.1231196682765,-14.7669045823054,
-48.568676241689));
#19789=CARTESIAN_POINT('Ctrl Pts',(-30.0339383600361,-14.7669045823054,
-48.5930128390463));
#19790=CARTESIAN_POINT('Ctrl Pts',(-29.7626759270632,-14.7669045823054,
-48.6502470251504));
#19791=CARTESIAN_POINT('Ctrl Pts',(-29.5761319200258,-14.7669045823054,
-48.6675682080606));
#19792=CARTESIAN_POINT('Ctrl Pts',(-29.3897569232175,-14.7669045823054,
-48.6675682080606));
#19793=CARTESIAN_POINT('',(-20.394360840366,-14.7669045823054,-6.6701627853663));
#19794=CARTESIAN_POINT('',(-9.75726988530523,-14.7669045823054,-19.1035039790228));
#19795=CARTESIAN_POINT('Origin',(0.0835265683620477,-14.7669045823054,0.0824317919394229));
#19796=CARTESIAN_POINT('',(-9.84678298317079,-14.7669045823054,-20.2531800132168));
#19797=CARTESIAN_POINT('Origin',(-10.0425103622231,-14.7669045823054,-19.6596180593406));
#19798=CARTESIAN_POINT('',(-46.3543559346078,-14.7669045823054,-32.2915721687179));
#19799=CARTESIAN_POINT('',(-48.0630165107499,-14.7669045823054,-32.8550039285778));
#19800=CARTESIAN_POINT('',(-47.352376130838,-14.7669045823054,-32.090024523005));
#19801=CARTESIAN_POINT('Ctrl Pts',(-47.352376130838,-14.7669045823054,-32.090024523005));
#19802=CARTESIAN_POINT('Ctrl Pts',(-47.3491535505513,-14.7669045823054,
-32.0947759639391));
#19803=CARTESIAN_POINT('Ctrl Pts',(-47.3458476093404,-14.7669045824339,
-32.0994580383575));
#19804=CARTESIAN_POINT('Ctrl Pts',(-47.3424616674655,-14.7669045818319,
-32.1040709445545));
#19805=CARTESIAN_POINT('Ctrl Pts',(-47.3295988859157,-14.7669045795448,
-32.1215948144007));
#19806=CARTESIAN_POINT('Ctrl Pts',(-47.3155850837535,-14.766904560918,-32.1381328097375));
#19807=CARTESIAN_POINT('Ctrl Pts',(-47.300598598152,-14.7669044772679,-32.1536717636188));
#19808=CARTESIAN_POINT('Ctrl Pts',(-47.2859977610431,-14.7669043957704,
-32.1688108522948));
#19809=CARTESIAN_POINT('Ctrl Pts',(-47.2704742897173,-14.7669042476547,
-32.1830021817911));
#19810=CARTESIAN_POINT('Ctrl Pts',(-47.2542053947165,-14.7669041441791,
-32.1962795816618));
#19811=CARTESIAN_POINT('Ctrl Pts',(-47.2459635205874,-14.7669040917581,
-32.2030059548108));
#19812=CARTESIAN_POINT('Ctrl Pts',(-47.2375295661659,-14.7669040484303,
-32.2094947744711));
#19813=CARTESIAN_POINT('Ctrl Pts',(-47.2289258183714,-14.7669040210232,
-32.215747440502));
#19814=CARTESIAN_POINT('Ctrl Pts',(-47.2256994129485,-14.7669040107455,
-32.2180921902636));
#19815=CARTESIAN_POINT('Ctrl Pts',(-47.2224491303327,-14.7669040026344,
-32.2204037309212));
#19816=CARTESIAN_POINT('Ctrl Pts',(-47.2191761458115,-14.7669039967743,
-32.2226821362962));
#19817=CARTESIAN_POINT('Ctrl Pts',(-47.2163122843555,-14.7669039916467,
-32.2246757409994));
#19818=CARTESIAN_POINT('Ctrl Pts',(-47.2134310417532,-14.7669039882399,
-32.2266439765019));
#19819=CARTESIAN_POINT('Ctrl Pts',(-47.2105332053557,-14.7669039865145,
-32.2285868922586));
#19820=CARTESIAN_POINT('Ctrl Pts',(-47.190248350573,-14.7669039744365,-32.2421873025555));
#19821=CARTESIAN_POINT('Ctrl Pts',(-47.1691503998211,-14.7669040526285,
-32.2545470452812));
#19822=CARTESIAN_POINT('Ctrl Pts',(-47.1475094146302,-14.7669041305354,
-32.2656830837792));
#19823=CARTESIAN_POINT('Ctrl Pts',(-47.1189011948645,-14.7669042335241,
-32.2804043283925));
#19824=CARTESIAN_POINT('Ctrl Pts',(-47.0892094885433,-14.7669043748298,
-32.2930959199778));
#19825=CARTESIAN_POINT('Ctrl Pts',(-47.0588007828424,-14.7669044578905,
-32.3039187888855));
#19826=CARTESIAN_POINT('Ctrl Pts',(-47.0464792335841,-14.7669044915466,
-32.3083041946202));
#19827=CARTESIAN_POINT('Ctrl Pts',(-47.034039892929,-14.7669045170158,-32.3123821562517));
#19828=CARTESIAN_POINT('Ctrl Pts',(-47.0215071201599,-14.7669045346655,
-32.3161610223019));
#19829=CARTESIAN_POINT('Ctrl Pts',(-46.984760110287,-14.7669045864155,-32.3272409349929));
#19830=CARTESIAN_POINT('Ctrl Pts',(-46.9472101748842,-14.7669045820527,
-32.3357586033484));
#19831=CARTESIAN_POINT('Ctrl Pts',(-46.9094706926473,-14.7669045822747,
-32.3419709457519));
#19832=CARTESIAN_POINT('Ctrl Pts',(-46.9025824505025,-14.7669045823153,
-32.3431048277297));
#19833=CARTESIAN_POINT('Ctrl Pts',(-46.8956879093258,-14.7669045823054,
-32.3441617712558));
#19834=CARTESIAN_POINT('Ctrl Pts',(-46.8887908496566,-14.7669045823054,
-32.3451431608411));
#19835=CARTESIAN_POINT('Ctrl Pts',(-46.8887819465176,-14.7669045823054,
-32.3451444276778));
#19836=CARTESIAN_POINT('Ctrl Pts',(-46.8887730433543,-14.7669045823054,
-32.3451456943933));
#19837=CARTESIAN_POINT('Ctrl Pts',(-46.8887641401665,-14.7669045823054,
-32.3451469609878));
#19838=CARTESIAN_POINT('Ctrl Pts',(-46.8664171403277,-14.7669045823054,
-32.3483261128546));
#19839=CARTESIAN_POINT('Ctrl Pts',(-46.8439049163153,-14.7669045826373,
-32.3507321698401));
#19840=CARTESIAN_POINT('Ctrl Pts',(-46.8213109513869,-14.7669045772469,
-32.3524046891501));
#19841=CARTESIAN_POINT('Ctrl Pts',(-46.7874200039943,-14.7669045691613,
-32.3549134681151));
#19842=CARTESIAN_POINT('Ctrl Pts',(-46.7533451388334,-14.766904546284,-32.3557717878912));
#19843=CARTESIAN_POINT('Ctrl Pts',(-46.719368101594,-14.7669045319054,-32.355113106567));
#19844=CARTESIAN_POINT('Ctrl Pts',(-46.6853910643546,-14.7669045175269,
-32.3544544252428));
#19845=CARTESIAN_POINT('Ctrl Pts',(-46.6515118550373,-14.7669045165844,
-32.3522787428086));
#19846=CARTESIAN_POINT('Ctrl Pts',(-46.6180122193358,-14.7669045221653,
-32.348719517369));
#19847=CARTESIAN_POINT('Ctrl Pts',(-46.585085028464,-14.7669045276508,-32.3452211122982));
#19848=CARTESIAN_POINT('Ctrl Pts',(-46.5523680825972,-14.766904544103,-32.3403868440443));
#19849=CARTESIAN_POINT('Ctrl Pts',(-46.5198412329201,-14.7669045570257,
-32.334270805382));
#19850=CARTESIAN_POINT('Ctrl Pts',(-46.4869494435169,-14.7669045700934,
-32.3280861469334));
#19851=CARTESIAN_POINT('Ctrl Pts',(-46.4542511090682,-14.7669045784001,
-32.3205902399477));
#19852=CARTESIAN_POINT('Ctrl Pts',(-46.4217455636826,-14.7669045808678,
-32.311790356695));
#19853=CARTESIAN_POINT('Ctrl Pts',(-46.3991860387965,-14.7669045825804,
-32.305683054606));
#19854=CARTESIAN_POINT('Ctrl Pts',(-46.3767197692559,-14.7669045823054,
-32.298946652969));
#19855=CARTESIAN_POINT('Ctrl Pts',(-46.3543559346078,-14.7669045823054,
-32.2915721687179));
#19856=CARTESIAN_POINT('',(-48.415424133227,-14.7669045823054,-30.4639852003989));
#19857=CARTESIAN_POINT('Origin',(0.0835265683620477,-14.7669045823054,0.0824317919394229));
#19858=CARTESIAN_POINT('',(-48.6664734316379,-14.7669045823054,-29.3908516996402));
#19859=CARTESIAN_POINT('Ctrl Pts',(-48.6664734316379,-14.7669045823054,
-29.3908516996402));
#19860=CARTESIAN_POINT('Ctrl Pts',(-48.6664734305346,-14.7669045823054,
-29.5212452714537));
#19861=CARTESIAN_POINT('Ctrl Pts',(-48.658159503563,-14.7669045823177,-29.6504238593144));
#19862=CARTESIAN_POINT('Ctrl Pts',(-48.6401750099693,-14.7669045822915,
-29.778166914327));
#19863=CARTESIAN_POINT('Ctrl Pts',(-48.6324798641135,-14.7669045822804,
-29.8328251917631));
#19864=CARTESIAN_POINT('Ctrl Pts',(-48.6230148766798,-14.7669045822595,
-29.8872207222031));
#19865=CARTESIAN_POINT('Ctrl Pts',(-48.6116767039643,-14.7669045822049,
-29.9413365514922));
#19866=CARTESIAN_POINT('Ctrl Pts',(-48.6115666059104,-14.7669045822044,
-29.9418620371803));
#19867=CARTESIAN_POINT('Ctrl Pts',(-48.6114563389905,-14.7669045822038,
-29.9423875282861));
#19868=CARTESIAN_POINT('Ctrl Pts',(-48.6113459026832,-14.7669045822033,
-29.9429130242052));
#19869=CARTESIAN_POINT('Ctrl Pts',(-48.5971465642682,-14.7669045821343,
-30.0104786153631));
#19870=CARTESIAN_POINT('Ctrl Pts',(-48.5801820330883,-14.7669045821572,
-30.0779908271464));
#19871=CARTESIAN_POINT('Ctrl Pts',(-48.559321523009,-14.7669045822029,-30.1443546643599));
#19872=CARTESIAN_POINT('Ctrl Pts',(-48.5417918489716,-14.7669045822413,
-30.2001220655312));
#19873=CARTESIAN_POINT('Ctrl Pts',(-48.5215119330852,-14.7669045822791,
-30.2550807409539));
#19874=CARTESIAN_POINT('Ctrl Pts',(-48.4977739691264,-14.7669045822934,
-30.3085755625293));
#19875=CARTESIAN_POINT('Ctrl Pts',(-48.4767816374474,-14.766904582306,-30.3558829491095));
#19876=CARTESIAN_POINT('Ctrl Pts',(-48.4530851649729,-14.7669045823054,
-30.4020462550889));
#19877=CARTESIAN_POINT('Ctrl Pts',(-48.4261572648105,-14.7669045823054,
-30.4465911244048));
#19878=CARTESIAN_POINT('Ctrl Pts',(-48.4226353067432,-14.7669045823054,
-30.4524172438162));
#19879=CARTESIAN_POINT('Ctrl Pts',(-48.4190580087251,-14.7669045823054,
-30.4582156362162));
#19880=CARTESIAN_POINT('Ctrl Pts',(-48.415424133227,-14.7669045823054,-30.4639852003989));
#19881=CARTESIAN_POINT('',(-48.6664734316379,-14.7669045823054,29.555715283519));
#19882=CARTESIAN_POINT('',(-48.6664734316379,-14.7669045823054,30.4833980594772));
#19883=CARTESIAN_POINT('',(-48.415424133227,-14.7669045823054,30.6288487842778));
#19884=CARTESIAN_POINT('Ctrl Pts',(-48.415424133227,-14.7669045823054,30.6288487842778));
#19885=CARTESIAN_POINT('Ctrl Pts',(-48.4653532024,-14.7669045823054,30.5495757400775));
#19886=CARTESIAN_POINT('Ctrl Pts',(-48.5042035781887,-14.7669045823054,
30.4639745645792));
#19887=CARTESIAN_POINT('Ctrl Pts',(-48.5675814652663,-14.7669045823054,
30.2890780285779));
#19888=CARTESIAN_POINT('Ctrl Pts',(-48.5919180626237,-14.7669045823054,
30.1998967203376));
#19889=CARTESIAN_POINT('Ctrl Pts',(-48.6491522487277,-14.7669045823054,
29.9286342873647));
#19890=CARTESIAN_POINT('Ctrl Pts',(-48.666473431638,-14.7669045823054,29.7420902803272));
#19891=CARTESIAN_POINT('Ctrl Pts',(-48.6664734316379,-14.7669045823054,
29.555715283519));
#19892=CARTESIAN_POINT('',(-37.6790715732587,-14.7669045823054,43.2010819542467));
#19893=CARTESIAN_POINT('Origin',(0.0835265683620477,-14.7669045823054,0.0824317919394229));
#19894=CARTESIAN_POINT('',(-36.6439262383654,-14.7669045823054,42.6081948668641));
#19895=CARTESIAN_POINT('Ctrl Pts',(-37.6790715732587,-14.7669045823054,
43.2010819542467));
#19896=CARTESIAN_POINT('Ctrl Pts',(-37.6627777835487,-14.7669045823054,
43.2153517848353));
#19897=CARTESIAN_POINT('Ctrl Pts',(-37.6455680600597,-14.7669045823054,
43.2284106239852));
#19898=CARTESIAN_POINT('Ctrl Pts',(-37.6275821014629,-14.7669045823054,
43.2401593818916));
#19899=CARTESIAN_POINT('Ctrl Pts',(-37.6098482742043,-14.7669045823054,
43.2517434429853));
#19900=CARTESIAN_POINT('Ctrl Pts',(-37.5913587176086,-14.7669045823054,
43.2620548305755));
#19901=CARTESIAN_POINT('Ctrl Pts',(-37.5722121171962,-14.7669045823054,
43.2709645071072));
#19902=CARTESIAN_POINT('Ctrl Pts',(-37.5576370725083,-14.7669045823054,
43.2777468564959));
#19903=CARTESIAN_POINT('Ctrl Pts',(-37.5426804759792,-14.7669045823054,
43.2837163812658));
#19904=CARTESIAN_POINT('Ctrl Pts',(-37.5273775591158,-14.7669045823054,
43.2887975366259));
#19905=CARTESIAN_POINT('Ctrl Pts',(-37.5273757146397,-14.7669045823054,
43.2887981490627));
#19906=CARTESIAN_POINT('Ctrl Pts',(-37.5273738701592,-14.7669045823054,
43.2887987614863));
#19907=CARTESIAN_POINT('Ctrl Pts',(-37.5273720256744,-14.7669045823054,
43.2887993738968));
#19908=CARTESIAN_POINT('Ctrl Pts',(-37.4715793276776,-14.7669045823054,
43.3073238062995));
#19909=CARTESIAN_POINT('Ctrl Pts',(-37.4120115906116,-14.7669045823054,
43.313801976715));
#19910=CARTESIAN_POINT('Ctrl Pts',(-37.3535343859751,-14.7669045823054,
43.309219604822));
#19911=CARTESIAN_POINT('Ctrl Pts',(-37.3535305195056,-14.7669045823054,
43.309219301839));
#19912=CARTESIAN_POINT('Ctrl Pts',(-37.3535266530408,-14.7669045823054,
43.3092189988076));
#19913=CARTESIAN_POINT('Ctrl Pts',(-37.3535227865809,-14.7669045823054,
43.3092186957278));
#19914=CARTESIAN_POINT('Ctrl Pts',(-37.2365686658092,-14.7669045823054,
43.3000510267261));
#19915=CARTESIAN_POINT('Ctrl Pts',(-37.1255044840321,-14.7669045823054,
43.2482414553837));
#19916=CARTESIAN_POINT('Ctrl Pts',(-37.0318179550061,-14.7669045823054,
43.1781038425302));
#19917=CARTESIAN_POINT('Ctrl Pts',(-37.0318117605224,-14.7669045823054,
43.1780992050834));
#19918=CARTESIAN_POINT('Ctrl Pts',(-37.0318055661156,-14.7669045823054,
43.1780945675506));
#19919=CARTESIAN_POINT('Ctrl Pts',(-37.0317993717856,-14.7669045823054,
43.1780899299318));
#19920=CARTESIAN_POINT('Ctrl Pts',(-37.020094653455,-14.7669045823054,43.1693267509767));
#19921=CARTESIAN_POINT('Ctrl Pts',(-37.0086245945463,-14.7669045833006,
43.160270378826));
#19922=CARTESIAN_POINT('Ctrl Pts',(-36.9973879816216,-14.7669045783028,
43.1509415772979));
#19923=CARTESIAN_POINT('Ctrl Pts',(-36.9704488983943,-14.7669045663207,
43.1285763536794));
#19924=CARTESIAN_POINT('Ctrl Pts',(-36.9448465063951,-14.766904502036,43.1046461982809));
#19925=CARTESIAN_POINT('Ctrl Pts',(-36.9205742577055,-14.7669043153494,
43.0794356615139));
#19926=CARTESIAN_POINT('Ctrl Pts',(-36.9093928981769,-14.7669042293495,
43.0678220661234));
#19927=CARTESIAN_POINT('Ctrl Pts',(-36.8984930719822,-14.766904120834,43.0559369352108));
#19928=CARTESIAN_POINT('Ctrl Pts',(-36.8878705135893,-14.7669040086953,
43.043808629559));
#19929=CARTESIAN_POINT('Ctrl Pts',(-36.8710296266393,-14.7669038309118,
43.0245805475074));
#19930=CARTESIAN_POINT('Ctrl Pts',(-36.8548899801924,-14.7669036396173,
43.0047405991125));
#19931=CARTESIAN_POINT('Ctrl Pts',(-36.8394444170864,-14.7669035207875,
42.9844004276988));
#19932=CARTESIAN_POINT('Ctrl Pts',(-36.8317216355334,-14.7669034613726,
42.9742303419919));
#19933=CARTESIAN_POINT('Ctrl Pts',(-36.824172374821,-14.7669034201738,42.9639352005286));
#19934=CARTESIAN_POINT('Ctrl Pts',(-36.8167957403039,-14.7669034045806,
42.9535289587375));
#19935=CARTESIAN_POINT('Ctrl Pts',(-36.8094191057869,-14.7669033889875,
42.9431227169463));
#19936=CARTESIAN_POINT('Ctrl Pts',(-36.8022150974665,-14.7669033991487,
42.9326053748268));
#19937=CARTESIAN_POINT('Ctrl Pts',(-36.7951828206651,-14.7669034367692,
42.9219908878338));
#19938=CARTESIAN_POINT('Ctrl Pts',(-36.7769301982716,-14.766903534415,42.8944404616412));
#19939=CARTESIAN_POINT('Ctrl Pts',(-36.7598249398862,-14.7669038199043,
42.8662332283621));
#19940=CARTESIAN_POINT('Ctrl Pts',(-36.7438303418086,-14.7669040506412,
42.8374123849365));
#19941=CARTESIAN_POINT('Ctrl Pts',(-36.7316543489533,-14.7669042262912,
42.8154723285542));
#19942=CARTESIAN_POINT('Ctrl Pts',(-36.7201231614195,-14.7669043666507,
42.793176123329));
#19943=CARTESIAN_POINT('Ctrl Pts',(-36.7092404677718,-14.766904445574,42.770539858458));
#19944=CARTESIAN_POINT('Ctrl Pts',(-36.6935378630025,-14.7669045594521,
42.7378780623783));
#19945=CARTESIAN_POINT('Ctrl Pts',(-36.6791792700311,-14.7669045735796,
42.7045103513217));
#19946=CARTESIAN_POINT('Ctrl Pts',(-36.6661264061134,-14.7669045795915,
42.6704888195698));
#19947=CARTESIAN_POINT('Ctrl Pts',(-36.6582496141909,-14.7669045832193,
42.6499584188713));
#19948=CARTESIAN_POINT('Ctrl Pts',(-36.6508492987573,-14.7669045823054,
42.629189708122));
#19949=CARTESIAN_POINT('Ctrl Pts',(-36.6439262383654,-14.7669045823054,
42.6081948668641));
#19950=CARTESIAN_POINT('',(-20.3943608403659,-14.7669045823054,-6.67016278536651));
#19951=CARTESIAN_POINT('Origin',(-44.291473431638,16.4830954176946,-44.2925682080606));
#19952=CARTESIAN_POINT('Origin',(-44.291473431638,13.4386401876617,-44.2925682080606));
#19953=CARTESIAN_POINT('Origin',(-44.291473431638,16.1705954176946,-44.2925682080606));
#19954=CARTESIAN_POINT('Origin',(0.0835265683620477,16.4830954176946,0.0824317919394229));
#19955=CARTESIAN_POINT('',(-48.2416470424902,16.3915662868154,-22.5111558702776));
#19956=CARTESIAN_POINT('',(-48.2616069551277,11.5746245485739,-4.13831849464094));
#19957=CARTESIAN_POINT('Ctrl Pts',(-48.2416470424886,16.3915662868154,-22.5111558702765));
#19958=CARTESIAN_POINT('Ctrl Pts',(-48.2463095265271,15.1541680928392,-19.5795487103057));
#19959=CARTESIAN_POINT('Ctrl Pts',(-48.2506569957559,14.0894359483377,-16.5909382447155));
#19960=CARTESIAN_POINT('Ctrl Pts',(-48.2559385859013,12.8480220597894,-11.9905975010272));
#19961=CARTESIAN_POINT('Ctrl Pts',(-48.2574906537671,12.4934998941785,-10.4347915160951));
#19962=CARTESIAN_POINT('Ctrl Pts',(-48.2600106799664,11.9258476364963,-7.30351014927071));
#19963=CARTESIAN_POINT('Ctrl Pts',(-48.2609809492583,11.7120008366799,-5.72500374474883));
#19964=CARTESIAN_POINT('Ctrl Pts',(-48.2616069550931,11.5746245485739,-4.13831849503741));
#19965=CARTESIAN_POINT('',(-4.13722371775065,11.5746245485364,-48.2627017315536));
#19966=CARTESIAN_POINT('Origin',(0.0835265683620477,11.5746245485738,0.0824317919394229));
#19967=CARTESIAN_POINT('',(-22.5100610938543,16.3915662868156,-48.2427418189112));
#19968=CARTESIAN_POINT('Ctrl Pts',(-4.13722371861476,11.5746245485739,-48.2627017315157));
#19969=CARTESIAN_POINT('Ctrl Pts',(-5.72250617307994,11.7118793817134,-48.2620762791354));
#19970=CARTESIAN_POINT('Ctrl Pts',(-7.29569335888353,11.9249456441311,-48.2611095568614));
#19971=CARTESIAN_POINT('Ctrl Pts',(-10.419797403947,12.4906656417943,-48.2585979169746));
#19972=CARTESIAN_POINT('Ctrl Pts',(-11.9729836285199,12.843980457976,-48.2570508371642));
#19973=CARTESIAN_POINT('Ctrl Pts',(-16.5789073885739,14.0856585112706,-48.2517672875344));
#19974=CARTESIAN_POINT('Ctrl Pts',(-19.5792793614228,15.1545164964592,-48.247402990174));
#19975=CARTESIAN_POINT('Ctrl Pts',(-22.5100610938539,16.3915662868154,-48.2427418189112));
#19976=CARTESIAN_POINT('Origin',(0.0835265683620477,16.3915662868154,0.0824317919394229));
#19977=CARTESIAN_POINT('Origin',(0.083526568362047,-85.4775827009602,-48.3550682080606));
#19978=CARTESIAN_POINT('',(4.28505819640515,11.7955954176946,-48.3550682080606));
#19979=CARTESIAN_POINT('',(0.0835265683620996,11.6131136241746,-48.3550682080606));
#19980=CARTESIAN_POINT('Origin',(0.0819794847533267,84.3502669982689,-48.3550682080606));
#19981=CARTESIAN_POINT('',(21.5192635553992,16.1706033824536,-48.3550682079476));
#19982=CARTESIAN_POINT('Ctrl Pts',(4.28505819640516,11.7955954176946,-48.3550682080605));
#19983=CARTESIAN_POINT('Ctrl Pts',(5.50013823173107,11.9012754508552,-48.3550682080566));
#19984=CARTESIAN_POINT('Ctrl Pts',(6.70990241723394,12.0520583728992,-48.3550682079193));
#19985=CARTESIAN_POINT('Ctrl Pts',(7.91463518434723,12.2455340352926,-48.3550682079632));
#19986=CARTESIAN_POINT('Ctrl Pts',(8.17547622965408,12.2874241501776,-48.3550682079727));
#19987=CARTESIAN_POINT('Ctrl Pts',(8.43608138895782,12.3313158147402,-48.3550682079893));
#19988=CARTESIAN_POINT('Ctrl Pts',(8.69645351250441,12.3771848834522,-48.3550682080079));
#19989=CARTESIAN_POINT('Ctrl Pts',(8.7750191265218,12.3910255799857,-48.3550682080135));
#19990=CARTESIAN_POINT('Ctrl Pts',(8.85355914623864,12.4050450140608,-48.3550682080107));
#19991=CARTESIAN_POINT('Ctrl Pts',(8.93207474413674,12.4192427232394,-48.3550682079984));
#19992=CARTESIAN_POINT('Ctrl Pts',(9.48447684182607,12.5191317203639,-48.3550682079116));
#19993=CARTESIAN_POINT('Ctrl Pts',(10.0363845144415,12.6280707956085,-48.3550682070548));
#19994=CARTESIAN_POINT('Ctrl Pts',(10.5869585665338,12.7454889373936,-48.3550682017512));
#19995=CARTESIAN_POINT('Ctrl Pts',(11.1518287905254,12.8659559514106,-48.35506819631));
#19996=CARTESIAN_POINT('Ctrl Pts',(11.7152965319533,12.9953485173926,-48.3550681859822));
#19997=CARTESIAN_POINT('Ctrl Pts',(12.2764461842882,13.1331031832615,-48.355068184015));
#19998=CARTESIAN_POINT('Ctrl Pts',(12.5381803751669,13.1973553945227,-48.3550681830974));
#19999=CARTESIAN_POINT('Ctrl Pts',(12.7994100068431,13.2634275010368,-48.3550681842804));
#20000=CARTESIAN_POINT('Ctrl Pts',(13.0600402582532,13.3312657045531,-48.3550681878717));
#20001=CARTESIAN_POINT('Ctrl Pts',(13.2556797364647,13.3821877700729,-48.3550681905676));
#20002=CARTESIAN_POINT('Ctrl Pts',(13.4510063934693,13.434106757518,-48.3550681928176));
#20003=CARTESIAN_POINT('Ctrl Pts',(13.645959769717,13.4869947668889,-48.3550681947288));
#20004=CARTESIAN_POINT('Ctrl Pts',(14.4497762714823,13.7050584675342,-48.3550682026087));
#20005=CARTESIAN_POINT('Ctrl Pts',(15.2484412867238,13.9395350034004,-48.3550682050813));
#20006=CARTESIAN_POINT('Ctrl Pts',(16.0422501539207,14.189298282416,-48.3550682064483));
#20007=CARTESIAN_POINT('Ctrl Pts',(16.8503556614315,14.4435598429592,-48.3550682078398));
#20008=CARTESIAN_POINT('Ctrl Pts',(17.6534285697549,14.7136635664416,-48.3550682079255));
#20009=CARTESIAN_POINT('Ctrl Pts',(18.4518008809203,14.9983707526325,-48.3550682080074));
#20010=CARTESIAN_POINT('Ctrl Pts',(19.2740592777951,15.2915959449672,-48.3550682080917));
#20011=CARTESIAN_POINT('Ctrl Pts',(20.0913316502591,15.600311376789,-48.3550682080606));
#20012=CARTESIAN_POINT('Ctrl Pts',(20.9040014843348,15.9231126709103,-48.3550682080606));
#20013=CARTESIAN_POINT('Ctrl Pts',(21.1093767204212,16.0046899476952,-48.3550682080606));
#20014=CARTESIAN_POINT('Ctrl Pts',(21.3144581104562,16.0871665859146,-48.3550682080606));
#20015=CARTESIAN_POINT('Ctrl Pts',(21.5192520383888,16.1705194395555,-48.3550682080606));
#20016=CARTESIAN_POINT('',(-21.3522103060312,16.1706033612892,-48.3550682079475));
#20017=CARTESIAN_POINT('',(0.083526568362047,16.1705954176946,-48.3550682080606));
#20018=CARTESIAN_POINT('',(-4.11800505968095,11.7955954176946,-48.3550682080606));
#20019=CARTESIAN_POINT('Ctrl Pts',(-21.3521988196773,16.1705196413539,-48.3550682080606));
#20020=CARTESIAN_POINT('Ctrl Pts',(-20.5487763954986,15.8435202228695,-48.3550682080606));
#20021=CARTESIAN_POINT('Ctrl Pts',(-19.7409251344067,15.5300086687594,-48.3550682080737));
#20022=CARTESIAN_POINT('Ctrl Pts',(-18.9282733738634,15.231367963779,-48.3550682080473));
#20023=CARTESIAN_POINT('Ctrl Pts',(-18.1328568981362,14.939061038971,-48.3550682080215));
#20024=CARTESIAN_POINT('Ctrl Pts',(-17.3328413075813,14.6610010609439,-48.3550682080443));
#20025=CARTESIAN_POINT('Ctrl Pts',(-16.5278966912028,14.3984390234986,-48.3550682072886));
#20026=CARTESIAN_POINT('Ctrl Pts',(-15.7437545768866,14.1426624806255,-48.3550682065524));
#20027=CARTESIAN_POINT('Ctrl Pts',(-14.9549348814219,13.9015932988569,-48.3550682052102));
#20028=CARTESIAN_POINT('Ctrl Pts',(-14.1611512443295,13.6763418789407,-48.3550682001227));
#20029=CARTESIAN_POINT('Ctrl Pts',(-13.9342291332018,13.6119483523507,-48.3550681986684));
#20030=CARTESIAN_POINT('Ctrl Pts',(-13.7069014694831,13.5488472154603,-48.3550681968855));
#20031=CARTESIAN_POINT('Ctrl Pts',(-13.4791618560963,13.4870636734958,-48.3550681946374));
#20032=CARTESIAN_POINT('Ctrl Pts',(-13.284209997429,13.4341751304712,-48.355068192713));
#20033=CARTESIAN_POINT('Ctrl Pts',(-13.0888824669268,13.3822549873819,-48.3550681904474));
#20034=CARTESIAN_POINT('Ctrl Pts',(-12.8932400676278,13.3313312754885,-48.3550681877328));
#20035=CARTESIAN_POINT('Ctrl Pts',(-12.3335737655675,13.1856558716668,-48.3550681799675));
#20036=CARTESIAN_POINT('Ctrl Pts',(-11.7711216017144,13.0481153497989,-48.3550681851995));
#20037=CARTESIAN_POINT('Ctrl Pts',(-11.2068238023173,12.9192577967038,-48.3550681923975));
#20038=CARTESIAN_POINT('Ctrl Pts',(-10.6541153068945,12.7930466642643,-48.3550681994477));
#20039=CARTESIAN_POINT('Ctrl Pts',(-10.0996349288977,12.6751650327118,-48.3550682055201));
#20040=CARTESIAN_POINT('Ctrl Pts',(-9.54424878778532,12.5661734818932,-48.3550682070987));
#20041=CARTESIAN_POINT('Ctrl Pts',(-9.28473868838682,12.5152460170309,-48.3550682078364));
#20042=CARTESIAN_POINT('Ctrl Pts',(-9.02503069905943,12.4662602454808,-48.355068207957));
#20043=CARTESIAN_POINT('Ctrl Pts',(-8.76521301459484,12.4192773203262,-48.3550682079981));
#20044=CARTESIAN_POINT('Ctrl Pts',(-8.68668667654382,12.405077374426,-48.3550682080105));
#20045=CARTESIAN_POINT('Ctrl Pts',(-8.6081361458596,12.3910557938695,-48.3550682080133));
#20046=CARTESIAN_POINT('Ctrl Pts',(-8.52956025973485,12.3772130393319,-48.3550682080077));
#20047=CARTESIAN_POINT('Ctrl Pts',(-7.3298348698903,12.1658567963019,-48.3550682079214));
#20048=CARTESIAN_POINT('Ctrl Pts',(-6.12517728947009,11.9964818480142,-48.3550682079949));
#20049=CARTESIAN_POINT('Ctrl Pts',(-4.91530765780725,11.8714667031496,-48.3550682080425));
#20050=CARTESIAN_POINT('Ctrl Pts',(-4.64979216840663,11.8440311377774,-48.355068208053));
#20051=CARTESIAN_POINT('Ctrl Pts',(-4.38402563457531,11.8187322172129,-48.3550682080596));
#20052=CARTESIAN_POINT('Ctrl Pts',(-4.11800505968097,11.7955954176945,-48.3550682080605));
#20053=CARTESIAN_POINT('Origin',(0.0850736592996893,84.3502670004067,-48.3550682139743));
#20054=CARTESIAN_POINT('Origin',(-48.3539734316379,-85.4775827009602,-44.2925682080605));
#20055=CARTESIAN_POINT('',(-48.3539734316379,-6.32940458230554,4.28396341998237));
#20056=CARTESIAN_POINT('',(-48.3539734316379,-6.14692278878557,0.0824317919393188));
#20057=CARTESIAN_POINT('Origin',(-48.3539734376932,-78.8840761710573,0.0808847054354922));
#20058=CARTESIAN_POINT('',(-48.3539734316292,-14.4544067125518,29.5557245537287));
#20059=CARTESIAN_POINT('Ctrl Pts',(-48.3539734316348,-6.32940458230555,
4.28396341998237));
#20060=CARTESIAN_POINT('Ctrl Pts',(-48.3539734314083,-6.60009088520904,
7.39624028683883));
#20061=CARTESIAN_POINT('Ctrl Pts',(-48.3539734245018,-7.165487581754,10.4492205117651));
#20062=CARTESIAN_POINT('Ctrl Pts',(-48.3539734271436,-7.96970388346465,
13.454151014626));
#20063=CARTESIAN_POINT('Ctrl Pts',(-48.3539734282648,-8.31099932795918,
14.729391381512));
#20064=CARTESIAN_POINT('Ctrl Pts',(-48.3539734303379,-8.695305697332,15.9959779893149));
#20065=CARTESIAN_POINT('Ctrl Pts',(-48.3539734312518,-9.11834864237836,
17.2547710529606));
#20066=CARTESIAN_POINT('Ctrl Pts',(-48.3539734313703,-9.17316448001786,
17.4178793071142));
#20067=CARTESIAN_POINT('Ctrl Pts',(-48.353973431397,-9.22862227451118,17.5808367859632));
#20068=CARTESIAN_POINT('Ctrl Pts',(-48.3539734313916,-9.28471651645581,
17.74365610972));
#20069=CARTESIAN_POINT('Ctrl Pts',(-48.3539734313723,-9.48472234839191,
18.3241936689119));
#20070=CARTESIAN_POINT('Ctrl Pts',(-48.3539734305475,-9.69311870415955,
18.9037446387506));
#20071=CARTESIAN_POINT('Ctrl Pts',(-48.353973430177,-9.90895820813048,19.4810918986109));
#20072=CARTESIAN_POINT('Ctrl Pts',(-48.3539734299785,-10.0245908848806,
19.7903967656244));
#20073=CARTESIAN_POINT('Ctrl Pts',(-48.3539734301286,-10.1423607380477,
20.0990689006501));
#20074=CARTESIAN_POINT('Ctrl Pts',(-48.3539734306861,-10.2621272193483,
20.4069177749615));
#20075=CARTESIAN_POINT('Ctrl Pts',(-48.353973431074,-10.3454600297986,20.6211172038148));
#20076=CARTESIAN_POINT('Ctrl Pts',(-48.3539734312712,-10.4297627624244,
20.8349374125696));
#20077=CARTESIAN_POINT('Ctrl Pts',(-48.3539734313944,-10.5149781806565,
21.0482886973521));
#20078=CARTESIAN_POINT('Ctrl Pts',(-48.3539734318711,-10.8449565878889,
21.8744457308332));
#20079=CARTESIAN_POINT('Ctrl Pts',(-48.3539734316591,-11.188740579391,22.6942362972106));
#20080=CARTESIAN_POINT('Ctrl Pts',(-48.3539734316028,-11.5450903892488,
23.5084157089998));
#20081=CARTESIAN_POINT('Ctrl Pts',(-48.353973431585,-11.6579509129727,23.7662766991778));
#20082=CARTESIAN_POINT('Ctrl Pts',(-48.3539734315666,-11.7720687209441,
24.0235665829017));
#20083=CARTESIAN_POINT('Ctrl Pts',(-48.3539734315544,-11.8874012527356,
24.280305717357));
#20084=CARTESIAN_POINT('Ctrl Pts',(-48.353973431512,-12.2879313738287,25.1719167399829));
#20085=CARTESIAN_POINT('Ctrl Pts',(-48.3539734315605,-12.7030439005446,
26.0569236215327));
#20086=CARTESIAN_POINT('Ctrl Pts',(-48.3539734315972,-13.1313454185141,
26.9359487176993));
#20087=CARTESIAN_POINT('Ctrl Pts',(-48.3539734316338,-13.5596469364837,
27.8149738138659));
#20088=CARTESIAN_POINT('Ctrl Pts',(-48.3539734316379,-14.001137100463,28.6880173360691));
#20089=CARTESIAN_POINT('Ctrl Pts',(-48.3539734316379,-14.4543739218735,
29.5557312928386));
#20090=CARTESIAN_POINT('',(-48.3539734316379,-14.4544045823054,-29.3908631559322));
#20091=CARTESIAN_POINT('',(-48.3539734316379,-14.4544045823054,-30.3185344755988));
#20092=CARTESIAN_POINT('',(-48.3539734316379,-6.32940458230556,-4.11909983610373));
#20093=CARTESIAN_POINT('Ctrl Pts',(-48.3539734316379,-14.4543736123986,
-29.3908678705539));
#20094=CARTESIAN_POINT('Ctrl Pts',(-48.3539734316379,-14.0009603589249,
-28.5228172256933));
#20095=CARTESIAN_POINT('Ctrl Pts',(-48.3539734316337,-13.5592886344727,
-27.6494060064744));
#20096=CARTESIAN_POINT('Ctrl Pts',(-48.3539734315961,-13.1308037218344,
-26.7699764159717));
#20097=CARTESIAN_POINT('Ctrl Pts',(-48.3539734315586,-12.7023188091961,
-25.890546825469));
#20098=CARTESIAN_POINT('Ctrl Pts',(-48.3539734315088,-12.2870210611745,
-25.0050986454736));
#20099=CARTESIAN_POINT('Ctrl Pts',(-48.3539734315522,-11.8863062114336,
-24.1130046264528));
#20100=CARTESIAN_POINT('Ctrl Pts',(-48.3539734315648,-11.7707122689893,
-23.8556628664549));
#20101=CARTESIAN_POINT('Ctrl Pts',(-48.3539734315836,-11.6563375248576,
-23.5977648578349));
#20102=CARTESIAN_POINT('Ctrl Pts',(-48.3539734316019,-11.5432249100059,
-23.3392899164854));
#20103=CARTESIAN_POINT('Ctrl Pts',(-48.3539734316532,-11.2263851142924,
-22.6152756434389));
#20104=CARTESIAN_POINT('Ctrl Pts',(-48.3539734317118,-10.9195690676833,
-21.8870351496141));
#20105=CARTESIAN_POINT('Ctrl Pts',(-48.3539734315538,-10.6234156307627,
-21.1534577234119));
#20106=CARTESIAN_POINT('Ctrl Pts',(-48.3539734315341,-10.5864935786647,
-21.0620011317553));
#20107=CARTESIAN_POINT('Ctrl Pts',(-48.3539734315083,-10.5497373137513,
-20.9704615520097));
#20108=CARTESIAN_POINT('Ctrl Pts',(-48.3539734314726,-10.5131481250882,
-20.8788368000147));
#20109=CARTESIAN_POINT('Ctrl Pts',(-48.353973431389,-10.4276256561533,-20.6646758608825));
#20110=CARTESIAN_POINT('Ctrl Pts',(-48.3539734312548,-10.3430386875929,
-20.4500850053422));
#20111=CARTESIAN_POINT('Ctrl Pts',(-48.3539734309901,-10.2594333452065,
-20.235123917639));
#20112=CARTESIAN_POINT('Ctrl Pts',(-48.3539734303323,-10.051669996851,-19.7009351436613));
#20113=CARTESIAN_POINT('Ctrl Pts',(-48.3539734307198,-9.85012639371284,
-19.1648181410921));
#20114=CARTESIAN_POINT('Ctrl Pts',(-48.3539734310814,-9.65537647176604,
-18.627378781688));
#20115=CARTESIAN_POINT('Ctrl Pts',(-48.3539734313171,-9.52849547986369,
-18.2772331265478));
#20116=CARTESIAN_POINT('Ctrl Pts',(-48.3539734314598,-9.40449887251127,
-17.9265254096188));
#20117=CARTESIAN_POINT('Ctrl Pts',(-48.3539734314675,-9.28355639505876,
-17.5754184692672));
#20118=CARTESIAN_POINT('Ctrl Pts',(-48.3539734314711,-9.22712679184453,
-17.4115982321832));
#20119=CARTESIAN_POINT('Ctrl Pts',(-48.3539734314525,-9.17133865071588,
-17.247630070549));
#20120=CARTESIAN_POINT('Ctrl Pts',(-48.3539734313696,-9.11619658428807,
-17.0834969853208));
#20121=CARTESIAN_POINT('Ctrl Pts',(-48.3539734305581,-8.57607118782138,
-15.4757870557661));
#20122=CARTESIAN_POINT('Ctrl Pts',(-48.353973428403,-8.09914441522936,-13.8554310180361));
#20123=CARTESIAN_POINT('Ctrl Pts',(-48.3539734276855,-7.69433779295044,
-12.2206426330261));
#20124=CARTESIAN_POINT('Ctrl Pts',(-48.3539734269937,-7.30405740045158,
-10.6445175959344));
#20125=CARTESIAN_POINT('Ctrl Pts',(-48.3539734277293,-6.98081414568337,
-9.05497754756053));
#20126=CARTESIAN_POINT('Ctrl Pts',(-48.3539734292173,-6.73255660928855,
-7.45043168080743));
#20127=CARTESIAN_POINT('Ctrl Pts',(-48.3539734302404,-6.56187116055321,
-6.3472521549798));
#20128=CARTESIAN_POINT('Ctrl Pts',(-48.3539734315641,-6.42663073464616,
-5.23697946849498));
#20129=CARTESIAN_POINT('Ctrl Pts',(-48.3539734316352,-6.32940458230556,
-4.11909983610374));
#20130=CARTESIAN_POINT('Origin',(-48.3539734376649,-78.8840761544994,0.0839788705204157));
#20131=CARTESIAN_POINT('Origin',(-39.6912298733813,16.4855954176946,-41.0181498645286));
#20132=CARTESIAN_POINT('',(-37.8722959448873,-8.24885981233827,-39.1992159360346));
#20133=CARTESIAN_POINT('Ctrl Pts',(-34.5978496132723,-3.61941807409669,
-35.9247696044197));
#20134=CARTESIAN_POINT('Ctrl Pts',(-35.144360826703,-4.3920600802535,-36.4712808178504));
#20135=CARTESIAN_POINT('Ctrl Pts',(-35.6908680880204,-5.16470767732064,
-37.0177880791678));
#20136=CARTESIAN_POINT('Ctrl Pts',(-36.7823498735465,-6.70785538323104,
-38.1092698646939));
#20137=CARTESIAN_POINT('Ctrl Pts',(-37.3273244157758,-7.4783554666459,-38.6542444069232));
#20138=CARTESIAN_POINT('Ctrl Pts',(-37.8722959448873,-8.24885981233827,
-39.1992159360346));
#20139=CARTESIAN_POINT('',(-39.0283172660189,-8.24885981233827,-40.3552372571663));
#20140=CARTESIAN_POINT('',(-35.219899890096,12.8136401876617,-36.5468198812434));
#20141=CARTESIAN_POINT('',(-35.1331064857663,12.8136401876617,-36.4600264769137));
#20142=CARTESIAN_POINT('',(-35.219899890096,12.8136401876617,-36.5468198812434));
#20143=CARTESIAN_POINT('Origin',(-41.017055088106,16.4855954176946,-39.6923246498039));
#20144=CARTESIAN_POINT('',(-39.198121159612,-8.24885981233827,-37.8733907213099));
#20145=CARTESIAN_POINT('',(-39.1110035352202,-8.24885981233827,-37.7862730969181));
#20146=CARTESIAN_POINT('',(-35.9236748279971,-3.61941807409669,-34.5989443896949));
#20147=CARTESIAN_POINT('Ctrl Pts',(-39.198121159612,-8.24885981233827,-37.8733907213099));
#20148=CARTESIAN_POINT('Ctrl Pts',(-38.6531496305005,-7.47835546664588,
-37.3284191921984));
#20149=CARTESIAN_POINT('Ctrl Pts',(-38.1081750882713,-6.70785538323099,
-36.7834446499691));
#20150=CARTESIAN_POINT('Ctrl Pts',(-37.0166933027451,-5.1647076773206,-35.6919628644429));
#20151=CARTESIAN_POINT('Ctrl Pts',(-36.4701860414278,-4.39206008025347,
-35.1454556031256));
#20152=CARTESIAN_POINT('Ctrl Pts',(-35.9236748279971,-3.61941807409669,
-34.5989443896949));
#20153=CARTESIAN_POINT('',(-35.9236748279974,11.9341984494207,-34.5989443896953));
#20154=CARTESIAN_POINT('',(-35.9236748279971,12.0636401876617,-34.5989443896949));
#20155=CARTESIAN_POINT('',(-36.5457251048207,12.8136401876617,-35.2209946665186));
#20156=CARTESIAN_POINT('',(-35.9236748279971,11.9341984494202,-34.5989443896949));
#20157=CARTESIAN_POINT('',(-40.3541424807436,12.8136401876617,-39.0294120424415));
#20158=CARTESIAN_POINT('Origin',(0.0835265683620477,-11.0169045823054,0.0824317919394229));
#20159=CARTESIAN_POINT('',(-9.89989012376418,-11.3294045823054,-19.3815610191817));
#20160=CARTESIAN_POINT('',(-9.89989012376418,-14.4544045823054,-19.3815610191817));
#20161=CARTESIAN_POINT('',(-9.89989012376418,-11.0169045823054,-19.3815610191817));
#20162=CARTESIAN_POINT('',(-20.6911418173041,-14.4544045823054,-6.76802647489247));
#20163=CARTESIAN_POINT('Origin',(0.0835265683620477,-14.4544045823054,0.0824317919394229));
#20164=CARTESIAN_POINT('',(-20.6911418173041,-11.3294045823054,-6.76802647489247));
#20165=CARTESIAN_POINT('',(-20.6911418173041,-11.0169045823054,-6.76802647489247));
#20166=CARTESIAN_POINT('Origin',(0.0835265683620477,-11.3294045823054,0.0824317919394229));
#20167=CARTESIAN_POINT('Origin',(0.0835265683620477,-13.2044045823054,0.0824317919394229));
#20168=CARTESIAN_POINT('',(-34.1929414312581,-13.2044045823054,-34.5829146143929));
#20169=CARTESIAN_POINT('',(-41.2766849510695,-13.2044045823054,-36.9187829158523));
#20170=CARTESIAN_POINT('',(-41.5387861275671,-13.2044045823054,-37.0052109222086));
#20171=CARTESIAN_POINT('',(-40.1126065460396,-13.2044045823054,-38.1801853354021));
#20172=CARTESIAN_POINT('Origin',(0.0835265683620477,-13.2044045823054,0.0824317919394229));
#20173=CARTESIAN_POINT('',(-32.9108164063353,-13.2044045823054,-35.8053910964449));
#20174=CARTESIAN_POINT('',(7.52116697235096,-13.2044045823054,-22.4729224553552));
#20175=CARTESIAN_POINT('Origin',(0.0835265683620477,-13.2044045823054,0.0824317919394229));
#20176=CARTESIAN_POINT('Origin',(7.61903066187713,16.4855954176946,-22.7697034322933));
#20177=CARTESIAN_POINT('',(-32.8129527168091,-12.8919045823054,-36.102172073383));
#20178=CARTESIAN_POINT('',(-39.0675209577957,-12.8919045823054,-38.1646193729747));
#20179=CARTESIAN_POINT('',(7.61903066187713,-12.8919045823054,-22.7697034322933));
#20180=CARTESIAN_POINT('',(-32.8129496113305,-7.07886051013308,-36.1021710493883));
#20181=CARTESIAN_POINT('Ctrl Pts',(-39.0675209577957,-12.8919045823054,
-38.1646193729747));
#20182=CARTESIAN_POINT('Ctrl Pts',(-37.4159861250462,-11.333902336486,-37.6200248582543));
#20183=CARTESIAN_POINT('Ctrl Pts',(-35.7569364419389,-9.78474033506735,
-37.0729523175167));
#20184=CARTESIAN_POINT('Ctrl Pts',(-34.0875946907817,-8.24794400051366,
-36.5224859617085));
#20185=CARTESIAN_POINT('Ctrl Pts',(-33.6633986356396,-7.85742903123153,
-36.3826070804306));
#20186=CARTESIAN_POINT('Ctrl Pts',(-33.2385378437358,-7.46771271973443,
-36.2425090018419));
#20187=CARTESIAN_POINT('Ctrl Pts',(-32.8129663798493,-7.07885337126046,
-36.102176578778));
#20188=CARTESIAN_POINT('',(-32.8129527168091,16.4855954176946,-36.102172073383));
#20189=CARTESIAN_POINT('Origin',(0.0835265683620477,-13.2044045823054,0.0824317919394229));
#20190=CARTESIAN_POINT('',(-39.8705894675228,-13.2044045823054,-27.8501855539351));
#20191=CARTESIAN_POINT('',(-46.5229781270741,-13.2044045823054,-30.0438143542121));
#20192=CARTESIAN_POINT('',(-46.726369315508,-13.2044045823054,-30.1108827098817));
#20193=CARTESIAN_POINT('',(-45.6231018412815,-13.2044045823054,-31.3923375671359));
#20194=CARTESIAN_POINT('Origin',(0.0835265683620477,-13.2044045823054,0.0824317919394229));
#20195=CARTESIAN_POINT('',(-38.9085015017574,-13.2044045823054,-29.1781944313494));
#20196=CARTESIAN_POINT('',(4.96196078618764,-13.2044045823054,-14.7118854886011));
#20197=CARTESIAN_POINT('Origin',(0.0835265683620477,-13.2044045823054,0.0824317919394229));
#20198=CARTESIAN_POINT('Origin',(4.37477864903062,16.4855954176946,-12.9311996269726));
#20199=CARTESIAN_POINT('',(-39.968453157049,-12.8919045823054,-27.553404576997));
#20200=CARTESIAN_POINT('',(-39.9684532734914,-6.59535001054288,-27.5534046153939));
#20201=CARTESIAN_POINT('',(-39.968453157049,-6.01690458230549,-27.553404576997));
#20202=CARTESIAN_POINT('',(-46.1602402810308,-12.8919045823054,-29.5951497689063));
#20203=CARTESIAN_POINT('Ctrl Pts',(-39.968453721219,-6.59534981969064,-27.5534047630323));
#20204=CARTESIAN_POINT('Ctrl Pts',(-42.0370533398943,-8.68909917212592,
-28.2355266191048));
#20205=CARTESIAN_POINT('Ctrl Pts',(-44.1004290564877,-10.788569829982,-28.9159258906075));
#20206=CARTESIAN_POINT('Ctrl Pts',(-46.1602402810309,-12.8919045823054,
-29.5951497689063));
#20207=CARTESIAN_POINT('',(-39.74712214338,-12.8919045823054,-27.4804205541405));
#20208=CARTESIAN_POINT('Origin',(0.0835265683620477,15.5455954176946,0.0824317919394229));
#20209=CARTESIAN_POINT('',(-28.9637578711591,16.1705954176946,-46.6214788225857));
#20210=CARTESIAN_POINT('Origin',(0.0835265683620477,16.1705954176946,0.0824317919394229));
#20211=CARTESIAN_POINT('',(-28.9637578711591,15.8580954176946,-46.6214788225857));
#20212=CARTESIAN_POINT('',(-28.9637578711591,15.5455954176946,-46.6214788225857));
#20213=CARTESIAN_POINT('Origin',(0.0835265683620477,15.8580954176946,0.0824317919394229));
#20214=CARTESIAN_POINT('Origin',(-48.3539734316379,15.5455954176946,-42.6687705759647));
#20215=CARTESIAN_POINT('',(-48.3539734316379,15.8580954176946,-39.9964034940395));
#20216=CARTESIAN_POINT('',(-48.3539734316379,16.1705954176946,-39.9964034940395));
#20217=CARTESIAN_POINT('',(-48.3539734316379,16.4830954176946,-39.9964034940395));
#20218=CARTESIAN_POINT('',(-48.3539734316379,16.1705954176946,-29.4599768141645));
#20219=CARTESIAN_POINT('',(-48.3539734316379,15.8580954176946,-42.6687705759647));
#20220=CARTESIAN_POINT('Origin',(-25.9704288655064,15.5455954176946,-48.3550682080606));
#20221=CARTESIAN_POINT('',(-29.4588820377419,15.8580954176946,-48.3550682080606));
#20222=CARTESIAN_POINT('',(-29.4588820377419,16.1705954176946,-48.3550682080606));
#20223=CARTESIAN_POINT('',(-29.4588820377419,16.4830954176946,-48.3550682080606));
#20224=CARTESIAN_POINT('',(-39.9953087176169,16.1705954176946,-48.3550682080606));
#20225=CARTESIAN_POINT('',(-39.9953087176169,16.1705954176946,-48.3550682080606));
#20226=CARTESIAN_POINT('',(-39.9953087176169,15.8580954176946,-48.3550682080606));
#20227=CARTESIAN_POINT('',(-39.9953087176169,15.5455954176946,-48.3550682080606));
#20228=CARTESIAN_POINT('',(-25.9704288655064,15.8580954176946,-48.3550682080606));
#20229=CARTESIAN_POINT('Origin',(0.0835265683620477,15.5455954176946,0.0824317919394229));
#20230=CARTESIAN_POINT('',(-48.0414734316379,15.5455954176946,-39.9964034940395));
#20231=CARTESIAN_POINT('Origin',(-47.4164734316379,15.5455954176946,-39.9964034940395));
#20232=CARTESIAN_POINT('',(-48.0414734316379,15.5455954176946,0.0824317919394229));
#20233=CARTESIAN_POINT('',(-29.1287992600201,15.5455954176946,-46.8868419510773));
#20234=CARTESIAN_POINT('Origin',(0.0835265683620477,15.5455954176946,0.0824317919394229));
#20235=CARTESIAN_POINT('',(-29.4588820377419,15.5455954176946,-48.0425682080606));
#20236=CARTESIAN_POINT('Origin',(-29.4588820377419,15.5455954176946,-47.4175682080606));
#20237=CARTESIAN_POINT('',(-39.9953087176169,15.5455954176946,-48.0425682080606));
#20238=CARTESIAN_POINT('',(0.0835265683620977,15.5455954176946,-48.0425682080605));
#20239=CARTESIAN_POINT('Origin',(-39.9953087176169,15.5455954176946,-47.4175682080606));
#20240=CARTESIAN_POINT('Origin',(-29.4588820377419,15.5455954176946,-47.4175682080606));
#20241=CARTESIAN_POINT('Origin',(-29.4588820377419,15.8580954176946,-47.4175682080606));
#20242=CARTESIAN_POINT('Origin',(-29.4588820377419,16.1705954176946,-47.4175682080606));
#20243=CARTESIAN_POINT('Origin',(-47.4164734316379,15.5455954176946,-39.9964034940395));
#20244=CARTESIAN_POINT('Origin',(-47.4164734316379,15.8580954176946,-39.9964034940395));
#20245=CARTESIAN_POINT('Origin',(-47.4164734316379,16.1705954176946,-39.9964034940395));
#20246=CARTESIAN_POINT('Origin',(-39.9953087176169,15.5455954176946,-47.4175682080606));
#20247=CARTESIAN_POINT('Origin',(-39.9953087176169,15.8580954176946,-47.4175682080606));
#20248=CARTESIAN_POINT('Origin',(-39.9953087176169,16.1705954176946,-47.4175682080606));
#20249=CARTESIAN_POINT('Origin',(0.0835265683620477,-6.01690458230549,0.0824317919394229));
#20250=CARTESIAN_POINT('',(31.6836214013763,-13.2959337131846,-45.8061901631445));
#20251=CARTESIAN_POINT('',(30.3297286714006,-13.2959337131846,-46.7096495545262));
#20252=CARTESIAN_POINT('Origin',(0.0835265683620477,-13.2959337131846,0.0824317919394229));
#20253=CARTESIAN_POINT('',(29.5826474545624,-12.6709337131846,-46.4458225157374));
#20254=CARTESIAN_POINT('Ctrl Pts',(30.3297286714006,-13.2959337131846,-46.7096495545262));
#20255=CARTESIAN_POINT('Ctrl Pts',(30.2953116335171,-13.2959337131846,-46.7318965812379));
#20256=CARTESIAN_POINT('Ctrl Pts',(30.2590829799862,-13.2919430659199,-46.7505039986476));
#20257=CARTESIAN_POINT('Ctrl Pts',(30.2221538011279,-13.2842290832321,-46.7650885650838));
#20258=CARTESIAN_POINT('Ctrl Pts',(30.1851131667048,-13.2764918190547,-46.779717149046));
#20259=CARTESIAN_POINT('Ctrl Pts',(30.1473660521867,-13.2650083398801,-46.7902992078703));
#20260=CARTESIAN_POINT('Ctrl Pts',(30.1100232324367,-13.2500137812862,-46.7964131006815));
#20261=CARTESIAN_POINT('Ctrl Pts',(30.0963576295144,-13.2445265233579,-46.7986504794341));
#20262=CARTESIAN_POINT('Ctrl Pts',(30.0827461978655,-13.2385687578801,-46.800289099107));
#20263=CARTESIAN_POINT('Ctrl Pts',(30.0692437277915,-13.232151003965,-46.8013068668765));
#20264=CARTESIAN_POINT('Ctrl Pts',(30.06896789394,-13.2320198995248,-46.801327658243));
#20265=CARTESIAN_POINT('Ctrl Pts',(30.0686921064576,-13.2318886036913,-46.801348190617));
#20266=CARTESIAN_POINT('Ctrl Pts',(30.0684163658334,-13.2317571165657,-46.80136846381));
#20267=CARTESIAN_POINT('Ctrl Pts',(30.0213645219584,-13.2093204091551,-46.8048278420269));
#20268=CARTESIAN_POINT('Ctrl Pts',(29.9767272365876,-13.1821368365904,-46.8010574025015));
#20269=CARTESIAN_POINT('Ctrl Pts',(29.9353668651223,-13.1520894283177,-46.7917741093876));
#20270=CARTESIAN_POINT('Ctrl Pts',(29.9003561104518,-13.126654878234,-46.7839159812753));
#20271=CARTESIAN_POINT('Ctrl Pts',(29.8676937058866,-13.0991694705196,-46.7721089114476));
#20272=CARTESIAN_POINT('Ctrl Pts',(29.8379008490097,-13.0707895719798,-46.7574125642514));
#20273=CARTESIAN_POINT('Ctrl Pts',(29.8376173879301,-13.0705195543472,-46.7572727373641));
#20274=CARTESIAN_POINT('Ctrl Pts',(29.8373341809497,-13.0702494422352,-46.7571326365248));
#20275=CARTESIAN_POINT('Ctrl Pts',(29.8370512286687,-13.0699792368,-46.7569922627404));
#20276=CARTESIAN_POINT('Ctrl Pts',(29.8166813000282,-13.0505269623214,-46.7468866577897));
#20277=CARTESIAN_POINT('Ctrl Pts',(29.7974702652244,-13.0305367697043,-46.7354061965312));
#20278=CARTESIAN_POINT('Ctrl Pts',(29.779419955612,-13.0101903794891,-46.722765565803));
#20279=CARTESIAN_POINT('Ctrl Pts',(29.7688872570839,-12.9983178743149,-46.7153895176619));
#20280=CARTESIAN_POINT('Ctrl Pts',(29.758748871208,-12.9863240855331,-46.7076190123881));
#20281=CARTESIAN_POINT('Ctrl Pts',(29.748998012555,-12.9742444051773,-46.6995004081416));
#20282=CARTESIAN_POINT('Ctrl Pts',(29.7356513039303,-12.9577100691025,-46.6883878847044));
#20283=CARTESIAN_POINT('Ctrl Pts',(29.7230341631078,-12.9410147689399,-46.6766208987538));
#20284=CARTESIAN_POINT('Ctrl Pts',(29.7111382215491,-12.9242496162066,-46.6643130148113));
#20285=CARTESIAN_POINT('Ctrl Pts',(29.7051902507697,-12.9158670398399,-46.6581590728401));
#20286=CARTESIAN_POINT('Ctrl Pts',(29.6994225797523,-12.9074670004228,-46.6518699062888));
#20287=CARTESIAN_POINT('Ctrl Pts',(29.6938341619597,-12.8990608878296,-46.6454597098703));
#20288=CARTESIAN_POINT('Ctrl Pts',(29.6882457441671,-12.8906547752363,-46.6390495134518));
#20289=CARTESIAN_POINT('Ctrl Pts',(29.6828365795893,-12.8822425894822,-46.6325182871528));
#20290=CARTESIAN_POINT('Ctrl Pts',(29.6776056213999,-12.8738357211132,-46.6258802250576));
#20291=CARTESIAN_POINT('Ctrl Pts',(29.661151233601,-12.8473912596384,-46.604999681954));
#20292=CARTESIAN_POINT('Ctrl Pts',(29.6462987841921,-12.820747274008,-46.5828657680258));
#20293=CARTESIAN_POINT('Ctrl Pts',(29.6330144113446,-12.7940681980236,-46.5596959484487));
#20294=CARTESIAN_POINT('Ctrl Pts',(29.6294060259108,-12.7868214585446,-46.5534024154062));
#20295=CARTESIAN_POINT('Ctrl Pts',(29.6259136021541,-12.7795722581719,-46.5470324354036));
#20296=CARTESIAN_POINT('Ctrl Pts',(29.6225370413182,-12.7723242153339,-46.5405903840077));
#20297=CARTESIAN_POINT('Ctrl Pts',(29.6102672896986,-12.7459862668495,-46.5171812483842));
#20298=CARTESIAN_POINT('Ctrl Pts',(29.5995238745078,-12.7196622748057,-46.4928211348268));
#20299=CARTESIAN_POINT('Ctrl Pts',(29.5902746512498,-12.693508739059,-46.4677171585527));
#20300=CARTESIAN_POINT('Ctrl Pts',(29.5876078409674,-12.6859679417289,-46.4604789786333));
#20301=CARTESIAN_POINT('Ctrl Pts',(29.5850654985989,-12.6784415052658,-46.4531790258387));
#20302=CARTESIAN_POINT('Ctrl Pts',(29.5826474545624,-12.6709337131846,-46.4458225157374));
#20303=CARTESIAN_POINT('',(27.4605785366061,-6.10843371318477,-39.9870540284925));
#20304=CARTESIAN_POINT('Origin',(79.5093886191839,-177.510309510992,-197.332122666226));
#20305=CARTESIAN_POINT('',(4.30427685474491,-6.1084337131847,-48.2627017315676));
#20306=CARTESIAN_POINT('Origin',(0.0835265683620477,-6.10843371318469,0.0824317919394229));
#20307=CARTESIAN_POINT('',(30.5121796307595,-14.6753754514266,-48.2295435588552));
#20308=CARTESIAN_POINT('Ctrl Pts',(4.30427685533897,-6.10843371318471,-48.2627017315157));
#20309=CARTESIAN_POINT('Ctrl Pts',(8.94175590178151,-6.50994980321315,-48.2608720750402));
#20310=CARTESIAN_POINT('Ctrl Pts',(13.4240603542055,-7.55645913600449,-48.2561124331622));
#20311=CARTESIAN_POINT('Ctrl Pts',(19.9841318245208,-9.80534906153842,-48.2470092000062));
#20312=CARTESIAN_POINT('Ctrl Pts',(22.1452414843856,-10.6692546575742,-48.2436494975834));
#20313=CARTESIAN_POINT('Ctrl Pts',(26.3834535137794,-12.5596572871779,-48.2367077593843));
#20314=CARTESIAN_POINT('Ctrl Pts',(28.4629814284201,-13.58630787804,-48.2331238453003));
#20315=CARTESIAN_POINT('Ctrl Pts',(30.5121796307589,-14.6753754514262,-48.2295435588551));
#20316=CARTESIAN_POINT('',(32.131950172941,-14.6753754514262,-47.17059386726));
#20317=CARTESIAN_POINT('Origin',(0.0835265683620477,-14.6753754514262,0.0824317919394229));
#20318=CARTESIAN_POINT('Origin',(-321.603193845972,-1402.95413117761,1241.62885743152));
#20319=CARTESIAN_POINT('Origin',(15.1746248258407,-11.0169045823054,5.05872969929124));
#20320=CARTESIAN_POINT('',(20.1223573965802,-11.3294045823054,-9.94574144911951));
#20321=CARTESIAN_POINT('',(20.1223573965802,-11.0169045823054,-9.94574144911951));
#20322=CARTESIAN_POINT('',(29.4342239561067,-11.3294045823054,-38.184865357424));
#20323=CARTESIAN_POINT('',(15.1746248258407,-11.3294045823054,5.05872969929124));
#20324=CARTESIAN_POINT('',(29.4342239561067,-12.8919045823054,-38.184865357424));
#20325=CARTESIAN_POINT('',(29.4342239561067,-11.0169045823054,-38.184865357424));
#20326=CARTESIAN_POINT('',(29.6409337685891,-13.5169045823054,-38.8117325886538));
#20327=CARTESIAN_POINT('Ctrl Pts',(29.6409337685891,-13.5169045823054,-38.8117325886538));
#20328=CARTESIAN_POINT('Ctrl Pts',(29.6292942393977,-13.516904574972,-38.7764346057018));
#20329=CARTESIAN_POINT('Ctrl Pts',(29.617680555433,-13.5137764691088,-38.7412150008653));
#20330=CARTESIAN_POINT('Ctrl Pts',(29.6062374009932,-13.5077394335824,-38.7065125430914));
#20331=CARTESIAN_POINT('Ctrl Pts',(29.5939633721145,-13.5012640557673,-38.6692903792972));
#20332=CARTESIAN_POINT('Ctrl Pts',(29.5818851650686,-13.4914421681939,-38.6326620639058));
#20333=CARTESIAN_POINT('Ctrl Pts',(29.5701745905273,-13.4784883891808,-38.5971486291694));
#20334=CARTESIAN_POINT('Ctrl Pts',(29.5582820089413,-13.4653332811016,-38.5610832407026));
#20335=CARTESIAN_POINT('Ctrl Pts',(29.5467680680181,-13.4489478321172,-38.5261661161798));
#20336=CARTESIAN_POINT('Ctrl Pts',(29.5358129510534,-13.4295031815268,-38.4929436786193));
#20337=CARTESIAN_POINT('Ctrl Pts',(29.5252137549884,-13.4106902683751,-38.4608006051502));
#20338=CARTESIAN_POINT('Ctrl Pts',(29.5151372397151,-13.3890130654928,-38.4302426110392));
#20339=CARTESIAN_POINT('Ctrl Pts',(29.505753620787,-13.3645846069503,-38.4017858911997));
#20340=CARTESIAN_POINT('Ctrl Pts',(29.502706973872,-13.3566532439626,-38.3925466437009));
#20341=CARTESIAN_POINT('Ctrl Pts',(29.499733451499,-13.348431556951,-38.3835291533526));
#20342=CARTESIAN_POINT('Ctrl Pts',(29.4968391572844,-13.3399225829037,-38.3747519299551));
#20343=CARTESIAN_POINT('Ctrl Pts',(29.4968079493295,-13.339830834222,-38.3746572888538));
#20344=CARTESIAN_POINT('Ctrl Pts',(29.4967767506818,-13.3397390509053,-38.3745626759776));
#20345=CARTESIAN_POINT('Ctrl Pts',(29.4967455613462,-13.3396472329756,-38.3744680913411));
#20346=CARTESIAN_POINT('Ctrl Pts',(29.485255261427,-13.3058210700066,-38.3396226603605));
#20347=CARTESIAN_POINT('Ctrl Pts',(29.475076277546,-13.267440322379,-38.3087539204414));
#20348=CARTESIAN_POINT('Ctrl Pts',(29.4664377760755,-13.2257618865122,-38.2825568404197));
#20349=CARTESIAN_POINT('Ctrl Pts',(29.4618903252278,-13.2038216646858,-38.2687662617925));
#20350=CARTESIAN_POINT('Ctrl Pts',(29.4577699082708,-13.1809667715091,-38.2562707041878));
#20351=CARTESIAN_POINT('Ctrl Pts',(29.4541112021333,-13.1573764603984,-38.245175328701));
#20352=CARTESIAN_POINT('Ctrl Pts',(29.4482111530888,-13.1193345987958,-38.2272828669731));
#20353=CARTESIAN_POINT('Ctrl Pts',(29.4435099348019,-13.0793753611095,-38.2130259739134));
#20354=CARTESIAN_POINT('Ctrl Pts',(29.4401602474623,-13.0382175959794,-38.2028677274188));
#20355=CARTESIAN_POINT('Ctrl Pts',(29.4368767709741,-12.9978733666794,-38.192910271649));
#20356=CARTESIAN_POINT('Ctrl Pts',(29.4348920783845,-12.9563778844129,-38.1868915019856));
#20357=CARTESIAN_POINT('Ctrl Pts',(29.4343654883888,-12.9144212112981,-38.1852945675748));
#20358=CARTESIAN_POINT('Ctrl Pts',(29.4342714552248,-12.9069290090975,-38.185009403032));
#20359=CARTESIAN_POINT('Ctrl Pts',(29.4342239572584,-12.8994221374127,-38.1848653609166));
#20360=CARTESIAN_POINT('Ctrl Pts',(29.4342239561067,-12.8919045823054,-38.184865357424));
#20361=CARTESIAN_POINT('',(31.8550769043756,-13.5169045823054,-45.5263329281778));
#20362=CARTESIAN_POINT('',(15.1746248258407,-13.5169045823054,5.05872969929124));
#20363=CARTESIAN_POINT('',(32.1607495565261,-14.4544045724555,-46.4533144140353));
#20364=CARTESIAN_POINT('Origin',(-385.578293801187,-1402.30169514568,1220.38019629327));
#20365=CARTESIAN_POINT('',(15.1746248258407,-14.4544045823054,5.05872969929124));
#20366=CARTESIAN_POINT('Origin',(20.8581949540281,-11.0169045823054,6.93289005877139));
#20367=CARTESIAN_POINT('',(20.8581949540281,-11.3294045823054,6.93289005877139));
#20368=CARTESIAN_POINT('',(20.8581949540281,-11.3294045823054,6.93289005877131));
#20369=CARTESIAN_POINT('',(20.8581949540281,-14.4544045823054,6.93289005877139));
#20370=CARTESIAN_POINT('',(20.8581949540281,-11.0169045823054,6.93289005877139));
#20371=CARTESIAN_POINT('',(37.1077603633878,-14.4544045474399,-42.3454676279164));
#20372=CARTESIAN_POINT('',(37.4052635491749,-14.4544045823054,-43.2476744274668));
#20373=CARTESIAN_POINT('',(36.7879602992159,-13.5169045823054,-41.3756434170181));
#20374=CARTESIAN_POINT('Origin',(-151.647538790397,-669.972713648666,530.072988729517));
#20375=CARTESIAN_POINT('',(34.4520919977564,-13.5169045823054,-34.2918998972067));
#20376=CARTESIAN_POINT('',(34.3920744991467,-13.5169045823054,-34.1098911056212));
#20377=CARTESIAN_POINT('Ctrl Pts',(34.2319046026008,-12.8919045823054,-33.6241606104486));
#20378=CARTESIAN_POINT('Ctrl Pts',(34.2319046026008,-12.9240089539757,-33.6241606104486));
#20379=CARTESIAN_POINT('Ctrl Pts',(34.2327660676948,-12.955801183813,-33.6267730855496));
#20380=CARTESIAN_POINT('Ctrl Pts',(34.2344596877549,-12.9870390822744,-33.6319091499924));
#20381=CARTESIAN_POINT('Ctrl Pts',(34.2361941274839,-13.0190298772671,-33.6371690039758));
#20382=CARTESIAN_POINT('Ctrl Pts',(34.2388012607647,-13.0504387215055,-33.6450753844307));
#20383=CARTESIAN_POINT('Ctrl Pts',(34.2422325669316,-13.0810143824795,-33.655481147807));
#20384=CARTESIAN_POINT('Ctrl Pts',(34.2446351437452,-13.1024232485338,-33.6627671912553));
#20385=CARTESIAN_POINT('Ctrl Pts',(34.2474414246086,-13.1234238076974,-33.6712775057571));
#20386=CARTESIAN_POINT('Ctrl Pts',(34.2506302568241,-13.1439346499851,-33.6809479437379));
#20387=CARTESIAN_POINT('Ctrl Pts',(34.25064462592,-13.1440270732421,-33.6809915193923));
#20388=CARTESIAN_POINT('Ctrl Pts',(34.2506590017993,-13.1441194808469,-33.6810351156181));
#20389=CARTESIAN_POINT('Ctrl Pts',(34.2506733844596,-13.1442118727969,-33.681078732408));
#20390=CARTESIAN_POINT('Ctrl Pts',(34.262088806318,-13.2175427492195,-33.7156970884852));
#20391=CARTESIAN_POINT('Ctrl Pts',(34.2778470820053,-13.2814833078763,-33.7634855632141));
#20392=CARTESIAN_POINT('Ctrl Pts',(34.297083605806,-13.3355724238096,-33.8218221572446));
#20393=CARTESIAN_POINT('Ctrl Pts',(34.2984164892935,-13.3393202157823,-33.8258642536082));
#20394=CARTESIAN_POINT('Ctrl Pts',(34.2997660765859,-13.3430206976121,-33.8299570058538));
#20395=CARTESIAN_POINT('Ctrl Pts',(34.3011320820256,-13.3466737099125,-33.8340995476976));
#20396=CARTESIAN_POINT('Ctrl Pts',(34.3011486427789,-13.3467179971708,-33.8341497697625));
#20397=CARTESIAN_POINT('Ctrl Pts',(34.30116520512,-13.3467622754629,-33.8341999966422));
#20398=CARTESIAN_POINT('Ctrl Pts',(34.3011817690487,-13.3468065447896,-33.8342502283365));
#20399=CARTESIAN_POINT('Ctrl Pts',(34.3222770796446,-13.4031865990188,-33.8982237706922));
#20400=CARTESIAN_POINT('Ctrl Pts',(34.3459380694435,-13.4450083105498,-33.9699779800617));
#20401=CARTESIAN_POINT('Ctrl Pts',(34.3718849768693,-13.4738659092279,-34.0486644527659));
#20402=CARTESIAN_POINT('Ctrl Pts',(34.3978462731079,-13.5027395108376,-34.127394560918));
#20403=CARTESIAN_POINT('Ctrl Pts',(34.4246047850287,-13.5169045582356,-34.2085423016968));
#20404=CARTESIAN_POINT('Ctrl Pts',(34.4520919977564,-13.5169045823054,-34.2918998972067));
#20405=CARTESIAN_POINT('Origin',(0.0835265683620477,-6.01690458230549,0.0824317919394229));
#20406=CARTESIAN_POINT('',(48.4286602621091,-6.10843422628167,-4.13831834965265));
#20407=CARTESIAN_POINT('',(36.459401449836,-6.10843371299757,-32.0401832164143));
#20408=CARTESIAN_POINT('Origin',(0.0835265683620477,-6.10843371318468,0.0824317919394229));
#20409=CARTESIAN_POINT('',(38.7825797314222,-12.6709337131846,-39.1280242913702));
#20410=CARTESIAN_POINT('Ctrl Pts',(36.4594014504071,-6.10843371318764,-32.0401832160548));
#20411=CARTESIAN_POINT('Ctrl Pts',(36.6177503688256,-6.54712953979038,-32.5236246202131));
#20412=CARTESIAN_POINT('Ctrl Pts',(36.7757172835296,-6.98698298252111,-33.0061517892532));
#20413=CARTESIAN_POINT('Ctrl Pts',(36.9334136781008,-7.42790908716257,-33.4877815134637));
#20414=CARTESIAN_POINT('Ctrl Pts',(37.0904935659948,-7.8671114118254,-33.967528328799));
#20415=CARTESIAN_POINT('Ctrl Pts',(37.2473051036632,-8.30737802775023,-34.4463847898388));
#20416=CARTESIAN_POINT('Ctrl Pts',(37.4039138029555,-8.74862497320324,-34.9243934293266));
#20417=CARTESIAN_POINT('Ctrl Pts',(37.5602173246846,-9.18901207710122,-35.4014705911098));
#20418=CARTESIAN_POINT('Ctrl Pts',(37.7163188570147,-9.63037569358639,-35.8777032990578));
#20419=CARTESIAN_POINT('Ctrl Pts',(37.8722380448622,-10.0726323508084,-36.3531585902921));
#20420=CARTESIAN_POINT('Ctrl Pts',(38.0277161383152,-10.5136378667497,-36.8272688215204));
#20421=CARTESIAN_POINT('Ctrl Pts',(38.1830129581763,-10.955531377762,-37.3006060886532));
#20422=CARTESIAN_POINT('Ctrl Pts',(38.3381019771589,-11.3982301184165,-37.7732605459248));
#20423=CARTESIAN_POINT('Ctrl Pts',(38.4864727775814,-11.8217518282566,-38.2254403366584));
#20424=CARTESIAN_POINT('Ctrl Pts',(38.63465313382,-12.2460105161165,-38.6769953773671));
#20425=CARTESIAN_POINT('Ctrl Pts',(38.7825797314222,-12.6709337131846,-39.1280242913702));
#20426=CARTESIAN_POINT('',(38.4984968574033,-13.2959337131846,-40.2737533112661));
#20427=CARTESIAN_POINT('Ctrl Pts',(38.4984968574034,-13.2959337131846,-40.273753311266));
#20428=CARTESIAN_POINT('Ctrl Pts',(38.5331904713011,-13.2959336603243,-40.2407284579781));
#20429=CARTESIAN_POINT('Ctrl Pts',(38.5644068713101,-13.291660512867,-40.2050259534244));
#20430=CARTESIAN_POINT('Ctrl Pts',(38.5925219243482,-13.2840750781511,-40.1676284350549));
#20431=CARTESIAN_POINT('Ctrl Pts',(38.6250024648541,-13.2753118359401,-40.1244241199653));
#20432=CARTESIAN_POINT('Ctrl Pts',(38.6533440434163,-13.2621273075647,-40.0789565662769));
#20433=CARTESIAN_POINT('Ctrl Pts',(38.6780885048562,-13.2459526169403,-40.032706281476));
#20434=CARTESIAN_POINT('Ctrl Pts',(38.6853255888349,-13.2412219585397,-40.0191793273347));
#20435=CARTESIAN_POINT('Ctrl Pts',(38.692254746233,-13.2362352705224,-40.005585284207));
#20436=CARTESIAN_POINT('Ctrl Pts',(38.6988890084814,-13.2310278528738,-39.9919609828319));
#20437=CARTESIAN_POINT('Ctrl Pts',(38.6989109743279,-13.2310106112676,-39.9919158731721));
#20438=CARTESIAN_POINT('Ctrl Pts',(38.6989329369403,-13.230993367242,-39.9918707631823));
#20439=CARTESIAN_POINT('Ctrl Pts',(38.6989548963189,-13.2309761207981,-39.9918256528639));
#20440=CARTESIAN_POINT('Ctrl Pts',(38.7427007443125,-13.1966190324461,-39.9019602168528));
#20441=CARTESIAN_POINT('Ctrl Pts',(38.7735109344404,-13.1525556490531,-39.810753760552));
#20442=CARTESIAN_POINT('Ctrl Pts',(38.7942479882117,-13.1028429791957,-39.7212397410345));
#20443=CARTESIAN_POINT('Ctrl Pts',(38.796698753037,-13.0969677924886,-39.7106607160278));
#20444=CARTESIAN_POINT('Ctrl Pts',(38.799008865195,-13.0910137402717,-39.7001053460992));
#20445=CARTESIAN_POINT('Ctrl Pts',(38.8011830809703,-13.0849875486837,-39.6895786502124));
#20446=CARTESIAN_POINT('Ctrl Pts',(38.8012082331003,-13.0849178354768,-39.6894568735118));
#20447=CARTESIAN_POINT('Ctrl Pts',(38.8012333665422,-13.0848481114876,-39.6893350995626));
#20448=CARTESIAN_POINT('Ctrl Pts',(38.8012584813034,-13.0847783767298,-39.6892133283766));
#20449=CARTESIAN_POINT('Ctrl Pts',(38.8063708461711,-13.0705831581647,-39.6644255660912));
#20450=CARTESIAN_POINT('Ctrl Pts',(38.8107403271801,-13.0558793142743,-39.6396345669642));
#20451=CARTESIAN_POINT('Ctrl Pts',(38.8143720370972,-13.0407301262923,-39.6149263152304));
#20452=CARTESIAN_POINT('Ctrl Pts',(38.8198463634219,-13.0178947125452,-39.5776818667505));
#20453=CARTESIAN_POINT('Ctrl Pts',(38.823645519602,-12.9940463246918,-39.5406227563601));
#20454=CARTESIAN_POINT('Ctrl Pts',(38.8257918572288,-12.9693962501975,-39.5040316466717));
#20455=CARTESIAN_POINT('Ctrl Pts',(38.8279381948557,-12.9447461757032,-39.4674405369834));
#20456=CARTESIAN_POINT('Ctrl Pts',(38.8284317229906,-12.9192944015675,-39.4313174373128));
#20457=CARTESIAN_POINT('Ctrl Pts',(38.8272948694351,-12.8932521061511,-39.3959450880251));
#20458=CARTESIAN_POINT('Ctrl Pts',(38.826328746216,-12.8711207892723,-39.3658848856384));
#20459=CARTESIAN_POINT('Ctrl Pts',(38.8242284614393,-12.8485482515867,-39.3363038677842));
#20460=CARTESIAN_POINT('Ctrl Pts',(38.8209322963513,-12.8255048445995,-39.3072258776694));
#20461=CARTESIAN_POINT('Ctrl Pts',(38.819056923723,-12.8123941618594,-39.2906817831558));
#20462=CARTESIAN_POINT('Ctrl Pts',(38.8167936529581,-12.799130872597,-39.2743010308738));
#20463=CARTESIAN_POINT('Ctrl Pts',(38.81412530896,-12.7857088195892,-39.2580927786456));
#20464=CARTESIAN_POINT('Ctrl Pts',(38.8093643068945,-12.7617604747961,-39.2291731481964));
#20465=CARTESIAN_POINT('Ctrl Pts',(38.8033163192104,-12.7373067239541,-39.2008001973807));
#20466=CARTESIAN_POINT('Ctrl Pts',(38.7959160408695,-12.7123167139302,-39.1730000886664));
#20467=CARTESIAN_POINT('Ctrl Pts',(38.7918790162404,-12.6986840799535,-39.1578344802393));
#20468=CARTESIAN_POINT('Ctrl Pts',(38.7874388547392,-12.6848916910894,-39.1428398006197));
#20469=CARTESIAN_POINT('Ctrl Pts',(38.7825797314222,-12.6709337131846,-39.1280242913702));
#20470=CARTESIAN_POINT('',(37.2320718162657,-13.2959337131846,-41.4424668154812));
#20471=CARTESIAN_POINT('Origin',(0.0835265683620477,-13.2959337131846,0.0824317919394229));
#20472=CARTESIAN_POINT('',(37.7005406317231,-14.6753754514262,-42.8699853978345));
#20473=CARTESIAN_POINT('Origin',(-133.456925507265,-671.736420006179,537.350524279956));
#20474=CARTESIAN_POINT('',(48.3955020421714,-14.675375306047,-30.3462213479384));
#20475=CARTESIAN_POINT('Origin',(0.0835265683620477,-14.6753754514262,0.0824317919394229));
#20476=CARTESIAN_POINT('Ctrl Pts',(48.395502411215,-14.6753748699083,-30.3462215803797));
#20477=CARTESIAN_POINT('Ctrl Pts',(48.3970165064124,-14.2165313286484,-29.4828741133762));
#20478=CARTESIAN_POINT('Ctrl Pts',(48.3985257931811,-13.7688961383428,-28.614397690063));
#20479=CARTESIAN_POINT('Ctrl Pts',(48.4000249035474,-13.3339028935805,-27.7401315814044));
#20480=CARTESIAN_POINT('Ctrl Pts',(48.4014813424394,-12.9112915277744,-26.8907510480124));
#20481=CARTESIAN_POINT('Ctrl Pts',(48.4029281735502,-12.5006127529904,-26.0359056762573));
#20482=CARTESIAN_POINT('Ctrl Pts',(48.4043602774117,-12.103139198672,-25.1750154147393));
#20483=CARTESIAN_POINT('Ctrl Pts',(48.4048913764569,-11.9557352073326,-24.855752260564));
#20484=CARTESIAN_POINT('Ctrl Pts',(48.4054204482461,-11.8101469177382,-24.5356580098551));
#20485=CARTESIAN_POINT('Ctrl Pts',(48.4059472256945,-11.6664376689278,-24.2147040460321));
#20486=CARTESIAN_POINT('Ctrl Pts',(48.4060000541633,-11.6520256252871,-24.1825168168067));
#20487=CARTESIAN_POINT('Ctrl Pts',(48.4060528586946,-11.6376325718392,-24.1503208891208));
#20488=CARTESIAN_POINT('Ctrl Pts',(48.4061056388366,-11.6232585917442,-24.118116222714));
#20489=CARTESIAN_POINT('Ctrl Pts',(48.4073722199955,-11.2783218091964,-23.3452910246814));
#20490=CARTESIAN_POINT('Ctrl Pts',(48.4086232798676,-10.9443666880957,-22.567421367977));
#20491=CARTESIAN_POINT('Ctrl Pts',(48.4098496480416,-10.6225428079207,-21.784018721879));
#20492=CARTESIAN_POINT('Ctrl Pts',(48.4102724995876,-10.5115779866166,-21.5139016174983));
#20493=CARTESIAN_POINT('Ctrl Pts',(48.4106924186025,-10.4020550274973,-21.2431269446329));
#20494=CARTESIAN_POINT('Ctrl Pts',(48.4111090387546,-10.2940198074426,-20.971675429716));
#20495=CARTESIAN_POINT('Ctrl Pts',(48.4111340145,-10.2875432600576,-20.9554023236105));
#20496=CARTESIAN_POINT('Ctrl Pts',(48.4111589786261,-10.2810720136184,-20.9391265270569));
#20497=CARTESIAN_POINT('Ctrl Pts',(48.4111839309784,-10.2746060938735,-20.922848081286));
#20498=CARTESIAN_POINT('Ctrl Pts',(48.4118827329214,-10.0935250792971,-20.4669628256337));
#20499=CARTESIAN_POINT('Ctrl Pts',(48.4125729062024,-9.91663263835351,-20.0090368445298));
#20500=CARTESIAN_POINT('Ctrl Pts',(48.4132521719491,-9.74425107303465,-19.5493017432801));
#20501=CARTESIAN_POINT('Ctrl Pts',(48.4139027926854,-9.57913893319766,-19.1089539242711));
#20502=CARTESIAN_POINT('Ctrl Pts',(48.4145434106902,-9.41816464515814,-18.6669448938639));
#20503=CARTESIAN_POINT('Ctrl Pts',(48.4151719180711,-9.26165511783415,-18.2234627935507));
#20504=CARTESIAN_POINT('Ctrl Pts',(48.415435037911,-9.19613359329876,-18.0378023816033));
#20505=CARTESIAN_POINT('Ctrl Pts',(48.4156960335652,-9.13139516041176,-17.851883727953));
#20506=CARTESIAN_POINT('Ctrl Pts',(48.4159547419103,-9.06746659619111,-17.6657206784883));
#20507=CARTESIAN_POINT('Ctrl Pts',(48.4159597463539,-9.06622996466504,-17.6621195480896));
#20508=CARTESIAN_POINT('Ctrl Pts',(48.4159647498858,-9.06499364665102,-17.6585183566049));
#20509=CARTESIAN_POINT('Ctrl Pts',(48.4159697525046,-9.06375764243243,-17.654917104426));
#20510=CARTESIAN_POINT('Ctrl Pts',(48.4171758193888,-8.76577296157743,-16.7867016363302));
#20511=CARTESIAN_POINT('Ctrl Pts',(48.418330759243,-8.48534970203332,-15.9132437322746));
#20512=CARTESIAN_POINT('Ctrl Pts',(48.4194226489004,-8.22405492478902,-15.0341112036849));
#20513=CARTESIAN_POINT('Ctrl Pts',(48.4197035105318,-8.15684330051223,-14.8079760860058));
#20514=CARTESIAN_POINT('Ctrl Pts',(48.4199801982767,-8.09089757124237,-14.5814654555463));
#20515=CARTESIAN_POINT('Ctrl Pts',(48.4202525046535,-8.02624496071548,-14.3545718466408));
#20516=CARTESIAN_POINT('Ctrl Pts',(48.4208747192833,-7.87851503755607,-13.8361244841013));
#20517=CARTESIAN_POINT('Ctrl Pts',(48.4214742831675,-7.73745329660274,-13.315369950669));
#20518=CARTESIAN_POINT('Ctrl Pts',(48.4220479333675,-7.60353311382448,-12.7927342626265));
#20519=CARTESIAN_POINT('Ctrl Pts',(48.4225989655767,-7.47489316188464,-12.2907051554594));
#20520=CARTESIAN_POINT('Ctrl Pts',(48.4231260855195,-7.35284273129863,-11.7869403092735));
#20521=CARTESIAN_POINT('Ctrl Pts',(48.4236265540814,-7.23775611982599,-11.2818266328076));
#20522=CARTESIAN_POINT('Ctrl Pts',(48.4238051253453,-7.19669227839415,-11.1015979541626));
#20523=CARTESIAN_POINT('Ctrl Pts',(48.4239803068534,-7.15651419440814,-10.9211957470908));
#20524=CARTESIAN_POINT('Ctrl Pts',(48.4241519678033,-7.11724012295319,-10.7406508058928));
#20525=CARTESIAN_POINT('Ctrl Pts',(48.4251874613739,-6.88033098026176,-9.65156720309959));
#20526=CARTESIAN_POINT('Ctrl Pts',(48.4260950282616,-6.67627260244589,-8.55708589982596));
#20527=CARTESIAN_POINT('Ctrl Pts',(48.426853401255,-6.50737682457182,-7.45682324763825));
#20528=CARTESIAN_POINT('Ctrl Pts',(48.4276117742484,-6.33848104669775,-6.35656059545055));
#20529=CARTESIAN_POINT('Ctrl Pts',(48.4282209516793,-6.20474805616907,-5.25051655743529));
#20530=CARTESIAN_POINT('Ctrl Pts',(48.4286600676394,-6.10843510301224,-4.13831837467277));
#20531=CARTESIAN_POINT('Origin',(0.0835265683620477,11.4830954176946,0.0824317919394229));
#20532=CARTESIAN_POINT('',(36.0852727571828,-3.61941807409668,-34.1625959873708));
#20533=CARTESIAN_POINT('',(36.0852727571828,11.9341984494201,-34.1625959873708));
#20534=CARTESIAN_POINT('',(36.0852727571828,11.4830954176946,-34.1625959873708));
#20535=CARTESIAN_POINT('',(36.0852727571827,11.9341984494201,34.3274595712498));
#20536=CARTESIAN_POINT('Origin',(0.0835265683620477,11.9341984494201,0.0824317919394229));
#20537=CARTESIAN_POINT('',(36.0852727571827,-3.61941807409668,34.3274595712498));
#20538=CARTESIAN_POINT('',(36.0852727571827,11.4830954176946,34.3274595712498));
#20539=CARTESIAN_POINT('Origin',(0.0835265683620477,-3.61941807409668,0.0824317919394229));
#20540=CARTESIAN_POINT('Origin',(0.0835265683620477,12.0636401876617,0.0824317919394229));
#20541=CARTESIAN_POINT('',(36.7737075413345,13.0346110567824,35.0125232743287));
#20542=CARTESIAN_POINT('',(36.1515914195991,12.155169318541,34.3905421902096));
#20543=CARTESIAN_POINT('',(36.7737075413348,13.0346110567825,35.0125232743285));
#20544=CARTESIAN_POINT('',(36.151591419599,12.1551693185413,-34.2256786063311));
#20545=CARTESIAN_POINT('Origin',(0.0835265683620477,12.1551693185409,0.0824317919394229));
#20546=CARTESIAN_POINT('',(36.7737075413349,13.0346110567825,-34.8476596904496));
#20547=CARTESIAN_POINT('',(36.1515914195989,12.1551693185409,-34.2256786063308));
#20548=CARTESIAN_POINT('',(49.9887116253026,13.0346110567825,-8.62119821111519));
#20549=CARTESIAN_POINT('Origin',(0.0835265683620477,13.0346110567825,0.0824317919394229));
#20550=CARTESIAN_POINT('',(49.9887116253026,13.0346110567825,8.78606179499438));
#20551=CARTESIAN_POINT('Ctrl Pts',(49.9887116253026,13.0346110567825,-8.62119821111519));
#20552=CARTESIAN_POINT('Ctrl Pts',(49.9893478560974,12.8871967548494,-7.75954228903555));
#20553=CARTESIAN_POINT('Ctrl Pts',(49.9899000357746,12.7606786217836,-6.89565773289813));
#20554=CARTESIAN_POINT('Ctrl Pts',(49.9903598055825,12.6558408130361,-6.02947623345575));
#20555=CARTESIAN_POINT('Ctrl Pts',(49.990665808201,12.5860653657491,-5.45298381838726));
#20556=CARTESIAN_POINT('Ctrl Pts',(49.990930885539,12.5258925150002,-4.8754741482685));
#20557=CARTESIAN_POINT('Ctrl Pts',(49.99115267096,12.4755408811194,-4.29692965082524));
#20558=CARTESIAN_POINT('Ctrl Pts',(49.9911538902138,12.4752640756467,-4.29374913272224));
#20559=CARTESIAN_POINT('Ctrl Pts',(49.9911551081487,12.4749875690303,-4.29056855464817));
#20560=CARTESIAN_POINT('Ctrl Pts',(49.9911563247646,12.4747113612848,-4.28738791693494));
#20561=CARTESIAN_POINT('Ctrl Pts',(49.9913179387918,12.4380202039338,-3.86487522247577));
#20562=CARTESIAN_POINT('Ctrl Pts',(49.9914565488923,12.4066244501982,-3.44160145281131));
#20563=CARTESIAN_POINT('Ctrl Pts',(49.9915720324612,12.3805167222718,-3.01783128710948));
#20564=CARTESIAN_POINT('Ctrl Pts',(49.991688629906,12.3541571769569,-2.5899737225819));
#20565=CARTESIAN_POINT('Ctrl Pts',(49.991781653618,12.3331879704902,-2.16160894685783));
#20566=CARTESIAN_POINT('Ctrl Pts',(49.9918507579081,12.3176520559872,-1.73299266868656));
#20567=CARTESIAN_POINT('Ctrl Pts',(49.9919186373041,12.3023915201941,-1.31197374165334));
#20568=CARTESIAN_POINT('Ctrl Pts',(49.9919634378385,12.292373396783,-0.890710996911061));
#20569=CARTESIAN_POINT('Ctrl Pts',(49.9919846138091,12.2876877721247,-0.469448250446118));
#20570=CARTESIAN_POINT('Ctrl Pts',(49.9919938577277,12.2856423625376,-0.285554976195753));
#20571=CARTESIAN_POINT('Ctrl Pts',(49.991998596967,12.2846137392985,-0.101661822245885));
#20572=CARTESIAN_POINT('Ctrl Pts',(49.9919987726311,12.2846124143566,0.0822099968334337));
#20573=CARTESIAN_POINT('Ctrl Pts',(49.9919987763777,12.2846123860983,0.0861316130377299));
#20574=CARTESIAN_POINT('Ctrl Pts',(49.9919987780095,12.2846128251731,0.0900531737555135));
#20575=CARTESIAN_POINT('Ctrl Pts',(49.991998777526,12.2846137316597,0.0939746783873438));
#20576=CARTESIAN_POINT('Ctrl Pts',(49.9919986349354,12.2848811103967,1.25066806982682));
#20577=CARTESIAN_POINT('Ctrl Pts',(49.9918145061858,12.3254286613201,2.40515107505473));
#20578=CARTESIAN_POINT('Ctrl Pts',(49.9914604149175,12.4051717607756,3.55744718045229));
#20579=CARTESIAN_POINT('Ctrl Pts',(49.9913692018685,12.4257133891542,3.85427585328813));
#20580=CARTESIAN_POINT('Ctrl Pts',(49.9912667127974,12.448855628615,4.15095943259262));
#20581=CARTESIAN_POINT('Ctrl Pts',(49.9911531925445,12.4745793828316,4.44749836453926));
#20582=CARTESIAN_POINT('Ctrl Pts',(49.9909438913061,12.522007163138,4.99423750681911));
#20583=CARTESIAN_POINT('Ctrl Pts',(49.990696665258,12.5782201197775,5.54055086955121));
#20584=CARTESIAN_POINT('Ctrl Pts',(49.9904129303823,12.6430432691593,6.08604846635906));
#20585=CARTESIAN_POINT('Ctrl Pts',(49.9901251899494,12.7087815433771,6.6392469910537));
#20586=CARTESIAN_POINT('Ctrl Pts',(49.9897999034691,12.7833747881785,7.19160655594086));
#20587=CARTESIAN_POINT('Ctrl Pts',(49.9894387770557,12.866586934251,7.74272639699184));
#20588=CARTESIAN_POINT('Ctrl Pts',(49.9892105457498,12.9191768752446,8.0910332402735));
#20589=CARTESIAN_POINT('Ctrl Pts',(49.9889680037392,12.9752083234145,8.43884503024982));
#20590=CARTESIAN_POINT('Ctrl Pts',(49.9887116253026,13.0346110567825,8.78606179499438));
#20591=CARTESIAN_POINT('Origin',(0.0835265683620477,13.0346110567825,0.0824317919394229));
#20592=CARTESIAN_POINT('Origin',(0.0835265683622866,-8.56135981233827,-68.3550682080606));
#20593=CARTESIAN_POINT('',(49.7710265683621,-8.56135981233827,-22.6228153633312));
#20594=CARTESIAN_POINT('',(49.7710265683622,-8.56135981233827,-44.2925682080604));
#20595=CARTESIAN_POINT('',(49.7710265683623,-8.56135981233827,-68.3550682080604));
#20596=CARTESIAN_POINT('',(44.4585265683622,-8.56135981233827,-49.6050682080606));
#20597=CARTESIAN_POINT('Origin',(44.4585265683622,-8.56135981233827,-44.2925682080604));
#20598=CARTESIAN_POINT('',(22.7887737236329,-8.56135981233827,-49.6050682080606));
#20599=CARTESIAN_POINT('',(0.0835265683622903,-8.56135981233827,-49.6050682080606));
#20600=CARTESIAN_POINT('',(37.8183782124907,-8.56135981233827,-39.4201868051553));
#20601=CARTESIAN_POINT('Origin',(0.0835265683620477,-8.56135981233827,0.0824317919394229));
#20602=CARTESIAN_POINT('',(38.9743995336223,-8.56135981233827,-40.5762081262869));
#20603=CARTESIAN_POINT('',(39.586145165457,-8.56135981233827,-37.6524198521889));
#20604=CARTESIAN_POINT('',(39.4990275410653,-8.56135981233827,-37.5653022277972));
#20605=CARTESIAN_POINT('Origin',(0.0835265683620477,-8.56135981233827,0.0824317919394229));
#20606=CARTESIAN_POINT('Origin',(0.0835265683622249,13.1261401876617,-50.6675682080606));
#20607=CARTESIAN_POINT('',(11.0320394968432,13.1261401876617,-49.6050682080606));
#20608=CARTESIAN_POINT('',(44.4585265683622,13.1261401876617,-49.6050682080606));
#20609=CARTESIAN_POINT('',(0.0835265683622251,13.1261401876617,-49.6050682080606));
#20610=CARTESIAN_POINT('',(49.7710265683622,13.1261401876617,-44.2925682080604));
#20611=CARTESIAN_POINT('Origin',(44.4585265683622,13.1261401876617,-44.2925682080604));
#20612=CARTESIAN_POINT('',(49.7710265683621,13.1261401876617,-10.8660811365416));
#20613=CARTESIAN_POINT('',(49.7710265683622,13.1261401876617,-50.6675682080604));
#20614=CARTESIAN_POINT('',(36.9337491106658,13.1261401876617,-35.0000237973977));
#20615=CARTESIAN_POINT('Origin',(0.0835265683620477,13.1261401876617,0.0824317919394229));
#20616=CARTESIAN_POINT('',(40.7421664865887,13.1261401876617,-38.8084411733206));
#20617=CARTESIAN_POINT('',(40.7421664865887,13.1261401876617,-38.8084411733205));
#20618=CARTESIAN_POINT('',(38.9743995336223,13.1261401876617,-40.5762081262869));
#20619=CARTESIAN_POINT('Origin',(39.8582830101055,13.1261401876617,-39.6923246498037));
#20620=CARTESIAN_POINT('',(35.1659821576994,13.1261401876617,-36.7677907503641));
#20621=CARTESIAN_POINT('',(35.0791887533698,13.1261401876617,-36.6809973460344));
#20622=CARTESIAN_POINT('Origin',(0.0835265683620477,13.1261401876617,0.0824317919394229));
#20623=CARTESIAN_POINT('Origin',(50.0835265683621,16.4830954176946,0.0824317919395974));
#20624=CARTESIAN_POINT('',(50.083526568362,-8.87385981233827,22.7876789472104));
#20625=CARTESIAN_POINT('',(50.0835265683619,-8.87385981233827,36.6697170232579));
#20626=CARTESIAN_POINT('',(50.0835265683621,-8.87385981233827,0.0824317919395974));
#20627=CARTESIAN_POINT('',(50.0835265683619,-14.4544045823054,36.6697170232579));
#20628=CARTESIAN_POINT('',(50.0835265683619,16.4830954176946,36.6697170232579));
#20629=CARTESIAN_POINT('',(50.0835265683622,-14.4544045823054,-44.2925682080604));
#20630=CARTESIAN_POINT('',(50.0835265683621,-14.4544045823054,0.0824317919395974));
#20631=CARTESIAN_POINT('',(50.0835265683622,-8.87385981233827,-44.2925682080604));
#20632=CARTESIAN_POINT('',(50.0835265683622,16.4830954176946,-44.2925682080604));
#20633=CARTESIAN_POINT('',(50.0835265683621,-8.87385981233827,-22.6228153633312));
#20634=CARTESIAN_POINT('',(50.0835265683621,-8.87385981233827,0.0824317919395974));
#20635=CARTESIAN_POINT('',(50.0835265683621,-8.69080155057986,-21.5378711661598));
#20636=CARTESIAN_POINT('Ctrl Pts',(50.0835265683621,-8.69080155057987,-21.5378711661598));
#20637=CARTESIAN_POINT('Ctrl Pts',(50.0835265683621,-8.73475654613112,-21.6480367600604));
#20638=CARTESIAN_POINT('Ctrl Pts',(50.0835265683621,-8.76821292000551,-21.7616061533008));
#20639=CARTESIAN_POINT('Ctrl Pts',(50.0835265683621,-8.79411643469755,-21.8764708457468));
#20640=CARTESIAN_POINT('Ctrl Pts',(50.0835265683621,-8.80879390138821,-21.9415555540326));
#20641=CARTESIAN_POINT('Ctrl Pts',(50.0835265683621,-8.8210476068989,-22.0070558185655));
#20642=CARTESIAN_POINT('Ctrl Pts',(50.083526568362,-8.83141832822413,-22.0725884285981));
#20643=CARTESIAN_POINT('Ctrl Pts',(50.0835265683619,-8.83143478595685,-22.072692425046));
#20644=CARTESIAN_POINT('Ctrl Pts',(50.0835265683619,-8.83145123875071,-22.0727964220728));
#20645=CARTESIAN_POINT('Ctrl Pts',(50.0835265683619,-8.83146768660594,-22.0729004196781));
#20646=CARTESIAN_POINT('Ctrl Pts',(50.0835265683616,-8.86014040550798,-22.2541942152644));
#20647=CARTESIAN_POINT('Ctrl Pts',(50.0835265683621,-8.87385980853305,-22.4375560999868));
#20648=CARTESIAN_POINT('Ctrl Pts',(50.0835265683621,-8.87385981233827,-22.6228153633312));
#20649=CARTESIAN_POINT('',(50.083526568362,-8.69080155057986,21.702734750039));
#20650=CARTESIAN_POINT('Ctrl Pts',(50.0835265683621,-8.69080155057986,-21.5378711661598));
#20651=CARTESIAN_POINT('Ctrl Pts',(50.0835265683621,-8.34768669240312,-20.6779139118167));
#20652=CARTESIAN_POINT('Ctrl Pts',(50.0835265683621,-8.01980178776899,-19.8131224223239));
#20653=CARTESIAN_POINT('Ctrl Pts',(50.083526568362,-7.7086638179161,-18.9430124229936));
#20654=CARTESIAN_POINT('Ctrl Pts',(50.0835265683619,-7.39752584806321,-18.0729024236633));
#20655=CARTESIAN_POINT('Ctrl Pts',(50.0835265683619,-7.10313511035522,-17.1974737894229));
#20656=CARTESIAN_POINT('Ctrl Pts',(50.083526568362,-6.8269564419545,-16.316264163741));
#20657=CARTESIAN_POINT('Ctrl Pts',(50.083526568362,-6.82354225770081,-16.3053704475622));
#20658=CARTESIAN_POINT('Ctrl Pts',(50.083526568362,-6.82013086172525,-16.294475845857));
#20659=CARTESIAN_POINT('Ctrl Pts',(50.083526568362,-6.81672225716413,-16.2835803575982));
#20660=CARTESIAN_POINT('Ctrl Pts',(50.0835265683622,-6.58377695494992,-15.5389786416461));
#20661=CARTESIAN_POINT('Ctrl Pts',(50.0835265683636,-6.36386066861884,-14.7901976392119));
#20662=CARTESIAN_POINT('Ctrl Pts',(50.0835265683606,-6.15798672711213,-14.0370234161259));
#20663=CARTESIAN_POINT('Ctrl Pts',(50.0835265683601,-6.12185688864097,-13.9048451383818));
#20664=CARTESIAN_POINT('Ctrl Pts',(50.0835265683594,-6.08615941337703,-13.7725316059818));
#20665=CARTESIAN_POINT('Ctrl Pts',(50.0835265683582,-6.05089962282675,-13.6400817274103));
#20666=CARTESIAN_POINT('Ctrl Pts',(50.0835265683581,-6.04778978459125,-13.6283999309435));
#20667=CARTESIAN_POINT('Ctrl Pts',(50.083526568358,-6.0446832728305,-13.6167166878872));
#20668=CARTESIAN_POINT('Ctrl Pts',(50.0835265683579,-6.04158009539427,-13.6050320163313));
#20669=CARTESIAN_POINT('Ctrl Pts',(50.0835265683529,-5.90116651460509,-13.0763202016747));
#20670=CARTESIAN_POINT('Ctrl Pts',(50.0835265683567,-5.76761845986938,-12.5448358405602));
#20671=CARTESIAN_POINT('Ctrl Pts',(50.083526568357,-5.64153128315162,-12.0117275204805));
#20672=CARTESIAN_POINT('Ctrl Pts',(50.0835265683572,-5.55530241465321,-11.647143837792));
#20673=CARTESIAN_POINT('Ctrl Pts',(50.0835265683583,-5.4725636069766,-11.2817995154151));
#20674=CARTESIAN_POINT('Ctrl Pts',(50.0835265683438,-5.39351662111518,-10.916053821918));
#20675=CARTESIAN_POINT('Ctrl Pts',(50.0835265683434,-5.39159586118404,-10.9071665801668));
#20676=CARTESIAN_POINT('Ctrl Pts',(50.0835265683431,-5.38967730441898,-10.898279165744));
#20677=CARTESIAN_POINT('Ctrl Pts',(50.0835265683427,-5.38776095106819,-10.8893915765148));
#20678=CARTESIAN_POINT('Ctrl Pts',(50.0835265681882,-4.60335148320456,-7.25148777604795));
#20679=CARTESIAN_POINT('Ctrl Pts',(50.0835265682258,-4.18752460344888,-3.58097782223435));
#20680=CARTESIAN_POINT('Ctrl Pts',(50.0835265683469,-4.19081815795072,0.126611260712779));
#20681=CARTESIAN_POINT('Ctrl Pts',(50.0835265683471,-4.1908242862358,0.133509935943779));
#20682=CARTESIAN_POINT('Ctrl Pts',(50.0835265683474,-4.19083186535593,0.140408739492022));
#20683=CARTESIAN_POINT('Ctrl Pts',(50.0835265683476,-4.1908408956384,0.147307671387013));
#20684=CARTESIAN_POINT('Ctrl Pts',(50.0835265683765,-4.19204516267736,1.06734049527786));
#20685=CARTESIAN_POINT('Ctrl Pts',(50.0835265683618,-4.21882226363321,1.98963515495041));
#20686=CARTESIAN_POINT('Ctrl Pts',(50.083526568362,-4.27143022964226,2.91421541345035));
#20687=CARTESIAN_POINT('Ctrl Pts',(50.083526568362,-4.27205281679694,2.92515732654982));
#20688=CARTESIAN_POINT('Ctrl Pts',(50.083526568362,-4.27267902824778,2.93609967822935));
#20689=CARTESIAN_POINT('Ctrl Pts',(50.083526568362,-4.27330886465573,2.94704246860311));
#20690=CARTESIAN_POINT('Ctrl Pts',(50.0835265683621,-4.32629862648307,3.86768765251147));
#20691=CARTESIAN_POINT('Ctrl Pts',(50.0835265683618,-4.40442769523305,4.78252778718964));
#20692=CARTESIAN_POINT('Ctrl Pts',(50.0835265683619,-4.50641515619369,5.69168642424652));
#20693=CARTESIAN_POINT('Ctrl Pts',(50.0835265683619,-4.50797212337508,5.70556587714443));
#20694=CARTESIAN_POINT('Ctrl Pts',(50.0835265683619,-4.50953465011834,5.71944400116706));
#20695=CARTESIAN_POINT('Ctrl Pts',(50.0835265683619,-4.51110273180188,5.73332079645939));
#20696=CARTESIAN_POINT('Ctrl Pts',(50.083526568362,-4.63310585043406,6.81299178557852));
#20697=CARTESIAN_POINT('Ctrl Pts',(50.083526568362,-4.78875206538555,7.88473847945899));
#20698=CARTESIAN_POINT('Ctrl Pts',(50.0835265683619,-4.97573014435409,8.94910172276016));
#20699=CARTESIAN_POINT('Ctrl Pts',(50.0835265683619,-5.104928022985,9.68455410244992));
#20700=CARTESIAN_POINT('Ctrl Pts',(50.0835265683619,-5.24908423887366,10.4164815427171));
#20701=CARTESIAN_POINT('Ctrl Pts',(50.0835265683619,-5.40742232363258,11.1450662553477));
#20702=CARTESIAN_POINT('Ctrl Pts',(50.0835265683619,-5.4105998810796,11.159687625708));
#20703=CARTESIAN_POINT('Ctrl Pts',(50.0835265683619,-5.41378314936642,11.1743076488218));
#20704=CARTESIAN_POINT('Ctrl Pts',(50.0835265683619,-5.41697212217387,11.1889263261959));
#20705=CARTESIAN_POINT('Ctrl Pts',(50.083526568362,-5.65900900139522,12.2984557150021));
#20706=CARTESIAN_POINT('Ctrl Pts',(50.083526568362,-5.9337967445744,13.4002686430632));
#20707=CARTESIAN_POINT('Ctrl Pts',(50.083526568362,-6.23869144824832,14.4949862172741));
#20708=CARTESIAN_POINT('Ctrl Pts',(50.083526568362,-6.54852480772613,15.6074359240422));
#20709=CARTESIAN_POINT('Ctrl Pts',(50.083526568362,-6.88944821129976,16.7125585971452));
#20710=CARTESIAN_POINT('Ctrl Pts',(50.083526568362,-7.25863482935653,17.8110201816428));
#20711=CARTESIAN_POINT('Ctrl Pts',(50.083526568362,-7.63718691654914,18.9373473700475));
#20712=CARTESIAN_POINT('Ctrl Pts',(50.083526568362,-8.04545424387804,20.056671259519));
#20713=CARTESIAN_POINT('Ctrl Pts',(50.083526568362,-8.48033670889165,21.1697240178476));
#20714=CARTESIAN_POINT('Ctrl Pts',(50.083526568362,-8.54981664757972,21.3475533019114));
#20715=CARTESIAN_POINT('Ctrl Pts',(50.083526568362,-8.61997584800288,21.5252225401305));
#20716=CARTESIAN_POINT('Ctrl Pts',(50.083526568362,-8.69080155057986,21.7027347500389));
#20717=CARTESIAN_POINT('Ctrl Pts',(50.083526568362,-8.87385981233827,22.7876789472104));
#20718=CARTESIAN_POINT('Ctrl Pts',(50.083526568362,-8.87385981188611,22.717742516166));
#20719=CARTESIAN_POINT('Ctrl Pts',(50.083526568362,-8.87185808464315,22.6477745033947));
#20720=CARTESIAN_POINT('Ctrl Pts',(50.0835265683619,-8.86782837150229,22.5779796471447));
#20721=CARTESIAN_POINT('Ctrl Pts',(50.0835265683618,-8.86373626040434,22.507104054799));
#20722=CARTESIAN_POINT('Ctrl Pts',(50.0835265683618,-8.85755327620425,22.4364053802177));
#20723=CARTESIAN_POINT('Ctrl Pts',(50.0835265683588,-8.84920383564881,22.3660776681213));
#20724=CARTESIAN_POINT('Ctrl Pts',(50.0835265683569,-8.84406583764724,22.3228000806222));
#20725=CARTESIAN_POINT('Ctrl Pts',(50.0835265683538,-8.83810648050989,22.2796626723357));
#20726=CARTESIAN_POINT('Ctrl Pts',(50.0835265683476,-8.83129827231312,22.2367110515669));
#20727=CARTESIAN_POINT('Ctrl Pts',(50.0835265683475,-8.83124617212743,22.2363823619392));
#20728=CARTESIAN_POINT('Ctrl Pts',(50.0835265683475,-8.83119402657744,22.2360536803506));
#20729=CARTESIAN_POINT('Ctrl Pts',(50.0835265683474,-8.83114183558509,22.235725006798));
#20730=CARTESIAN_POINT('Ctrl Pts',(50.0835265683309,-8.81326914157238,22.1231714497214));
#20731=CARTESIAN_POINT('Ctrl Pts',(50.0835265683519,-8.79011900704274,22.011837783367));
#20732=CARTESIAN_POINT('Ctrl Pts',(50.0835265683584,-8.75874571255292,21.9024044661432));
#20733=CARTESIAN_POINT('Ctrl Pts',(50.0835265683624,-8.73944301755183,21.8350746565177));
#20734=CARTESIAN_POINT('Ctrl Pts',(50.083526568362,-8.71702701275813,21.7684643500544));
#20735=CARTESIAN_POINT('Ctrl Pts',(50.083526568362,-8.69080155058071,21.7027347500411));
#20736=CARTESIAN_POINT('Origin',(44.4585265683622,16.4830954176946,-44.2925682080604));
#20737=CARTESIAN_POINT('Origin',(44.4585265683622,-8.87385981233827,-44.2925682080604));
#20738=CARTESIAN_POINT('Origin',(44.4585265683622,-14.4544045823054,-44.2925682080604));
#20739=CARTESIAN_POINT('Origin',(50.0835265683621,16.4830954176946,0.0824317919395974));
#20740=CARTESIAN_POINT('',(50.0835265683622,16.1705954176946,-44.2925682080604));
#20741=CARTESIAN_POINT('',(50.0835265683619,16.1705954176946,36.6697170232579));
#20742=CARTESIAN_POINT('',(50.0835265683619,16.1705954176946,44.4574317919394));
#20743=CARTESIAN_POINT('',(50.0835265683619,13.4386401876617,36.6697170232579));
#20744=CARTESIAN_POINT('',(50.0835265683619,16.4830954176946,36.6697170232579));
#20745=CARTESIAN_POINT('',(50.083526568362,13.4386401876617,11.0309447204208));
#20746=CARTESIAN_POINT('',(50.0835265683621,13.4386401876617,0.0824317919395974));
#20747=CARTESIAN_POINT('',(50.083526568362,13.2555819259033,8.74809679815803));
#20748=CARTESIAN_POINT('Ctrl Pts',(50.083526568362,13.2555819259033,8.74809679815823));
#20749=CARTESIAN_POINT('Ctrl Pts',(50.083526568362,13.2969611279801,8.98893971344353));
#20750=CARTESIAN_POINT('Ctrl Pts',(50.083526568362,13.3294628820991,9.23096941458519));
#20751=CARTESIAN_POINT('Ctrl Pts',(50.083526568362,13.3553162053205,9.47374987915283));
#20752=CARTESIAN_POINT('Ctrl Pts',(50.083526568362,13.3699153107393,9.61084550765334));
#20753=CARTESIAN_POINT('Ctrl Pts',(50.083526568362,13.3823932020092,9.74818076138043));
#20754=CARTESIAN_POINT('Ctrl Pts',(50.083526568362,13.3931443825075,9.88567820112658));
#20755=CARTESIAN_POINT('Ctrl Pts',(50.083526568362,13.3931495855304,9.88574474287337));
#20756=CARTESIAN_POINT('Ctrl Pts',(50.083526568362,13.3931547881236,9.88581128464174));
#20757=CARTESIAN_POINT('Ctrl Pts',(50.083526568362,13.3931599902869,9.8858778264317));
#20758=CARTESIAN_POINT('Ctrl Pts',(50.083526568362,13.4229505456848,10.2669340808595));
#20759=CARTESIAN_POINT('Ctrl Pts',(50.083526568362,13.4386401851025,10.6486001469402));
#20760=CARTESIAN_POINT('Ctrl Pts',(50.083526568362,13.4386401876617,11.0309447204208));
#20761=CARTESIAN_POINT('',(50.0835265683621,13.2555819259033,-8.58323321427883));
#20762=CARTESIAN_POINT('Ctrl Pts',(50.083526568362,13.2555819259033,8.74809679815803));
#20763=CARTESIAN_POINT('Ctrl Pts',(50.083526568362,13.0482120855562,7.54112464899445));
#20764=CARTESIAN_POINT('Ctrl Pts',(50.083526568362,12.8826695792778,6.33137948099875));
#20765=CARTESIAN_POINT('Ctrl Pts',(50.083526568362,12.760436564522,5.11876132513915));
#20766=CARTESIAN_POINT('Ctrl Pts',(50.083526568362,12.6392785940108,3.91680819437184));
#20767=CARTESIAN_POINT('Ctrl Pts',(50.083526568362,12.560671682904,2.7120323854556));
#20768=CARTESIAN_POINT('Ctrl Pts',(50.083526568362,12.5260083297323,1.50434227373321));
#20769=CARTESIAN_POINT('Ctrl Pts',(50.083526568362,12.5125314172724,1.03479930038698));
#20770=CARTESIAN_POINT('Ctrl Pts',(50.083526568362,12.5056965050864,0.564815860197846));
#20771=CARTESIAN_POINT('Ctrl Pts',(50.0835265683621,12.5055833090018,0.0943868073395787));
#20772=CARTESIAN_POINT('Ctrl Pts',(50.0835265683621,12.5055832718468,0.0942323956936116));
#20773=CARTESIAN_POINT('Ctrl Pts',(50.083526568362,12.5055832354158,0.0940779840217097));
#20774=CARTESIAN_POINT('Ctrl Pts',(50.083526568362,12.505583199709,0.0939235723238649));
#20775=CARTESIAN_POINT('Ctrl Pts',(50.083526568362,12.5054760332769,-0.369510401693673));
#20776=CARTESIAN_POINT('Ctrl Pts',(50.0835265683624,12.5119501585697,-0.833607667675453));
#20777=CARTESIAN_POINT('Ctrl Pts',(50.0835265683571,12.5248910213244,-1.2978410246897));
#20778=CARTESIAN_POINT('Ctrl Pts',(50.0835265683517,12.537901838647,-1.76458389320593));
#20779=CARTESIAN_POINT('Ctrl Pts',(50.0835265683393,12.5574495854738,-2.23146564927433));
#20780=CARTESIAN_POINT('Ctrl Pts',(50.0835265683302,12.5834701483639,-2.69795234473062));
#20781=CARTESIAN_POINT('Ctrl Pts',(50.0835265683213,12.6088446209642,-3.15285618067797));
#20782=CARTESIAN_POINT('Ctrl Pts',(50.0835265683192,12.6403747667627,-3.60738548981518));
#20783=CARTESIAN_POINT('Ctrl Pts',(50.0835265683316,12.6780474220394,-4.06102862482723));
#20784=CARTESIAN_POINT('Ctrl Pts',(50.0835265683335,12.6835738954316,-4.12757680670609));
#20785=CARTESIAN_POINT('Ctrl Pts',(50.0835265683355,12.6892326346535,-4.19410587081538));
#20786=CARTESIAN_POINT('Ctrl Pts',(50.0835265683378,12.6950236788078,-4.26061414818264));
#20787=CARTESIAN_POINT('Ctrl Pts',(50.083526568338,12.6955171094319,-4.26628104001408));
#20788=CARTESIAN_POINT('Ctrl Pts',(50.0835265683381,12.6960114970034,-4.27194774229855));
#20789=CARTESIAN_POINT('Ctrl Pts',(50.0835265683383,12.6965068414371,-4.27761425314022));
#20790=CARTESIAN_POINT('Ctrl Pts',(50.0835265683662,12.7706053471226,-5.12526683034168));
#20791=CARTESIAN_POINT('Ctrl Pts',(50.0835265683616,12.865971940895,-5.97068200817664));
#20792=CARTESIAN_POINT('Ctrl Pts',(50.083526568362,12.9818931825585,-6.81390647641708));
#20793=CARTESIAN_POINT('Ctrl Pts',(50.0835265683622,13.0631188030526,-7.40475099866104));
#20794=CARTESIAN_POINT('Ctrl Pts',(50.0835265683621,13.1544351593156,-7.99452016890981));
#20795=CARTESIAN_POINT('Ctrl Pts',(50.0835265683621,13.2555819259033,-8.58323321427884));
#20796=CARTESIAN_POINT('',(50.0835265683621,13.4386401876617,-10.8660811365416));
#20797=CARTESIAN_POINT('Ctrl Pts',(50.0835265683621,13.4386401876617,-10.8660811365416));
#20798=CARTESIAN_POINT('Ctrl Pts',(50.0835265683621,13.4386401861139,-10.6249936669031));
#20799=CARTESIAN_POINT('Ctrl Pts',(50.0835265683622,13.4323889945138,-10.3840575949856));
#20800=CARTESIAN_POINT('Ctrl Pts',(50.083526568362,13.4203066131559,-10.1434070400552));
#20801=CARTESIAN_POINT('Ctrl Pts',(50.0835265683619,13.4132400183933,-10.002658300158));
#20802=CARTESIAN_POINT('Ctrl Pts',(50.0835265683617,13.4041776979157,-9.86200706428455));
#20803=CARTESIAN_POINT('Ctrl Pts',(50.0835265683608,13.393195553816,-9.72147949723203));
#20804=CARTESIAN_POINT('Ctrl Pts',(50.0835265683608,13.3931761734939,-9.72123150654036));
#20805=CARTESIAN_POINT('Ctrl Pts',(50.0835265683608,13.3931567875857,-9.72098351656411));
#20806=CARTESIAN_POINT('Ctrl Pts',(50.0835265683608,13.3931373960889,-9.72073552730331));
#20807=CARTESIAN_POINT('Ctrl Pts',(50.0835265683585,13.3633415593949,-9.33968977198554));
#20808=CARTESIAN_POINT('Ctrl Pts',(50.0835265683621,13.320346515891,-8.96018808653365));
#20809=CARTESIAN_POINT('Ctrl Pts',(50.0835265683621,13.2555819259033,-8.58323321427883));
#20810=CARTESIAN_POINT('',(50.0835265683622,13.4386401876617,-44.2925682080604));
#20811=CARTESIAN_POINT('',(50.0835265683621,13.4386401876617,0.0824317919395974));
#20812=CARTESIAN_POINT('',(50.0835265683622,16.4830954176946,-44.2925682080604));
#20813=CARTESIAN_POINT('Origin',(44.4585265683622,16.4830954176946,-44.2925682080604));
#20814=CARTESIAN_POINT('Origin',(44.4585265683622,13.4386401876617,-44.2925682080604));
#20815=CARTESIAN_POINT('Origin',(44.4585265683622,16.1705954176946,-44.2925682080604));
#20816=CARTESIAN_POINT('Origin',(0.0835265683620477,16.4830954176946,0.0824317919394229));
#20817=CARTESIAN_POINT('',(22.6771142305789,16.3915662868157,-48.242741818912));
#20818=CARTESIAN_POINT('',(4.30427685447661,11.5746245485365,-48.2627017315535));
#20819=CARTESIAN_POINT('Ctrl Pts',(22.677114230578,16.3915662868154,-48.2427418189112));
#20820=CARTESIAN_POINT('Ctrl Pts',(19.7455070706072,15.1541680928392,-48.2474043029498));
#20821=CARTESIAN_POINT('Ctrl Pts',(16.756896605017,14.0894359483377,-48.2517517721786));
#20822=CARTESIAN_POINT('Ctrl Pts',(12.1565558613288,12.8480220597895,-48.257033362324));
#20823=CARTESIAN_POINT('Ctrl Pts',(10.6007498763966,12.4934998941785,-48.2585854301897));
#20824=CARTESIAN_POINT('Ctrl Pts',(7.46946850957225,11.9258476364964,-48.261105456389));
#20825=CARTESIAN_POINT('Ctrl Pts',(5.89096210505037,11.7120008366799,-48.2620757256809));
#20826=CARTESIAN_POINT('Ctrl Pts',(4.30427685533896,11.5746245485739,-48.2627017315157));
#20827=CARTESIAN_POINT('',(48.4286600918519,11.5746245485739,-4.13831849464002));
#20828=CARTESIAN_POINT('Origin',(0.0835265683620477,11.5746245485739,0.0824317919394229));
#20829=CARTESIAN_POINT('',(48.4087001792128,16.3915662868156,-22.5111558702767));
#20830=CARTESIAN_POINT('Ctrl Pts',(48.4286600918172,11.5746245485739,-4.13831849503729));
#20831=CARTESIAN_POINT('Ctrl Pts',(48.4280346394369,11.7118793817134,-5.72360094950246));
#20832=CARTESIAN_POINT('Ctrl Pts',(48.4270679171629,11.9249456441311,-7.29678813530604));
#20833=CARTESIAN_POINT('Ctrl Pts',(48.4245562772761,12.4906656417943,-10.4208921803695));
#20834=CARTESIAN_POINT('Ctrl Pts',(48.4230091974657,12.8439804579761,-11.9740784049424));
#20835=CARTESIAN_POINT('Ctrl Pts',(48.4177256478359,14.0856585112706,-16.5800021649963));
#20836=CARTESIAN_POINT('Ctrl Pts',(48.4133613504756,15.1545164964592,-19.5803741378453));
#20837=CARTESIAN_POINT('Ctrl Pts',(48.4087001792127,16.3915662868154,-22.5111558702763));
#20838=CARTESIAN_POINT('Origin',(0.0835265683620477,16.3915662868154,0.0824317919394229));
#20839=CARTESIAN_POINT('Origin',(48.5210265683621,-85.4775827009602,0.0824317919395913));
#20840=CARTESIAN_POINT('',(48.521026568362,11.7955954176946,4.28396341998253));
#20841=CARTESIAN_POINT('',(48.5210265683621,11.6131136241746,0.0824317919395203));
#20842=CARTESIAN_POINT('Origin',(48.5210265683762,84.3502669988373,0.0808847077731101));
#20843=CARTESIAN_POINT('',(48.5210265682489,16.1706033824536,21.518168778977));
#20844=CARTESIAN_POINT('Ctrl Pts',(48.5210265683619,11.7955954176945,4.28396341998253));
#20845=CARTESIAN_POINT('Ctrl Pts',(48.5210265683581,11.9012754513054,5.49904346048471));
#20846=CARTESIAN_POINT('Ctrl Pts',(48.5210265682208,12.0520583741837,6.7088076511187));
#20847=CARTESIAN_POINT('Ctrl Pts',(48.5210265682647,12.245534037766,7.91354042332108));
#20848=CARTESIAN_POINT('Ctrl Pts',(48.5210265682742,12.2874241519058,8.17438146348642));
#20849=CARTESIAN_POINT('Ctrl Pts',(48.5210265682907,12.3313158156439,8.43498661765798));
#20850=CARTESIAN_POINT('Ctrl Pts',(48.5210265683094,12.3771848834538,8.69535873608156));
#20851=CARTESIAN_POINT('Ctrl Pts',(48.521026568315,12.3910255799873,8.77392435009892));
#20852=CARTESIAN_POINT('Ctrl Pts',(48.5210265683122,12.4050450140625,8.85246436981573));
#20853=CARTESIAN_POINT('Ctrl Pts',(48.5210265682998,12.4192427232413,8.93097996771382));
#20854=CARTESIAN_POINT('Ctrl Pts',(48.521026568213,12.5191317203718,9.48338206543068));
#20855=CARTESIAN_POINT('Ctrl Pts',(48.5210265673562,12.6280707956221,10.0352897380736));
#20856=CARTESIAN_POINT('Ctrl Pts',(48.5210265620527,12.7454889374133,10.5858637901934));
#20857=CARTESIAN_POINT('Ctrl Pts',(48.5210265566114,12.8659559514214,11.150734014142));
#20858=CARTESIAN_POINT('Ctrl Pts',(48.5210265462836,12.9953485173926,11.714201755527));
#20859=CARTESIAN_POINT('Ctrl Pts',(48.5210265443164,13.1331031832496,12.2753514078195));
#20860=CARTESIAN_POINT('Ctrl Pts',(48.5210265433988,13.1973553945139,12.5370855987138));
#20861=CARTESIAN_POINT('Ctrl Pts',(48.5210265445818,13.2634275010315,12.7983152304055));
#20862=CARTESIAN_POINT('Ctrl Pts',(48.5210265481732,13.3312657045515,13.0589454818311));
#20863=CARTESIAN_POINT('Ctrl Pts',(48.521026550869,13.382187770071,13.2545849600426));
#20864=CARTESIAN_POINT('Ctrl Pts',(48.521026553119,13.4341067575158,13.4499116170473));
#20865=CARTESIAN_POINT('Ctrl Pts',(48.5210265550302,13.4869947668864,13.6448649932951));
#20866=CARTESIAN_POINT('Ctrl Pts',(48.5210265629102,13.705058467528,14.4486814950525));
#20867=CARTESIAN_POINT('Ctrl Pts',(48.5210265653827,13.9395350033909,15.2473465102858));
#20868=CARTESIAN_POINT('Ctrl Pts',(48.5210265667497,14.1892982824036,16.0411553774744));
#20869=CARTESIAN_POINT('Ctrl Pts',(48.5210265681412,14.4435598429467,16.8492608849858));
#20870=CARTESIAN_POINT('Ctrl Pts',(48.5210265682269,14.7136635664295,17.6523337933097));
#20871=CARTESIAN_POINT('Ctrl Pts',(48.5210265683088,14.998370752621,18.4507061044753));
#20872=CARTESIAN_POINT('Ctrl Pts',(48.5210265683931,15.2915959449578,19.2729645013546));
#20873=CARTESIAN_POINT('Ctrl Pts',(48.5210265683619,15.600311376782,20.0902368738228));
#20874=CARTESIAN_POINT('Ctrl Pts',(48.521026568362,15.9231126709056,20.9029067079027));
#20875=CARTESIAN_POINT('Ctrl Pts',(48.521026568362,16.004689947692,21.1082819439924));
#20876=CARTESIAN_POINT('Ctrl Pts',(48.521026568362,16.0871665859128,21.3133633340306));
#20877=CARTESIAN_POINT('Ctrl Pts',(48.521026568362,16.1705194395551,21.5181572619665));
#20878=CARTESIAN_POINT('',(48.5210265682481,16.1706033612914,-21.3533050824651));
#20879=CARTESIAN_POINT('',(48.5210265683621,16.1705954176946,0.0824317919395913));
#20880=CARTESIAN_POINT('',(48.5210265683621,11.7955954176946,-4.11909983610349));
#20881=CARTESIAN_POINT('Ctrl Pts',(48.5210265683621,16.1705196413332,-21.3532935961081));
#20882=CARTESIAN_POINT('Ctrl Pts',(48.5210265683621,15.8435202227035,-20.5498711716006));
#20883=CARTESIAN_POINT('Ctrl Pts',(48.5210265683753,15.5300086684673,-19.7420199101728));
#20884=CARTESIAN_POINT('Ctrl Pts',(48.5210265683489,15.2313679633776,-18.9293681492881));
#20885=CARTESIAN_POINT('Ctrl Pts',(48.521026568323,14.9390610384528,-18.1339516731999));
#20886=CARTESIAN_POINT('Ctrl Pts',(48.5210265683458,14.661001060326,-17.3339360822784));
#20887=CARTESIAN_POINT('Ctrl Pts',(48.5210265675901,14.3984390227961,-16.5289914655286));
#20888=CARTESIAN_POINT('Ctrl Pts',(48.5210265668539,14.1426624798295,-15.7448493508167));
#20889=CARTESIAN_POINT('Ctrl Pts',(48.5210265655117,13.9015932979829,-14.9560296549517));
#20890=CARTESIAN_POINT('Ctrl Pts',(48.5210265604243,13.6763418780025,-14.162246017455));
#20891=CARTESIAN_POINT('Ctrl Pts',(48.5210265589699,13.6119483517376,-13.9353239074224));
#20892=CARTESIAN_POINT('Ctrl Pts',(48.521026557187,13.5488472151597,-13.7079962448028));
#20893=CARTESIAN_POINT('Ctrl Pts',(48.5210265549389,13.4870636734946,-13.4802566325191));
#20894=CARTESIAN_POINT('Ctrl Pts',(48.5210265530145,13.43417513047,-13.2853047738518));
#20895=CARTESIAN_POINT('Ctrl Pts',(48.5210265507489,13.3822549873809,-13.0899772433496));
#20896=CARTESIAN_POINT('Ctrl Pts',(48.5210265480343,13.3313312754876,-12.8943348440505));
#20897=CARTESIAN_POINT('Ctrl Pts',(48.521026540269,13.1856558716782,-12.334668542036));
#20898=CARTESIAN_POINT('Ctrl Pts',(48.521026545501,13.0481153498219,-11.7722163782289));
#20899=CARTESIAN_POINT('Ctrl Pts',(48.521026552699,12.9192577967369,-11.207918578878));
#20900=CARTESIAN_POINT('Ctrl Pts',(48.5210265597492,12.7930466642987,-10.6552100834632));
#20901=CARTESIAN_POINT('Ctrl Pts',(48.5210265658216,12.6751650327471,-10.1007297054743));
#20902=CARTESIAN_POINT('Ctrl Pts',(48.5210265674002,12.5661734819284,-9.54534356437002));
#20903=CARTESIAN_POINT('Ctrl Pts',(48.5210265681379,12.5152460170547,-9.28583346491732));
#20904=CARTESIAN_POINT('Ctrl Pts',(48.5210265682585,12.4662602454938,-9.02612547553568));
#20905=CARTESIAN_POINT('Ctrl Pts',(48.5210265682996,12.4192773203291,-8.76630779101686));
#20906=CARTESIAN_POINT('Ctrl Pts',(48.521026568312,12.4050773744288,-8.68778145296586));
#20907=CARTESIAN_POINT('Ctrl Pts',(48.5210265683148,12.3910557938721,-8.60923092228166));
#20908=CARTESIAN_POINT('Ctrl Pts',(48.5210265683092,12.3772130393344,-8.53065503615693));
#20909=CARTESIAN_POINT('Ctrl Pts',(48.5210265682229,12.1658567976611,-7.33092965402482));
#20910=CARTESIAN_POINT('Ctrl Pts',(48.5210265682964,11.996481850192,-6.12627208137987));
#20911=CARTESIAN_POINT('Ctrl Pts',(48.521026568344,11.8714667055606,-4.91640245756147));
#20912=CARTESIAN_POINT('Ctrl Pts',(48.5210265683544,11.8440311392596,-4.65088696039834));
#20913=CARTESIAN_POINT('Ctrl Pts',(48.5210265683611,11.8187322178908,-4.38512041878988));
#20914=CARTESIAN_POINT('Ctrl Pts',(48.521026568362,11.7955954176946,-4.11909983610349));
#20915=CARTESIAN_POINT('Origin',(48.5210265743749,84.3502669996413,0.0839788824233628));
#20916=CARTESIAN_POINT('Origin',(41.1841082248303,16.4855954176946,-39.6923246498037));
#20917=CARTESIAN_POINT('',(36.0907279647213,-3.61941807409669,-34.5989443896948));
#20918=CARTESIAN_POINT('',(39.3651742963362,-8.24885981233827,-37.8733907213097));
#20919=CARTESIAN_POINT('Ctrl Pts',(36.0907279647213,-3.61941807409669,-34.5989443896948));
#20920=CARTESIAN_POINT('Ctrl Pts',(36.637239178152,-4.3920600802535,-35.1454556031255));
#20921=CARTESIAN_POINT('Ctrl Pts',(37.1837464394694,-5.16470767732064,-35.6919628644429));
#20922=CARTESIAN_POINT('Ctrl Pts',(38.2752282249955,-6.70785538323104,-36.783444649969));
#20923=CARTESIAN_POINT('Ctrl Pts',(38.8202027672248,-7.4783554666459,-37.3284191921982));
#20924=CARTESIAN_POINT('Ctrl Pts',(39.3651742963362,-8.24885981233827,-37.8733907213097));
#20925=CARTESIAN_POINT('',(40.5211956174679,-8.24885981233827,-39.0294120424414));
#20926=CARTESIAN_POINT('',(36.712778241545,12.8136401876617,-35.2209946665185));
#20927=CARTESIAN_POINT('',(36.6259848372153,12.8136401876617,-35.1342012621888));
#20928=CARTESIAN_POINT('',(36.0907279647213,11.9341984494202,-34.5989443896948));
#20929=CARTESIAN_POINT('',(36.712778241545,12.8136401876617,-35.2209946665185));
#20930=CARTESIAN_POINT('',(36.0907279647213,-3.74885981233827,-34.5989443896948));
#20931=CARTESIAN_POINT('Origin',(39.8582830101055,16.4855954176946,-41.0181498645285));
#20932=CARTESIAN_POINT('',(38.0393490816115,-8.24885981233827,-39.1992159360345));
#20933=CARTESIAN_POINT('',(37.9522314572197,-8.24885981233827,-39.1120983116427));
#20934=CARTESIAN_POINT('Ctrl Pts',(38.0393490816115,-8.24885981233827,-39.1992159360345));
#20935=CARTESIAN_POINT('Ctrl Pts',(37.4943775525,-7.4783554666459,-38.654244406923));
#20936=CARTESIAN_POINT('Ctrl Pts',(36.9494030102707,-6.70785538323103,-38.1092698646938));
#20937=CARTESIAN_POINT('Ctrl Pts',(35.8579212247446,-5.16470767732064,-37.0177880791676));
#20938=CARTESIAN_POINT('Ctrl Pts',(35.3114139634272,-4.39206008025349,-36.4712808178503));
#20939=CARTESIAN_POINT('Ctrl Pts',(34.7649027499965,-3.61941807409669,-35.9247696044196));
#20940=CARTESIAN_POINT('',(35.3869530268202,12.8136401876617,-36.5468198812432));
#20941=CARTESIAN_POINT('',(34.7649027499965,11.9341984494202,-35.9247696044196));
#20942=CARTESIAN_POINT('',(39.1953704027431,12.8136401876617,-40.3552372571661));
#20943=CARTESIAN_POINT('Origin',(0.0835265683620477,-11.0169045823054,0.0824317919394229));
#20944=CARTESIAN_POINT('',(19.5475193794832,-11.3294045823054,-9.90098490018674));
#20945=CARTESIAN_POINT('',(19.5475193794832,-11.0169045823054,-9.90098490018674));
#20946=CARTESIAN_POINT('Origin',(0.0835265683620477,-14.4544045823054,0.0824317919394229));
#20947=CARTESIAN_POINT('Origin',(0.0835265683620477,-11.3294045823054,0.0824317919394229));
#20948=CARTESIAN_POINT('Origin',(0.0835265683620477,-13.2044045823054,0.0824317919394229));
#20949=CARTESIAN_POINT('',(34.7488729746945,-13.2044045823054,-34.1940362076806));
#20950=CARTESIAN_POINT('',(37.084741276154,-13.2044045823054,-41.2777797274919));
#20951=CARTESIAN_POINT('',(37.1711692825102,-13.2044045823054,-41.5398809039896));
#20952=CARTESIAN_POINT('',(38.3461436957037,-13.2044045823054,-40.1137013224621));
#20953=CARTESIAN_POINT('Origin',(0.0835265683620477,-13.2044045823054,0.0824317919394229));
#20954=CARTESIAN_POINT('',(35.9713494567465,-13.2044045823054,-32.9119111827578));
#20955=CARTESIAN_POINT('',(22.6388808156566,-13.2044045823054,7.52007219592841));
#20956=CARTESIAN_POINT('Origin',(0.0835265683620477,-13.2044045823054,0.0824317919394229));
#20957=CARTESIAN_POINT('Origin',(22.9356617925947,16.4855954176946,7.61793588545459));
#20958=CARTESIAN_POINT('',(36.2681304336846,-12.8919045823054,-32.8140474932316));
#20959=CARTESIAN_POINT('',(38.3305777332763,-12.8919045823054,-39.0686157342182));
#20960=CARTESIAN_POINT('',(22.9356617925947,-12.8919045823054,7.61793588545459));
#20961=CARTESIAN_POINT('',(36.2681294096903,-7.07886051013668,-32.8140443877542));
#20962=CARTESIAN_POINT('Ctrl Pts',(38.3305777332763,-12.8919045823054,-39.0686157342182));
#20963=CARTESIAN_POINT('Ctrl Pts',(37.7859832182751,-11.3339023356853,-37.4170809006171));
#20964=CARTESIAN_POINT('Ctrl Pts',(37.2389106772517,-9.78474033348405,-35.7580312166432));
#20965=CARTESIAN_POINT('Ctrl Pts',(36.688444321157,-8.24794399815022,-34.0886894646172));
#20966=CARTESIAN_POINT('Ctrl Pts',(36.5485654401618,-7.85742902966216,-33.6644934103323));
#20967=CARTESIAN_POINT('Ctrl Pts',(36.4084673618567,-7.46771271895524,-33.2396326192889));
#20968=CARTESIAN_POINT('Ctrl Pts',(36.2681349390778,-7.07885337126685,-32.8140611562666));
#20969=CARTESIAN_POINT('',(36.2681304336846,16.4855954176946,-32.8140474932316));
#20970=CARTESIAN_POINT('Origin',(0.0835265683620477,-13.2044045823054,0.0824317919394229));
#20971=CARTESIAN_POINT('',(28.0161439142367,-13.2044045823054,-39.8716842439453));
#20972=CARTESIAN_POINT('',(30.2097727145137,-13.2044045823054,-46.5240729034966));
#20973=CARTESIAN_POINT('',(30.2768410701833,-13.2044045823054,-46.7274640919305));
#20974=CARTESIAN_POINT('',(31.5582959274376,-13.2044045823054,-45.624196617704));
#20975=CARTESIAN_POINT('Origin',(0.0835265683620477,-13.2044045823054,0.0824317919394229));
#20976=CARTESIAN_POINT('',(29.344152791651,-13.2044045823054,-38.9095962781799));
#20977=CARTESIAN_POINT('',(14.8778438489026,-13.2044045823054,4.96086600976507));
#20978=CARTESIAN_POINT('Origin',(0.0835265683620477,-13.2044045823054,0.0824317919394229));
#20979=CARTESIAN_POINT('Origin',(13.0971579872741,16.4855954176946,4.37368387260805));
#20980=CARTESIAN_POINT('',(27.7193629372986,-12.8919045823054,-39.9695479334715));
#20981=CARTESIAN_POINT('',(27.719362975691,-6.59535001059349,-39.9695480499001));
#20982=CARTESIAN_POINT('',(27.7193629372986,-6.01690458230549,-39.9695479334715));
#20983=CARTESIAN_POINT('',(29.7611081292079,-12.8919045823054,-46.1613350574533));
#20984=CARTESIAN_POINT('Ctrl Pts',(27.7193631233119,-6.59534981976386,-39.9695484975747));
#20985=CARTESIAN_POINT('Ctrl Pts',(28.4014849791012,-8.68909917313932,-42.0381481153913));
#20986=CARTESIAN_POINT('Ctrl Pts',(29.0818842509084,-10.7885698299844,-44.101523832908));
#20987=CARTESIAN_POINT('Ctrl Pts',(29.761108129208,-12.8919045823054,-46.1613350574534));
#20988=CARTESIAN_POINT('',(27.6463789144421,-12.8919045823054,-39.7482169198025));
#20989=CARTESIAN_POINT('Origin',(0.0835265683620477,15.5455954176946,0.0824317919394229));
#20990=CARTESIAN_POINT('Origin',(0.0835265683620477,16.1705954176946,0.0824317919394229));
#20991=CARTESIAN_POINT('',(46.7874371828873,15.5455954176946,-28.9648526475816));
#20992=CARTESIAN_POINT('Origin',(0.0835265683620477,15.8580954176946,0.0824317919394229));
#20993=CARTESIAN_POINT('Origin',(42.8347289362664,15.5455954176946,-48.3550682080604));
#20994=CARTESIAN_POINT('',(40.1623618543411,15.8580954176946,-48.3550682080604));
#20995=CARTESIAN_POINT('',(40.1623618543411,16.1705954176946,-48.3550682080604));
#20996=CARTESIAN_POINT('',(40.1623618543411,16.4830954176946,-48.3550682080604));
#20997=CARTESIAN_POINT('',(29.6259351744661,16.1705954176946,-48.3550682080605));
#20998=CARTESIAN_POINT('',(42.8347289362664,15.8580954176946,-48.3550682080604));
#20999=CARTESIAN_POINT('Origin',(48.5210265683621,15.5455954176946,-25.9715236419289));
#21000=CARTESIAN_POINT('',(48.5210265683621,16.4830954176946,-29.4599768141643));
#21001=CARTESIAN_POINT('',(48.5210265683622,16.1705954176946,-39.9964034940393));
#21002=CARTESIAN_POINT('',(48.5210265683622,16.1705954176946,-39.9964034940393));
#21003=CARTESIAN_POINT('',(48.5210265683622,15.8580954176946,-39.9964034940393));
#21004=CARTESIAN_POINT('',(48.5210265683622,15.5455954176946,-39.9964034940393));
#21005=CARTESIAN_POINT('',(48.5210265683621,15.8580954176946,-25.9715236419289));
#21006=CARTESIAN_POINT('Origin',(0.0835265683620477,15.5455954176946,0.0824317919394229));
#21007=CARTESIAN_POINT('',(40.1623618543411,15.5455954176946,-48.0425682080604));
#21008=CARTESIAN_POINT('Origin',(40.1623618543411,15.5455954176946,-47.4175682080604));
#21009=CARTESIAN_POINT('',(29.6259351744661,15.5455954176946,-48.0425682080605));
#21010=CARTESIAN_POINT('',(0.0835265683622157,15.5455954176946,-48.0425682080606));
#21011=CARTESIAN_POINT('',(29.2958523967443,15.5455954176946,-46.8868419510772));
#21012=CARTESIAN_POINT('Origin',(29.6259351744661,15.5455954176946,-47.4175682080605));
#21013=CARTESIAN_POINT('Origin',(0.0835265683620477,15.5455954176946,0.0824317919394229));
#21014=CARTESIAN_POINT('',(48.2085265683622,15.5455954176946,-39.9964034940393));
#21015=CARTESIAN_POINT('',(48.208526568362,15.5455954176946,0.0824317919396409));
#21016=CARTESIAN_POINT('Origin',(47.5835265683622,15.5455954176946,-39.9964034940393));
#21017=CARTESIAN_POINT('Origin',(47.5835265683621,15.5455954176946,-29.4599768141643));
#21018=CARTESIAN_POINT('Origin',(40.1623618543411,15.5455954176946,-47.4175682080604));
#21019=CARTESIAN_POINT('Origin',(40.1623618543411,15.8580954176946,-47.4175682080604));
#21020=CARTESIAN_POINT('Origin',(40.1623618543411,16.1705954176946,-47.4175682080604));
#21021=CARTESIAN_POINT('Origin',(47.5835265683622,15.5455954176946,-39.9964034940393));
#21022=CARTESIAN_POINT('Origin',(47.5835265683622,15.8580954176946,-39.9964034940393));
#21023=CARTESIAN_POINT('Origin',(47.5835265683622,16.1705954176946,-39.9964034940393));
#21024=CARTESIAN_POINT('Origin',(0.0835265683620477,-6.01690458230549,0.0824317919394229));
#21025=CARTESIAN_POINT('',(45.9721485234461,-13.2959337131846,31.6825266249535));
#21026=CARTESIAN_POINT('',(46.8756079148278,-13.2959337131846,30.3286338949778));
#21027=CARTESIAN_POINT('Origin',(0.0835265683620477,-13.2959337131846,0.0824317919394229));
#21028=CARTESIAN_POINT('',(46.611780876039,-12.6709337131846,29.5815526781396));
#21029=CARTESIAN_POINT('Ctrl Pts',(46.8756079148278,-13.2959337131846,30.3286338949778));
#21030=CARTESIAN_POINT('Ctrl Pts',(46.8978549415453,-13.2959337131846,30.2942168570853));
#21031=CARTESIAN_POINT('Ctrl Pts',(46.9164623589588,-13.2919430659178,30.2579882035445));
#21032=CARTESIAN_POINT('Ctrl Pts',(46.9310469253967,-13.2842290832261,30.2210590246762));
#21033=CARTESIAN_POINT('Ctrl Pts',(46.9456755093586,-13.2764918190456,30.1840183902481));
#21034=CARTESIAN_POINT('Ctrl Pts',(46.9562575681815,-13.2650083398673,30.1462712757252));
#21035=CARTESIAN_POINT('Ctrl Pts',(46.96237146099,-13.2500137812688,30.1089284559708));
#21036=CARTESIAN_POINT('Ctrl Pts',(46.964608839739,-13.2445265233453,30.095262853063));
#21037=CARTESIAN_POINT('Ctrl Pts',(46.9662474594096,-13.2385687578732,30.0816514214285));
#21038=CARTESIAN_POINT('Ctrl Pts',(46.967265227178,-13.232151003965,30.0681489513688));
#21039=CARTESIAN_POINT('Ctrl Pts',(46.9672860185445,-13.2320198995247,30.0678731175172));
#21040=CARTESIAN_POINT('Ctrl Pts',(46.9673065509185,-13.2318886036912,30.0675973300348));
#21041=CARTESIAN_POINT('Ctrl Pts',(46.9673268241115,-13.2317571165656,30.0673215894106));
#21042=CARTESIAN_POINT('Ctrl Pts',(46.9707862023296,-13.209320409148,30.0202697455207));
#21043=CARTESIAN_POINT('Ctrl Pts',(46.9670157628007,-13.1821368365731,29.9756324601365));
#21044=CARTESIAN_POINT('Ctrl Pts',(46.9577324696803,-13.1520894282891,29.93427208866));
#21045=CARTESIAN_POINT('Ctrl Pts',(46.949874341568,-13.1266548782133,29.8992613340045));
#21046=CARTESIAN_POINT('Ctrl Pts',(46.9380672717436,-13.0991694705089,29.8665989294526));
#21047=CARTESIAN_POINT('Ctrl Pts',(46.923370924553,-13.0707895719798,29.8368060725869));
#21048=CARTESIAN_POINT('Ctrl Pts',(46.9232310976656,-13.0705195543472,29.8365226115073));
#21049=CARTESIAN_POINT('Ctrl Pts',(46.9230909968264,-13.0702494422352,29.8362394045269));
#21050=CARTESIAN_POINT('Ctrl Pts',(46.922950623042,-13.0699792368,29.8359564522459));
#21051=CARTESIAN_POINT('Ctrl Pts',(46.9128450180912,-13.0505269623212,29.8155865236052));
#21052=CARTESIAN_POINT('Ctrl Pts',(46.9013645568325,-13.0305367697038,29.7963754888012));
#21053=CARTESIAN_POINT('Ctrl Pts',(46.8887239261041,-13.0101903794884,29.7783251791885));
#21054=CARTESIAN_POINT('Ctrl Pts',(46.8813478779631,-12.9983178743144,29.7677924806607));
#21055=CARTESIAN_POINT('Ctrl Pts',(46.8735773726895,-12.9863240855329,29.7576540947851));
#21056=CARTESIAN_POINT('Ctrl Pts',(46.8654587684432,-12.9742444051773,29.7479032361322));
#21057=CARTESIAN_POINT('Ctrl Pts',(46.8543462450059,-12.9577100691025,29.7345565275075));
#21058=CARTESIAN_POINT('Ctrl Pts',(46.8425792590554,-12.9410147689399,29.721939386685));
#21059=CARTESIAN_POINT('Ctrl Pts',(46.8302713751129,-12.9242496162066,29.7100434451263));
#21060=CARTESIAN_POINT('Ctrl Pts',(46.8241174331417,-12.9158670398399,29.704095474347));
#21061=CARTESIAN_POINT('Ctrl Pts',(46.8178282665904,-12.9074670004228,29.6983278033295));
#21062=CARTESIAN_POINT('Ctrl Pts',(46.8114180701719,-12.8990608878296,29.6927393855369));
#21063=CARTESIAN_POINT('Ctrl Pts',(46.8050078737534,-12.8906547752363,29.6871509677443));
#21064=CARTESIAN_POINT('Ctrl Pts',(46.7984766474544,-12.8822425894822,29.6817418031665));
#21065=CARTESIAN_POINT('Ctrl Pts',(46.7918385853592,-12.8738357211132,29.6765108449771));
#21066=CARTESIAN_POINT('Ctrl Pts',(46.7709580422564,-12.8473912596395,29.6600564571789));
#21067=CARTESIAN_POINT('Ctrl Pts',(46.7488241283292,-12.8207472740102,29.6452040077705));
#21068=CARTESIAN_POINT('Ctrl Pts',(46.7256543087531,-12.7940681980269,29.6319196349234));
#21069=CARTESIAN_POINT('Ctrl Pts',(46.7193607757097,-12.7868214585468,29.6283112494891));
#21070=CARTESIAN_POINT('Ctrl Pts',(46.7129907957061,-12.779572258173,29.6248188257318));
#21071=CARTESIAN_POINT('Ctrl Pts',(46.7065487443092,-12.7723242153339,29.6214422648954));
#21072=CARTESIAN_POINT('Ctrl Pts',(46.6831396086853,-12.745986266849,29.6091725132756));
#21073=CARTESIAN_POINT('Ctrl Pts',(46.6587794951275,-12.7196622748047,29.5984290980846));
#21074=CARTESIAN_POINT('Ctrl Pts',(46.6336755188529,-12.6935087390576,29.5891798748265));
#21075=CARTESIAN_POINT('Ctrl Pts',(46.6264373389339,-12.6859679417279,29.5865130645443));
#21076=CARTESIAN_POINT('Ctrl Pts',(46.6191373861398,-12.6784415052653,29.583970722176));
#21077=CARTESIAN_POINT('Ctrl Pts',(46.611780876039,-12.6709337131846,29.5815526781396));
#21078=CARTESIAN_POINT('',(40.153012388794,-6.10843371318466,27.4594837601833));
#21079=CARTESIAN_POINT('Origin',(197.498086264171,-177.510315224915,79.5082955755947));
#21080=CARTESIAN_POINT('',(48.4286600918429,-6.1084337131593,4.30318207832973));
#21081=CARTESIAN_POINT('Origin',(0.0835265683620477,-6.10843371318469,0.0824317919394229));
#21082=CARTESIAN_POINT('',(48.3955019191566,-14.6753754514266,30.5110848543371));
#21083=CARTESIAN_POINT('Ctrl Pts',(48.4286600918172,-6.10843371318471,4.30318207891645));
#21084=CARTESIAN_POINT('Ctrl Pts',(48.4268304353416,-6.50994980321315,8.94066112535899));
#21085=CARTESIAN_POINT('Ctrl Pts',(48.4220707934636,-7.55645913600447,13.422965577783));
#21086=CARTESIAN_POINT('Ctrl Pts',(48.4129675603076,-9.80534906153841,19.9830370480983));
#21087=CARTESIAN_POINT('Ctrl Pts',(48.4096078578849,-10.6692546575742,22.1441467079631));
#21088=CARTESIAN_POINT('Ctrl Pts',(48.4026661196857,-12.5596572871779,26.382358737357));
#21089=CARTESIAN_POINT('Ctrl Pts',(48.3990822056017,-13.58630787804,28.4618866519976));
#21090=CARTESIAN_POINT('Ctrl Pts',(48.3955019191565,-14.6753754514262,30.5110848543364));
#21091=CARTESIAN_POINT('',(47.3365522275616,-14.6753754514262,32.1308553965182));
#21092=CARTESIAN_POINT('Origin',(0.0835265683620477,-14.6753754514262,0.0824317919394229));
#21093=CARTESIAN_POINT('Origin',(-1241.46289905476,-1402.95413115888,-321.604288607832));
#21094=CARTESIAN_POINT('Origin',(-4.89277133898972,-11.0169045823054,15.1735300494181));
#21095=CARTESIAN_POINT('',(46.6192727743382,-14.4544045724546,32.1596547801037));
#21096=CARTESIAN_POINT('',(18.8497068160573,-14.4544045823054,23.0026252115117));
#21097=CARTESIAN_POINT('',(-4.89277133898972,-14.4544045823054,15.1735300494181));
#21098=CARTESIAN_POINT('',(18.8497068160573,-11.3294045823054,23.0026252115117));
#21099=CARTESIAN_POINT('',(18.8497068160573,-11.0169045823054,23.0026252115117));
#21100=CARTESIAN_POINT('',(38.3508237177255,-11.3294045823054,29.4331291796839));
#21101=CARTESIAN_POINT('',(-4.89277133898972,-11.3294045823054,15.1735300494181));
#21102=CARTESIAN_POINT('',(38.3508237177255,-12.8919045823054,29.4331291796839));
#21103=CARTESIAN_POINT('',(38.3508237177255,-11.0169045823054,29.4331291796839));
#21104=CARTESIAN_POINT('',(38.9776909489554,-13.5169045823054,29.6398389921663));
#21105=CARTESIAN_POINT('Ctrl Pts',(38.9776909489554,-13.5169045823054,29.6398389921663));
#21106=CARTESIAN_POINT('Ctrl Pts',(38.9423929660079,-13.516904574972,29.6281994629764));
#21107=CARTESIAN_POINT('Ctrl Pts',(38.9071733611761,-13.5137764691096,29.6165857790133));
#21108=CARTESIAN_POINT('Ctrl Pts',(38.8724709034065,-13.5077394335846,29.6051426245749));
#21109=CARTESIAN_POINT('Ctrl Pts',(38.8352487396173,-13.5012640557713,29.5928685956978));
#21110=CARTESIAN_POINT('Ctrl Pts',(38.7986204242306,-13.4914421682004,29.5807903886535));
#21111=CARTESIAN_POINT('Ctrl Pts',(38.7631069894986,-13.4784883891908,29.5690798141137));
#21112=CARTESIAN_POINT('Ctrl Pts',(38.7270416010364,-13.4653332811151,29.5571872325292));
#21113=CARTESIAN_POINT('Ctrl Pts',(38.6921244765178,-13.4489478321352,29.5456732916074));
#21114=CARTESIAN_POINT('Ctrl Pts',(38.6589020389608,-13.42950318155,29.5347181746438));
#21115=CARTESIAN_POINT('Ctrl Pts',(38.6267589654953,-13.4106902684037,29.52411897858));
#21116=CARTESIAN_POINT('Ctrl Pts',(38.5962009713873,-13.3890130655275,29.5140424633077));
#21117=CARTESIAN_POINT('Ctrl Pts',(38.5677442515497,-13.3645846069919,29.5046588443803));
#21118=CARTESIAN_POINT('Ctrl Pts',(38.558505004034,-13.3566532439914,29.5016121974597));
#21119=CARTESIAN_POINT('Ctrl Pts',(38.5494875136696,-13.3484315569659,29.4986386750814));
#21120=CARTESIAN_POINT('Ctrl Pts',(38.5407102902568,-13.3399225829036,29.4957443808616));
#21121=CARTESIAN_POINT('Ctrl Pts',(38.5406156491554,-13.339830834222,29.4957131729067));
#21122=CARTESIAN_POINT('Ctrl Pts',(38.5405210362793,-13.3397390509053,29.4956819742591));
#21123=CARTESIAN_POINT('Ctrl Pts',(38.5404264516427,-13.3396472329756,29.4956507849234));
#21124=CARTESIAN_POINT('Ctrl Pts',(38.5055810206749,-13.305821070019,29.4841604850084));
#21125=CARTESIAN_POINT('Ctrl Pts',(38.4747122807658,-13.2674403224072,29.4739815011308));
#21126=CARTESIAN_POINT('Ctrl Pts',(38.4485152007503,-13.2257618865581,29.4653429996623));
#21127=CARTESIAN_POINT('Ctrl Pts',(38.4347246221117,-13.2038216647177,29.4607955488109));
#21128=CARTESIAN_POINT('Ctrl Pts',(38.4222290644973,-13.1809667715254,29.4566751318507));
#21129=CARTESIAN_POINT('Ctrl Pts',(38.4111336890027,-13.1573764603983,29.4530164257106));
#21130=CARTESIAN_POINT('Ctrl Pts',(38.3932412272899,-13.1193345988278,29.4471163766711));
#21131=CARTESIAN_POINT('Ctrl Pts',(38.3789843342392,-13.079375361177,29.4424151583871));
#21132=CARTESIAN_POINT('Ctrl Pts',(38.3688260877462,-13.0382175960838,29.4390654710481));
#21133=CARTESIAN_POINT('Ctrl Pts',(38.3588686319705,-12.9978733667896,29.4357819945579));
#21134=CARTESIAN_POINT('Ctrl Pts',(38.3528498623,-12.9563778845286,29.433797301966));
#21135=CARTESIAN_POINT('Ctrl Pts',(38.3512529278809,-12.9144212114187,29.4332707119675));
#21136=CARTESIAN_POINT('Ctrl Pts',(38.3509677633351,-12.9069290091781,29.4331766788025));
#21137=CARTESIAN_POINT('Ctrl Pts',(38.3508237212182,-12.899422137453,29.4331291808356));
#21138=CARTESIAN_POINT('Ctrl Pts',(38.3508237177256,-12.8919045823054,29.4331291796839));
#21139=CARTESIAN_POINT('',(45.6922912884794,-13.5169045823054,31.8539821279529));
#21140=CARTESIAN_POINT('',(-4.89277133898972,-13.5169045823054,15.1735300494181));
#21141=CARTESIAN_POINT('Origin',(-1220.21421106998,-1402.3016656762,-385.579379660149));
#21142=CARTESIAN_POINT('Origin',(-6.76693169846985,-11.0169045823054,20.8571001776055));
#21143=CARTESIAN_POINT('',(33.7901189707501,-12.8919045823054,34.2308098261781));
#21144=CARTESIAN_POINT('',(33.7901189707501,-11.3294045823054,34.2308098261781));
#21145=CARTESIAN_POINT('',(33.7901189707501,-11.0169045823054,34.2308098261781));
#21146=CARTESIAN_POINT('',(-6.76693169846985,-11.3294045823054,20.8571001776055));
#21147=CARTESIAN_POINT('',(-6.76693169846985,-11.3294045823054,20.8571001776055));
#21148=CARTESIAN_POINT('',(-6.76693169846985,-14.4544045823054,20.8571001776055));
#21149=CARTESIAN_POINT('',(-6.76693169846985,-11.0169045823054,20.8571001776055));
#21150=CARTESIAN_POINT('',(42.5114259882145,-14.4544045474401,37.1066655869754));
#21151=CARTESIAN_POINT('',(43.4136327877683,-14.4544045823054,37.4041687727522));
#21152=CARTESIAN_POINT('',(41.5416017773197,-13.5169045823054,36.7868655227931));
#21153=CARTESIAN_POINT('Origin',(-529.90702904109,-669.972712130993,-151.648633150656));
#21154=CARTESIAN_POINT('',(34.4578582575083,-13.5169045823054,34.4509972213337));
#21155=CARTESIAN_POINT('',(34.2758494659228,-13.5169045823054,34.390979722724));
#21156=CARTESIAN_POINT('Ctrl Pts',(33.7901189707501,-12.8919045823054,34.2308098261781));
#21157=CARTESIAN_POINT('Ctrl Pts',(33.7901189707501,-12.9240089539701,34.2308098261781));
#21158=CARTESIAN_POINT('Ctrl Pts',(33.7927314458503,-12.955801183802,34.2316712912717));
#21159=CARTESIAN_POINT('Ctrl Pts',(33.7978675102913,-12.9870390822583,34.2333649113313));
#21160=CARTESIAN_POINT('Ctrl Pts',(33.8031273642748,-13.0190298772567,34.2350993510602));
#21161=CARTESIAN_POINT('Ctrl Pts',(33.8110337447306,-13.0504387215006,34.2377064843414));
#21162=CARTESIAN_POINT('Ctrl Pts',(33.8214395081087,-13.0810143824798,34.2411377905089));
#21163=CARTESIAN_POINT('Ctrl Pts',(33.8287255515569,-13.102423248534,34.2435403673225));
#21164=CARTESIAN_POINT('Ctrl Pts',(33.8372358660587,-13.1234238076975,34.2463466481858));
#21165=CARTESIAN_POINT('Ctrl Pts',(33.8469063040395,-13.1439346499851,34.2495354804013));
#21166=CARTESIAN_POINT('Ctrl Pts',(33.8469498796939,-13.1440270732421,34.2495498494972));
#21167=CARTESIAN_POINT('Ctrl Pts',(33.8469934759197,-13.1441194808469,34.2495642253765));
#21168=CARTESIAN_POINT('Ctrl Pts',(33.8470370927095,-13.144211872797,34.2495786080368));
#21169=CARTESIAN_POINT('Ctrl Pts',(33.8816554487368,-13.2175427491137,34.2609940298788));
#21170=CARTESIAN_POINT('Ctrl Pts',(33.9294439233777,-13.2814833076921,34.276752305537));
#21171=CARTESIAN_POINT('Ctrl Pts',(33.9877805172936,-13.3355724235757,34.2959888293));
#21172=CARTESIAN_POINT('Ctrl Pts',(33.9918226137392,-13.3393202156285,34.2973217128146));
#21173=CARTESIAN_POINT('Ctrl Pts',(33.995915366069,-13.3430206975362,34.2986713001347));
#21174=CARTESIAN_POINT('Ctrl Pts',(34.0000579079991,-13.3466737099127,34.3000373056028));
#21175=CARTESIAN_POINT('Ctrl Pts',(34.0001081300639,-13.346717997171,34.3000538663561));
#21176=CARTESIAN_POINT('Ctrl Pts',(34.0001583569437,-13.3467622754631,34.3000704286972));
#21177=CARTESIAN_POINT('Ctrl Pts',(34.0002085886379,-13.3468065447898,34.3000869926259));
#21178=CARTESIAN_POINT('Ctrl Pts',(34.0641821309938,-13.4031865990189,34.3211823032219));
#21179=CARTESIAN_POINT('Ctrl Pts',(34.1359363403631,-13.44500831055,34.3448432930207));
#21180=CARTESIAN_POINT('Ctrl Pts',(34.2146228130674,-13.4738659092282,34.3707902004465));
#21181=CARTESIAN_POINT('Ctrl Pts',(34.2933529212196,-13.5027395108379,34.3967514966851));
#21182=CARTESIAN_POINT('Ctrl Pts',(34.3745006619984,-13.5169045582356,34.423510008606));
#21183=CARTESIAN_POINT('Ctrl Pts',(34.4578582575083,-13.5169045823054,34.4509972213337));
#21184=CARTESIAN_POINT('Origin',(0.0835265683620477,-6.01690458230549,0.0824317919394229));
#21185=CARTESIAN_POINT('',(4.30427670995454,-6.10843422628143,48.4275654856862));
#21186=CARTESIAN_POINT('',(32.2061415767159,-6.10843371299758,36.4583066734133));
#21187=CARTESIAN_POINT('Origin',(0.0835265683620477,-6.10843371318469,0.0824317919394229));
#21188=CARTESIAN_POINT('',(39.2939826516718,-12.6709337131846,38.7814849549994));
#21189=CARTESIAN_POINT('Ctrl Pts',(32.2061415763564,-6.10843371318765,36.4583066739843));
#21190=CARTESIAN_POINT('Ctrl Pts',(32.6895829804899,-6.54712953976792,36.6166555923948));
#21191=CARTESIAN_POINT('Ctrl Pts',(33.1721101495054,-6.98698298247605,36.7746225070907));
#21192=CARTESIAN_POINT('Ctrl Pts',(33.6537398736913,-7.42790908709483,36.9323189016539));
#21193=CARTESIAN_POINT('Ctrl Pts',(34.1334866890221,-7.86711141175329,37.0893987895464));
#21194=CARTESIAN_POINT('Ctrl Pts',(34.6123431500573,-8.30737802767375,37.2462103272133));
#21195=CARTESIAN_POINT('Ctrl Pts',(35.0903517895406,-8.74862497312237,37.402819026504));
#21196=CARTESIAN_POINT('Ctrl Pts',(35.5674289513232,-9.18901207701961,37.559122548233));
#21197=CARTESIAN_POINT('Ctrl Pts',(36.0436616592707,-9.63037569350405,37.7152240805629));
#21198=CARTESIAN_POINT('Ctrl Pts',(36.5191169505044,-10.0726323507254,37.8711432684101));
#21199=CARTESIAN_POINT('Ctrl Pts',(36.993227181731,-10.5136378666649,38.0266213618626));
#21200=CARTESIAN_POINT('Ctrl Pts',(37.4665644488621,-10.9555313776754,38.1819181817231));
#21201=CARTESIAN_POINT('Ctrl Pts',(37.939218906132,-11.3982301183281,38.3370072007052));
#21202=CARTESIAN_POINT('Ctrl Pts',(38.3913986968972,-11.8217518281976,38.4853780011381));
#21203=CARTESIAN_POINT('Ctrl Pts',(38.8429537376373,-12.246010516087,38.6335583573869));
#21204=CARTESIAN_POINT('Ctrl Pts',(39.2939826516718,-12.6709337131846,38.7814849549994));
#21205=CARTESIAN_POINT('',(40.4397116715677,-13.2959337131846,38.4974020809805));
#21206=CARTESIAN_POINT('Ctrl Pts',(40.4397116715676,-13.2959337131846,38.4974020809807));
#21207=CARTESIAN_POINT('Ctrl Pts',(40.4066868182815,-13.2959336603245,38.5320956948767));
#21208=CARTESIAN_POINT('Ctrl Pts',(40.3709843137298,-13.2916605128677,38.5633120948844));
#21209=CARTESIAN_POINT('Ctrl Pts',(40.3335867953624,-13.2840750781525,38.5914271479214));
#21210=CARTESIAN_POINT('Ctrl Pts',(40.2903824802747,-13.2753118359423,38.6239076884263));
#21211=CARTESIAN_POINT('Ctrl Pts',(40.2449149265883,-13.2621273075678,38.6522492669877));
#21212=CARTESIAN_POINT('Ctrl Pts',(40.1986646417893,-13.2459526169444,38.6769937284272));
#21213=CARTESIAN_POINT('Ctrl Pts',(40.1851376876442,-13.2412219585426,38.6842308124082));
#21214=CARTESIAN_POINT('Ctrl Pts',(40.1715436445126,-13.2362352705239,38.6911599698083));
#21215=CARTESIAN_POINT('Ctrl Pts',(40.1579193431335,-13.2310278528738,38.6977942320586));
#21216=CARTESIAN_POINT('Ctrl Pts',(40.1578742334737,-13.2310106112676,38.6978161979052));
#21217=CARTESIAN_POINT('Ctrl Pts',(40.1578291234839,-13.230993367242,38.6978381605175));
#21218=CARTESIAN_POINT('Ctrl Pts',(40.1577840131655,-13.2309761207982,38.6978601198961));
#21219=CARTESIAN_POINT('Ctrl Pts',(40.0679185768218,-13.1966190323189,38.7416059680517));
#21220=CARTESIAN_POINT('Ctrl Pts',(39.9767121201785,-13.152555648727,38.7724161582456));
#21221=CARTESIAN_POINT('Ctrl Pts',(39.8871981003423,-13.1028429786438,38.7931532120191));
#21222=CARTESIAN_POINT('Ctrl Pts',(39.8766190756684,-13.0969677921157,38.7956039767589));
#21223=CARTESIAN_POINT('Ctrl Pts',(39.8660637060712,-13.091013740083,38.7979140888403));
#21224=CARTESIAN_POINT('Ctrl Pts',(39.855537010514,-13.0849875486837,38.8000883045475));
#21225=CARTESIAN_POINT('Ctrl Pts',(39.8554152338134,-13.0849178354767,38.8001134566775));
#21226=CARTESIAN_POINT('Ctrl Pts',(39.8552934598642,-13.0848481114876,38.8001385901193));
#21227=CARTESIAN_POINT('Ctrl Pts',(39.8551716886783,-13.0847783767298,38.8001637048806));
#21228=CARTESIAN_POINT('Ctrl Pts',(39.8303839263928,-13.0705831581647,38.8052760697483));
#21229=CARTESIAN_POINT('Ctrl Pts',(39.8055929272658,-13.0558793142743,38.8096455507573));
#21230=CARTESIAN_POINT('Ctrl Pts',(39.780884675532,-13.0407301262923,38.8132772606744));
#21231=CARTESIAN_POINT('Ctrl Pts',(39.7436402270521,-13.0178947125452,38.8187515869991));
#21232=CARTESIAN_POINT('Ctrl Pts',(39.7065811166617,-12.9940463246918,38.8225507431792));
#21233=CARTESIAN_POINT('Ctrl Pts',(39.6699900069733,-12.9693962501975,38.8246970808061));
#21234=CARTESIAN_POINT('Ctrl Pts',(39.633398897285,-12.9447461757032,38.8268434184329));
#21235=CARTESIAN_POINT('Ctrl Pts',(39.5972757976144,-12.9192944015675,38.8273369465679));
#21236=CARTESIAN_POINT('Ctrl Pts',(39.5619034483267,-12.8932521061511,38.8262000930124));
#21237=CARTESIAN_POINT('Ctrl Pts',(39.5318432459393,-12.8711207892717,38.8252339697932));
#21238=CARTESIAN_POINT('Ctrl Pts',(39.5022622280843,-12.8485482515855,38.8231336850165));
#21239=CARTESIAN_POINT('Ctrl Pts',(39.4731842379688,-12.8255048445977,38.8198375199283));
#21240=CARTESIAN_POINT('Ctrl Pts',(39.4566401434559,-12.8123941618582,38.8179621473));
#21241=CARTESIAN_POINT('Ctrl Pts',(39.4402593911746,-12.7991308725963,38.8156988765352));
#21242=CARTESIAN_POINT('Ctrl Pts',(39.4240511389472,-12.7857088195892,38.8130305325372));
#21243=CARTESIAN_POINT('Ctrl Pts',(39.3951315085124,-12.7617604748081,38.8082695304741));
#21244=CARTESIAN_POINT('Ctrl Pts',(39.3667585577106,-12.7373067239787,38.802221542794));
#21245=CARTESIAN_POINT('Ctrl Pts',(39.3389584490096,-12.7123167139678,38.7948212644581));
#21246=CARTESIAN_POINT('Ctrl Pts',(39.3237928405683,-12.6986840799789,38.790784239826));
#21247=CARTESIAN_POINT('Ctrl Pts',(39.3087981609348,-12.6848916911023,38.7863440783211));
#21248=CARTESIAN_POINT('Ctrl Pts',(39.2939826516718,-12.6709337131846,38.7814849549994));
#21249=CARTESIAN_POINT('',(41.6084251757828,-13.2959337131846,37.2309770398429));
#21250=CARTESIAN_POINT('Origin',(0.0835265683620477,-13.2959337131846,0.0824317919394229));
#21251=CARTESIAN_POINT('',(43.0359437581361,-14.6753754514262,37.6994458553003));
#21252=CARTESIAN_POINT('Origin',(-537.184566063455,-671.736419692119,-133.458018919704));
#21253=CARTESIAN_POINT('',(30.51217970824,-14.675375306047,48.3944072657487));
#21254=CARTESIAN_POINT('Origin',(0.0835265683620477,-14.6753754514262,0.0824317919394229));
#21255=CARTESIAN_POINT('Ctrl Pts',(30.5121799406814,-14.6753748699083,48.3944076347922));
#21256=CARTESIAN_POINT('Ctrl Pts',(29.6488324750175,-14.2165313293604,48.3959217299873));
#21257=CARTESIAN_POINT('Ctrl Pts',(28.7803560530607,-13.7688961397319,48.3974310167534));
#21258=CARTESIAN_POINT('Ctrl Pts',(27.9060899457771,-13.3339028956054,48.3989301271172));
#21259=CARTESIAN_POINT('Ctrl Pts',(27.056709414216,-12.9112915306634,48.4003865660059));
#21260=CARTESIAN_POINT('Ctrl Pts',(26.2018640443159,-12.5006127566903,48.4018333971136));
#21261=CARTESIAN_POINT('Ctrl Pts',(25.3409737846802,-12.1031392031217,48.4032655009723));
#21262=CARTESIAN_POINT('Ctrl Pts',(25.0217106273087,-11.9557352102624,48.4037966000229));
#21263=CARTESIAN_POINT('Ctrl Pts',(24.7016163733872,-11.8101469191841,48.4043256718175));
#21264=CARTESIAN_POINT('Ctrl Pts',(24.3806624063341,-11.6664376689275,48.4048524492713));
#21265=CARTESIAN_POINT('Ctrl Pts',(24.3484751771087,-11.6520256252868,48.4049052777401));
#21266=CARTESIAN_POINT('Ctrl Pts',(24.3162792494227,-11.6376325718389,48.4049580822714));
#21267=CARTESIAN_POINT('Ctrl Pts',(24.2840745830158,-11.6232585917439,48.4050108624134));
#21268=CARTESIAN_POINT('Ctrl Pts',(23.5112493892555,-11.2783218111032,48.4062774435657));
#21269=CARTESIAN_POINT('Ctrl Pts',(22.7333797368795,-10.9443666917881,48.4075285034311));
#21270=CARTESIAN_POINT('Ctrl Pts',(21.9499770951734,-10.622542813258,48.4087548715985));
#21271=CARTESIAN_POINT('Ctrl Pts',(21.679859986483,-10.5115779901286,48.4091777231513));
#21272=CARTESIAN_POINT('Ctrl Pts',(21.4090853092871,-10.4020550292294,48.409597642173));
#21273=CARTESIAN_POINT('Ctrl Pts',(21.137633790018,-10.2940198074425,48.4100142623316));
#21274=CARTESIAN_POINT('Ctrl Pts',(21.1213606839124,-10.2875432600575,48.410039238077));
#21275=CARTESIAN_POINT('Ctrl Pts',(21.1050848873588,-10.2810720136182,48.4100642022031));
#21276=CARTESIAN_POINT('Ctrl Pts',(21.0888064415878,-10.2746060938733,48.4100891545555));
#21277=CARTESIAN_POINT('Ctrl Pts',(20.6329211858941,-10.0935250792803,48.4107879564984));
#21278=CARTESIAN_POINT('Ctrl Pts',(20.1749952047483,-9.9166326383212,48.4114781297796));
#21279=CARTESIAN_POINT('Ctrl Pts',(19.7152601034564,-9.74425107298764,48.4121573955266));
#21280=CARTESIAN_POINT('Ctrl Pts',(19.2749122844202,-9.57913893314155,48.4128080162631));
#21281=CARTESIAN_POINT('Ctrl Pts',(18.8329032539855,-9.41816464509348,48.4134486342682));
#21282=CARTESIAN_POINT('Ctrl Pts',(18.3894211536449,-9.26165511776138,48.4140771416491));
#21283=CARTESIAN_POINT('Ctrl Pts',(18.2037607417664,-9.19613359325097,48.414340261489));
#21284=CARTESIAN_POINT('Ctrl Pts',(18.0178420881853,-9.13139516038838,48.414601257143));
#21285=CARTESIAN_POINT('Ctrl Pts',(17.8316790387899,-9.06746659619147,48.414859965488));
#21286=CARTESIAN_POINT('Ctrl Pts',(17.8280779083912,-9.06622996466542,48.4148649699316));
#21287=CARTESIAN_POINT('Ctrl Pts',(17.8244767169066,-9.06499364665141,48.4148699734635));
#21288=CARTESIAN_POINT('Ctrl Pts',(17.8208754647278,-9.06375764243283,48.4148749760823));
#21289=CARTESIAN_POINT('Ctrl Pts',(16.9526599969218,-8.76577296167702,48.4160810429658));
#21290=CARTESIAN_POINT('Ctrl Pts',(16.0792020931599,-8.48534970221955,48.4172359828182));
#21291=CARTESIAN_POINT('Ctrl Pts',(15.2000695648677,-8.22405492504872,48.4183278724742));
#21292=CARTESIAN_POINT('Ctrl Pts',(14.9739344468961,-8.15684330068117,48.4186087341057));
#21293=CARTESIAN_POINT('Ctrl Pts',(14.7474238161432,-8.09089757132381,48.4188854218506));
#21294=CARTESIAN_POINT('Ctrl Pts',(14.5205302069433,-8.02624496071279,48.4191577282275));
#21295=CARTESIAN_POINT('Ctrl Pts',(14.0020828443853,-7.87851503754759,48.4197799428567));
#21296=CARTESIAN_POINT('Ctrl Pts',(13.4813283109344,-7.73745329658892,48.4203795067404));
#21297=CARTESIAN_POINT('Ctrl Pts',(12.958692622873,-7.60353311380589,48.4209531569399));
#21298=CARTESIAN_POINT('Ctrl Pts',(12.4566635157299,-7.47489316187225,48.4215041891486));
#21299=CARTESIAN_POINT('Ctrl Pts',(11.9528986695681,-7.35284273129184,48.4220313090909));
#21300=CARTESIAN_POINT('Ctrl Pts',(11.4477849931265,-7.23775611982421,48.4225317776524));
#21301=CARTESIAN_POINT('Ctrl Pts',(11.2675563144811,-7.1966922783921,48.4227103489162));
#21302=CARTESIAN_POINT('Ctrl Pts',(11.0871541074089,-7.15651419440583,48.4228855304241));
#21303=CARTESIAN_POINT('Ctrl Pts',(10.9066091662104,-7.11724012295064,48.423057191374));
#21304=CARTESIAN_POINT('Ctrl Pts',(9.81752556341492,-6.88033098025773,48.4240926849439));
#21305=CARTESIAN_POINT('Ctrl Pts',(8.72304426013872,-6.67627260244091,48.4250002518316));
#21306=CARTESIAN_POINT('Ctrl Pts',(7.62278160794834,-6.50737682456698,48.4257586248259));
#21307=CARTESIAN_POINT('Ctrl Pts',(6.52251895575796,-6.33848104669305,48.4265169978202));
#21308=CARTESIAN_POINT('Ctrl Pts',(5.41647491773991,-6.20474805616561,48.4271261752529));
#21309=CARTESIAN_POINT('Ctrl Pts',(4.30427673497461,-6.10843510301176,48.4275652912163));
#21310=CARTESIAN_POINT('Origin',(0.0835265683620477,11.4830954176946,0.0824317919394229));
#21311=CARTESIAN_POINT('',(34.3285543476724,11.4830954176946,36.0841779807601));
#21312=CARTESIAN_POINT('',(-34.1615012109487,11.4830954176946,36.0841779807597));
#21313=CARTESIAN_POINT('Origin',(0.0835265683620477,12.0636401876617,0.0824317919394229));
#21314=CARTESIAN_POINT('',(-34.8465649140277,13.0346110567823,36.7726127649112));
#21315=CARTESIAN_POINT('',(-34.8465649140274,13.0346110567825,36.7726127649118));
#21316=CARTESIAN_POINT('',(35.0136180507511,13.0346110567825,36.7726127649121));
#21317=CARTESIAN_POINT('',(34.3916369666324,12.1551693185409,36.1504966431761));
#21318=CARTESIAN_POINT('',(8.7871565714169,13.0346110567825,49.98761684888));
#21319=CARTESIAN_POINT('Origin',(0.0835265683620477,13.0346110567825,0.0824317919394229));
#21320=CARTESIAN_POINT('',(-8.62010343469277,13.0346110567825,49.98761684888));
#21321=CARTESIAN_POINT('Ctrl Pts',(8.7871565714169,13.0346110567825,49.98761684888));
#21322=CARTESIAN_POINT('Ctrl Pts',(7.92550064906484,12.8871967548028,49.9882530796749));
#21323=CARTESIAN_POINT('Ctrl Pts',(7.06161609265391,12.7606786217037,49.9888052593523));
#21324=CARTESIAN_POINT('Ctrl Pts',(6.19543459293618,12.6558408129365,49.98926502916));
#21325=CARTESIAN_POINT('Ctrl Pts',(5.61894217814055,12.5860653656916,49.9895710317781));
#21326=CARTESIAN_POINT('Ctrl Pts',(5.04143250829548,12.5258925149755,49.9898361091157));
#21327=CARTESIAN_POINT('Ctrl Pts',(4.46288801112708,12.4755408811181,49.9900578945362));
#21328=CARTESIAN_POINT('Ctrl Pts',(4.45970749302406,12.4752640756455,49.9900591137899));
#21329=CARTESIAN_POINT('Ctrl Pts',(4.45652691494998,12.4749875690291,49.9900603317248));
#21330=CARTESIAN_POINT('Ctrl Pts',(4.45334627723674,12.4747113612835,49.9900615483407));
#21331=CARTESIAN_POINT('Ctrl Pts',(4.030833582814,12.4380202039354,49.9902231623675));
#21332=CARTESIAN_POINT('Ctrl Pts',(3.60755981318608,12.4066244502022,49.9903617724682));
#21333=CARTESIAN_POINT('Ctrl Pts',(3.18378964752083,12.3805167222776,49.9904772560375));
#21334=CARTESIAN_POINT('Ctrl Pts',(2.75593208301871,12.3541571769636,49.9905938534827));
#21335=CARTESIAN_POINT('Ctrl Pts',(2.32756730732015,12.3331879704976,49.9906868771953));
#21336=CARTESIAN_POINT('Ctrl Pts',(1.89895102917436,12.3176520559944,49.9907559814859));
#21337=CARTESIAN_POINT('Ctrl Pts',(1.47793210215791,12.3023915202009,49.9908238608825));
#21338=CARTESIAN_POINT('Ctrl Pts',(1.05666935743236,12.2923733967889,49.9908686614172));
#21339=CARTESIAN_POINT('Ctrl Pts',(0.635406610984126,12.2876877721288,49.9908898373879));
#21340=CARTESIAN_POINT('Ctrl Pts',(0.451513336654972,12.28564236254,49.9908990813066));
#21341=CARTESIAN_POINT('Ctrl Pts',(0.267620182626321,12.2846137392999,49.9909038205458));
#21342=CARTESIAN_POINT('Ctrl Pts',(0.0837483634682333,12.2846124143579,
49.9909039962098));
#21343=CARTESIAN_POINT('Ctrl Pts',(0.0798267472639425,12.2846123860996,
49.9909039999564));
#21344=CARTESIAN_POINT('Ctrl Pts',(0.0759051865461643,12.2846128251744,
49.9909040015881));
#21345=CARTESIAN_POINT('Ctrl Pts',(0.0719836819143394,12.2846137316609,
49.9909040011047));
#21346=CARTESIAN_POINT('Ctrl Pts',(-1.08470971159645,12.2848811103974,49.990903858513));
#21347=CARTESIAN_POINT('Ctrl Pts',(-2.23919271888792,12.3254286614639,49.9907197297609));
#21348=CARTESIAN_POINT('Ctrl Pts',(-3.39148882634123,12.4051717612022,49.990365638491));
#21349=CARTESIAN_POINT('Ctrl Pts',(-3.68831749711159,12.4257133894741,49.9902744254423));
#21350=CARTESIAN_POINT('Ctrl Pts',(-3.98500107435261,12.4488556287919,49.9901719363719));
#21351=CARTESIAN_POINT('Ctrl Pts',(-4.28154000423778,12.4745793828298,49.9900584161199));
#21352=CARTESIAN_POINT('Ctrl Pts',(-4.82827914657013,12.5220071631409,49.9898491148816));
#21353=CARTESIAN_POINT('Ctrl Pts',(-5.37459250935462,12.578220119787,49.9896018888339));
#21354=CARTESIAN_POINT('Ctrl Pts',(-5.92009010621466,12.643043269177,49.9893181539585));
#21355=CARTESIAN_POINT('Ctrl Pts',(-6.47328863096735,12.7087815434037,49.9890304135258));
#21356=CARTESIAN_POINT('Ctrl Pts',(-7.02564819591232,12.7833747882158,49.9887051270459));
#21357=CARTESIAN_POINT('Ctrl Pts',(-7.5767680370208,12.8665869343008,49.9883440006327));
#21358=CARTESIAN_POINT('Ctrl Pts',(-7.92507488019195,12.9191768752799,49.9881157693269));
#21359=CARTESIAN_POINT('Ctrl Pts',(-8.27288667005804,12.9752083234333,49.9878732273165));
#21360=CARTESIAN_POINT('Ctrl Pts',(-8.62010343469276,13.0346110567825,49.98761684888));
#21361=CARTESIAN_POINT('Origin',(0.0835265683620477,13.0346110567825,0.0824317919394229));
#21362=CARTESIAN_POINT('Origin',(0.0835265683620477,16.4830954176946,50.0824317919394));
#21363=CARTESIAN_POINT('',(-22.6217205869088,-8.87385981233827,50.0824317919394));
#21364=CARTESIAN_POINT('',(-21.5367763897373,-8.69080155057986,50.0824317919394));
#21365=CARTESIAN_POINT('Ctrl Pts',(-22.6217205869088,-8.87385981233827,
50.0824317919394));
#21366=CARTESIAN_POINT('Ctrl Pts',(-22.5517841558568,-8.87385981188611,
50.0824317919394));
#21367=CARTESIAN_POINT('Ctrl Pts',(-22.4818161430779,-8.87185808464267,
50.0824317919395));
#21368=CARTESIAN_POINT('Ctrl Pts',(-22.4120212868203,-8.86782837150089,
50.0824317919394));
#21369=CARTESIAN_POINT('Ctrl Pts',(-22.3411456944659,-8.86373626040192,
50.0824317919393));
#21370=CARTESIAN_POINT('Ctrl Pts',(-22.2704470198759,-8.85755327620029,
50.0824317919393));
#21371=CARTESIAN_POINT('Ctrl Pts',(-22.2001193077708,-8.84920383564279,
50.0824317919363));
#21372=CARTESIAN_POINT('Ctrl Pts',(-22.1568417202882,-8.84406583764253,
50.0824317919344));
#21373=CARTESIAN_POINT('Ctrl Pts',(-22.1137043120179,-8.83810648050711,
50.0824317919313));
#21374=CARTESIAN_POINT('Ctrl Pts',(-22.0707526912653,-8.83129827231295,
50.082431791925));
#21375=CARTESIAN_POINT('Ctrl Pts',(-22.0704240016376,-8.83124617212726,
50.082431791925));
#21376=CARTESIAN_POINT('Ctrl Pts',(-22.070095320049,-8.83119402657727,50.0824317919249));
#21377=CARTESIAN_POINT('Ctrl Pts',(-22.0697666464964,-8.83114183558492,
50.0824317919249));
#21378=CARTESIAN_POINT('Ctrl Pts',(-21.9572130892569,-8.81326914154647,
50.0824317919083));
#21379=CARTESIAN_POINT('Ctrl Pts',(-21.8458794227438,-8.79011900697435,
50.0824317919293));
#21380=CARTESIAN_POINT('Ctrl Pts',(-21.7364461053673,-8.75874571241513,
50.0824317919358));
#21381=CARTESIAN_POINT('Ctrl Pts',(-21.6691162959035,-8.73944301744465,
50.0824317919398));
#21382=CARTESIAN_POINT('Ctrl Pts',(-21.6025059895988,-8.71702701269503,
50.0824317919394));
#21383=CARTESIAN_POINT('Ctrl Pts',(-21.5367763897394,-8.69080155058071,
50.0824317919394));
#21384=CARTESIAN_POINT('',(-44.2914734316384,-8.87385981233827,50.082431791939));
#21385=CARTESIAN_POINT('',(0.0835265683620477,-8.87385981233827,50.0824317919394));
#21386=CARTESIAN_POINT('',(-44.2914734316384,-14.4544045823054,50.082431791939));
#21387=CARTESIAN_POINT('',(-44.2914734316384,16.4830954176946,50.082431791939));
#21388=CARTESIAN_POINT('',(44.458526568362,-14.4544045823054,50.0824317919394));
#21389=CARTESIAN_POINT('',(0.0835265683620477,-14.4544045823054,50.0824317919394));
#21390=CARTESIAN_POINT('',(44.458526568362,-8.87385981233827,50.0824317919394));
#21391=CARTESIAN_POINT('',(44.458526568362,16.4830954176946,50.0824317919394));
#21392=CARTESIAN_POINT('',(22.7887737236329,-8.87385981233827,50.0824317919394));
#21393=CARTESIAN_POINT('',(0.0835265683620477,-8.87385981233827,50.0824317919394));
#21394=CARTESIAN_POINT('',(21.7038295264614,-8.69080155057986,50.0824317919394));
#21395=CARTESIAN_POINT('Ctrl Pts',(21.7038295264614,-8.69080155057986,50.0824317919394));
#21396=CARTESIAN_POINT('Ctrl Pts',(21.8139951203631,-8.7347565461317,50.0824317919394));
#21397=CARTESIAN_POINT('Ctrl Pts',(21.9275645136047,-8.76821292000628,50.0824317919394));
#21398=CARTESIAN_POINT('Ctrl Pts',(22.0424292060519,-8.79411643469838,50.0824317919394));
#21399=CARTESIAN_POINT('Ctrl Pts',(22.1075139143365,-8.80879390138867,50.0824317919394));
#21400=CARTESIAN_POINT('Ctrl Pts',(22.1730141788683,-8.82104760689908,50.0824317919394));
#21401=CARTESIAN_POINT('Ctrl Pts',(22.2385467888997,-8.83141832822413,50.0824317919393));
#21402=CARTESIAN_POINT('Ctrl Pts',(22.2386507853477,-8.83143478595685,50.0824317919393));
#21403=CARTESIAN_POINT('Ctrl Pts',(22.2387547823744,-8.83145123875071,50.0824317919393));
#21404=CARTESIAN_POINT('Ctrl Pts',(22.2388587799798,-8.83146768660594,50.0824317919393));
#21405=CARTESIAN_POINT('Ctrl Pts',(22.4201525755661,-8.86014040550798,50.0824317919389));
#21406=CARTESIAN_POINT('Ctrl Pts',(22.6035144602885,-8.87385980853305,50.0824317919394));
#21407=CARTESIAN_POINT('Ctrl Pts',(22.7887737236329,-8.87385981233827,50.0824317919394));
#21408=CARTESIAN_POINT('Ctrl Pts',(21.7038295264614,-8.69080155057986,50.0824317919394));
#21409=CARTESIAN_POINT('Ctrl Pts',(20.8438722721191,-8.34768669240134,50.0824317919394));
#21410=CARTESIAN_POINT('Ctrl Pts',(19.9790807826263,-8.0198017877672,50.0824317919394));
#21411=CARTESIAN_POINT('Ctrl Pts',(19.1089707832958,-7.70866381791472,50.0824317919393));
#21412=CARTESIAN_POINT('Ctrl Pts',(18.2388607839653,-7.39752584806224,50.0824317919392));
#21413=CARTESIAN_POINT('Ctrl Pts',(17.3634321497246,-7.10313511035514,50.0824317919392));
#21414=CARTESIAN_POINT('Ctrl Pts',(16.4822225240427,-6.82695644195446,50.0824317919394));
#21415=CARTESIAN_POINT('Ctrl Pts',(16.4713288078639,-6.82354225770076,50.0824317919394));
#21416=CARTESIAN_POINT('Ctrl Pts',(16.4604342061586,-6.8201308617252,50.0824317919394));
#21417=CARTESIAN_POINT('Ctrl Pts',(16.4495387178998,-6.81672225716408,50.0824317919394));
#21418=CARTESIAN_POINT('Ctrl Pts',(15.7049370028632,-6.58377695523626,50.0824317919395));
#21419=CARTESIAN_POINT('Ctrl Pts',(14.9561560013555,-6.36386066915742,50.0824317919409));
#21420=CARTESIAN_POINT('Ctrl Pts',(14.2029817792061,-6.15798672786968,50.0824317919379));
#21421=CARTESIAN_POINT('Ctrl Pts',(14.0708035005379,-6.12185688913941,50.0824317919374));
#21422=CARTESIAN_POINT('Ctrl Pts',(13.9384899672118,-6.08615941362245,50.0824317919367));
#21423=CARTESIAN_POINT('Ctrl Pts',(13.8060400877123,-6.05089962282538,50.0824317919355));
#21424=CARTESIAN_POINT('Ctrl Pts',(13.7943582912455,-6.04778978458991,50.0824317919354));
#21425=CARTESIAN_POINT('Ctrl Pts',(13.7826750481892,-6.04468327282916,50.0824317919353));
#21426=CARTESIAN_POINT('Ctrl Pts',(13.7709903766333,-6.04158009539295,50.0824317919352));
#21427=CARTESIAN_POINT('Ctrl Pts',(13.2422785619911,-5.90116651460846,50.0824317919303));
#21428=CARTESIAN_POINT('Ctrl Pts',(12.7107942008915,-5.76761845987533,50.082431791934));
#21429=CARTESIAN_POINT('Ctrl Pts',(12.1776858808268,-5.64153128315994,50.0824317919343));
#21430=CARTESIAN_POINT('Ctrl Pts',(11.8131021981237,-5.5553024146573,50.0824317919345));
#21431=CARTESIAN_POINT('Ctrl Pts',(11.4477578757322,-5.47256360697682,50.0824317919357));
#21432=CARTESIAN_POINT('Ctrl Pts',(11.0820121822203,-5.39351662111253,50.0824317919211));
#21433=CARTESIAN_POINT('Ctrl Pts',(11.073124940469,-5.3915958611814,50.0824317919208));
#21434=CARTESIAN_POINT('Ctrl Pts',(11.0642375260462,-5.38967730441635,50.0824317919204));
#21435=CARTESIAN_POINT('Ctrl Pts',(11.055349936817,-5.38776095106557,50.0824317919201));
#21436=CARTESIAN_POINT('Ctrl Pts',(7.4174461363494,-4.60335148320463,50.0824317917656));
#21437=CARTESIAN_POINT('Ctrl Pts',(3.74693618253599,-4.18752460344888,50.0824317918031));
#21438=CARTESIAN_POINT('Ctrl Pts',(0.0393470995888544,-4.1908181579504,
50.0824317919243));
#21439=CARTESIAN_POINT('Ctrl Pts',(0.0324484243578657,-4.19082428623548,
50.0824317919245));
#21440=CARTESIAN_POINT('Ctrl Pts',(0.0255496208096622,-4.19083186535561,
50.0824317919247));
#21441=CARTESIAN_POINT('Ctrl Pts',(0.0186506889146812,-4.19084089563808,
50.082431791925));
#21442=CARTESIAN_POINT('Ctrl Pts',(-0.901382134976211,-4.19204516267696,
50.0824317919539));
#21443=CARTESIAN_POINT('Ctrl Pts',(-1.82367679464876,-4.21882226363321,
50.0824317919392));
#21444=CARTESIAN_POINT('Ctrl Pts',(-2.7482570531487,-4.27143022964227,50.0824317919393));
#21445=CARTESIAN_POINT('Ctrl Pts',(-2.75919896624817,-4.27205281679695,
50.0824317919393));
#21446=CARTESIAN_POINT('Ctrl Pts',(-2.7701413179277,-4.27267902824778,50.0824317919394));
#21447=CARTESIAN_POINT('Ctrl Pts',(-2.78108410830146,-4.27330886465574,
50.0824317919394));
#21448=CARTESIAN_POINT('Ctrl Pts',(-3.70172929220981,-4.32629862648306,
50.0824317919395));
#21449=CARTESIAN_POINT('Ctrl Pts',(-4.616569426888,-4.40442769523306,50.0824317919392));
#21450=CARTESIAN_POINT('Ctrl Pts',(-5.52572806394492,-4.50641515619345,
50.0824317919393));
#21451=CARTESIAN_POINT('Ctrl Pts',(-5.53960751684282,-4.50797212337484,
50.0824317919393));
#21452=CARTESIAN_POINT('Ctrl Pts',(-5.55348564086543,-4.50953465011809,
50.0824317919393));
#21453=CARTESIAN_POINT('Ctrl Pts',(-5.56736243615774,-4.51110273180162,
50.0824317919393));
#21454=CARTESIAN_POINT('Ctrl Pts',(-6.6470334253265,-4.63310585043909,50.0824317919394));
#21455=CARTESIAN_POINT('Ctrl Pts',(-7.71878011925584,-4.78875206539942,
50.0824317919394));
#21456=CARTESIAN_POINT('Ctrl Pts',(-8.78314336260521,-4.9757301443796,50.0824317919394));
#21457=CARTESIAN_POINT('Ctrl Pts',(-9.5185957422456,-5.10492802300404,50.0824317919393));
#21458=CARTESIAN_POINT('Ctrl Pts',(-10.2505231824639,-5.24908423888419,
50.0824317919393));
#21459=CARTESIAN_POINT('Ctrl Pts',(-10.979107895046,-5.40742232363259,50.0824317919393));
#21460=CARTESIAN_POINT('Ctrl Pts',(-10.9937292654063,-5.41059988107961,
50.0824317919393));
#21461=CARTESIAN_POINT('Ctrl Pts',(-11.0083492885202,-5.41378314936643,
50.0824317919393));
#21462=CARTESIAN_POINT('Ctrl Pts',(-11.0229679658942,-5.41697212217387,
50.0824317919393));
#21463=CARTESIAN_POINT('Ctrl Pts',(-12.1324973546702,-5.65900900138861,
50.0824317919394));
#21464=CARTESIAN_POINT('Ctrl Pts',(-13.2343102827012,-5.93379674455981,
50.0824317919394));
#21465=CARTESIAN_POINT('Ctrl Pts',(-14.3290278568824,-6.23869144822421,
50.0824317919394));
#21466=CARTESIAN_POINT('Ctrl Pts',(-15.4414775636244,-6.5485248076935,50.0824317919394));
#21467=CARTESIAN_POINT('Ctrl Pts',(-16.5466002367016,-6.88944821125723,
50.0824317919394));
#21468=CARTESIAN_POINT('Ctrl Pts',(-17.6450618211739,-7.25863482930252,
50.0824317919394));
#21469=CARTESIAN_POINT('Ctrl Pts',(-18.7713890095441,-7.63718691648054,
50.0824317919394));
#21470=CARTESIAN_POINT('Ctrl Pts',(-19.8907128989818,-8.04545424379275,
50.0824317919394));
#21471=CARTESIAN_POINT('Ctrl Pts',(-21.0037656572773,-8.4803367087874,50.0824317919394));
#21472=CARTESIAN_POINT('Ctrl Pts',(-21.1815949414308,-8.54981664750956,
50.0824317919394));
#21473=CARTESIAN_POINT('Ctrl Pts',(-21.3592641797394,-8.61997584796747,
50.0824317919394));
#21474=CARTESIAN_POINT('Ctrl Pts',(-21.5367763897373,-8.69080155057986,
50.0824317919394));
#21475=CARTESIAN_POINT('Origin',(44.4585265683621,16.4830954176946,44.4574317919394));
#21476=CARTESIAN_POINT('Origin',(44.4585265683621,-8.87385981233827,44.4574317919394));
#21477=CARTESIAN_POINT('Origin',(44.4585265683621,-14.4544045823054,44.4574317919394));
#21478=CARTESIAN_POINT('Origin',(0.0835265683620477,16.4830954176946,50.0824317919394));
#21479=CARTESIAN_POINT('',(-44.2914734316384,16.1705954176946,50.082431791939));
#21480=CARTESIAN_POINT('',(-44.2914734316384,13.4386401876617,50.082431791939));
#21481=CARTESIAN_POINT('',(-44.2914734316384,16.4830954176946,50.082431791939));
#21482=CARTESIAN_POINT('',(-10.8649863601191,13.4386401876617,50.0824317919394));
#21483=CARTESIAN_POINT('',(0.0835265683620477,13.4386401876617,50.0824317919394));
#21484=CARTESIAN_POINT('',(-8.58213843785641,13.2555819259033,50.0824317919394));
#21485=CARTESIAN_POINT('Ctrl Pts',(-8.5821384378566,13.2555819259034,50.0824317919394));
#21486=CARTESIAN_POINT('Ctrl Pts',(-8.82298135330014,13.2969611280073,50.0824317919394));
#21487=CARTESIAN_POINT('Ctrl Pts',(-9.06501105460157,13.3294628821421,50.0824317919394));
#21488=CARTESIAN_POINT('Ctrl Pts',(-9.3077915193297,13.3553162053718,50.0824317919394));
#21489=CARTESIAN_POINT('Ctrl Pts',(-9.44488714767125,13.3699153107688,50.0824317919394));
#21490=CARTESIAN_POINT('Ctrl Pts',(-9.58222240123873,13.3823932020222,50.0824317919394));
#21491=CARTESIAN_POINT('Ctrl Pts',(-9.71971984082492,13.3931443825079,50.0824317919394));
#21492=CARTESIAN_POINT('Ctrl Pts',(-9.71978638257171,13.3931495855308,50.0824317919394));
#21493=CARTESIAN_POINT('Ctrl Pts',(-9.71985292434008,13.3931547881239,50.0824317919394));
#21494=CARTESIAN_POINT('Ctrl Pts',(-9.71991946613004,13.3931599902873,50.0824317919394));
#21495=CARTESIAN_POINT('Ctrl Pts',(-10.1009757205579,13.4229505456848,50.0824317919394));
#21496=CARTESIAN_POINT('Ctrl Pts',(-10.4826417866386,13.4386401851025,50.0824317919394));
#21497=CARTESIAN_POINT('Ctrl Pts',(-10.8649863601191,13.4386401876617,50.0824317919394));
#21498=CARTESIAN_POINT('',(8.74919157458055,13.2555819259033,50.0824317919394));
#21499=CARTESIAN_POINT('Ctrl Pts',(-8.58213843785641,13.2555819259033,50.0824317919394));
#21500=CARTESIAN_POINT('Ctrl Pts',(-7.37516628549685,13.0482120850067,50.0824317919394));
#21501=CARTESIAN_POINT('Ctrl Pts',(-6.16542111429013,12.8826695784009,50.0824317919394));
#21502=CARTESIAN_POINT('Ctrl Pts',(-4.95280295520423,12.7604365635511,50.0824317919394));
#21503=CARTESIAN_POINT('Ctrl Pts',(-3.75084982134647,12.6392785929576,50.0824317919394));
#21504=CARTESIAN_POINT('Ctrl Pts',(-2.54607400932527,12.5606716819902,50.0824317919394));
#21505=CARTESIAN_POINT('Ctrl Pts',(-1.3383838944826,12.5260083291904,50.0824317919394));
#21506=CARTESIAN_POINT('Ctrl Pts',(-0.868840927440839,12.5125314170909,
50.0824317919394));
#21507=CARTESIAN_POINT('Ctrl Pts',(-0.398857493567957,12.5056965050877,
50.0824317919394));
#21508=CARTESIAN_POINT('Ctrl Pts',(0.0715715529620946,12.5055833090051,
50.0824317919394));
#21509=CARTESIAN_POINT('Ctrl Pts',(0.071725964608064,12.5055832718501,50.0824317919394));
#21510=CARTESIAN_POINT('Ctrl Pts',(0.0718803762799654,12.5055832354192,
50.0824317919394));
#21511=CARTESIAN_POINT('Ctrl Pts',(0.0720347879778126,12.5055831997124,
50.0824317919394));
#21512=CARTESIAN_POINT('Ctrl Pts',(0.535468761960413,12.5054760332808,50.0824317919394));
#21513=CARTESIAN_POINT('Ctrl Pts',(0.99956602790721,12.5119501585725,50.0824317919398));
#21514=CARTESIAN_POINT('Ctrl Pts',(1.4637993848865,12.5248910213249,50.0824317919345));
#21515=CARTESIAN_POINT('Ctrl Pts',(1.9305422533797,12.5379018386455,50.0824317919291));
#21516=CARTESIAN_POINT('Ctrl Pts',(2.39742400942509,12.5574495854694,50.0824317919166));
#21517=CARTESIAN_POINT('Ctrl Pts',(2.86391070485841,12.5834701483563,50.0824317919075));
#21518=CARTESIAN_POINT('Ctrl Pts',(3.31881454076369,12.6088446209523,50.0824317918986));
#21519=CARTESIAN_POINT('Ctrl Pts',(3.77334384985895,12.6403747667456,50.0824317918966));
#21520=CARTESIAN_POINT('Ctrl Pts',(4.22698698482929,12.6780474220166,50.082431791909));
#21521=CARTESIAN_POINT('Ctrl Pts',(4.29353516680801,12.6835738954168,50.0824317919108));
#21522=CARTESIAN_POINT('Ctrl Pts',(4.36006423101712,12.6892326346471,50.0824317919129));
#21523=CARTESIAN_POINT('Ctrl Pts',(4.42657250848413,12.6950236788102,50.0824317919151));
#21524=CARTESIAN_POINT('Ctrl Pts',(4.43223940031558,12.6955171094344,50.0824317919153));
#21525=CARTESIAN_POINT('Ctrl Pts',(4.43790610260004,12.6960114970058,50.0824317919155));
#21526=CARTESIAN_POINT('Ctrl Pts',(4.44357261344172,12.6965068414395,50.0824317919157));
#21527=CARTESIAN_POINT('Ctrl Pts',(5.29122519267014,12.7706053473037,50.0824317919435));
#21528=CARTESIAN_POINT('Ctrl Pts',(6.13664037252339,12.865971941344,50.082431791939));
#21529=CARTESIAN_POINT('Ctrl Pts',(6.97986484277041,12.9818931833795,50.0824317919393));
#21530=CARTESIAN_POINT('Ctrl Pts',(7.57070936299085,13.0631188036627,50.0824317919395));
#21531=CARTESIAN_POINT('Ctrl Pts',(8.16047853122286,13.1544351596487,50.0824317919394));
#21532=CARTESIAN_POINT('Ctrl Pts',(8.74919157458055,13.2555819259033,50.0824317919394));
#21533=CARTESIAN_POINT('',(11.0320394968433,13.4386401876617,50.0824317919394));
#21534=CARTESIAN_POINT('Ctrl Pts',(11.0320394968433,13.4386401876617,50.0824317919394));
#21535=CARTESIAN_POINT('Ctrl Pts',(10.7909520272503,13.4386401861139,50.0824317919394));
#21536=CARTESIAN_POINT('Ctrl Pts',(10.5500159553784,13.4323889945159,50.0824317919395));
#21537=CARTESIAN_POINT('Ctrl Pts',(10.3093654004934,13.4203066131624,50.0824317919393));
#21538=CARTESIAN_POINT('Ctrl Pts',(10.1686166605505,13.4132400183987,50.0824317919392));
#21539=CARTESIAN_POINT('Ctrl Pts',(10.0279654246317,13.4041776979188,50.082431791939));
#21540=CARTESIAN_POINT('Ctrl Pts',(9.88743785753373,13.3931955538157,50.0824317919381));
#21541=CARTESIAN_POINT('Ctrl Pts',(9.88718986684206,13.3931761734936,50.0824317919381));
#21542=CARTESIAN_POINT('Ctrl Pts',(9.88694187686581,13.3931567875853,50.0824317919381));
#21543=CARTESIAN_POINT('Ctrl Pts',(9.88669388760501,13.3931373960886,50.0824317919381));
#21544=CARTESIAN_POINT('Ctrl Pts',(9.50564813228723,13.363341559395,50.0824317919358));
#21545=CARTESIAN_POINT('Ctrl Pts',(9.12614644683353,13.3203465159016,50.0824317919394));
#21546=CARTESIAN_POINT('Ctrl Pts',(8.74919157458055,13.2555819259033,50.0824317919394));
#21547=CARTESIAN_POINT('',(44.458526568362,13.4386401876617,50.0824317919394));
#21548=CARTESIAN_POINT('',(0.0835265683620477,13.4386401876617,50.0824317919394));
#21549=CARTESIAN_POINT('',(44.458526568362,16.1705954176946,50.0824317919394));
#21550=CARTESIAN_POINT('',(44.458526568362,16.4830954176946,50.0824317919394));
#21551=CARTESIAN_POINT('',(-44.2914734316384,16.1705954176946,50.0824317919394));
#21552=CARTESIAN_POINT('Origin',(44.4585265683621,16.4830954176946,44.4574317919394));
#21553=CARTESIAN_POINT('Origin',(44.4585265683621,13.4386401876617,44.4574317919394));
#21554=CARTESIAN_POINT('Origin',(44.4585265683621,16.1705954176946,44.4574317919394));
#21555=CARTESIAN_POINT('Origin',(0.0835265683620477,16.4830954176946,0.0824317919394229));
#21556=CARTESIAN_POINT('',(48.4087001792127,16.3915662868156,22.6760194541559));
#21557=CARTESIAN_POINT('',(48.428660091855,11.5746245485365,4.30318207805399));
#21558=CARTESIAN_POINT('Ctrl Pts',(48.4087001792126,16.3915662868154,22.6760194541555));
#21559=CARTESIAN_POINT('Ctrl Pts',(48.4133626632511,15.1541680928392,19.7444122941847));
#21560=CARTESIAN_POINT('Ctrl Pts',(48.41771013248,14.0894359483376,16.7558018285945));
#21561=CARTESIAN_POINT('Ctrl Pts',(48.4229917226254,12.8480220597894,12.1554610849062));
#21562=CARTESIAN_POINT('Ctrl Pts',(48.4245437904912,12.4934998941785,10.599655099974));
#21563=CARTESIAN_POINT('Ctrl Pts',(48.4270638166904,11.9258476364963,7.46837373314965));
#21564=CARTESIAN_POINT('Ctrl Pts',(48.4280340859824,11.7120008366799,5.88986732862775));
#21565=CARTESIAN_POINT('Ctrl Pts',(48.4286600918172,11.5746245485738,4.30318207891633));
#21566=CARTESIAN_POINT('',(4.30427685494149,11.5746245485738,48.4275653154293));
#21567=CARTESIAN_POINT('Origin',(0.0835265683620477,11.5746245485738,0.0824317919394229));
#21568=CARTESIAN_POINT('',(22.6771142305786,16.3915662868157,48.4076054027901));
#21569=CARTESIAN_POINT('Ctrl Pts',(4.30427685533877,11.5746245485738,48.4275653153946));
#21570=CARTESIAN_POINT('Ctrl Pts',(5.88955930980395,11.7118793817134,48.4269398630142));
#21571=CARTESIAN_POINT('Ctrl Pts',(7.46274649560755,11.9249456441311,48.4259731407403));
#21572=CARTESIAN_POINT('Ctrl Pts',(10.5868505406711,12.4906656417943,48.4234615008534));
#21573=CARTESIAN_POINT('Ctrl Pts',(12.140036765244,12.843980457976,48.4219144210431));
#21574=CARTESIAN_POINT('Ctrl Pts',(16.7459605252979,14.0856585112706,48.4166308714132));
#21575=CARTESIAN_POINT('Ctrl Pts',(19.7463324981469,15.1545164964592,48.4122665740529));
#21576=CARTESIAN_POINT('Ctrl Pts',(22.677114230578,16.3915662868154,48.40760540279));
#21577=CARTESIAN_POINT('Origin',(0.0835265683620477,16.3915662868154,0.0824317919394229));
#21578=CARTESIAN_POINT('Origin',(0.0835265683620484,-85.4775827009602,48.5199317919394));
#21579=CARTESIAN_POINT('',(-4.11800505968102,11.7955954176946,48.5199317919394));
#21580=CARTESIAN_POINT('',(0.0835265683619702,11.6131136241746,48.5199317919394));
#21581=CARTESIAN_POINT('Origin',(0.0850736516346928,84.3502669679634,48.5199317979947));
#21582=CARTESIAN_POINT('',(-21.3522104186698,16.1706033824526,48.5199317918264));
#21583=CARTESIAN_POINT('Ctrl Pts',(-4.11800505968102,11.7955954176946,48.5199317919393));
#21584=CARTESIAN_POINT('Ctrl Pts',(-5.3330850955866,11.9012754509056,48.5199317919355));
#21585=CARTESIAN_POINT('Ctrl Pts',(-6.54284928166413,12.052058373043,48.5199317917982));
#21586=CARTESIAN_POINT('Ctrl Pts',(-7.74758204934735,12.2455340355694,48.5199317918421));
#21587=CARTESIAN_POINT('Ctrl Pts',(-8.00842309407842,12.2874241503709,48.5199317918516));
#21588=CARTESIAN_POINT('Ctrl Pts',(-8.26902825280743,12.3313158148411,48.5199317918681));
#21589=CARTESIAN_POINT('Ctrl Pts',(-8.52940037578031,12.3771848834521,48.5199317918868));
#21590=CARTESIAN_POINT('Ctrl Pts',(-8.60796598979772,12.3910255799855,48.5199317918924));
#21591=CARTESIAN_POINT('Ctrl Pts',(-8.68650600951455,12.4050450140606,48.5199317918896));
#21592=CARTESIAN_POINT('Ctrl Pts',(-8.76502160741265,12.4192427232393,48.5199317918772));
#21593=CARTESIAN_POINT('Ctrl Pts',(-9.31742370497652,12.5191317203411,48.5199317917904));
#21594=CARTESIAN_POINT('Ctrl Pts',(-9.86933137746676,12.628070795559,48.5199317909336));
#21595=CARTESIAN_POINT('Ctrl Pts',(-10.4199054294347,12.7454889373136,48.5199317856301));
#21596=CARTESIAN_POINT('Ctrl Pts',(-10.9847756532994,12.8659559512995,48.5199317801888));
#21597=CARTESIAN_POINT('Ctrl Pts',(-11.5482433946011,12.9953485172464,48.5199317698611));
#21598=CARTESIAN_POINT('Ctrl Pts',(-12.1093930468112,13.1331031830766,48.5199317678938));
#21599=CARTESIAN_POINT('Ctrl Pts',(-12.3711272379419,13.1973553943959,48.5199317669762));
#21600=CARTESIAN_POINT('Ctrl Pts',(-12.6323568698691,13.2634275009716,48.5199317681592));
#21601=CARTESIAN_POINT('Ctrl Pts',(-12.8929871215291,13.3312657045529,48.5199317717506));
#21602=CARTESIAN_POINT('Ctrl Pts',(-13.0886265997407,13.3821877700727,48.5199317744464));
#21603=CARTESIAN_POINT('Ctrl Pts',(-13.2839532567454,13.4341067575178,48.5199317766964));
#21604=CARTESIAN_POINT('Ctrl Pts',(-13.4789066329929,13.4869947668886,48.5199317786076));
#21605=CARTESIAN_POINT('Ctrl Pts',(-14.2827231347708,13.7050584675371,48.5199317864876));
#21606=CARTESIAN_POINT('Ctrl Pts',(-15.0813881500244,13.9395350034094,48.5199317889602));
#21607=CARTESIAN_POINT('Ctrl Pts',(-15.8751970172333,14.1892982824324,48.5199317903271));
#21608=CARTESIAN_POINT('Ctrl Pts',(-16.6833025247604,14.4435598429844,48.5199317917186));
#21609=CARTESIAN_POINT('Ctrl Pts',(-17.4863754330999,14.7136635664768,48.5199317918044));
#21610=CARTESIAN_POINT('Ctrl Pts',(-18.2847477442816,14.9983707526771,48.5199317918862));
#21611=CARTESIAN_POINT('Ctrl Pts',(-19.1070061411662,15.2915959450188,48.5199317919706));
#21612=CARTESIAN_POINT('Ctrl Pts',(-19.9242785136404,15.6003113768466,48.5199317919394));
#21613=CARTESIAN_POINT('Ctrl Pts',(-20.7369483477271,15.9231126709707,48.5199317919394));
#21614=CARTESIAN_POINT('Ctrl Pts',(-20.9423235837733,16.0046899477393,48.5199317919394));
#21615=CARTESIAN_POINT('Ctrl Pts',(-21.1474049737681,16.0871665859416,48.5199317919394));
#21616=CARTESIAN_POINT('Ctrl Pts',(-21.3521989016608,16.170519439565,48.5199317919394));
#21617=CARTESIAN_POINT('',(21.5192634427593,16.17060336129,48.5199317918263));
#21618=CARTESIAN_POINT('',(0.0835265683620484,16.1705954176946,48.5199317919394));
#21619=CARTESIAN_POINT('',(4.28505819640496,11.7955954176946,48.5199317919394));
#21620=CARTESIAN_POINT('Ctrl Pts',(21.5192519564043,16.1705196413466,48.5199317919394));
#21621=CARTESIAN_POINT('Ctrl Pts',(20.7158295319576,15.8435202227492,48.5199317919394));
#21622=CARTESIAN_POINT('Ctrl Pts',(19.9079782705932,15.5300086685378,48.5199317919526));
#21623=CARTESIAN_POINT('Ctrl Pts',(19.0953265097735,15.2313679634678,48.5199317919262));
#21624=CARTESIAN_POINT('Ctrl Pts',(18.299910033755,14.9390610385645,48.5199317919003));
#21625=CARTESIAN_POINT('Ctrl Pts',(17.4998944429049,14.6610010604542,48.5199317919232));
#21626=CARTESIAN_POINT('Ctrl Pts',(16.6949498262278,14.3984390229379,48.5199317911674));
#21627=CARTESIAN_POINT('Ctrl Pts',(15.9108077115892,14.1426624799854,48.5199317904312));
#21628=CARTESIAN_POINT('Ctrl Pts',(15.1219880157985,13.90159329815,48.519931789089));
#21629=CARTESIAN_POINT('Ctrl Pts',(14.3282043783767,13.6763418781801,48.5199317840016));
#21630=CARTESIAN_POINT('Ctrl Pts',(14.1012822681381,13.6119483518537,48.5199317825472));
#21631=CARTESIAN_POINT('Ctrl Pts',(13.8739546053117,13.5488472152168,48.5199317807643));
#21632=CARTESIAN_POINT('Ctrl Pts',(13.6462149928204,13.4870636734954,48.5199317785163));
#21633=CARTESIAN_POINT('Ctrl Pts',(13.4512631341532,13.4341751304708,48.5199317765919));
#21634=CARTESIAN_POINT('Ctrl Pts',(13.255935603651,13.3822549873816,48.5199317743262));
#21635=CARTESIAN_POINT('Ctrl Pts',(13.0602932043519,13.3313312754882,48.5199317716117));
#21636=CARTESIAN_POINT('Ctrl Pts',(12.500626902414,13.1856558716985,48.5199317638463));
#21637=CARTESIAN_POINT('Ctrl Pts',(11.9381747386843,13.0481153498591,48.5199317690783));
#21638=CARTESIAN_POINT('Ctrl Pts',(11.3738769394113,12.9192577967887,48.5199317762763));
#21639=CARTESIAN_POINT('Ctrl Pts',(10.8211684440881,12.7930466643683,48.5199317833265));
#21640=CARTESIAN_POINT('Ctrl Pts',(10.2666880661914,12.6751650328318,48.5199317893989));
#21641=CARTESIAN_POINT('Ctrl Pts',(9.71130192517919,12.5661734820257,48.5199317909776));
#21642=CARTESIAN_POINT('Ctrl Pts',(9.45179182555766,12.5152460171163,48.5199317917152));
#21643=CARTESIAN_POINT('Ctrl Pts',(9.19208383600685,12.4662602455223,48.5199317918358));
#21644=CARTESIAN_POINT('Ctrl Pts',(8.93226615131867,12.4192773203273,48.5199317918769));
#21645=CARTESIAN_POINT('Ctrl Pts',(8.85373981326765,12.4050773744271,48.5199317918893));
#21646=CARTESIAN_POINT('Ctrl Pts',(8.77518928258344,12.3910557938706,48.5199317918922));
#21647=CARTESIAN_POINT('Ctrl Pts',(8.69661339645869,12.377213039333,48.5199317918865));
#21648=CARTESIAN_POINT('Ctrl Pts',(7.49688801165072,12.1658567971894,48.5199317918003));
#21649=CARTESIAN_POINT('Ctrl Pts',(6.29223043630813,11.9964818494364,48.5199317918738));
#21650=CARTESIAN_POINT('Ctrl Pts',(5.08236080976824,11.871466704724,48.5199317919214));
#21651=CARTESIAN_POINT('Ctrl Pts',(4.81684531529824,11.8440311387453,48.5199317919318));
#21652=CARTESIAN_POINT('Ctrl Pts',(4.55107877638799,11.8187322176555,48.5199317919385));
#21653=CARTESIAN_POINT('Ctrl Pts',(4.28505819640497,11.7955954176945,48.5199317919394));
#21654=CARTESIAN_POINT('Origin',(0.0819794773143091,84.3502670306517,48.5199317979381));
#21655=CARTESIAN_POINT('Origin',(39.8582830101054,16.4855954176946,41.1830134484075));
#21656=CARTESIAN_POINT('',(34.7649027499964,-3.61941807409669,36.0896331882986));
#21657=CARTESIAN_POINT('',(38.0393490816114,-8.24885981233827,39.3640795199135));
#21658=CARTESIAN_POINT('Ctrl Pts',(34.7649027499964,-3.61941807409669,36.0896331882986));
#21659=CARTESIAN_POINT('Ctrl Pts',(35.3114139634271,-4.3920600802535,36.6361444017293));
#21660=CARTESIAN_POINT('Ctrl Pts',(35.8579212247445,-5.16470767732065,37.1826516630466));
#21661=CARTESIAN_POINT('Ctrl Pts',(36.9494030102706,-6.70785538323105,38.2741334485728));
#21662=CARTESIAN_POINT('Ctrl Pts',(37.4943775524999,-7.4783554666459,38.819107990802));
#21663=CARTESIAN_POINT('Ctrl Pts',(38.0393490816114,-8.24885981233827,39.3640795199135));
#21664=CARTESIAN_POINT('',(39.195370402743,-8.24885981233827,40.5201008410451));
#21665=CARTESIAN_POINT('',(35.3869530268201,12.8136401876617,36.7116834651222));
#21666=CARTESIAN_POINT('',(35.3001596224904,12.8136401876617,36.6248900607926));
#21667=CARTESIAN_POINT('',(34.7649027499964,11.9341984494202,36.0896331882986));
#21668=CARTESIAN_POINT('',(35.3869530268201,12.8136401876617,36.7116834651222));
#21669=CARTESIAN_POINT('',(34.7649027499964,-3.74885981233827,36.0896331882986));
#21670=CARTESIAN_POINT('Origin',(41.1841082248301,16.4855954176946,39.8571882336827));
#21671=CARTESIAN_POINT('',(39.3651742963361,-8.24885981233827,38.0382543051887));
#21672=CARTESIAN_POINT('',(39.2780566719443,-8.24885981233827,37.9511366807969));
#21673=CARTESIAN_POINT('',(36.0907279647212,-3.61941807409669,34.7638079735738));
#21674=CARTESIAN_POINT('Ctrl Pts',(39.3651742963361,-8.24885981233827,38.0382543051887));
#21675=CARTESIAN_POINT('Ctrl Pts',(38.8202027672246,-7.4783554666459,37.4932827760772));
#21676=CARTESIAN_POINT('Ctrl Pts',(38.2752282249954,-6.70785538323104,36.948308233848));
#21677=CARTESIAN_POINT('Ctrl Pts',(37.1837464394692,-5.16470767732064,35.8568264483218));
#21678=CARTESIAN_POINT('Ctrl Pts',(36.6372391781519,-4.3920600802535,35.3103191870045));
#21679=CARTESIAN_POINT('Ctrl Pts',(36.0907279647212,-3.61941807409669,34.7638079735738));
#21680=CARTESIAN_POINT('',(36.0907279647215,11.9341984494207,34.7638079735741));
#21681=CARTESIAN_POINT('',(36.0907279647212,12.0636401876617,34.7638079735738));
#21682=CARTESIAN_POINT('',(36.7127782415448,12.8136401876617,35.3858582503974));
#21683=CARTESIAN_POINT('',(36.0907279647212,11.9341984494202,34.7638079735738));
#21684=CARTESIAN_POINT('',(40.5211956174677,12.8136401876617,39.1942756263203));
#21685=CARTESIAN_POINT('Origin',(0.0835265683620477,-11.0169045823054,0.0824317919394229));
#21686=CARTESIAN_POINT('',(10.0669432604883,-11.3294045823054,19.5464246030606));
#21687=CARTESIAN_POINT('',(10.0669432604883,-14.4544045823054,19.5464246030606));
#21688=CARTESIAN_POINT('',(10.0669432604883,-11.0169045823054,19.5464246030606));
#21689=CARTESIAN_POINT('Origin',(0.0835265683620477,-14.4544045823054,0.0824317919394229));
#21690=CARTESIAN_POINT('Origin',(0.0835265683620477,-11.3294045823054,0.0824317919394229));
#21691=CARTESIAN_POINT('Origin',(0.0835265683620477,-13.2044045823054,0.0824317919394229));
#21692=CARTESIAN_POINT('',(34.3599945679822,-13.2044045823054,34.7477781982718));
#21693=CARTESIAN_POINT('',(41.4437380877936,-13.2044045823054,37.0836464997312));
#21694=CARTESIAN_POINT('',(41.7058392642912,-13.2044045823054,37.1700745060874));
#21695=CARTESIAN_POINT('',(40.2796596827637,-13.2044045823054,38.3450489192809));
#21696=CARTESIAN_POINT('Origin',(0.0835265683620477,-13.2044045823054,0.0824317919394229));
#21697=CARTESIAN_POINT('',(33.0778695430594,-13.2044045823054,35.9702546803237));
#21698=CARTESIAN_POINT('',(-7.35411383562686,-13.2044045823054,22.6377860392341));
#21699=CARTESIAN_POINT('Origin',(0.0835265683620477,-13.2044045823054,0.0824317919394229));
#21700=CARTESIAN_POINT('Origin',(-7.45197752515304,16.4855954176946,22.9345670161721));
#21701=CARTESIAN_POINT('',(32.9800058535332,-12.8919045823054,36.2670356572618));
#21702=CARTESIAN_POINT('',(39.2345740945198,-12.8919045823054,38.3294829568536));
#21703=CARTESIAN_POINT('',(-7.45197752515304,-12.8919045823054,22.9345670161721));
#21704=CARTESIAN_POINT('',(32.9800027480559,-7.07886051013688,36.2670346332676));
#21705=CARTESIAN_POINT('Ctrl Pts',(39.2345740945198,-12.8919045823054,38.3294829568536));
#21706=CARTESIAN_POINT('Ctrl Pts',(37.5830392601106,-11.3339023349487,37.7848884415858));
#21707=CARTESIAN_POINT('Ctrl Pts',(35.9239895753391,-9.78474033199855,37.2378159002995));
#21708=CARTESIAN_POINT('Ctrl Pts',(34.2546478225026,-8.24794399593134,36.6873495439375));
#21709=CARTESIAN_POINT('Ctrl Pts',(33.8304517690206,-7.85742902818579,36.5474706632071));
#21710=CARTESIAN_POINT('Ctrl Pts',(33.4055909787826,-7.46771271821857,36.4073725851676));
#21711=CARTESIAN_POINT('Ctrl Pts',(32.9800195165679,-7.07885337126715,36.267040162655));
#21712=CARTESIAN_POINT('',(32.9800058535332,16.4855954176946,36.2670356572618));
#21713=CARTESIAN_POINT('Origin',(0.0835265683620477,-13.2044045823054,0.0824317919394229));
#21714=CARTESIAN_POINT('',(40.0376426042469,-13.2044045823054,28.0150491378139));
#21715=CARTESIAN_POINT('',(46.6900312637982,-13.2044045823054,30.2086779380909));
#21716=CARTESIAN_POINT('',(46.8934224522321,-13.2044045823054,30.2757462937605));
#21717=CARTESIAN_POINT('',(45.7901549780056,-13.2044045823054,31.5572011510148));
#21718=CARTESIAN_POINT('Origin',(0.0835265683620477,-13.2044045823054,0.0824317919394229));
#21719=CARTESIAN_POINT('',(39.0755546384815,-13.2044045823054,29.3430580152282));
#21720=CARTESIAN_POINT('',(-4.79490764946354,-13.2044045823054,14.87674907248));
#21721=CARTESIAN_POINT('Origin',(0.0835265683620477,-13.2044045823054,0.0824317919394229));
#21722=CARTESIAN_POINT('Origin',(-4.20772551230653,16.4855954176946,13.0960632108515));
#21723=CARTESIAN_POINT('',(46.3272934177549,-12.8919045823054,29.7600133527852));
#21724=CARTESIAN_POINT('Ctrl Pts',(40.1355068578762,-6.59534981976388,27.7182683468891));
#21725=CARTESIAN_POINT('Ctrl Pts',(42.2041064756925,-8.68909917313972,28.4003902026783));
#21726=CARTESIAN_POINT('Ctrl Pts',(44.2674821932045,-10.7885698299899,29.0807894744839));
#21727=CARTESIAN_POINT('Ctrl Pts',(46.327293417755,-12.8919045823054,29.7600133527852));
#21728=CARTESIAN_POINT('',(39.9141752801041,-12.8919045823054,27.6452841380193));
#21729=CARTESIAN_POINT('Origin',(0.0835265683620477,15.5455954176946,0.0824317919394229));
#21730=CARTESIAN_POINT('',(29.1308110078832,16.1705954176946,46.7863424064645));
#21731=CARTESIAN_POINT('Origin',(0.0835265683620477,16.1705954176946,0.0824317919394229));
#21732=CARTESIAN_POINT('',(29.1308110078832,15.8580954176946,46.7863424064645));
#21733=CARTESIAN_POINT('',(29.1308110078832,15.5455954176946,46.7863424064645));
#21734=CARTESIAN_POINT('Origin',(0.0835265683620477,15.8580954176946,0.0824317919394229));
#21735=CARTESIAN_POINT('Origin',(48.5210265683621,15.5455954176946,42.8336341598436));
#21736=CARTESIAN_POINT('',(48.5210265683621,15.8580954176946,35.8884670232579));
#21737=CARTESIAN_POINT('',(48.5210265683621,15.8580954176946,42.8336341598436));
#21738=CARTESIAN_POINT('',(48.5210265683621,16.1705954176946,35.8884670232579));
#21739=CARTESIAN_POINT('',(48.5210265683621,15.5455954176946,35.8884670232579));
#21740=CARTESIAN_POINT('',(48.5210265683621,16.1705954176946,29.6248403980433));
#21741=CARTESIAN_POINT('Origin',(26.1374820022305,15.5455954176946,48.5199317919394));
#21742=CARTESIAN_POINT('',(29.625935174466,15.8580954176946,48.5199317919394));
#21743=CARTESIAN_POINT('',(29.625935174466,16.1705954176946,48.5199317919394));
#21744=CARTESIAN_POINT('',(29.625935174466,16.4830954176946,48.5199317919394));
#21745=CARTESIAN_POINT('',(40.162361854341,16.1705954176946,48.5199317919394));
#21746=CARTESIAN_POINT('',(40.162361854341,16.1705954176946,48.5199317919394));
#21747=CARTESIAN_POINT('',(40.162361854341,15.8580954176946,48.5199317919394));
#21748=CARTESIAN_POINT('',(40.162361854341,15.5455954176946,48.5199317919394));
#21749=CARTESIAN_POINT('',(26.1374820022305,15.8580954176946,48.5199317919394));
#21750=CARTESIAN_POINT('Origin',(0.0835265683620477,15.5455954176946,0.0824317919394229));
#21751=CARTESIAN_POINT('',(48.2085265683621,15.5455954176946,35.8884670232579));
#21752=CARTESIAN_POINT('',(46.958526568362,15.5455954176946,35.8884670232579));
#21753=CARTESIAN_POINT('',(0.0835265683620477,15.5455954176946,35.8884670232579));
#21754=CARTESIAN_POINT('',(48.2085265683621,15.5455954176946,29.6248403980433));
#21755=CARTESIAN_POINT('',(48.2085265683621,15.5455954176946,0.0824317919394229));
#21756=CARTESIAN_POINT('',(47.0528003113788,15.5455954176946,29.2947576203215));
#21757=CARTESIAN_POINT('Origin',(47.583526568362,15.5455954176946,29.6248403980433));
#21758=CARTESIAN_POINT('',(29.2958523967441,15.5455954176946,47.0517055349562));
#21759=CARTESIAN_POINT('Origin',(0.0835265683620477,15.5455954176946,0.0824317919394229));
#21760=CARTESIAN_POINT('',(29.625935174466,15.5455954176946,48.2074317919394));
#21761=CARTESIAN_POINT('Origin',(29.625935174466,15.5455954176946,47.5824317919394));
#21762=CARTESIAN_POINT('',(40.162361854341,15.5455954176946,48.2074317919394));
#21763=CARTESIAN_POINT('',(0.0835265683619977,15.5455954176946,48.2074317919394));
#21764=CARTESIAN_POINT('',(40.667792997167,15.5455954176946,47.2147847331159));
#21765=CARTESIAN_POINT('Origin',(40.162361854341,15.5455954176946,47.5824317919394));
#21766=CARTESIAN_POINT('Origin',(44.4585265683621,15.5455954176946,44.4574317919394));
#21767=CARTESIAN_POINT('',(46.9585265683621,15.5455954176946,38.3884670232579));
#21768=CARTESIAN_POINT('',(0.0835265683620477,15.5455954176946,38.3884670232579));
#21769=CARTESIAN_POINT('',(46.9585265683619,15.5455954176946,0.0824317919392602));
#21770=CARTESIAN_POINT('Origin',(29.625935174466,15.5455954176946,47.5824317919394));
#21771=CARTESIAN_POINT('Origin',(29.625935174466,15.8580954176946,47.5824317919394));
#21772=CARTESIAN_POINT('Origin',(29.625935174466,16.1705954176946,47.5824317919394));
#21773=CARTESIAN_POINT('Origin',(47.583526568362,15.5455954176946,40.1612670779183));
#21774=CARTESIAN_POINT('Origin',(40.162361854341,15.5455954176946,47.5824317919394));
#21775=CARTESIAN_POINT('Origin',(40.162361854341,15.8580954176946,47.5824317919394));
#21776=CARTESIAN_POINT('Origin',(40.162361854341,16.1705954176946,47.5824317919394));
#21777=CARTESIAN_POINT('Origin',(0.0835265683620477,-6.01690458230549,0.0824317919394229));
#21778=CARTESIAN_POINT('',(-31.5165682646525,-13.2959337131846,45.9710537470232));
#21779=CARTESIAN_POINT('',(-30.1626755346769,-13.2959337131846,46.8745131384048));
#21780=CARTESIAN_POINT('Origin',(0.0835265683620477,-13.2959337131846,0.0824317919394229));
#21781=CARTESIAN_POINT('',(-29.4155943178386,-12.6709337131846,46.6106860996161));
#21782=CARTESIAN_POINT('Ctrl Pts',(-30.1626755346769,-13.2959337131846,
46.8745131384048));
#21783=CARTESIAN_POINT('Ctrl Pts',(-30.128258496796,-13.2959337131846,46.8967601651148));
#21784=CARTESIAN_POINT('Ctrl Pts',(-30.0920298432681,-13.2919430659205,
46.9153675825233));
#21785=CARTESIAN_POINT('Ctrl Pts',(-30.0551006644128,-13.2842290832339,
46.929952148959));
#21786=CARTESIAN_POINT('Ctrl Pts',(-30.0180600299975,-13.2764918190586,
46.9445807329187));
#21787=CARTESIAN_POINT('Ctrl Pts',(-29.9803129154874,-13.2650083398877,
46.9551627917423));
#21788=CARTESIAN_POINT('Ctrl Pts',(-29.9429700957448,-13.2500137812989,
46.9612766845548));
#21789=CARTESIAN_POINT('Ctrl Pts',(-29.9293044928118,-13.244526523367,46.96351406331));
#21790=CARTESIAN_POINT('Ctrl Pts',(-29.9156930611522,-13.238568757885,46.9651526829848));
#21791=CARTESIAN_POINT('Ctrl Pts',(-29.9021905910678,-13.232151003965,46.9661704507551));
#21792=CARTESIAN_POINT('Ctrl Pts',(-29.9019147572162,-13.2320198995247,
46.9661912421216));
#21793=CARTESIAN_POINT('Ctrl Pts',(-29.9016389697338,-13.2318886036912,
46.9662117744956));
#21794=CARTESIAN_POINT('Ctrl Pts',(-29.9013632291097,-13.2317571165656,
46.9662320476885));
#21795=CARTESIAN_POINT('Ctrl Pts',(-29.8543113852301,-13.2093204091529,
46.9696914259059));
#21796=CARTESIAN_POINT('Ctrl Pts',(-29.8096740998552,-13.1821368365851,
46.9659209863793));
#21797=CARTESIAN_POINT('Ctrl Pts',(-29.7683137283865,-13.1520894283089,
46.9566376932634));
#21798=CARTESIAN_POINT('Ctrl Pts',(-29.7333029737206,-13.1266548782276,
46.9487795651511));
#21799=CARTESIAN_POINT('Ctrl Pts',(-29.7006405691595,-13.0991694705162,
46.9369724953244));
#21800=CARTESIAN_POINT('Ctrl Pts',(-29.670847712286,-13.0707895719797,46.92227614813));
#21801=CARTESIAN_POINT('Ctrl Pts',(-29.6705642512064,-13.0705195543472,
46.9221363212426));
#21802=CARTESIAN_POINT('Ctrl Pts',(-29.670281044226,-13.0702494422352,46.9219962204034));
#21803=CARTESIAN_POINT('Ctrl Pts',(-29.669998091945,-13.0699792367999,46.921855846619));
#21804=CARTESIAN_POINT('Ctrl Pts',(-29.649628163306,-13.0505269623229,46.9117502416691));
#21805=CARTESIAN_POINT('Ctrl Pts',(-29.6304171285035,-13.0305367697073,
46.9002697804115));
#21806=CARTESIAN_POINT('Ctrl Pts',(-29.6123668188922,-13.0101903794937,
46.8876291496845));
#21807=CARTESIAN_POINT('Ctrl Pts',(-29.6018341203628,-12.9983178743179,
46.8802531015425));
#21808=CARTESIAN_POINT('Ctrl Pts',(-29.5916957344855,-12.9863240855347,
46.8724825962677));
#21809=CARTESIAN_POINT('Ctrl Pts',(-29.5819448758312,-12.9742444051773,
46.8643639920203));
#21810=CARTESIAN_POINT('Ctrl Pts',(-29.5685981672066,-12.9577100691025,
46.853251468583));
#21811=CARTESIAN_POINT('Ctrl Pts',(-29.555981026384,-12.9410147689399,46.8414844826325));
#21812=CARTESIAN_POINT('Ctrl Pts',(-29.5440850848253,-12.9242496162066,
46.82917659869));
#21813=CARTESIAN_POINT('Ctrl Pts',(-29.538137114046,-12.9158670398399,46.8230226567187));
#21814=CARTESIAN_POINT('Ctrl Pts',(-29.5323694430285,-12.9074670004228,
46.8167334901675));
#21815=CARTESIAN_POINT('Ctrl Pts',(-29.5267810252359,-12.8990608878296,
46.810323293749));
#21816=CARTESIAN_POINT('Ctrl Pts',(-29.5211926074433,-12.8906547752363,
46.8039130973305));
#21817=CARTESIAN_POINT('Ctrl Pts',(-29.5157834428655,-12.8822425894822,
46.7973818710315));
#21818=CARTESIAN_POINT('Ctrl Pts',(-29.5105524846761,-12.8738357211132,
46.7907438089363));
#21819=CARTESIAN_POINT('Ctrl Pts',(-29.4940980968796,-12.8473912596422,
46.7698632658357));
#21820=CARTESIAN_POINT('Ctrl Pts',(-29.4792456474726,-12.8207472740157,
46.7477293519109));
#21821=CARTESIAN_POINT('Ctrl Pts',(-29.4659612746266,-12.7940681980352,
46.7245595323374));
#21822=CARTESIAN_POINT('Ctrl Pts',(-29.4623528891908,-12.7868214585523,
46.7182659992916));
#21823=CARTESIAN_POINT('Ctrl Pts',(-29.4588604654321,-12.7795722581758,
46.7118960192856));
#21824=CARTESIAN_POINT('Ctrl Pts',(-29.4554839045944,-12.7723242153339,
46.7054539678863));
#21825=CARTESIAN_POINT('Ctrl Pts',(-29.4432141529765,-12.745986266853,46.6820448322659));
#21826=CARTESIAN_POINT('Ctrl Pts',(-29.432470737787,-12.7196622748127,46.657684718712));
#21827=CARTESIAN_POINT('Ctrl Pts',(-29.4232215145298,-12.6935087390695,
46.6325807424414));
#21828=CARTESIAN_POINT('Ctrl Pts',(-29.420554704246,-12.6859679417359,46.6253425625187));
#21829=CARTESIAN_POINT('Ctrl Pts',(-29.4180123618763,-12.6784415052693,
46.6180426097208));
#21830=CARTESIAN_POINT('Ctrl Pts',(-29.4155943178386,-12.6709337131846,
46.6106860996161));
#21831=CARTESIAN_POINT('',(-27.2935253998822,-6.10843371318464,40.1519176123711));
#21832=CARTESIAN_POINT('Origin',(-79.3423351452487,-177.510308399964,197.496985230816));
#21833=CARTESIAN_POINT('',(-4.13722371802816,-6.1084337131593,48.4275653154203));
#21834=CARTESIAN_POINT('Origin',(0.0835265683620477,-6.10843371318469,0.0824317919394229));
#21835=CARTESIAN_POINT('',(-30.3451264940354,-14.6753754514266,48.394407142734));
#21836=CARTESIAN_POINT('Ctrl Pts',(-4.13722371861488,-6.10843371318471,
48.4275653153946));
#21837=CARTESIAN_POINT('Ctrl Pts',(-8.77470276505741,-6.50994980321315,
48.425735658919));
#21838=CARTESIAN_POINT('Ctrl Pts',(-13.2570072174814,-7.55645913600449,
48.420976017041));
#21839=CARTESIAN_POINT('Ctrl Pts',(-19.8170786877967,-9.80534906153842,
48.411872783885));
#21840=CARTESIAN_POINT('Ctrl Pts',(-21.9781883476615,-10.6692546575742,
48.4085130814623));
#21841=CARTESIAN_POINT('Ctrl Pts',(-26.2164003770554,-12.5596572871779,
48.4015713432632));
#21842=CARTESIAN_POINT('Ctrl Pts',(-28.295928291696,-13.58630787804,48.3979874291792));
#21843=CARTESIAN_POINT('Ctrl Pts',(-30.3451264940348,-14.6753754514262,
48.3944071427339));
#21844=CARTESIAN_POINT('',(-31.9648970362172,-14.6753754514262,47.3354574511386));
#21845=CARTESIAN_POINT('Origin',(0.0835265683620477,-14.6753754514262,0.0824317919394229));
#21846=CARTESIAN_POINT('Origin',(321.770247061695,-1402.95413116479,-1241.46399381397));
#21847=CARTESIAN_POINT('Origin',(-15.0075716891166,-11.0169045823054,-4.8938661154125));
#21848=CARTESIAN_POINT('',(-29.2671708193829,-11.3294045823054,38.3497289413026));
#21849=CARTESIAN_POINT('',(-15.0075716891166,-11.3294045823054,-4.8938661154125));
#21850=CARTESIAN_POINT('',(-29.2671708193829,-12.8919045823054,38.3497289413026));
#21851=CARTESIAN_POINT('',(-29.2671708193829,-11.0169045823054,38.3497289413026));
#21852=CARTESIAN_POINT('',(-29.4738806318652,-13.5169045823054,38.9765961725324));
#21853=CARTESIAN_POINT('Ctrl Pts',(-29.4738806318652,-13.5169045823054,
38.9765961725324));
#21854=CARTESIAN_POINT('Ctrl Pts',(-29.4622411026741,-13.516904574972,38.9412981895812));
#21855=CARTESIAN_POINT('Ctrl Pts',(-29.4506274187098,-13.5137764691089,
38.9060785847456));
#21856=CARTESIAN_POINT('Ctrl Pts',(-29.4391842642702,-13.5077394335828,
38.8713761269725));
#21857=CARTESIAN_POINT('Ctrl Pts',(-29.4269102353917,-13.501264055768,38.8341539631789));
#21858=CARTESIAN_POINT('Ctrl Pts',(-29.414832028346,-13.491442168195,38.797525647788));
#21859=CARTESIAN_POINT('Ctrl Pts',(-29.4031214538049,-13.4784883891823,
38.7620122130522));
#21860=CARTESIAN_POINT('Ctrl Pts',(-29.3912288722191,-13.4653332811037,
38.725946824586));
#21861=CARTESIAN_POINT('Ctrl Pts',(-29.3797149312961,-13.4489478321199,
38.6910297000638));
#21862=CARTESIAN_POINT('Ctrl Pts',(-29.3687598143315,-13.4295031815302,
38.6578072625039));
#21863=CARTESIAN_POINT('Ctrl Pts',(-29.3581606182668,-13.4106902683796,
38.6256641890356));
#21864=CARTESIAN_POINT('Ctrl Pts',(-29.3480841029937,-13.3890130654984,
38.5951061949253));
#21865=CARTESIAN_POINT('Ctrl Pts',(-29.3387004840658,-13.3645846069573,
38.5666494750863));
#21866=CARTESIAN_POINT('Ctrl Pts',(-29.3356538371499,-13.3566532439675,
38.5574102275847));
#21867=CARTESIAN_POINT('Ctrl Pts',(-29.332680314776,-13.3484315569536,38.5483927372337));
#21868=CARTESIAN_POINT('Ctrl Pts',(-29.3297860205605,-13.3399225829038,
38.5396155138337));
#21869=CARTESIAN_POINT('Ctrl Pts',(-29.3297548126056,-13.3398308342221,
38.5395208727323));
#21870=CARTESIAN_POINT('Ctrl Pts',(-29.329723613958,-13.3397390509054,38.5394262598562));
#21871=CARTESIAN_POINT('Ctrl Pts',(-29.3296924246223,-13.3396472329757,
38.5393316752196));
#21872=CARTESIAN_POINT('Ctrl Pts',(-29.3182021246964,-13.3058210699871,
38.5044862442188));
#21873=CARTESIAN_POINT('Ctrl Pts',(-29.3080231408104,-13.2674403223344,
38.4736175042842));
#21874=CARTESIAN_POINT('Ctrl Pts',(-29.2993846393367,-13.2257618864395,
38.4474204242529));
#21875=CARTESIAN_POINT('Ctrl Pts',(-29.294837188495,-13.2038216646352,38.433629845644));
#21876=CARTESIAN_POINT('Ctrl Pts',(-29.2907167715431,-13.1809667714828,
38.4211342880547));
#21877=CARTESIAN_POINT('Ctrl Pts',(-29.2870580654097,-13.1573764603981,
38.4100389125803));
#21878=CARTESIAN_POINT('Ctrl Pts',(-29.2811580163661,-13.1193345988007,
38.392146450855));
#21879=CARTESIAN_POINT('Ctrl Pts',(-29.2764567980797,-13.0793753611201,
38.377889557797));
#21880=CARTESIAN_POINT('Ctrl Pts',(-29.2731071107402,-13.0382175959962,
38.3677313113026));
#21881=CARTESIAN_POINT('Ctrl Pts',(-29.2698236342539,-12.9978733667247,
38.3577738555386));
#21882=CARTESIAN_POINT('Ctrl Pts',(-29.2678389416643,-12.9563778844883,
38.3517550858753));
#21883=CARTESIAN_POINT('Ctrl Pts',(-29.2673123516664,-12.9144212114036,
38.3501581514577));
#21884=CARTESIAN_POINT('Ctrl Pts',(-29.2672183185014,-12.906929009168,38.3498729869122));
#21885=CARTESIAN_POINT('Ctrl Pts',(-29.2671708205346,-12.899422137448,38.3497289447954));
#21886=CARTESIAN_POINT('Ctrl Pts',(-29.2671708193829,-12.8919045823054,
38.3497289413026));
#21887=CARTESIAN_POINT('',(-31.6880237676519,-13.5169045823054,45.6911965120565));
#21888=CARTESIAN_POINT('',(-15.0075716891166,-13.5169045823054,-4.8938661154125));
#21889=CARTESIAN_POINT('',(-31.9936964198019,-14.4544045724565,46.6181779979126));
#21890=CARTESIAN_POINT('Origin',(385.745342703142,-1402.30168122098,-1220.21532002388));
#21891=CARTESIAN_POINT('',(-15.0075716891166,-14.4544045823054,-4.8938661154125));
#21892=CARTESIAN_POINT('Origin',(-20.691141817304,-11.0169045823054,-6.76802647489269));
#21893=CARTESIAN_POINT('',(-34.064851465877,-12.8919045823054,33.7890241943272));
#21894=CARTESIAN_POINT('',(-34.064851465877,-11.3294045823054,33.7890241943272));
#21895=CARTESIAN_POINT('',(-34.064851465877,-11.0169045823054,33.7890241943272));
#21896=CARTESIAN_POINT('',(-20.691141817304,-11.3294045823054,-6.76802647489269));
#21897=CARTESIAN_POINT('',(-36.9407072266747,-14.4544045474394,42.5103312117922));
#21898=CARTESIAN_POINT('',(-37.2382104124512,-14.4544045823054,43.4125380113454));
#21899=CARTESIAN_POINT('',(-36.6209071624921,-13.5169045823054,41.5405070008967));
#21900=CARTESIAN_POINT('Origin',(151.814591741463,-669.972712918203,-529.908124501381));
#21901=CARTESIAN_POINT('',(-34.2850388610326,-13.5169045823054,34.4567634810854));
#21902=CARTESIAN_POINT('',(-34.2250213624229,-13.5169045823054,34.2747546894998));
#21903=CARTESIAN_POINT('Ctrl Pts',(-34.064851465877,-12.8919045823054,33.7890241943272));
#21904=CARTESIAN_POINT('Ctrl Pts',(-34.064851465877,-12.9240089539691,33.7890241943272));
#21905=CARTESIAN_POINT('Ctrl Pts',(-34.0657129309706,-12.9558011837999,
33.7916366694271));
#21906=CARTESIAN_POINT('Ctrl Pts',(-34.06740655103,-12.9870390822551,33.7967727338678));
#21907=CARTESIAN_POINT('Ctrl Pts',(-34.0691409907585,-13.0190298772458,
33.8020325878498));
#21908=CARTESIAN_POINT('Ctrl Pts',(-34.0717481240388,-13.0504387214823,
33.8099389683029));
#21909=CARTESIAN_POINT('Ctrl Pts',(-34.0751794302049,-13.0810143824546,
33.8203447316771));
#21910=CARTESIAN_POINT('Ctrl Pts',(-34.0775820070192,-13.1024232485175,
33.8276307751273));
#21911=CARTESIAN_POINT('Ctrl Pts',(-34.0803882878835,-13.1234238076895,
33.8361410896319));
#21912=CARTESIAN_POINT('Ctrl Pts',(-34.0835771201002,-13.1439346499851,
33.8458115276165));
#21913=CARTESIAN_POINT('Ctrl Pts',(-34.0835914891961,-13.1440270732421,
33.8458551032709));
#21914=CARTESIAN_POINT('Ctrl Pts',(-34.0836058650754,-13.1441194808469,
33.8458986994968));
#21915=CARTESIAN_POINT('Ctrl Pts',(-34.0836202477357,-13.144211872797,33.8459423162866));
#21916=CARTESIAN_POINT('Ctrl Pts',(-34.0950356695748,-13.2175427490952,
33.8805606723052));
#21917=CARTESIAN_POINT('Ctrl Pts',(-34.1107939452279,-13.2814833076597,
33.9283491469307));
#21918=CARTESIAN_POINT('Ctrl Pts',(-34.1300304689843,-13.3355724235347,
33.9866857408265));
#21919=CARTESIAN_POINT('Ctrl Pts',(-34.1313633525036,-13.3393202156014,
33.9907278372865));
#21920=CARTESIAN_POINT('Ctrl Pts',(-34.1327129398286,-13.3430206975228,
33.994820589631));
#21921=CARTESIAN_POINT('Ctrl Pts',(-34.1340789453017,-13.3466737099126,
33.9989631315761));
#21922=CARTESIAN_POINT('Ctrl Pts',(-34.134095506055,-13.3467179971709,33.999013353641));
#21923=CARTESIAN_POINT('Ctrl Pts',(-34.1341120683961,-13.346762275463,33.9990635805207));
#21924=CARTESIAN_POINT('Ctrl Pts',(-34.1341286323248,-13.3468065447897,
33.999113812215));
#21925=CARTESIAN_POINT('Ctrl Pts',(-34.1552239429207,-13.4031865990188,
34.0630873545708));
#21926=CARTESIAN_POINT('Ctrl Pts',(-34.1788849327196,-13.4450083105498,
34.1348415639403));
#21927=CARTESIAN_POINT('Ctrl Pts',(-34.2048318401454,-13.4738659092281,
34.2135280366445));
#21928=CARTESIAN_POINT('Ctrl Pts',(-34.230793136384,-13.502739510838,34.2922581447966));
#21929=CARTESIAN_POINT('Ctrl Pts',(-34.2575516483048,-13.5169045582356,
34.3734058855754));
#21930=CARTESIAN_POINT('Ctrl Pts',(-34.2850388610326,-13.5169045823054,
34.4567634810853));
#21931=CARTESIAN_POINT('Origin',(0.0835265683620477,-6.01690458230549,0.0824317919394229));
#21932=CARTESIAN_POINT('',(-48.2616071253848,-6.10843422628149,4.30318193353179));
#21933=CARTESIAN_POINT('',(-36.2923483131121,-6.10843371299756,32.2050468002929));
#21934=CARTESIAN_POINT('Origin',(0.0835265683620477,-6.10843371318468,0.0824317919394229));
#21935=CARTESIAN_POINT('',(-38.6155265946984,-12.6709337131846,39.2928878752488));
#21936=CARTESIAN_POINT('Ctrl Pts',(-36.2923483136832,-6.10843371318764,
32.2050467999334));
#21937=CARTESIAN_POINT('Ctrl Pts',(-36.4506972320925,-6.54712953976467,
32.6884882040633));
#21938=CARTESIAN_POINT('Ctrl Pts',(-36.6086641467873,-6.98698298246954,
33.1710153730752));
#21939=CARTESIAN_POINT('Ctrl Pts',(-36.7663605413492,-7.42790908708504,
33.6526450972576));
#21940=CARTESIAN_POINT('Ctrl Pts',(-36.9234404292421,-7.8671114117444,34.1323919125894));
#21941=CARTESIAN_POINT('Ctrl Pts',(-37.0802519669093,-8.30737802766575,
34.6112483736256));
#21942=CARTESIAN_POINT('Ctrl Pts',(-37.2368606662004,-8.74862497311526,
35.0892570131099));
#21943=CARTESIAN_POINT('Ctrl Pts',(-37.3931641879297,-9.18901207701331,
35.5663341748934));
#21944=CARTESIAN_POINT('Ctrl Pts',(-37.5492657202599,-9.63037569349855,
36.0425668828417));
#21945=CARTESIAN_POINT('Ctrl Pts',(-37.7051849081074,-10.0726323507207,
36.5180221740763));
#21946=CARTESIAN_POINT('Ctrl Pts',(-37.8606630015596,-10.5136378666595,
36.9921324053022));
#21947=CARTESIAN_POINT('Ctrl Pts',(-38.0159598214199,-10.9555313776692,
37.4654696724325));
#21948=CARTESIAN_POINT('Ctrl Pts',(-38.1710488404017,-11.3982301183212,
37.9381241297016));
#21949=CARTESIAN_POINT('Ctrl Pts',(-38.3194196408354,-11.8217518281929,
38.3903039204693));
#21950=CARTESIAN_POINT('Ctrl Pts',(-38.467599997085,-12.2460105160847,38.8418589612118));
#21951=CARTESIAN_POINT('Ctrl Pts',(-38.6155265946984,-12.6709337131846,
39.2928878752488));
#21952=CARTESIAN_POINT('',(-38.3314437206795,-13.2959337131846,40.4386168951447));
#21953=CARTESIAN_POINT('Ctrl Pts',(-38.3314437206796,-13.2959337131846,
40.4386168951445));
#21954=CARTESIAN_POINT('Ctrl Pts',(-38.366137334587,-13.2959336603242,40.4055920418474));
#21955=CARTESIAN_POINT('Ctrl Pts',(-38.3973537346038,-13.2916605128646,
40.369889537283));
#21956=CARTESIAN_POINT('Ctrl Pts',(-38.425468787648,-13.2840750781447,40.3324920189021));
#21957=CARTESIAN_POINT('Ctrl Pts',(-38.4579493281595,-13.2753118359295,
40.2892877038012));
#21958=CARTESIAN_POINT('Ctrl Pts',(-38.4862909067256,-13.2621273075482,
40.2438201501008));
#21959=CARTESIAN_POINT('Ctrl Pts',(-38.511035368168,-13.2459526169172,40.1975698652882));
#21960=CARTESIAN_POINT('Ctrl Pts',(-38.5182724521339,-13.2412219585235,
40.1840429111689));
#21961=CARTESIAN_POINT('Ctrl Pts',(-38.5252016095202,-13.236235270514,40.1704488680634));
#21962=CARTESIAN_POINT('Ctrl Pts',(-38.5318358717577,-13.2310278528739,
40.1568245667105));
#21963=CARTESIAN_POINT('Ctrl Pts',(-38.5318578376043,-13.2310106112677,
40.1567794570507));
#21964=CARTESIAN_POINT('Ctrl Pts',(-38.5318798002166,-13.2309933672421,
40.1567343470609));
#21965=CARTESIAN_POINT('Ctrl Pts',(-38.5319017595952,-13.2309761207983,
40.1566892367425));
#21966=CARTESIAN_POINT('Ctrl Pts',(-38.5756476076969,-13.1966190323616,
40.0668238005097));
#21967=CARTESIAN_POINT('Ctrl Pts',(-38.6064577978686,-13.1525556488358,
39.9756173439807));
#21968=CARTESIAN_POINT('Ctrl Pts',(-38.6271948516412,-13.1028429788279,
39.8861033242508));
#21969=CARTESIAN_POINT('Ctrl Pts',(-38.6296456164096,-13.0969677922401,
39.8755242994658));
#21970=CARTESIAN_POINT('Ctrl Pts',(-38.6319557285166,-13.091013740146,39.8649689297581));
#21971=CARTESIAN_POINT('Ctrl Pts',(-38.6341299442465,-13.0849875486837,
39.8544422340909));
#21972=CARTESIAN_POINT('Ctrl Pts',(-38.6341550963765,-13.0849178354768,
39.8543204573904));
#21973=CARTESIAN_POINT('Ctrl Pts',(-38.6341802298183,-13.0848481114876,
39.8541986834411));
#21974=CARTESIAN_POINT('Ctrl Pts',(-38.6342053445796,-13.0847783767298,
39.8540769122552));
#21975=CARTESIAN_POINT('Ctrl Pts',(-38.6393177094473,-13.0705831581647,
39.8292891499698));
#21976=CARTESIAN_POINT('Ctrl Pts',(-38.6436871904562,-13.0558793142743,
39.8044981508428));
#21977=CARTESIAN_POINT('Ctrl Pts',(-38.6473189003734,-13.0407301262923,
39.779789899109));
#21978=CARTESIAN_POINT('Ctrl Pts',(-38.6527932266981,-13.0178947125452,
39.7425454506291));
#21979=CARTESIAN_POINT('Ctrl Pts',(-38.6565923828782,-12.9940463246918,
39.7054863402387));
#21980=CARTESIAN_POINT('Ctrl Pts',(-38.658738720505,-12.9693962501975,39.6688952305503));
#21981=CARTESIAN_POINT('Ctrl Pts',(-38.6608850581318,-12.9447461757032,
39.6323041208619));
#21982=CARTESIAN_POINT('Ctrl Pts',(-38.6613785862668,-12.9192944015675,
39.5961810211914));
#21983=CARTESIAN_POINT('Ctrl Pts',(-38.6602417327113,-12.893252106151,39.5608086719037));
#21984=CARTESIAN_POINT('Ctrl Pts',(-38.6592756094922,-12.8711207892723,
39.530748469517));
#21985=CARTESIAN_POINT('Ctrl Pts',(-38.6571753247155,-12.8485482515866,
39.5011674516628));
#21986=CARTESIAN_POINT('Ctrl Pts',(-38.6538791596275,-12.8255048445994,
39.472089461548));
#21987=CARTESIAN_POINT('Ctrl Pts',(-38.6520037869991,-12.8123941618594,
39.4555453670344));
#21988=CARTESIAN_POINT('Ctrl Pts',(-38.6497405162343,-12.7991308725969,
39.4391646147524));
#21989=CARTESIAN_POINT('Ctrl Pts',(-38.6470721722362,-12.7857088195892,
39.4229563625242));
#21990=CARTESIAN_POINT('Ctrl Pts',(-38.6423111701721,-12.7617604748036,
39.394036732084));
#21991=CARTESIAN_POINT('Ctrl Pts',(-38.6362631824905,-12.7373067239694,
39.3656637812769));
#21992=CARTESIAN_POINT('Ctrl Pts',(-38.6288629041527,-12.7123167139536,
39.337863672571));
#21993=CARTESIAN_POINT('Ctrl Pts',(-38.6248258795218,-12.6986840799693,
39.3226980641349));
#21994=CARTESIAN_POINT('Ctrl Pts',(-38.6203857180183,-12.6848916910974,
39.3077033845067));
#21995=CARTESIAN_POINT('Ctrl Pts',(-38.6155265946984,-12.6709337131846,
39.2928878752488));
#21996=CARTESIAN_POINT('',(-37.0650186795419,-13.2959337131846,41.6073303993598));
#21997=CARTESIAN_POINT('Origin',(0.0835265683620477,-13.2959337131846,0.0824317919394229));
#21998=CARTESIAN_POINT('',(-37.5334874949993,-14.6753754514262,43.0348489817131));
#21999=CARTESIAN_POINT('Origin',(133.62398877783,-671.736422462057,-537.185659742862));
#22000=CARTESIAN_POINT('',(-48.2284489054473,-14.6753753060473,30.5110849318178));
#22001=CARTESIAN_POINT('Origin',(0.0835265683620477,-14.6753754514262,0.0824317919394229));
#22002=CARTESIAN_POINT('Ctrl Pts',(-48.2284492744908,-14.6753748699083,
30.5110851642587));
#22003=CARTESIAN_POINT('Ctrl Pts',(-48.2299633696893,-14.2165313283052,
29.6477376966094));
#22004=CARTESIAN_POINT('Ctrl Pts',(-48.2314726564589,-13.7688961376732,
28.7792612726429));
#22005=CARTESIAN_POINT('Ctrl Pts',(-48.2329717668262,-13.3339028926044,
27.9049951633218));
#22006=CARTESIAN_POINT('Ctrl Pts',(-48.2344282057187,-12.911291526629,27.0556146295442));
#22007=CARTESIAN_POINT('Ctrl Pts',(-48.2358750368302,-12.5006127516871,
26.2007692573981));
#22008=CARTESIAN_POINT('Ctrl Pts',(-48.2373071406924,-12.1031391972242,
25.3398789954832));
#22009=CARTESIAN_POINT('Ctrl Pts',(-48.2378382397359,-11.9557352063792,
25.0206158423475));
#22010=CARTESIAN_POINT('Ctrl Pts',(-48.2383673115233,-11.8101469172675,
24.7005215926836));
#22011=CARTESIAN_POINT('Ctrl Pts',(-48.2388940889699,-11.6664376689275,
24.3795676299112));
#22012=CARTESIAN_POINT('Ctrl Pts',(-48.2389469174388,-11.6520256252869,
24.3473804006859));
#22013=CARTESIAN_POINT('Ctrl Pts',(-48.2389997219701,-11.6376325718389,
24.315184473));
#22014=CARTESIAN_POINT('Ctrl Pts',(-48.2390525021121,-11.623258591744,24.2829798065931));
#22015=CARTESIAN_POINT('Ctrl Pts',(-48.2403190832725,-11.2783218088442,
23.5101546077717));
#22016=CARTESIAN_POINT('Ctrl Pts',(-48.2415701431461,-10.9443666874141,
22.732284950268));
#22017=CARTESIAN_POINT('Ctrl Pts',(-48.242796511321,-10.6225428069351,21.9488823033592));
#22018=CARTESIAN_POINT('Ctrl Pts',(-48.2432193628657,-10.511577985968,21.6787651997743));
#22019=CARTESIAN_POINT('Ctrl Pts',(-48.2436392818792,-10.4020550271772,
21.4079905277086));
#22020=CARTESIAN_POINT('Ctrl Pts',(-48.2440559020298,-10.2940198074422,
21.1365390135953));
#22021=CARTESIAN_POINT('Ctrl Pts',(-48.2440808777753,-10.2875432600572,
21.1202659074898));
#22022=CARTESIAN_POINT('Ctrl Pts',(-48.2441058419013,-10.2810720136179,
21.1039901109362));
#22023=CARTESIAN_POINT('Ctrl Pts',(-48.2441307942536,-10.274606093873,21.0877116651653));
#22024=CARTESIAN_POINT('Ctrl Pts',(-48.2448295961963,-10.0935250793195,
20.6318264095713));
#22025=CARTESIAN_POINT('Ctrl Pts',(-48.2455197694772,-9.91663263839809,
20.1739004285262));
#22026=CARTESIAN_POINT('Ctrl Pts',(-48.246199035224,-9.74425107310023,19.7141653273356));
#22027=CARTESIAN_POINT('Ctrl Pts',(-48.2468496559605,-9.5791389332757,19.2738175083628));
#22028=CARTESIAN_POINT('Ctrl Pts',(-48.2474902739655,-9.418164645248,18.831808477992));
#22029=CARTESIAN_POINT('Ctrl Pts',(-48.2481187813464,-9.26165511793492,
18.3883263777155));
#22030=CARTESIAN_POINT('Ctrl Pts',(-48.2483819011865,-9.19613359336515,
18.2026659656731));
#22031=CARTESIAN_POINT('Ctrl Pts',(-48.2486428968409,-9.13139516044456,
18.0167473119276));
#22032=CARTESIAN_POINT('Ctrl Pts',(-48.2489016051861,-9.06746659619111,
17.8305842623673));
#22033=CARTESIAN_POINT('Ctrl Pts',(-48.2489066096297,-9.06622996466504,
17.8269831319686));
#22034=CARTESIAN_POINT('Ctrl Pts',(-48.2489116131617,-9.06499364665102,
17.823381940484));
#22035=CARTESIAN_POINT('Ctrl Pts',(-48.2489166157804,-9.06375764243243,
17.8197806883051));
#22036=CARTESIAN_POINT('Ctrl Pts',(-48.2501226826645,-8.76577296160725,
16.9515652202961));
#22037=CARTESIAN_POINT('Ctrl Pts',(-48.2512776225182,-8.48534970208909,
16.0781073163287));
#22038=CARTESIAN_POINT('Ctrl Pts',(-48.252369512175,-8.22405492486658,15.1989747878282));
#22039=CARTESIAN_POINT('Ctrl Pts',(-48.2526503738063,-8.1568433005625,14.9728396700614));
#22040=CARTESIAN_POINT('Ctrl Pts',(-48.2529270615511,-8.09089757126633,
14.746329039514));
#22041=CARTESIAN_POINT('Ctrl Pts',(-48.2531993679279,-8.02624496071412,
14.5194354305203));
#22042=CARTESIAN_POINT('Ctrl Pts',(-48.2538215825573,-7.87851503755292,
14.0009880679757));
#22043=CARTESIAN_POINT('Ctrl Pts',(-48.2544211464411,-7.73745329659788,
13.4802335345385));
#22044=CARTESIAN_POINT('Ctrl Pts',(-48.2549947966408,-7.60353311381806,
12.957597846491));
#22045=CARTESIAN_POINT('Ctrl Pts',(-48.2555458288495,-7.47489316188283,
12.4555687393428));
#22046=CARTESIAN_POINT('Ctrl Pts',(-48.2560729487919,-7.35284273130093,
11.951803893176));
#22047=CARTESIAN_POINT('Ctrl Pts',(-48.2565734173535,-7.23775611983193,
11.4466902167293));
#22048=CARTESIAN_POINT('Ctrl Pts',(-48.2567519886166,-7.19669227855575,
11.2664615387687));
#22049=CARTESIAN_POINT('Ctrl Pts',(-48.2569271701239,-7.15651419471867,
11.0860593323825));
#22050=CARTESIAN_POINT('Ctrl Pts',(-48.2570988310731,-7.11724012340575,
10.9055143918711));
#22051=CARTESIAN_POINT('Ctrl Pts',(-48.2581343246436,-6.88033098059543,
9.81643078873517));
#22052=CARTESIAN_POINT('Ctrl Pts',(-48.2590418915315,-6.67627260268059,
8.72194948511542));
#22053=CARTESIAN_POINT('Ctrl Pts',(-48.2598002645257,-6.50737682473014,
7.62168683257795));
#22054=CARTESIAN_POINT('Ctrl Pts',(-48.2605586375199,-6.3384810467797,6.52142418004048));
#22055=CARTESIAN_POINT('Ctrl Pts',(-48.2611678149523,-6.20474805619726,
5.41538014167176));
#22056=CARTESIAN_POINT('Ctrl Pts',(-48.2616069309149,-6.10843510301187,
4.30318195855187));
#22057=CARTESIAN_POINT('Origin',(0.0835265683613308,-8.56135981233827,68.5199317919394));
#22058=CARTESIAN_POINT('',(-49.6039734316379,-8.56135981233827,22.7876789472102));
#22059=CARTESIAN_POINT('',(-49.603973431638,-8.56135981233827,44.4574317919389));
#22060=CARTESIAN_POINT('',(-49.603973431638,-8.56135981233827,68.5199317919394));
#22061=CARTESIAN_POINT('',(-44.2914734316384,-8.56135981233827,49.7699317919394));
#22062=CARTESIAN_POINT('Origin',(-44.2914734316384,-8.56135981233827,44.457431791939));
#22063=CARTESIAN_POINT('',(-22.6217205869088,-8.56135981233827,49.7699317919394));
#22064=CARTESIAN_POINT('',(0.0835265683613272,-8.56135981233827,49.7699317919394));
#22065=CARTESIAN_POINT('',(-37.6513250757669,-8.56135981233827,39.5850503890339));
#22066=CARTESIAN_POINT('Origin',(0.0835265683620477,-8.56135981233827,0.0824317919394229));
#22067=CARTESIAN_POINT('',(-38.8073463968985,-8.56135981233827,40.7410717101655));
#22068=CARTESIAN_POINT('',(-38.8073463968985,-8.56135981233827,40.7410717101655));
#22069=CARTESIAN_POINT('',(-40.5751133498648,-8.56135981233827,38.9733047571991));
#22070=CARTESIAN_POINT('Origin',(-39.6912298733817,-8.56135981233827,39.8571882336823));
#22071=CARTESIAN_POINT('',(-39.4190920287332,-8.56135981233827,37.8172834360675));
#22072=CARTESIAN_POINT('',(-39.3319744043414,-8.56135981233827,37.7301658116757));
#22073=CARTESIAN_POINT('Origin',(0.0835265683620477,-8.56135981233827,0.0824317919394229));
#22074=CARTESIAN_POINT('Origin',(0.0835265683615161,13.1261401876617,50.8324317919394));
#22075=CARTESIAN_POINT('',(-10.8649863601191,13.1261401876617,49.7699317919394));
#22076=CARTESIAN_POINT('',(-44.2914734316384,13.1261401876617,49.7699317919394));
#22077=CARTESIAN_POINT('',(0.0835265683615159,13.1261401876617,49.7699317919394));
#22078=CARTESIAN_POINT('',(-49.603973431638,13.1261401876617,44.4574317919389));
#22079=CARTESIAN_POINT('Origin',(-44.2914734316384,13.1261401876617,44.457431791939));
#22080=CARTESIAN_POINT('',(-49.603973431638,13.1261401876617,11.0309447204206));
#22081=CARTESIAN_POINT('',(-49.603973431638,13.1261401876617,50.8324317919394));
#22082=CARTESIAN_POINT('',(-36.7666959739419,13.1261401876617,35.1648873812763));
#22083=CARTESIAN_POINT('Origin',(0.0835265683620477,13.1261401876617,0.0824317919394229));
#22084=CARTESIAN_POINT('',(-40.5751133498648,13.1261401876617,38.9733047571991));
#22085=CARTESIAN_POINT('',(-34.9989290209756,13.1261401876617,36.9326543342427));
#22086=CARTESIAN_POINT('',(-34.9121356166459,13.1261401876617,36.845860929913));
#22087=CARTESIAN_POINT('Origin',(0.0835265683620477,13.1261401876617,0.0824317919394229));
#22088=CARTESIAN_POINT('Origin',(-44.2914734316384,16.4830954176946,44.457431791939));
#22089=CARTESIAN_POINT('Origin',(-44.2914734316384,-8.87385981233827,44.457431791939));
#22090=CARTESIAN_POINT('Origin',(-44.2914734316384,-14.4544045823054,44.457431791939));
#22091=CARTESIAN_POINT('Origin',(-44.2914734316384,16.4830954176946,44.457431791939));
#22092=CARTESIAN_POINT('Origin',(-44.2914734316384,13.4386401876617,44.457431791939));
#22093=CARTESIAN_POINT('Origin',(-44.2914734316384,16.1705954176946,44.457431791939));
#22094=CARTESIAN_POINT('Origin',(0.0835265683620477,16.4830954176946,0.0824317919394229));
#22095=CARTESIAN_POINT('',(-22.5100610938546,16.3915662868155,48.4076054027908));
#22096=CARTESIAN_POINT('',(-4.13722371782189,11.5746245485739,48.4275653154638));
#22097=CARTESIAN_POINT('Ctrl Pts',(-22.5100610938539,16.3915662868154,48.40760540279));
#22098=CARTESIAN_POINT('Ctrl Pts',(-19.5784539338831,15.1541680928392,48.4122678868286));
#22099=CARTESIAN_POINT('Ctrl Pts',(-16.5898434682929,14.0894359483377,48.4166153560574));
#22100=CARTESIAN_POINT('Ctrl Pts',(-11.9895027246046,12.8480220597895,48.4218969462028));
#22101=CARTESIAN_POINT('Ctrl Pts',(-10.4336967396725,12.4934998941785,48.4234490140686));
#22102=CARTESIAN_POINT('Ctrl Pts',(-7.30241537284812,11.9258476364963,48.4259690402679));
#22103=CARTESIAN_POINT('Ctrl Pts',(-5.72390896832624,11.7120008366799,48.4269393095598));
#22104=CARTESIAN_POINT('Ctrl Pts',(-4.13722371861483,11.5746245485739,48.4275653153946));
#22105=CARTESIAN_POINT('',(-48.261606955131,11.5746245485364,4.30318207805214));
#22106=CARTESIAN_POINT('Origin',(0.0835265683620477,11.5746245485738,0.0824317919394229));
#22107=CARTESIAN_POINT('',(-48.2416470424886,16.3915662868156,22.6760194541557));
#22108=CARTESIAN_POINT('Ctrl Pts',(-48.2616069550931,11.5746245485739,4.30318207891625));
#22109=CARTESIAN_POINT('Ctrl Pts',(-48.2609815027128,11.7118793817134,5.88846453338143));
#22110=CARTESIAN_POINT('Ctrl Pts',(-48.2600147804388,11.9249456441311,7.46165171918502));
#22111=CARTESIAN_POINT('Ctrl Pts',(-48.257503140552,12.4906656417943,10.5857557642485));
#22112=CARTESIAN_POINT('Ctrl Pts',(-48.2559560607416,12.843980457976,12.1389419888214));
#22113=CARTESIAN_POINT('Ctrl Pts',(-48.2506725111118,14.0856585112706,16.7448657488753));
#22114=CARTESIAN_POINT('Ctrl Pts',(-48.2463082137514,15.1545164964592,19.7452377217243));
#22115=CARTESIAN_POINT('Ctrl Pts',(-48.2416470424886,16.3915662868154,22.6760194541553));
#22116=CARTESIAN_POINT('Origin',(0.0835265683620477,16.3915662868154,0.0824317919394229));
#22117=CARTESIAN_POINT('Origin',(-41.0170550881064,16.4855954176946,39.8571882336823));
#22118=CARTESIAN_POINT('',(-35.9236748279974,-3.61941807409669,34.7638079735734));
#22119=CARTESIAN_POINT('',(-39.1981211596124,-8.24885981233827,38.0382543051883));
#22120=CARTESIAN_POINT('Ctrl Pts',(-35.9236748279974,-3.61941807409669,
34.7638079735734));
#22121=CARTESIAN_POINT('Ctrl Pts',(-36.4701860414282,-4.3920600802535,35.3103191870041));
#22122=CARTESIAN_POINT('Ctrl Pts',(-37.0166933027455,-5.16470767732066,
35.8568264483215));
#22123=CARTESIAN_POINT('Ctrl Pts',(-38.1081750882717,-6.70785538323106,
36.9483082338476));
#22124=CARTESIAN_POINT('Ctrl Pts',(-38.6531496305009,-7.47835546664591,
37.4932827760768));
#22125=CARTESIAN_POINT('Ctrl Pts',(-39.1981211596124,-8.24885981233827,
38.0382543051883));
#22126=CARTESIAN_POINT('',(-40.354142480744,-8.24885981233827,39.1942756263199));
#22127=CARTESIAN_POINT('',(-36.5457251048211,12.8136401876617,35.3858582503971));
#22128=CARTESIAN_POINT('',(-36.4589317004915,12.8136401876617,35.2990648460674));
#22129=CARTESIAN_POINT('',(-35.9236748279974,11.9341984494202,34.7638079735734));
#22130=CARTESIAN_POINT('',(-36.5457251048211,12.8136401876617,35.3858582503971));
#22131=CARTESIAN_POINT('',(-35.9236748279975,-3.74885981233827,34.7638079735734));
#22132=CARTESIAN_POINT('Origin',(-39.6912298733817,16.4855954176946,41.1830134484071));
#22133=CARTESIAN_POINT('',(-37.8722959448877,-8.24885981233827,39.3640795199131));
#22134=CARTESIAN_POINT('',(-37.7851783204959,-8.24885981233827,39.2769618955213));
#22135=CARTESIAN_POINT('',(-34.5978496132727,-3.61941807409669,36.0896331882982));
#22136=CARTESIAN_POINT('Ctrl Pts',(-37.8722959448877,-8.24885981233827,
39.3640795199131));
#22137=CARTESIAN_POINT('Ctrl Pts',(-37.3273244157762,-7.4783554666459,38.8191079908016));
#22138=CARTESIAN_POINT('Ctrl Pts',(-36.7823498735469,-6.70785538323104,
38.2741334485724));
#22139=CARTESIAN_POINT('Ctrl Pts',(-35.6908680880207,-5.16470767732064,
37.1826516630462));
#22140=CARTESIAN_POINT('Ctrl Pts',(-35.1443608267034,-4.39206008025349,
36.6361444017289));
#22141=CARTESIAN_POINT('Ctrl Pts',(-34.5978496132727,-3.61941807409669,
36.0896331882982));
#22142=CARTESIAN_POINT('',(-34.5978496132729,11.9341984494205,36.0896331882984));
#22143=CARTESIAN_POINT('',(-34.5978496132727,12.0636401876617,36.0896331882982));
#22144=CARTESIAN_POINT('',(-35.2198998900963,12.8136401876617,36.7116834651218));
#22145=CARTESIAN_POINT('',(-34.5978496132727,11.9341984494202,36.0896331882982));
#22146=CARTESIAN_POINT('',(-39.0283172660193,12.8136401876617,40.5201008410447));
#22147=CARTESIAN_POINT('Origin',(0.0835265683620477,-11.0169045823054,0.0824317919394229));
#22148=CARTESIAN_POINT('Origin',(0.0835265683620477,-14.4544045823054,0.0824317919394229));
#22149=CARTESIAN_POINT('Origin',(0.0835265683620477,-11.3294045823054,0.0824317919394229));
#22150=CARTESIAN_POINT('Origin',(0.0835265683620477,-13.2044045823054,0.0824317919394229));
#22151=CARTESIAN_POINT('',(-34.5818198379706,-13.2044045823054,34.3588997915592));
#22152=CARTESIAN_POINT('',(-36.9176881394301,-13.2044045823054,41.4426433113705));
#22153=CARTESIAN_POINT('',(-37.0041161457864,-13.2044045823054,41.7047444878682));
#22154=CARTESIAN_POINT('',(-38.1790905589799,-13.2044045823054,40.2785649063406));
#22155=CARTESIAN_POINT('Origin',(0.0835265683620477,-13.2044045823054,0.0824317919394229));
#22156=CARTESIAN_POINT('',(-35.8042963200226,-13.2044045823054,33.0767747666364));
#22157=CARTESIAN_POINT('',(-22.4718276789325,-13.2044045823054,-7.35520861204973));
#22158=CARTESIAN_POINT('Origin',(0.0835265683620477,-13.2044045823054,0.0824317919394229));
#22159=CARTESIAN_POINT('Origin',(-22.7686086558706,16.4855954176946,-7.4530723015759));
#22160=CARTESIAN_POINT('',(-38.1635245965525,-12.8919045823054,39.2334793180968));
#22161=CARTESIAN_POINT('',(-22.7686086558706,-12.8919045823054,-7.4530723015759));
#22162=CARTESIAN_POINT('Ctrl Pts',(-38.1635245965525,-12.8919045823054,
39.2334793180967));
#22163=CARTESIAN_POINT('Ctrl Pts',(-37.6189300816584,-11.3339023360117,
37.5819444848208));
#22164=CARTESIAN_POINT('Ctrl Pts',(-37.0718575407512,-9.78474033410477,
35.9228948011991));
#22165=CARTESIAN_POINT('Ctrl Pts',(-36.52139118477,-8.24794399907487,34.2535530495173));
#22166=CARTESIAN_POINT('Ctrl Pts',(-36.3815123036638,-7.85742903027376,
33.8293569948958));
#22167=CARTESIAN_POINT('Ctrl Pts',(-36.2414142252472,-7.46771271925601,
33.4044962035141));
#22168=CARTESIAN_POINT('Ctrl Pts',(-36.1010818023558,-7.07885337125988,
32.9789247401509));
#22169=CARTESIAN_POINT('Origin',(0.0835265683620477,-13.2044045823054,0.0824317919394229));
#22170=CARTESIAN_POINT('',(-27.8490907775129,-13.2044045823054,40.036547827824));
#22171=CARTESIAN_POINT('',(-30.0427195777899,-13.2044045823054,46.6889364873753));
#22172=CARTESIAN_POINT('',(-30.1097879334595,-13.2044045823054,46.8923276758091));
#22173=CARTESIAN_POINT('',(-31.3912427907138,-13.2044045823054,45.7890602015826));
#22174=CARTESIAN_POINT('Origin',(0.0835265683620477,-13.2044045823054,0.0824317919394229));
#22175=CARTESIAN_POINT('',(-29.1770996549271,-13.2044045823054,39.0744598620586));
#22176=CARTESIAN_POINT('',(-14.7107907121785,-13.2044045823054,-4.79600242588632));
#22177=CARTESIAN_POINT('Origin',(0.0835265683620477,-13.2044045823054,0.0824317919394229));
#22178=CARTESIAN_POINT('Origin',(-12.93010485055,16.4855954176946,-4.20882028872929));
#22179=CARTESIAN_POINT('',(-27.5523098005748,-12.8919045823054,40.1344115173502));
#22180=CARTESIAN_POINT('',(-27.5523098389671,-6.59535001059396,40.1344116337787));
#22181=CARTESIAN_POINT('',(-27.5523098005748,-6.01690458230549,40.1344115173502));
#22182=CARTESIAN_POINT('',(-29.5940549924842,-12.8919045823054,46.326198641332));
#22183=CARTESIAN_POINT('Ctrl Pts',(-27.5523099865879,-6.59534981976455,
40.1344120814527));
#22184=CARTESIAN_POINT('Ctrl Pts',(-28.2344318423759,-8.68909917314417,
42.2030116992655));
#22185=CARTESIAN_POINT('Ctrl Pts',(-28.914831114185,-10.7885698299828,44.266387416788));
#22186=CARTESIAN_POINT('Ctrl Pts',(-29.5940549924842,-12.8919045823054,
46.326198641332));
#22187=CARTESIAN_POINT('',(-27.4793257777183,-12.8919045823054,39.9130805036812));
#22188=CARTESIAN_POINT('Origin',(0.0835265683620477,15.5455954176946,0.0824317919394229));
#22189=CARTESIAN_POINT('',(-46.6203840461634,16.1705954176946,29.1297162314601));
#22190=CARTESIAN_POINT('Origin',(0.0835265683620477,16.1705954176946,0.0824317919394229));
#22191=CARTESIAN_POINT('',(-46.6203840461634,15.8580954176946,29.1297162314601));
#22192=CARTESIAN_POINT('',(-46.6203840461634,15.5455954176946,29.1297162314601));
#22193=CARTESIAN_POINT('Origin',(0.0835265683620477,15.8580954176946,0.0824317919394229));
#22194=CARTESIAN_POINT('Origin',(-42.6676757995426,15.5455954176946,48.519931791939));
#22195=CARTESIAN_POINT('',(-39.9953087176173,15.8580954176946,48.519931791939));
#22196=CARTESIAN_POINT('',(-39.9953087176173,16.1705954176946,48.519931791939));
#22197=CARTESIAN_POINT('',(-39.9953087176173,16.4830954176946,48.519931791939));
#22198=CARTESIAN_POINT('',(-29.4588820377423,16.1705954176946,48.5199317919391));
#22199=CARTESIAN_POINT('',(-42.6676757995426,15.8580954176946,48.519931791939));
#22200=CARTESIAN_POINT('Origin',(-48.3539734316382,15.5455954176946,26.1363872258074));
#22201=CARTESIAN_POINT('',(-48.3539734316382,15.8580954176946,29.6248403980428));
#22202=CARTESIAN_POINT('',(-48.3539734316382,16.1705954176946,29.6248403980428));
#22203=CARTESIAN_POINT('',(-48.3539734316382,16.4830954176946,29.6248403980428));
#22204=CARTESIAN_POINT('',(-48.3539734316384,16.1705954176946,40.1612670779178));
#22205=CARTESIAN_POINT('',(-48.3539734316384,15.5455954176946,40.1612670779178));
#22206=CARTESIAN_POINT('',(-48.3539734316382,15.8580954176946,26.1363872258074));
#22207=CARTESIAN_POINT('Origin',(0.0835265683620477,15.5455954176946,0.0824317919394229));
#22208=CARTESIAN_POINT('',(-40.5007398604433,15.5455954176946,47.2147847331155));
#22209=CARTESIAN_POINT('Origin',(-44.2914734316384,15.5455954176946,44.457431791939));
#22210=CARTESIAN_POINT('',(-39.9953087176173,15.5455954176946,48.207431791939));
#22211=CARTESIAN_POINT('Origin',(-39.9953087176173,15.5455954176946,47.582431791939));
#22212=CARTESIAN_POINT('',(-29.4588820377423,15.5455954176946,48.2074317919391));
#22213=CARTESIAN_POINT('',(0.0835265683615436,15.5455954176946,48.2074317919394));
#22214=CARTESIAN_POINT('',(-29.1287992600205,15.5455954176946,47.0517055349559));
#22215=CARTESIAN_POINT('Origin',(-29.4588820377423,15.5455954176946,47.5824317919391));
#22216=CARTESIAN_POINT('',(-46.885747174655,15.5455954176946,29.294757620321));
#22217=CARTESIAN_POINT('Origin',(0.0835265683620477,15.5455954176946,0.0824317919394229));
#22218=CARTESIAN_POINT('',(-48.0414734316383,15.5455954176946,29.6248403980429));
#22219=CARTESIAN_POINT('Origin',(-47.4164734316383,15.5455954176946,29.6248403980429));
#22220=CARTESIAN_POINT('',(-48.0414734316379,15.5455954176946,0.0824317919388688));
#22221=CARTESIAN_POINT('Origin',(-47.4164734316383,15.5455954176946,29.6248403980429));
#22222=CARTESIAN_POINT('Origin',(-47.4164734316383,15.8580954176946,29.6248403980429));
#22223=CARTESIAN_POINT('Origin',(-47.4164734316383,16.1705954176946,29.6248403980429));
#22224=CARTESIAN_POINT('Origin',(-39.9953087176173,15.5455954176946,47.582431791939));
#22225=CARTESIAN_POINT('Origin',(-39.9953087176173,15.8580954176946,47.582431791939));
#22226=CARTESIAN_POINT('Origin',(-39.9953087176173,16.1705954176946,47.582431791939));
#22227=CARTESIAN_POINT('Origin',(-47.4164734316384,15.5455954176946,40.1612670779178));
#22228=CARTESIAN_POINT('Origin',(-44.2914734316384,16.1705954176946,44.457431791939));
#22229=CARTESIAN_POINT('Origin',(-41.0061710032694,16.1705954176946,46.8471376742919));
#22230=CARTESIAN_POINT('Origin',(-39.9953087176173,16.1705954176946,47.582431791939));
#22231=CARTESIAN_POINT('Origin',(-39.9953087176173,16.1705954176946,48.832431791939));
#22232=CARTESIAN_POINT('Origin',(-42.6676757995426,16.1705954176946,48.832431791939));
#22233=CARTESIAN_POINT('Origin',(-29.4588820377424,16.1705954176946,48.8324317919391));
#22234=CARTESIAN_POINT('Origin',(-48.6664734316382,16.1705954176946,26.1363872258074));
#22235=CARTESIAN_POINT('Origin',(-48.6664734316382,16.1705954176946,29.6248403980428));
#22236=CARTESIAN_POINT('Origin',(-29.4588820377423,16.1705954176946,47.5824317919391));
#22237=CARTESIAN_POINT('Origin',(-28.7987164822987,16.1705954176946,46.5209792779726));
#22238=CARTESIAN_POINT('Origin',(-47.4164734316383,16.1705954176946,29.6248403980429));
#22239=CARTESIAN_POINT('Origin',(-46.3550209176718,16.1705954176946,28.9646748425992));
#22240=CARTESIAN_POINT('Origin',(0.0835265683620477,16.1705954176946,0.0824317919394229));
#22241=CARTESIAN_POINT('Origin',(-44.2914734316384,15.8580954176946,44.457431791939));
#22242=CARTESIAN_POINT('Origin',(-40.5007398604433,15.8580954176946,47.2147847331155));
#22243=CARTESIAN_POINT('Origin',(-39.9953087176173,15.8580954176946,47.582431791939));
#22244=CARTESIAN_POINT('Origin',(-39.9953087176173,15.8580954176946,48.207431791939));
#22245=CARTESIAN_POINT('Origin',(0.0835265683615436,15.8580954176946,48.2074317919394));
#22246=CARTESIAN_POINT('Origin',(-29.4588820377423,15.8580954176946,48.2074317919391));
#22247=CARTESIAN_POINT('Origin',(-48.0414734316379,15.8580954176946,0.0824317919388688));
#22248=CARTESIAN_POINT('Origin',(-48.0414734316382,15.8580954176946,29.6248403980429));
#22249=CARTESIAN_POINT('Origin',(-29.4588820377423,15.8580954176946,47.5824317919391));
#22250=CARTESIAN_POINT('Origin',(-29.1287992600205,15.8580954176946,47.0517055349559));
#22251=CARTESIAN_POINT('Origin',(-47.4164734316383,15.8580954176946,29.6248403980429));
#22252=CARTESIAN_POINT('Origin',(-46.885747174655,15.8580954176946,29.294757620321));
#22253=CARTESIAN_POINT('Origin',(0.0835265683620477,15.8580954176946,0.0824317919394229));
#22254=CARTESIAN_POINT('Ctrl Pts',(0.0835265683815503,-6.00666333723547,
48.5199460669664));
#22255=CARTESIAN_POINT('Ctrl Pts',(0.434571873255604,-6.0013252951217,48.519945950593));
#22256=CARTESIAN_POINT('Ctrl Pts',(0.78566911589282,-5.99973567328053,48.5184885224505));
#22257=CARTESIAN_POINT('Ctrl Pts',(1.48799467904377,-5.99820579736959,48.508757702106));
#22258=CARTESIAN_POINT('Ctrl Pts',(1.83922299955751,-5.99826554329982,48.5004843099039));
#22259=CARTESIAN_POINT('Ctrl Pts',(2.54183792081169,-5.99418693015785,48.4732202209189));
#22260=CARTESIAN_POINT('Ctrl Pts',(2.89280484433907,-5.99381953117288,48.4556040546384));
#22261=CARTESIAN_POINT('Ctrl Pts',(3.59436240935176,-5.99717808806743,48.4131737559656));
#22262=CARTESIAN_POINT('Ctrl Pts',(3.94495305083707,-6.00090404394696,48.3883596235733));
#22263=CARTESIAN_POINT('Ctrl Pts',(4.29550794738001,-6.007051447105,48.3603316468569));
#22264=CARTESIAN_POINT('Ctrl Pts',(0.0835265683810243,-5.9853111687807,
48.5199456014727));
#22265=CARTESIAN_POINT('Ctrl Pts',(0.356716052653991,-5.98270666392053,
48.5198859104315));
#22266=CARTESIAN_POINT('Ctrl Pts',(0.652301278133249,-5.98152768121034,
48.5186918880741));
#22267=CARTESIAN_POINT('Ctrl Pts',(1.29495516994804,-5.97907559060103,48.5103258778986));
#22268=CARTESIAN_POINT('Ctrl Pts',(1.64203235073192,-5.97774718230165,48.5030276183598));
#22269=CARTESIAN_POINT('Ctrl Pts',(2.39436889948374,-5.97194742955331,48.4746917382514));
#22270=CARTESIAN_POINT('Ctrl Pts',(2.76993041040138,-5.97081802552572,48.455949685341));
#22271=CARTESIAN_POINT('Ctrl Pts',(3.5267082710891,-5.97321241327176,48.409676657807));
#22272=CARTESIAN_POINT('Ctrl Pts',(3.90792462085919,-5.97673620504541,48.3821456831835));
#22273=CARTESIAN_POINT('Ctrl Pts',(4.29540257294,-5.98314272027373,48.3503998997031));
#22274=CARTESIAN_POINT('Ctrl Pts',(0.0835265683704475,-5.96223275463529,
48.5195872927805));
#22275=CARTESIAN_POINT('Ctrl Pts',(0.339530012943145,-5.96240686080331,
48.5196215918919));
#22276=CARTESIAN_POINT('Ctrl Pts',(0.626534465003536,-5.96239709811646,
48.5182575867091));
#22277=CARTESIAN_POINT('Ctrl Pts',(1.26276365256779,-5.96099214798698,48.509167391216));
#22278=CARTESIAN_POINT('Ctrl Pts',(1.61199486653157,-5.95954166014411,48.5013148775363));
#22279=CARTESIAN_POINT('Ctrl Pts',(2.3728618208734,-5.95413393118491,48.4721918658653));
#22280=CARTESIAN_POINT('Ctrl Pts',(2.75490258993289,-5.95257589046813,48.4528734062177));
#22281=CARTESIAN_POINT('Ctrl Pts',(3.52251156374742,-5.95314193699468,48.4051808771888));
#22282=CARTESIAN_POINT('Ctrl Pts',(3.90807774412224,-5.95526602423799,48.3768070663115));
#22283=CARTESIAN_POINT('Ctrl Pts',(4.29560464263447,-5.95992641567859,48.3444127441005));
#22284=CARTESIAN_POINT('Ctrl Pts',(0.0835265683683665,-5.92795641804995,
48.5154826407816));
#22285=CARTESIAN_POINT('Ctrl Pts',(0.36133241049536,-5.92787973562297,48.5154600083354));
#22286=CARTESIAN_POINT('Ctrl Pts',(0.667559641547024,-5.92723732580272,
48.5133469044261));
#22287=CARTESIAN_POINT('Ctrl Pts',(1.32724155701544,-5.92511301754089,48.5020950495901));
#22288=CARTESIAN_POINT('Ctrl Pts',(1.68069642931525,-5.92360346889918,48.4928930594121));
#22289=CARTESIAN_POINT('Ctrl Pts',(2.42513999617731,-5.91998502842382,48.4637155122407));
#22290=CARTESIAN_POINT('Ctrl Pts',(2.80138061701086,-5.91860436677903,48.4445443128851));
#22291=CARTESIAN_POINT('Ctrl Pts',(3.55227792514613,-5.91737158402242,48.3973032871643));
#22292=CARTESIAN_POINT('Ctrl Pts',(3.92693056632441,-5.91751946291059,48.369233977527));
#22293=CARTESIAN_POINT('Ctrl Pts',(4.29606146924342,-5.91876732373882,48.3374043064722));
#22294=CARTESIAN_POINT('Ctrl Pts',(0.0835265683679874,-5.90583775506839,
48.5199317919394));
#22295=CARTESIAN_POINT('Ctrl Pts',(0.400320847750857,-5.9058377550684,48.5199317919394));
#22296=CARTESIAN_POINT('Ctrl Pts',(0.734351631213873,-5.90562906540037,
48.5168141308035));
#22297=CARTESIAN_POINT('Ctrl Pts',(1.42391097883914,-5.90495067814671,48.5026532295386));
#22298=CARTESIAN_POINT('Ctrl Pts',(1.77943547629603,-5.90448098056109,48.4916098859256));
#22299=CARTESIAN_POINT('Ctrl Pts',(2.49892525008987,-5.90343694889075,48.4610292841221));
#22300=CARTESIAN_POINT('Ctrl Pts',(2.86288646455625,-5.90286261480602,48.4414922321787));
#22301=CARTESIAN_POINT('Ctrl Pts',(3.58624099388631,-5.90176568155595,48.3944770847012));
#22302=CARTESIAN_POINT('Ctrl Pts',(3.94563026526353,-5.9012430823906,48.3669995056144));
#22303=CARTESIAN_POINT('Ctrl Pts',(4.2963162261579,-5.90082453639418,48.3363830244465));
#22304=CARTESIAN_POINT('Ctrl Pts',(0.0835265683620106,-5.88746284406389,
48.5199317919394));
#22305=CARTESIAN_POINT('Ctrl Pts',(0.43481398105989,-5.88746284406389,48.5199317919394));
#22306=CARTESIAN_POINT('Ctrl Pts',(0.786101399028904,-5.88746284406389,
48.5161104362146));
#22307=CARTESIAN_POINT('Ctrl Pts',(1.48859334813907,-5.88746284406389,48.50082319184));
#22308=CARTESIAN_POINT('Ctrl Pts',(1.8397978898232,-5.88746284406389,48.489357302818));
#22309=CARTESIAN_POINT('Ctrl Pts',(2.5420408938028,-5.88746284406389,48.4587755322629));
#22310=CARTESIAN_POINT('Ctrl Pts',(2.89307936664319,-5.88746284406389,48.439659649984));
#22311=CARTESIAN_POINT('Ctrl Pts',(3.59490640778672,-5.88746284406389,48.3937688119853));
#22312=CARTESIAN_POINT('Ctrl Pts',(3.9456949866378,-5.88746284406389,48.3669938551438));
#22313=CARTESIAN_POINT('Ctrl Pts',(4.2963162261579,-5.88746284406389,48.3363830244465));
#22314=CARTESIAN_POINT('',(0.0835265683815503,-6.00666333723547,48.5199460669664));
#22315=CARTESIAN_POINT('Ctrl Pts',(0.0835265683620321,-5.88746284406389,
48.5199317919394));
#22316=CARTESIAN_POINT('Ctrl Pts',(0.0835265683679874,-5.90583775506839,
48.5199317919394));
#22317=CARTESIAN_POINT('Ctrl Pts',(0.0835265683683665,-5.92795641804995,
48.5154826407816));
#22318=CARTESIAN_POINT('Ctrl Pts',(0.0835265683704475,-5.96223275463529,
48.5195872927805));
#22319=CARTESIAN_POINT('Ctrl Pts',(0.0835265683810243,-5.9853111687807,
48.5199456014727));
#22320=CARTESIAN_POINT('Ctrl Pts',(0.0835265683815503,-6.00666333723547,
48.5199460669664));
#22321=CARTESIAN_POINT('',(4.29550794738001,-6.00705144710501,48.360331646857));
#22322=CARTESIAN_POINT('Ctrl Pts',(4.2963162261579,-5.88746284406389,48.3363830244465));
#22323=CARTESIAN_POINT('Ctrl Pts',(4.2963162261579,-5.89466520940775,48.3363830244465));
#22324=CARTESIAN_POINT('Ctrl Pts',(4.2962385509138,-5.90314351486558,48.3366383003061));
#22325=CARTESIAN_POINT('Ctrl Pts',(4.29613103097065,-5.9126635514535,48.3374208419226));
#22326=CARTESIAN_POINT('Ctrl Pts',(4.29603170548146,-5.92145803425842,48.338143743429));
#22327=CARTESIAN_POINT('Ctrl Pts',(4.29590711917709,-5.93114147445235,48.339318986334));
#22328=CARTESIAN_POINT('Ctrl Pts',(4.29579418047257,-5.94148964487015,48.3411521533193));
#22329=CARTESIAN_POINT('Ctrl Pts',(4.29568497044383,-5.95149617003368,48.3429247982243));
#22330=CARTESIAN_POINT('Ctrl Pts',(4.29558678798446,-5.96212379582482,48.3453142106815));
#22331=CARTESIAN_POINT('Ctrl Pts',(4.29552981876319,-5.97313476325662,48.3484700316399));
#22332=CARTESIAN_POINT('Ctrl Pts',(4.29547705488659,-5.98333292489416,48.3513928967225));
#22333=CARTESIAN_POINT('Ctrl Pts',(4.29545968136764,-5.99385899411772,48.354973634109));
#22334=CARTESIAN_POINT('Ctrl Pts',(4.29549777905033,-6.00450404015459,48.3592865236346));
#22335=CARTESIAN_POINT('Ctrl Pts',(4.29550081548163,-6.00535246317496,48.3596302661365));
#22336=CARTESIAN_POINT('Ctrl Pts',(4.29550420195006,-6.00620163512509,48.3599786327558));
#22337=CARTESIAN_POINT('Ctrl Pts',(4.29550794738001,-6.00705144710501,48.360331646857));
#22338=CARTESIAN_POINT('Ctrl Pts',(4.29550794738001,-6.00705144710501,48.360331646857));
#22339=CARTESIAN_POINT('Ctrl Pts',(3.59439815429413,-5.99475664078893,48.4163876002896));
#22340=CARTESIAN_POINT('Ctrl Pts',(2.89314538143878,-5.99214762358687,48.4595881764264));
#22341=CARTESIAN_POINT('Ctrl Pts',(1.48791553893041,-6.0003048498708,48.5141163543965));
#22342=CARTESIAN_POINT('Ctrl Pts',(0.785617178129657,-5.99598725300791,
48.5199458342196));
#22343=CARTESIAN_POINT('Ctrl Pts',(0.0835265683815503,-6.00666333723547,
48.5199460669664));
#22344=CARTESIAN_POINT('Ctrl Pts',(0.0835265683815503,-6.00666333723547,
48.5199460669664));
#22345=CARTESIAN_POINT('Ctrl Pts',(0.434571873255867,-6.01200137934908,
48.5199461833399));
#22346=CARTESIAN_POINT('Ctrl Pts',(0.785441202115477,-6.02125184123583,
48.5184889915199));
#22347=CARTESIAN_POINT('Ctrl Pts',(1.48685396085203,-6.04818290219913,48.5151613829932));
#22348=CARTESIAN_POINT('Ctrl Pts',(1.83739739072896,-6.06586350127568,48.5132909662866));
#22349=CARTESIAN_POINT('Ctrl Pts',(2.88857791145589,-6.13245845075531,48.5108119660871));
#22350=CARTESIAN_POINT('Ctrl Pts',(3.59085026662451,-6.17306838545285,48.5061181031007));
#22351=CARTESIAN_POINT('Ctrl Pts',(4.29256571553473,-6.20946968450873,48.4959174422579));
#22352=CARTESIAN_POINT('Ctrl Pts',(0.434571873255604,-6.0013252951217,48.519945950593));
#22353=CARTESIAN_POINT('Ctrl Pts',(0.707588293216581,-6.00879525432306,
48.5190043349161));
#22354=CARTESIAN_POINT('Ctrl Pts',(0.99833096149102,-6.01828947675665,48.5172889554697));
#22355=CARTESIAN_POINT('Ctrl Pts',(1.61221600115967,-6.04432658407314,48.5134046445675));
#22356=CARTESIAN_POINT('Ctrl Pts',(1.93535675298704,-6.06089216512314,48.5112385621328));
#22357=CARTESIAN_POINT('Ctrl Pts',(2.94880361840312,-6.12571278894254,48.5075991346784));
#22358=CARTESIAN_POINT('Ctrl Pts',(3.62682139079342,-6.16367997403223,48.5021196905958));
#22359=CARTESIAN_POINT('Ctrl Pts',(4.29322406284948,-6.19747947412217,48.4909193590357));
#22360=CARTESIAN_POINT('Ctrl Pts',(0.78566911589282,-5.99973567328053,48.5184885224505));
#22361=CARTESIAN_POINT('Ctrl Pts',(0.998676155525609,-6.00835114797884,
48.5169166777064));
#22362=CARTESIAN_POINT('Ctrl Pts',(1.24336152129271,-6.01789996842701,48.5149008816205));
#22363=CARTESIAN_POINT('Ctrl Pts',(1.78640027159867,-6.04289085428944,48.5103147763974));
#22364=CARTESIAN_POINT('Ctrl Pts',(2.08475122678728,-6.05836696395433,48.5077487407917));
#22365=CARTESIAN_POINT('Ctrl Pts',(3.04577953853793,-6.11975101512501,48.5025662257011));
#22366=CARTESIAN_POINT('Ctrl Pts',(3.68879008339862,-6.15479195325804,48.4962278198683));
#22367=CARTESIAN_POINT('Ctrl Pts',(4.29389279897283,-6.18527410484422,48.4847891628839));
#22368=CARTESIAN_POINT('Ctrl Pts',(1.48799467904377,-5.99820579736959,48.508757702106));
#22369=CARTESIAN_POINT('Ctrl Pts',(1.61377824566997,-6.00829173506077,48.5070409830128));
#22370=CARTESIAN_POINT('Ctrl Pts',(1.78770681959273,-6.01814206512117,48.505001360523));
#22371=CARTESIAN_POINT('Ctrl Pts',(2.21034411610889,-6.04173521008607,48.4999506928767));
#22372=CARTESIAN_POINT('Ctrl Pts',(2.45904980201447,-6.05552058030387,48.4969449896348));
#22373=CARTESIAN_POINT('Ctrl Pts',(3.28508024419413,-6.10935599904099,48.4895414181676));
#22374=CARTESIAN_POINT('Ctrl Pts',(3.8343859391826,-6.13882811018934,48.4820050858304));
#22375=CARTESIAN_POINT('Ctrl Pts',(4.29532856800228,-6.16205725113852,48.4713889284506));
#22376=CARTESIAN_POINT('Ctrl Pts',(1.83922299955751,-5.99826554329982,48.5004843099039));
#22377=CARTESIAN_POINT('Ctrl Pts',(1.93779750844287,-6.00864450579839,48.4992338112119));
#22378=CARTESIAN_POINT('Ctrl Pts',(2.0870291104974,-6.0187257861122,48.4974612117992));
#22379=CARTESIAN_POINT('Ctrl Pts',(2.46011313068803,-6.04195544062546,48.4926406006817));
#22380=CARTESIAN_POINT('Ctrl Pts',(2.68396271458218,-6.05514353311732,48.4895975747639));
#22381=CARTESIAN_POINT('Ctrl Pts',(3.42741006465308,-6.10489083408599,48.4815303852945));
#22382=CARTESIAN_POINT('Ctrl Pts',(3.91801310236138,-6.13175228789483,48.4736742225201));
#22383=CARTESIAN_POINT('Ctrl Pts',(4.29609560090838,-6.15104576671075,48.464118890169));
#22384=CARTESIAN_POINT('Ctrl Pts',(2.89314538143878,-5.99214762358687,48.4595881764264));
#22385=CARTESIAN_POINT('Ctrl Pts',(2.95442665208855,-6.00381665756757,48.4591554550777));
#22386=CARTESIAN_POINT('Ctrl Pts',(3.05143599671236,-6.01569196513297,48.4585450694277));
#22387=CARTESIAN_POINT('Ctrl Pts',(3.28969174328989,-6.04033961885394,48.4565445600394));
#22388=CARTESIAN_POINT('Ctrl Pts',(3.43093652567676,-6.0531346611766,48.455157285322));
#22389=CARTESIAN_POINT('Ctrl Pts',(3.88020206841996,-6.09364276617912,48.4510874243783));
#22390=CARTESIAN_POINT('Ctrl Pts',(4.15587729830959,-6.11446024451104,48.4470450295077));
#22391=CARTESIAN_POINT('Ctrl Pts',(4.2986604235491,-6.12223844465217,48.4422855877233));
#22392=CARTESIAN_POINT('Ctrl Pts',(3.59439815429413,-5.99475664078893,48.4163876002896));
#22393=CARTESIAN_POINT('Ctrl Pts',(3.631373897052,-6.00697011627484,48.4176356671024));
#22394=CARTESIAN_POINT('Ctrl Pts',(3.69355131163527,-6.02014444454774,48.4189800887165));
#22395=CARTESIAN_POINT('Ctrl Pts',(3.838713446485,-6.04594588203951,48.4216081073813));
#22396=CARTESIAN_POINT('Ctrl Pts',(3.92169816675145,-6.05857299125839,48.422891704432));
#22397=CARTESIAN_POINT('Ctrl Pts',(4.15746922912413,-6.0919301033921,48.4262709574895));
#22398=CARTESIAN_POINT('Ctrl Pts',(4.29707247280368,-6.10813589078398,48.4278950754018));
#22399=CARTESIAN_POINT('Ctrl Pts',(4.30071410004382,-6.10843369230011,48.4278763391901));
#22400=CARTESIAN_POINT('Ctrl Pts',(4.29550794738001,-6.007051447105,48.3603316468569));
#22401=CARTESIAN_POINT('Ctrl Pts',(4.29556063460001,-6.01900581052064,48.3652975204339));
#22402=CARTESIAN_POINT('Ctrl Pts',(4.29569371583991,-6.03128117156189,48.3719827330256));
#22403=CARTESIAN_POINT('Ctrl Pts',(4.29625434599585,-6.05467770199134,48.3864516772668));
#22404=CARTESIAN_POINT('Ctrl Pts',(4.29668189491191,-6.06579887137954,48.3942354089164));
#22405=CARTESIAN_POINT('Ctrl Pts',(4.29860676262888,-6.09473681170808,48.4157241439942));
#22406=CARTESIAN_POINT('Ctrl Pts',(4.3007463023986,-6.10812801481236,48.4275666875517));
#22407=CARTESIAN_POINT('Ctrl Pts',(4.30427685533891,-6.1084337131847,48.4275653153946));
#22408=CARTESIAN_POINT('Ctrl Pts',(4.29550794738001,-6.00705144710501,48.360331646857));
#22409=CARTESIAN_POINT('Ctrl Pts',(4.29571869526291,-6.05486867452994,48.3801950471849));
#22410=CARTESIAN_POINT('Ctrl Pts',(4.29721573529237,-6.10782181536582,48.4275676114412));
#22411=CARTESIAN_POINT('Ctrl Pts',(4.30427675511517,-6.10843370450313,48.4275653154304));
#22412=CARTESIAN_POINT('',(4.29256570756032,-6.20946977623549,48.4959172211618));
#22413=CARTESIAN_POINT('Ctrl Pts',(4.30427669622714,-6.10843371319295,48.4275653292943));
#22414=CARTESIAN_POINT('Ctrl Pts',(4.30071403889905,-6.10843410331512,48.4278767682018));
#22415=CARTESIAN_POINT('Ctrl Pts',(4.29866039809464,-6.12223873054906,48.4422858044068));
#22416=CARTESIAN_POINT('Ctrl Pts',(4.29524066002814,-6.16064820739695,48.4713966576509));
#22417=CARTESIAN_POINT('Ctrl Pts',(4.29388241016422,-6.18548926373562,48.4859212758134));
#22418=CARTESIAN_POINT('Ctrl Pts',(4.29256571553473,-6.20946968450872,48.4959174422579));
#22419=CARTESIAN_POINT('Ctrl Pts',(4.29256571553473,-6.20946968450872,48.4959174422579));
#22420=CARTESIAN_POINT('Ctrl Pts',(3.59085026662451,-6.17306838545285,48.5061181031007));
#22421=CARTESIAN_POINT('Ctrl Pts',(2.88857791145589,-6.13245845075531,48.5108119660871));
#22422=CARTESIAN_POINT('Ctrl Pts',(1.48700388381999,-6.04366518478247,48.5141172996865));
#22423=CARTESIAN_POINT('Ctrl Pts',(0.785617178130183,-6.01733942146269,
48.5199462997133));
#22424=CARTESIAN_POINT('Ctrl Pts',(0.0835265683815503,-6.00666333723547,
48.5199460669664));
#22425=CARTESIAN_POINT('Ctrl Pts',(0.0835265683815503,-6.00666333723547,
48.5199460669664));
#22426=CARTESIAN_POINT('Ctrl Pts',(0.083526568382076,-6.02801550569024,
48.5199465324602));
#22427=CARTESIAN_POINT('Ctrl Pts',(0.0835265683917245,-6.05386667280684,
48.5195892904706));
#22428=CARTESIAN_POINT('Ctrl Pts',(0.0835265683750737,-6.10694539169996,
48.521354690718));
#22429=CARTESIAN_POINT('Ctrl Pts',(0.0835265683690384,-6.12148849588211,
48.5199317919394));
#22430=CARTESIAN_POINT('Ctrl Pts',(0.0835265683620147,-6.14692278878554,
48.5199317919394));
#22431=CARTESIAN_POINT('Ctrl Pts',(0.434571873255867,-6.01200137934908,
48.5199461833399));
#22432=CARTESIAN_POINT('Ctrl Pts',(0.356369924026296,-6.03090918789886,
48.5198869612841));
#22433=CARTESIAN_POINT('Ctrl Pts',(0.356156584407958,-6.05382055712373,
48.519586959623));
#22434=CARTESIAN_POINT('Ctrl Pts',(0.394869806313788,-6.10695822375808,
48.5213559145512));
#22435=CARTESIAN_POINT('Ctrl Pts',(0.433796367857451,-6.12148849588211,
48.5199317919394));
#22436=CARTESIAN_POINT('Ctrl Pts',(0.433874220973527,-6.14692278878554,
48.5199317919394));
#22437=CARTESIAN_POINT('Ctrl Pts',(0.785441202115477,-6.02125184123583,
48.5184889915199));
#22438=CARTESIAN_POINT('Ctrl Pts',(0.651973538428245,-6.03698783585496,
48.5195752075049));
#22439=CARTESIAN_POINT('Ctrl Pts',(0.651610339577195,-6.05830967273444,
48.5196902430867));
#22440=CARTESIAN_POINT('Ctrl Pts',(0.717676140419002,-6.11145963930962,
48.5214911612938));
#22441=CARTESIAN_POINT('Ctrl Pts',(0.784105140129702,-6.12687873284897,
48.5199317919388));
#22442=CARTESIAN_POINT('Ctrl Pts',(0.784221873585039,-6.15072449281721,
48.5199317919388));
#22443=CARTESIAN_POINT('Ctrl Pts',(1.48685396085203,-6.04818290219913,48.5151613829932));
#22444=CARTESIAN_POINT('Ctrl Pts',(1.29453399477866,-6.05935112779906,48.5183112784905));
#22445=CARTESIAN_POINT('Ctrl Pts',(1.29397444382209,-6.07865710025977,48.5193460059679));
#22446=CARTESIAN_POINT('Ctrl Pts',(1.3890700537892,-6.12977840933564,48.5214366576208));
#22447=CARTESIAN_POINT('Ctrl Pts',(1.48472521472664,-6.14643370208422,48.5199317919371));
#22448=CARTESIAN_POINT('Ctrl Pts',(1.48483467245509,-6.16593130894387,48.5199317919372));
#22449=CARTESIAN_POINT('Ctrl Pts',(1.83739739072896,-6.06586350127568,48.5132909662866));
#22450=CARTESIAN_POINT('Ctrl Pts',(1.64148768190344,-6.07568031733619,48.5173741424648));
#22451=CARTESIAN_POINT('Ctrl Pts',(1.64088163807406,-6.09455995772352,48.518913524595));
#22452=CARTESIAN_POINT('Ctrl Pts',(1.73765605564234,-6.14361803658467,48.5212544268102));
#22453=CARTESIAN_POINT('Ctrl Pts',(1.83503651705134,-6.16059843435261,48.5199317919361));
#22454=CARTESIAN_POINT('Ctrl Pts',(1.83509981871363,-6.17733642103887,48.5199317919363));
#22455=CARTESIAN_POINT('Ctrl Pts',(2.88857791145589,-6.13245845075531,48.5108119660871));
#22456=CARTESIAN_POINT('Ctrl Pts',(2.76813631530143,-6.14582978514633,48.5172046544333));
#22457=CARTESIAN_POINT('Ctrl Pts',(2.7675104507475,-6.16286923349053,48.5194534620087));
#22458=CARTESIAN_POINT('Ctrl Pts',(2.82637284101024,-6.19966838879308,48.5212339924787));
#22459=CARTESIAN_POINT('Ctrl Pts',(2.88586109583122,-6.21324540616175,48.5199317919341));
#22460=CARTESIAN_POINT('Ctrl Pts',(2.88564773843035,-6.22295686941886,48.5199317919344));
#22461=CARTESIAN_POINT('Ctrl Pts',(3.59085026662451,-6.17306838545285,48.5061181031007));
#22462=CARTESIAN_POINT('Ctrl Pts',(3.5189080182867,-6.1918452082941,48.5141149281106));
#22463=CARTESIAN_POINT('Ctrl Pts',(3.51790722546928,-6.21237399283442,48.5175683503188));
#22464=CARTESIAN_POINT('Ctrl Pts',(3.55158573837203,-6.24739159904062,48.5204767822306));
#22465=CARTESIAN_POINT('Ctrl Pts',(3.58626504409221,-6.2618804207065,48.5199317919341));
#22466=CARTESIAN_POINT('Ctrl Pts',(3.58568299282961,-6.26857731779886,48.5199317919344));
#22467=CARTESIAN_POINT('Ctrl Pts',(4.29256571553473,-6.20946968450873,48.4959174422579));
#22468=CARTESIAN_POINT('Ctrl Pts',(4.29124902090524,-6.23345010528185,48.5059136087023));
#22469=CARTESIAN_POINT('Ctrl Pts',(4.28995382260361,-6.25674581560883,48.5119171961227));
#22470=CARTESIAN_POINT('Ctrl Pts',(4.28744009183432,-6.29803503999845,48.5189262877413));
#22471=CARTESIAN_POINT('Ctrl Pts',(4.28622155936666,-6.31602855406109,48.5199317919394));
#22472=CARTESIAN_POINT('Ctrl Pts',(4.2850581964051,-6.32940458230552,48.5199317919394));
#22473=CARTESIAN_POINT('Ctrl Pts',(4.2925656916115,-6.20946995968903,48.4959167789697));
#22474=CARTESIAN_POINT('Ctrl Pts',(4.29202349410917,-6.21934480701988,48.5000331414517));
#22475=CARTESIAN_POINT('Ctrl Pts',(4.2914804459715,-6.2291557048318,48.503523063216));
#22476=CARTESIAN_POINT('Ctrl Pts',(4.29094213463875,-6.23871408127371,48.5064309619194));
#22477=CARTESIAN_POINT('Ctrl Pts',(4.29037097470351,-6.24885572484954,48.5095163051661));
#22478=CARTESIAN_POINT('Ctrl Pts',(4.28980525582109,-6.25871184341276,48.5119471308067));
#22479=CARTESIAN_POINT('Ctrl Pts',(4.28924924924487,-6.26808527594654,48.5138297415884));
#22480=CARTESIAN_POINT('Ctrl Pts',(4.28866783601525,-6.27788702634898,48.5157983780426));
#22481=CARTESIAN_POINT('Ctrl Pts',(4.2880971014353,-6.28716030960548,48.5171691011132));
#22482=CARTESIAN_POINT('Ctrl Pts',(4.28753800272483,-6.2957252017121,48.5181018578833));
#22483=CARTESIAN_POINT('Ctrl Pts',(4.28693020589066,-6.30503610551124,48.5191158588125));
#22484=CARTESIAN_POINT('Ctrl Pts',(4.28633616809252,-6.31350977078174,48.5196144990409));
#22485=CARTESIAN_POINT('Ctrl Pts',(4.28575192091124,-6.32097498479555,48.5198172708104));
#22486=CARTESIAN_POINT('Ctrl Pts',(4.28551932677286,-6.323946954669,48.5198979961036));
#22487=CARTESIAN_POINT('Ctrl Pts',(4.28528823042114,-6.32675971428291,48.5199317800711));
#22488=CARTESIAN_POINT('Ctrl Pts',(4.2850581964051,-6.32940458230551,48.5199317919363));
#22489=CARTESIAN_POINT('Ctrl Pts',(0.0835265683620147,-6.14692278878557,
48.5199317919394));
#22490=CARTESIAN_POINT('Ctrl Pts',(0.0835265683690384,-6.12148849588211,
48.5199317919394));
#22491=CARTESIAN_POINT('Ctrl Pts',(0.0835265683750737,-6.10694539169996,
48.521354690718));
#22492=CARTESIAN_POINT('Ctrl Pts',(0.0835265683917245,-6.05386667280684,
48.5195892904706));
#22493=CARTESIAN_POINT('Ctrl Pts',(0.083526568382076,-6.02801550569024,
48.5199465324602));
#22494=CARTESIAN_POINT('Ctrl Pts',(0.0835265683815503,-6.00666333723547,
48.5199460669664));
#22495=CARTESIAN_POINT('Ctrl Pts',(0.0835265683815503,-6.00666333723547,
48.5199460669664));
#22496=CARTESIAN_POINT('Ctrl Pts',(-0.267518736492503,-6.01200137934925,
48.5199461833398));
#22497=CARTESIAN_POINT('Ctrl Pts',(-0.618388065344823,-6.02125184123478,
48.5184889915195));
#22498=CARTESIAN_POINT('Ctrl Pts',(-1.31980082405271,-6.04818290219398,
48.5151613829919));
#22499=CARTESIAN_POINT('Ctrl Pts',(-1.67034425390828,-6.06586350126765,
48.5132909662846));
#22500=CARTESIAN_POINT('Ctrl Pts',(-2.72152477454993,-6.13245845073777,
48.5108119660831));
#22501=CARTESIAN_POINT('Ctrl Pts',(-3.42379712957049,-6.17306838542386,
48.5061181030979));
#22502=CARTESIAN_POINT('Ctrl Pts',(-4.12551257835428,-6.20946968446904,
48.4959174422579));
#22503=CARTESIAN_POINT('Ctrl Pts',(0.083526568382076,-6.02801550569024,
48.5199465324602));
#22504=CARTESIAN_POINT('Ctrl Pts',(-0.189316787260607,-6.03090918789797,
48.5198869612836));
#22505=CARTESIAN_POINT('Ctrl Pts',(-0.484920401653545,-6.03698783585283,
48.5195752075044));
#22506=CARTESIAN_POINT('Ctrl Pts',(-1.12748085797788,-6.05935112779399,
48.51831127849));
#22507=CARTESIAN_POINT('Ctrl Pts',(-1.47443454508558,-6.07568031732946,
48.5173741424643));
#22508=CARTESIAN_POINT('Ctrl Pts',(-2.60108317843058,-6.14582978513443,
48.5172046544322));
#22509=CARTESIAN_POINT('Ctrl Pts',(-3.35185488132463,-6.19184520827618,
48.5141149281108));
#22510=CARTESIAN_POINT('Ctrl Pts',(-4.12419588396466,-6.23345010526292,
48.5059136087023));
#22511=CARTESIAN_POINT('Ctrl Pts',(0.0835265683917245,-6.05386667280684,
48.5195892904706));
#22512=CARTESIAN_POINT('Ctrl Pts',(-0.189103447624509,-6.0538205571228,
48.5195869596226));
#22513=CARTESIAN_POINT('Ctrl Pts',(-0.484557202789109,-6.05830967273256,
48.5196902430863));
#22514=CARTESIAN_POINT('Ctrl Pts',(-1.12692130702108,-6.07865710025598,
48.5193460059677));
#22515=CARTESIAN_POINT('Ctrl Pts',(-1.47382850126476,-6.09455995771879,
48.518913524595));
#22516=CARTESIAN_POINT('Ctrl Pts',(-2.60045731391633,-6.16286923348301,
48.5194534620086));
#22517=CARTESIAN_POINT('Ctrl Pts',(-3.35085408858969,-6.21237399282374,
48.5175683503199));
#22518=CARTESIAN_POINT('Ctrl Pts',(-4.12290068577714,-6.25674581559982,
48.5119171961227));
#22519=CARTESIAN_POINT('Ctrl Pts',(0.0835265683750737,-6.10694539169996,
48.521354690718));
#22520=CARTESIAN_POINT('Ctrl Pts',(-0.227816669563641,-6.1069582237576,
48.521355914551));
#22521=CARTESIAN_POINT('Ctrl Pts',(-0.550623003667509,-6.11145963930881,
48.5214911612936));
#22522=CARTESIAN_POINT('Ctrl Pts',(-1.22201691703506,-6.12977840933438,
48.5214366576209));
#22523=CARTESIAN_POINT('Ctrl Pts',(-1.57060291888689,-6.14361803658331,
48.5212544268105));
#22524=CARTESIAN_POINT('Ctrl Pts',(-2.65931970425501,-6.1996683887915,48.5212339924792));
#22525=CARTESIAN_POINT('Ctrl Pts',(-3.38453260161145,-6.24739159903889,
48.5204767822314));
#22526=CARTESIAN_POINT('Ctrl Pts',(-4.12038695511613,-6.29803503999888,
48.5189262877413));
#22527=CARTESIAN_POINT('Ctrl Pts',(0.0835265683690384,-6.12148849588211,
48.5199317919394));
#22528=CARTESIAN_POINT('Ctrl Pts',(-0.266743231119374,-6.12148849588211,
48.5199317919394));
#22529=CARTESIAN_POINT('Ctrl Pts',(-0.6170520033925,-6.12687873284897,48.5199317919388));
#22530=CARTESIAN_POINT('Ctrl Pts',(-1.31767207799207,-6.14643370208422,
48.5199317919371));
#22531=CARTESIAN_POINT('Ctrl Pts',(-1.66798338031851,-6.1605984343526,48.5199317919361));
#22532=CARTESIAN_POINT('Ctrl Pts',(-2.71880795910365,-6.21324540616174,
48.5199317919341));
#22533=CARTESIAN_POINT('Ctrl Pts',(-3.41921190736816,-6.26188042070648,
48.5199317919341));
#22534=CARTESIAN_POINT('Ctrl Pts',(-4.11916842264263,-6.31602855406106,
48.5199317919394));
#22535=CARTESIAN_POINT('Ctrl Pts',(0.0835265683620147,-6.14692278878554,
48.5199317919394));
#22536=CARTESIAN_POINT('Ctrl Pts',(-0.266821084249497,-6.14692278878554,
48.5199317919394));
#22537=CARTESIAN_POINT('Ctrl Pts',(-0.617168736861009,-6.15072449281721,
48.5199317919388));
#22538=CARTESIAN_POINT('Ctrl Pts',(-1.31778153573106,-6.16593130894387,
48.5199317919372));
#22539=CARTESIAN_POINT('Ctrl Pts',(-1.6680466819896,-6.17733642103887,48.5199317919363));
#22540=CARTESIAN_POINT('Ctrl Pts',(-2.71859460170632,-6.22295686941886,
48.5199317919344));
#22541=CARTESIAN_POINT('Ctrl Pts',(-3.41862985610558,-6.26857731779886,
48.5199317919344));
#22542=CARTESIAN_POINT('Ctrl Pts',(-4.11800505968107,-6.32940458230553,
48.5199317919394));
#22543=CARTESIAN_POINT('',(-4.12551257076669,-6.20946977174738,48.495917231884));
#22544=CARTESIAN_POINT('Ctrl Pts',(-4.11800505968107,-6.32940458230551,
48.5199317919367));
#22545=CARTESIAN_POINT('Ctrl Pts',(-4.11858674116184,-6.32271656818346,
48.5199317638787));
#22546=CARTESIAN_POINT('Ctrl Pts',(-4.11917549964439,-6.31495176722324,
48.5197172285933));
#22547=CARTESIAN_POINT('Ctrl Pts',(-4.11977717145446,-6.30626433210882,
48.5190688039378));
#22548=CARTESIAN_POINT('Ctrl Pts',(-4.12032674885696,-6.29832907912767,
48.5184765216804));
#22549=CARTESIAN_POINT('Ctrl Pts',(-4.12088712278166,-6.28962376481006,
48.517520333247));
#22550=CARTESIAN_POINT('Ctrl Pts',(-4.12145907343358,-6.28030805427432,
48.5160324259247));
#22551=CARTESIAN_POINT('Ctrl Pts',(-4.12200326888234,-6.27144440972983,
48.5146167226812));
#22552=CARTESIAN_POINT('Ctrl Pts',(-4.12255791867854,-6.26202846118951,
48.5127182234746));
#22553=CARTESIAN_POINT('Ctrl Pts',(-4.12312024912556,-6.25223759022031,
48.5102148793545));
#22554=CARTESIAN_POINT('Ctrl Pts',(-4.12365584850649,-6.24291214028643,
48.5078305347612));
#22555=CARTESIAN_POINT('Ctrl Pts',(-4.12419834333242,-6.23324739180506,
48.5048965752648));
#22556=CARTESIAN_POINT('Ctrl Pts',(-4.12474286125808,-6.22342541541294,
48.5013450104422));
#22557=CARTESIAN_POINT('Ctrl Pts',(-4.12499921694512,-6.21880128939725,
48.4996729555891));
#22558=CARTESIAN_POINT('Ctrl Pts',(-4.12525599093568,-6.214142666,48.4978646482433));
#22559=CARTESIAN_POINT('Ctrl Pts',(-4.12551255559153,-6.20946994630408,
48.4959168111364));
#22560=CARTESIAN_POINT('Ctrl Pts',(-4.12551257835429,-6.20946968446903,
48.4959174422579));
#22561=CARTESIAN_POINT('Ctrl Pts',(-3.42379712957049,-6.17306838542386,
48.5061181030979));
#22562=CARTESIAN_POINT('Ctrl Pts',(-2.72152477454993,-6.13245845073777,
48.5108119660831));
#22563=CARTESIAN_POINT('Ctrl Pts',(-1.31995074702773,-6.04366518477761,
48.514117299685));
#22564=CARTESIAN_POINT('Ctrl Pts',(-0.618564041366555,-6.01733942146302,
48.5199462997132));
#22565=CARTESIAN_POINT('Ctrl Pts',(0.0835265683815503,-6.00666333723547,
48.5199460669664));
#22566=CARTESIAN_POINT('Ctrl Pts',(0.0835265683815503,-6.00666333723547,
48.5199460669664));
#22567=CARTESIAN_POINT('Ctrl Pts',(-0.267518736492766,-6.00132529512186,
48.519945950593));
#22568=CARTESIAN_POINT('Ctrl Pts',(-0.61861597912618,-5.99973567328081,
48.5184885224508));
#22569=CARTESIAN_POINT('Ctrl Pts',(-1.32094154226152,-5.99820579736984,
48.5087577021076));
#22570=CARTESIAN_POINT('Ctrl Pts',(-1.67216986276346,-5.99826554329992,
48.5004843099067));
#22571=CARTESIAN_POINT('Ctrl Pts',(-2.7260922445975,-5.99214762358588,48.4595881764337));
#22572=CARTESIAN_POINT('Ctrl Pts',(-3.42734501754431,-5.9947566407883,48.4163876002916));
#22573=CARTESIAN_POINT('Ctrl Pts',(-4.128454810656,-6.007051447105,48.3603316468569));
#22574=CARTESIAN_POINT('Ctrl Pts',(-0.267518736492503,-6.01200137934925,
48.5199461833399));
#22575=CARTESIAN_POINT('Ctrl Pts',(-0.54053515644952,-6.00879525432305,
48.519004334916));
#22576=CARTESIAN_POINT('Ctrl Pts',(-0.831623018753302,-6.00835114797875,
48.5169166777066));
#22577=CARTESIAN_POINT('Ctrl Pts',(-1.44672510888142,-6.00829173506044,
48.5070409830143));
#22578=CARTESIAN_POINT('Ctrl Pts',(-1.77074437164332,-6.00864450579794,
48.4992338112145));
#22579=CARTESIAN_POINT('Ctrl Pts',(-2.7873735152434,-6.00381665756613,48.4591554550849));
#22580=CARTESIAN_POINT('Ctrl Pts',(-3.46432076030098,-6.006970116274,48.4176356671043));
#22581=CARTESIAN_POINT('Ctrl Pts',(-4.12850749787601,-6.01900581052063,
48.3652975204339));
#22582=CARTESIAN_POINT('Ctrl Pts',(-0.618388065344823,-6.02125184123478,
48.5184889915195));
#22583=CARTESIAN_POINT('Ctrl Pts',(-0.831277824717596,-6.01828947675541,
48.5172889554692));
#22584=CARTESIAN_POINT('Ctrl Pts',(-1.07630838450787,-6.01789996842512,
48.5149008816201));
#22585=CARTESIAN_POINT('Ctrl Pts',(-1.62065368277726,-6.01814206511781,
48.5050013605236));
#22586=CARTESIAN_POINT('Ctrl Pts',(-1.91997597366274,-6.01872578610802,
48.4974612118007));
#22587=CARTESIAN_POINT('Ctrl Pts',(-2.88438285982273,-6.015691965127,48.4585450694341));
#22588=CARTESIAN_POINT('Ctrl Pts',(-3.52649817488522,-6.02014444454682,
48.4189800887184));
#22589=CARTESIAN_POINT('Ctrl Pts',(-4.12864057911591,-6.03128117156189,
48.3719827330256));
#22590=CARTESIAN_POINT('Ctrl Pts',(-1.31980082405271,-6.04818290219398,
48.5151613829919));
#22591=CARTESIAN_POINT('Ctrl Pts',(-1.44516286435873,-6.04432658406756,
48.5134046445656));
#22592=CARTESIAN_POINT('Ctrl Pts',(-1.61934713476681,-6.04289085428145,
48.5103147763951));
#22593=CARTESIAN_POINT('Ctrl Pts',(-2.04329097920305,-6.0417352100729,48.4999506928749));
#22594=CARTESIAN_POINT('Ctrl Pts',(-2.29305999373915,-6.0419554406095,48.4926406006807));
#22595=CARTESIAN_POINT('Ctrl Pts',(-3.12263860626336,-6.04033961883415,
48.4565445600434));
#22596=CARTESIAN_POINT('Ctrl Pts',(-3.67166030973921,-6.04594588203862,
48.4216081073828));
#22597=CARTESIAN_POINT('Ctrl Pts',(-4.12920120927185,-6.05467770199134,
48.3864516772669));
#22598=CARTESIAN_POINT('Ctrl Pts',(-1.67034425390828,-6.06586350126765,
48.5132909662846));
#22599=CARTESIAN_POINT('Ctrl Pts',(-1.76830361616495,-6.06089216511445,
48.51123856213));
#22600=CARTESIAN_POINT('Ctrl Pts',(-1.91769808992094,-6.05836696394206,
48.5077487407884));
#22601=CARTESIAN_POINT('Ctrl Pts',(-2.29199666504518,-6.05552058028394,
48.4969449896315));
#22602=CARTESIAN_POINT('Ctrl Pts',(-2.51690957755418,-6.05514353309333,
48.4895975747613));
#22603=CARTESIAN_POINT('Ctrl Pts',(-3.2638833885578,-6.05313466114755,48.4551572853244));
#22604=CARTESIAN_POINT('Ctrl Pts',(-3.75464503000896,-6.0585729912576,48.4228917044332));
#22605=CARTESIAN_POINT('Ctrl Pts',(-4.1296287581879,-6.06579887137954,48.3942354089164));
#22606=CARTESIAN_POINT('Ctrl Pts',(-2.72152477454993,-6.13245845073777,
48.5108119660831));
#22607=CARTESIAN_POINT('Ctrl Pts',(-2.78175048147961,-6.12571278892217,
48.507599134673));
#22608=CARTESIAN_POINT('Ctrl Pts',(-2.87872640152294,-6.1197510150967,48.5025662256946));
#22609=CARTESIAN_POINT('Ctrl Pts',(-3.11802710698666,-6.10935599899705,
48.4895414181605));
#22610=CARTESIAN_POINT('Ctrl Pts',(-3.26035692734462,-6.10489083403437,
48.4815303852878));
#22611=CARTESIAN_POINT('Ctrl Pts',(-3.71314893100167,-6.09364276612037,
48.4510874243765));
#22612=CARTESIAN_POINT('Ctrl Pts',(-3.99041609239207,-6.09193010339169,
48.4262709574899));
#22613=CARTESIAN_POINT('Ctrl Pts',(-4.13155362590487,-6.09473681170807,
48.4157241439942));
#22614=CARTESIAN_POINT('Ctrl Pts',(-3.42379712957049,-6.17306838542386,
48.5061181030979));
#22615=CARTESIAN_POINT('Ctrl Pts',(-3.45976825369342,-6.1636799739977,48.5021196905914));
#22616=CARTESIAN_POINT('Ctrl Pts',(-3.52173694617229,-6.15479195321228,
48.4962278198627));
#22617=CARTESIAN_POINT('Ctrl Pts',(-3.66733280171424,-6.13882811012295,
48.4820050858237));
#22618=CARTESIAN_POINT('Ctrl Pts',(-3.75095996477732,-6.13175228781906,
48.4736742225135));
#22619=CARTESIAN_POINT('Ctrl Pts',(-3.98882416065135,-6.11446024442977,
48.4470450295045));
#22620=CARTESIAN_POINT('Ctrl Pts',(-4.13001933607927,-6.10813589078394,
48.4278950754018));
#22621=CARTESIAN_POINT('Ctrl Pts',(-4.13369316567458,-6.10812801481237,
48.4275666875517));
#22622=CARTESIAN_POINT('Ctrl Pts',(-4.12551257835428,-6.20946968446904,
48.4959174422579));
#22623=CARTESIAN_POINT('Ctrl Pts',(-4.12617092554909,-6.1974794740721,48.4909193590357));
#22624=CARTESIAN_POINT('Ctrl Pts',(-4.12683966151712,-6.18527410478074,
48.484789162884));
#22625=CARTESIAN_POINT('Ctrl Pts',(-4.12827543030072,-6.16205725105381,
48.4713889284507));
#22626=CARTESIAN_POINT('Ctrl Pts',(-4.12904246311627,-6.15104576661825,
48.4641188901692));
#22627=CARTESIAN_POINT('Ctrl Pts',(-4.13160728578581,-6.12223844456225,
48.4422855877235));
#22628=CARTESIAN_POINT('Ctrl Pts',(-4.13366096331981,-6.10843369230011,
48.4278763391901));
#22629=CARTESIAN_POINT('Ctrl Pts',(-4.13722371861489,-6.1084337131847,48.4275653153946));
#22630=CARTESIAN_POINT('Ctrl Pts',(-4.12551257835429,-6.20946968446903,
48.4959174422579));
#22631=CARTESIAN_POINT('Ctrl Pts',(-4.12682927274388,-6.18548926367518,
48.4859212758135));
#22632=CARTESIAN_POINT('Ctrl Pts',(-4.12818752222643,-6.16064820730358,
48.4713966576511));
#22633=CARTESIAN_POINT('Ctrl Pts',(-4.13160728578581,-6.12223844456225,
48.4422855877235));
#22634=CARTESIAN_POINT('Ctrl Pts',(-4.13366096331981,-6.10843369230011,
48.4278763391901));
#22635=CARTESIAN_POINT('Ctrl Pts',(-4.13722371861488,-6.10843371318471,
48.4275653153946));
#22636=CARTESIAN_POINT('',(-4.128454810656,-6.00705144710501,48.3603316468569));
#22637=CARTESIAN_POINT('Ctrl Pts',(-4.128454810656,-6.00705144710501,48.3603316468569));
#22638=CARTESIAN_POINT('Ctrl Pts',(-4.12847724605468,-6.01214188287171,
48.3624462270809));
#22639=CARTESIAN_POINT('Ctrl Pts',(-4.12851349521485,-6.01712839937856,
48.3648008414081));
#22640=CARTESIAN_POINT('Ctrl Pts',(-4.12856659590172,-6.02202475059606,
48.3673129480271));
#22641=CARTESIAN_POINT('Ctrl Pts',(-4.12863240824478,-6.0280932285195,48.3704264223024));
#22642=CARTESIAN_POINT('Ctrl Pts',(-4.12872385551699,-6.03402509336409,
48.3737833452877));
#22643=CARTESIAN_POINT('Ctrl Pts',(-4.12884968366995,-6.03985134815184,
48.3773045718558));
#22644=CARTESIAN_POINT('Ctrl Pts',(-4.12887227551138,-6.04089742425802,
48.3779367911994));
#22645=CARTESIAN_POINT('Ctrl Pts',(-4.12889598882607,-6.04194007207302,
48.3785744384767));
#22646=CARTESIAN_POINT('Ctrl Pts',(-4.12892089419388,-6.04297943677661,
48.3792172051462));
#22647=CARTESIAN_POINT('Ctrl Pts',(-4.12907740642859,-6.04951109266998,
48.3832565290626));
#22648=CARTESIAN_POINT('Ctrl Pts',(-4.12927928721199,-6.05591440502064,
48.3874952504182));
#22649=CARTESIAN_POINT('Ctrl Pts',(-4.12955440546488,-6.06221540874182,
48.3918795150871));
#22650=CARTESIAN_POINT('Ctrl Pts',(-4.129749144932,-6.06667550578774,48.3949828692134));
#22651=CARTESIAN_POINT('Ctrl Pts',(-4.12998024811885,-6.07108307587747,
48.3981593533735));
#22652=CARTESIAN_POINT('Ctrl Pts',(-4.13027038076022,-6.07544485148905,
48.401398320609));
#22653=CARTESIAN_POINT('Ctrl Pts',(-4.13051585714226,-6.07913527698313,
48.4041387566893));
#22654=CARTESIAN_POINT('Ctrl Pts',(-4.13080237637701,-6.08279191115652,
48.406923377578));
#22655=CARTESIAN_POINT('Ctrl Pts',(-4.1311632911292,-6.08641490063092,48.409745887031));
#22656=CARTESIAN_POINT('Ctrl Pts',(-4.13142089737007,-6.08900084286116,
48.4117604792459));
#22657=CARTESIAN_POINT('Ctrl Pts',(-4.13171554465927,-6.09157063046096,
48.4137952446382));
#22658=CARTESIAN_POINT('Ctrl Pts',(-4.13208086203652,-6.09412272337342,
48.4158470897808));
#22659=CARTESIAN_POINT('Ctrl Pts',(-4.13233561746212,-6.09590243481497,
48.4172779515879));
#22660=CARTESIAN_POINT('Ctrl Pts',(-4.1326236272006,-6.09767362900813,48.4187172631575));
#22661=CARTESIAN_POINT('Ctrl Pts',(-4.13297918313311,-6.09943558046489,
48.4201632417151));
#22662=CARTESIAN_POINT('Ctrl Pts',(-4.1332181244978,-6.10061965038779,48.4211349709376));
#22663=CARTESIAN_POINT('Ctrl Pts',(-4.13348648933834,-6.10179994098431,
48.4221101275599));
#22664=CARTESIAN_POINT('Ctrl Pts',(-4.13381763546866,-6.1029736298463,48.4230849222562));
#22665=CARTESIAN_POINT('Ctrl Pts',(-4.13401726738067,-6.10368118983316,
48.4236725786145));
#22666=CARTESIAN_POINT('Ctrl Pts',(-4.13423928223204,-6.10438688630814,
48.4242605993929));
#22667=CARTESIAN_POINT('Ctrl Pts',(-4.13450789108345,-6.10508829918447,
48.4248456081052));
#22668=CARTESIAN_POINT('Ctrl Pts',(-4.13468189352899,-6.10554266826118,
48.4252245715908));
#22669=CARTESIAN_POINT('Ctrl Pts',(-4.13487545529636,-6.10599659049777,
48.4256034524709));
#22670=CARTESIAN_POINT('Ctrl Pts',(-4.1351077826707,-6.10644310670885,48.425975005762));
#22671=CARTESIAN_POINT('Ctrl Pts',(-4.13523410076814,-6.10668588084782,
48.4261770220115));
#22672=CARTESIAN_POINT('Ctrl Pts',(-4.13537284994624,-6.10692799624868,
48.4263781398347));
#22673=CARTESIAN_POINT('Ctrl Pts',(-4.13553088498902,-6.10716341124115,
48.4265725981583));
#22674=CARTESIAN_POINT('Ctrl Pts',(-4.13565915175361,-6.10735448227761,
48.4267304273306));
#22675=CARTESIAN_POINT('Ctrl Pts',(-4.13579977890918,-6.10754133617494,
48.4268840707421));
#22676=CARTESIAN_POINT('Ctrl Pts',(-4.13596274135563,-6.10771844494464,
48.4270278886976));
#22677=CARTESIAN_POINT('Ctrl Pts',(-4.13604422257886,-6.10780699932949,
48.4270997976754));
#22678=CARTESIAN_POINT('Ctrl Pts',(-4.13612859947745,-6.10789132123182,
48.4271678595123));
#22679=CARTESIAN_POINT('Ctrl Pts',(-4.1362343104114,-6.10798127288396,48.4272394029535));
#22680=CARTESIAN_POINT('Ctrl Pts',(-4.13628716587837,-6.10802624871004,
48.4272751746741));
#22681=CARTESIAN_POINT('Ctrl Pts',(-4.13634156485444,-6.10807104932053,
48.4273106966924));
#22682=CARTESIAN_POINT('Ctrl Pts',(-4.13643190669548,-6.10813310869716,
48.4273588375411));
#22683=CARTESIAN_POINT('Ctrl Pts',(-4.13647707759982,-6.10816413837435,
48.4273829079569));
#22684=CARTESIAN_POINT('Ctrl Pts',(-4.13654110267543,-6.10820885152138,
48.4274176883991));
#22685=CARTESIAN_POINT('Ctrl Pts',(-4.13665996059634,-6.10826888896282,
48.427461956441));
#22686=CARTESIAN_POINT('Ctrl Pts',(-4.13674745395857,-6.10831308355725,
48.427494542909));
#22687=CARTESIAN_POINT('Ctrl Pts',(-4.13686461503084,-6.10836602282818,
48.4275326992659));
#22688=CARTESIAN_POINT('Ctrl Pts',(-4.13702847377054,-6.10840319283375,
48.4275531996689));
#22689=CARTESIAN_POINT('Ctrl Pts',(-4.1370872137358,-6.1084165175111,48.4275605486389));
#22690=CARTESIAN_POINT('Ctrl Pts',(-4.13715198788423,-6.10842750223913,
48.4275653432463));
#22691=CARTESIAN_POINT('Ctrl Pts',(-4.13722371803033,-6.10843371313409,
48.4275653153948));
#22692=CARTESIAN_POINT('Ctrl Pts',(-4.128454810656,-6.00705144710501,48.3603316468569));
#22693=CARTESIAN_POINT('Ctrl Pts',(-3.42734501754431,-5.9947566407883,48.4163876002916));
#22694=CARTESIAN_POINT('Ctrl Pts',(-2.7260922445975,-5.99214762358588,48.4595881764337));
#22695=CARTESIAN_POINT('Ctrl Pts',(-1.32086240215211,-6.00030484987126,
48.5141163543976));
#22696=CARTESIAN_POINT('Ctrl Pts',(-0.618564041367084,-5.99598725300824,
48.5199458342196));
#22697=CARTESIAN_POINT('Ctrl Pts',(0.0835265683815503,-6.00666333723547,
48.5199460669664));
#22698=CARTESIAN_POINT('Ctrl Pts',(-48.353987706665,-6.00666333723547,0.0824317919588709));
#22699=CARTESIAN_POINT('Ctrl Pts',(-48.3539881721587,-6.02801550569024,
0.082431791959394));
#22700=CARTESIAN_POINT('Ctrl Pts',(-48.3536309301691,-6.05386667280685,
0.0824317919690549));
#22701=CARTESIAN_POINT('Ctrl Pts',(-48.3553963304166,-6.10694539169998,
0.082431791952385));
#22702=CARTESIAN_POINT('Ctrl Pts',(-48.3539734316379,-6.12148849588211,
0.0824317919463454));
#22703=CARTESIAN_POINT('Ctrl Pts',(-48.3539734316379,-6.14692278878554,
0.0824317919393188));
#22704=CARTESIAN_POINT('Ctrl Pts',(-48.3539878230387,-6.01200137934915,
0.433477096833169));
#22705=CARTESIAN_POINT('Ctrl Pts',(-48.3539286009829,-6.0309091878989,0.355275147603605));
#22706=CARTESIAN_POINT('Ctrl Pts',(-48.3536285993218,-6.05382055712376,
0.355061807985282));
#22707=CARTESIAN_POINT('Ctrl Pts',(-48.3553975542498,-6.10695822375809,
0.393775029891096));
#22708=CARTESIAN_POINT('Ctrl Pts',(-48.3539734316379,-6.12148849588211,
0.432701591434755));
#22709=CARTESIAN_POINT('Ctrl Pts',(-48.3539734316379,-6.14692278878554,
0.432779444550827));
#22710=CARTESIAN_POINT('Ctrl Pts',(-48.3525306312191,-6.02125184123593,
0.784346425692766));
#22711=CARTESIAN_POINT('Ctrl Pts',(-48.353616847204,-6.03698783585502,0.650878762005552));
#22712=CARTESIAN_POINT('Ctrl Pts',(-48.3537318827856,-6.05830967273448,
0.650515563154517));
#22713=CARTESIAN_POINT('Ctrl Pts',(-48.3555328009924,-6.11145963930963,
0.716581363996309));
#22714=CARTESIAN_POINT('Ctrl Pts',(-48.3539734316373,-6.12687873284897,
0.783010363707002));
#22715=CARTESIAN_POINT('Ctrl Pts',(-48.3539734316373,-6.15072449281721,
0.783127097162336));
#22716=CARTESIAN_POINT('Ctrl Pts',(-48.3492030226928,-6.04818290219923,
1.48575918442931));
#22717=CARTESIAN_POINT('Ctrl Pts',(-48.3523529181898,-6.05935112779917,
1.29343921835598));
#22718=CARTESIAN_POINT('Ctrl Pts',(-48.353387645667,-6.07865710025985,1.29287966739942));
#22719=CARTESIAN_POINT('Ctrl Pts',(-48.3554782973195,-6.12977840933566,
1.38797527736651));
#22720=CARTESIAN_POINT('Ctrl Pts',(-48.3539734316356,-6.14643370208422,
1.48363043830394));
#22721=CARTESIAN_POINT('Ctrl Pts',(-48.3539734316357,-6.16593130894386,
1.48373989603238));
#22722=CARTESIAN_POINT('Ctrl Pts',(-48.3473326059861,-6.06586350127576,
1.83630261430625));
#22723=CARTESIAN_POINT('Ctrl Pts',(-48.3514157821642,-6.0756803173363,1.64039290548077));
#22724=CARTESIAN_POINT('Ctrl Pts',(-48.3529551642942,-6.09455995772361,
1.6397868616514));
#22725=CARTESIAN_POINT('Ctrl Pts',(-48.3552960665089,-6.14361803658471,
1.73656127921966));
#22726=CARTESIAN_POINT('Ctrl Pts',(-48.3539734316346,-6.1605984343526,1.83394174062863));
#22727=CARTESIAN_POINT('Ctrl Pts',(-48.3539734316348,-6.17733642103886,
1.83400504229092));
#22728=CARTESIAN_POINT('Ctrl Pts',(-48.3448536057857,-6.13245845075532,
2.88748313503321));
#22729=CARTESIAN_POINT('Ctrl Pts',(-48.3512462941318,-6.14582978514638,
2.76704153887883));
#22730=CARTESIAN_POINT('Ctrl Pts',(-48.3534951017072,-6.16286923349057,
2.76641567432489));
#22731=CARTESIAN_POINT('Ctrl Pts',(-48.3552756321772,-6.19966838879309,
2.82527806458757));
#22732=CARTESIAN_POINT('Ctrl Pts',(-48.3539734316326,-6.21324540616174,
2.8847663194085));
#22733=CARTESIAN_POINT('Ctrl Pts',(-48.3539734316329,-6.22295686941885,
2.88455296200763));
#22734=CARTESIAN_POINT('Ctrl Pts',(-48.3401597427993,-6.17306838545285,
3.5897554902018));
#22735=CARTESIAN_POINT('Ctrl Pts',(-48.3481565678091,-6.19184520829409,
3.51781324186406));
#22736=CARTESIAN_POINT('Ctrl Pts',(-48.3516099900174,-6.21237399283442,
3.51681244904663));
#22737=CARTESIAN_POINT('Ctrl Pts',(-48.3545184219291,-6.24739159904061,
3.55049096194934));
#22738=CARTESIAN_POINT('Ctrl Pts',(-48.3539734316326,-6.26188042070648,
3.58517026766949));
#22739=CARTESIAN_POINT('Ctrl Pts',(-48.3539734316329,-6.26857731779884,
3.58458821640688));
#22740=CARTESIAN_POINT('Ctrl Pts',(-48.3299590819564,-6.20946968450872,
4.29147093911199));
#22741=CARTESIAN_POINT('Ctrl Pts',(-48.3399552484009,-6.23345010528184,
4.29015424448251));
#22742=CARTESIAN_POINT('Ctrl Pts',(-48.3459588358212,-6.25674581560882,
4.28885904618088));
#22743=CARTESIAN_POINT('Ctrl Pts',(-48.3529679274398,-6.29803503999844,
4.28634531541159));
#22744=CARTESIAN_POINT('Ctrl Pts',(-48.3539734316379,-6.31602855406108,
4.28512678294393));
#22745=CARTESIAN_POINT('Ctrl Pts',(-48.3539734316379,-6.32940458230551,
4.28396341998237));
#22746=CARTESIAN_POINT('',(-48.3299588608603,-6.20946977623549,4.29147093113758));
#22747=CARTESIAN_POINT('',(-48.353987706665,-6.00666333723547,0.0824317919588709));
#22748=CARTESIAN_POINT('Ctrl Pts',(-48.3299590819564,-6.2094696845087,4.291470939112));
#22749=CARTESIAN_POINT('Ctrl Pts',(-48.3401597427993,-6.17306838545285,
3.5897554902018));
#22750=CARTESIAN_POINT('Ctrl Pts',(-48.3448536057857,-6.13245845075532,
2.88748313503321));
#22751=CARTESIAN_POINT('Ctrl Pts',(-48.3481589393863,-6.04366518478258,
1.48590910739726));
#22752=CARTESIAN_POINT('Ctrl Pts',(-48.3539879394125,-6.01733942146283,
0.784522401707471));
#22753=CARTESIAN_POINT('Ctrl Pts',(-48.353987706665,-6.00666333723547,0.0824317919588709));
#22754=CARTESIAN_POINT('Ctrl Pts',(-48.3299584186682,-6.20946995968904,
4.29147091518876));
#22755=CARTESIAN_POINT('Ctrl Pts',(-48.3340747811502,-6.2193448070199,4.29092871768642));
#22756=CARTESIAN_POINT('Ctrl Pts',(-48.3375647029145,-6.22915570483183,
4.29038566954877));
#22757=CARTESIAN_POINT('Ctrl Pts',(-48.3404726016179,-6.23871408127374,
4.28984735821603));
#22758=CARTESIAN_POINT('Ctrl Pts',(-48.3435579448646,-6.24885572484959,
4.28927619828079));
#22759=CARTESIAN_POINT('Ctrl Pts',(-48.3459887705052,-6.25871184341282,
4.28871047939837));
#22760=CARTESIAN_POINT('Ctrl Pts',(-48.3478713812869,-6.26808527594661,
4.28815447282215));
#22761=CARTESIAN_POINT('Ctrl Pts',(-48.3498400177411,-6.27788702634906,
4.28757305959252));
#22762=CARTESIAN_POINT('Ctrl Pts',(-48.3512107408118,-6.28716030960557,
4.28700232501256));
#22763=CARTESIAN_POINT('Ctrl Pts',(-48.3521434975818,-6.2957252017122,4.2864432263021));
#22764=CARTESIAN_POINT('Ctrl Pts',(-48.353157498511,-6.30503610551134,4.28583542946793));
#22765=CARTESIAN_POINT('Ctrl Pts',(-48.3536561387394,-6.31350977078185,
4.28524139166978));
#22766=CARTESIAN_POINT('Ctrl Pts',(-48.3538589105089,-6.32097498479566,
4.28465714448851));
#22767=CARTESIAN_POINT('Ctrl Pts',(-48.3539396358021,-6.32394695466908,
4.28442455035012));
#22768=CARTESIAN_POINT('Ctrl Pts',(-48.3539734197696,-6.32675971428296,
4.28419345399841));
#22769=CARTESIAN_POINT('Ctrl Pts',(-48.3539734316348,-6.32940458230554,
4.28396341998237));
#22770=CARTESIAN_POINT('Ctrl Pts',(-48.3539734316379,-6.14692278878557,
0.0824317919393188));
#22771=CARTESIAN_POINT('Ctrl Pts',(-48.3539734316379,-6.12148849588211,
0.0824317919463454));
#22772=CARTESIAN_POINT('Ctrl Pts',(-48.3553963304166,-6.10694539169998,
0.082431791952385));
#22773=CARTESIAN_POINT('Ctrl Pts',(-48.3536309301691,-6.05386667280685,
0.0824317919690549));
#22774=CARTESIAN_POINT('Ctrl Pts',(-48.3539881721587,-6.02801550569024,
0.082431791959394));
#22775=CARTESIAN_POINT('Ctrl Pts',(-48.353987706665,-6.00666333723547,0.0824317919588709));
#22776=CARTESIAN_POINT('Ctrl Pts',(-48.353987706665,-6.00666333723547,0.0824317919588709));
#22777=CARTESIAN_POINT('Ctrl Pts',(-48.3539878230381,-6.01200137934917,
-0.268613512915165));
#22778=CARTESIAN_POINT('Ctrl Pts',(-48.3525306312174,-6.02125184123468,
-0.619482841767479));
#22779=CARTESIAN_POINT('Ctrl Pts',(-48.3492030226894,-6.04818290219387,
-1.32089560047537));
#22780=CARTESIAN_POINT('Ctrl Pts',(-48.3473326059821,-6.06586350126756,
-1.67143903033095));
#22781=CARTESIAN_POINT('Ctrl Pts',(-48.3448536057816,-6.13245845073776,
-2.72261955097263));
#22782=CARTESIAN_POINT('Ctrl Pts',(-48.3401597427964,-6.17306838542386,
-3.42489190599315));
#22783=CARTESIAN_POINT('Ctrl Pts',(-48.3299590819564,-6.20946968446904,
-4.12660735477694));
#22784=CARTESIAN_POINT('Ctrl Pts',(-48.3539881721587,-6.02801550569024,
0.082431791959394));
#22785=CARTESIAN_POINT('Ctrl Pts',(-48.3539286009819,-6.03090918789793,
-0.190411563683277));
#22786=CARTESIAN_POINT('Ctrl Pts',(-48.3536168472025,-6.03698783585276,
-0.486015178076197));
#22787=CARTESIAN_POINT('Ctrl Pts',(-48.3523529181877,-6.05935112779389,
-1.1285756344005));
#22788=CARTESIAN_POINT('Ctrl Pts',(-48.351415782162,-6.07568031732935,-1.47552932150819));
#22789=CARTESIAN_POINT('Ctrl Pts',(-48.3512462941307,-6.14582978513439,
-2.60217795485319));
#22790=CARTESIAN_POINT('Ctrl Pts',(-48.3481565678094,-6.19184520827618,
-3.35294965774719));
#22791=CARTESIAN_POINT('Ctrl Pts',(-48.3399552484008,-6.23345010526292,
-4.12529066038733));
#22792=CARTESIAN_POINT('Ctrl Pts',(-48.3536309301691,-6.05386667280685,
0.0824317919690549));
#22793=CARTESIAN_POINT('Ctrl Pts',(-48.353628599321,-6.05382055712278,-0.190198224047172));
#22794=CARTESIAN_POINT('Ctrl Pts',(-48.3537318827846,-6.05830967273253,
-0.485651979211756));
#22795=CARTESIAN_POINT('Ctrl Pts',(-48.3533876456657,-6.07865710025591,
-1.1280160834437));
#22796=CARTESIAN_POINT('Ctrl Pts',(-48.352955164293,-6.0945599577187,-1.47492327768737));
#22797=CARTESIAN_POINT('Ctrl Pts',(-48.3534951017072,-6.16286923348297,
-2.60155209033893));
#22798=CARTESIAN_POINT('Ctrl Pts',(-48.3516099900184,-6.21237399282373,
-3.35194886501225));
#22799=CARTESIAN_POINT('Ctrl Pts',(-48.3459588358212,-6.25674581559982,
-4.12399546219981));
#22800=CARTESIAN_POINT('Ctrl Pts',(-48.3553963304166,-6.10694539169998,
0.082431791952385));
#22801=CARTESIAN_POINT('Ctrl Pts',(-48.3553975542495,-6.1069582237576,-0.228911445986326));
#22802=CARTESIAN_POINT('Ctrl Pts',(-48.3555328009921,-6.11145963930882,
-0.551717780090184));
#22803=CARTESIAN_POINT('Ctrl Pts',(-48.3554782973193,-6.12977840933436,
-1.22311169345771));
#22804=CARTESIAN_POINT('Ctrl Pts',(-48.3552960665088,-6.14361803658328,
-1.57169769530953));
#22805=CARTESIAN_POINT('Ctrl Pts',(-48.3552756321777,-6.19966838879149,
-2.66041448067764));
#22806=CARTESIAN_POINT('Ctrl Pts',(-48.35451842193,-6.24739159903889,-3.38562737803406));
#22807=CARTESIAN_POINT('Ctrl Pts',(-48.3529679274398,-6.29803503999889,
-4.12148173153879));
#22808=CARTESIAN_POINT('Ctrl Pts',(-48.3539734316379,-6.12148849588211,
0.0824317919463454));
#22809=CARTESIAN_POINT('Ctrl Pts',(-48.3539734316379,-6.12148849588211,
-0.267838007542064));
#22810=CARTESIAN_POINT('Ctrl Pts',(-48.3539734316373,-6.12687873284897,
-0.618146779815187));
#22811=CARTESIAN_POINT('Ctrl Pts',(-48.3539734316356,-6.14643370208422,
-1.31876685441475));
#22812=CARTESIAN_POINT('Ctrl Pts',(-48.3539734316346,-6.1605984343526,-1.66907815674119));
#22813=CARTESIAN_POINT('Ctrl Pts',(-48.3539734316326,-6.21324540616174,
-2.71990273552632));
#22814=CARTESIAN_POINT('Ctrl Pts',(-48.3539734316326,-6.26188042070648,
-3.42030668379082));
#22815=CARTESIAN_POINT('Ctrl Pts',(-48.3539734316379,-6.31602855406106,
-4.12026319906529));
#22816=CARTESIAN_POINT('Ctrl Pts',(-48.3539734316379,-6.14692278878554,
0.0824317919393188));
#22817=CARTESIAN_POINT('Ctrl Pts',(-48.3539734316379,-6.14692278878554,
-0.26791586067219));
#22818=CARTESIAN_POINT('Ctrl Pts',(-48.3539734316373,-6.15072449281721,
-0.618263513283698));
#22819=CARTESIAN_POINT('Ctrl Pts',(-48.3539734316357,-6.16593130894387,
-1.31887631215375));
#22820=CARTESIAN_POINT('Ctrl Pts',(-48.3539734316348,-6.17733642103887,
-1.66914145841228));
#22821=CARTESIAN_POINT('Ctrl Pts',(-48.3539734316329,-6.22295686941886,
-2.71968937812899));
#22822=CARTESIAN_POINT('Ctrl Pts',(-48.3539734316329,-6.26857731779886,
-3.41972463252824));
#22823=CARTESIAN_POINT('Ctrl Pts',(-48.3539734316379,-6.32940458230553,
-4.11909983610373));
#22824=CARTESIAN_POINT('',(-48.3299588715825,-6.2094697717474,-4.12660734718935));
#22825=CARTESIAN_POINT('Ctrl Pts',(-48.3539734316352,-6.32940458230556,
-4.11909983610374));
#22826=CARTESIAN_POINT('Ctrl Pts',(-48.3539734035773,-6.32271656818349,
-4.1196815175845));
#22827=CARTESIAN_POINT('Ctrl Pts',(-48.3537588682918,-6.31495176722325,
-4.12027027606706));
#22828=CARTESIAN_POINT('Ctrl Pts',(-48.3531104436363,-6.30626433210883,
-4.12087194787713));
#22829=CARTESIAN_POINT('Ctrl Pts',(-48.3525181613788,-6.29832907912765,
-4.12142152527963));
#22830=CARTESIAN_POINT('Ctrl Pts',(-48.3515619729455,-6.28962376480999,
-4.12198189920433));
#22831=CARTESIAN_POINT('Ctrl Pts',(-48.3500740656231,-6.28030805427421,
-4.12255384985624));
#22832=CARTESIAN_POINT('Ctrl Pts',(-48.3486583623796,-6.27144440972966,
-4.12309804530501));
#22833=CARTESIAN_POINT('Ctrl Pts',(-48.346759863173,-6.26202846118927,-4.12365269510123));
#22834=CARTESIAN_POINT('Ctrl Pts',(-48.3442565190529,-6.25223759022,-4.12421502554824));
#22835=CARTESIAN_POINT('Ctrl Pts',(-48.3418721744595,-6.24291214028606,
-4.12475062492918));
#22836=CARTESIAN_POINT('Ctrl Pts',(-48.3389382149631,-6.23324739180464,
-4.1252931197551));
#22837=CARTESIAN_POINT('Ctrl Pts',(-48.3353866501404,-6.22342541541245,
-4.12583763768076));
#22838=CARTESIAN_POINT('Ctrl Pts',(-48.3337145952874,-6.21880128939694,
-4.12609399336779));
#22839=CARTESIAN_POINT('Ctrl Pts',(-48.3319062879416,-6.21414266599987,
-4.12635076735834));
#22840=CARTESIAN_POINT('Ctrl Pts',(-48.3299584508348,-6.20946994630412,
-4.12660733201417));
#22841=CARTESIAN_POINT('Ctrl Pts',(-48.3299590819564,-6.20946968446903,
-4.12660735477694));
#22842=CARTESIAN_POINT('Ctrl Pts',(-48.3401597427964,-6.17306838542386,
-3.42489190599315));
#22843=CARTESIAN_POINT('Ctrl Pts',(-48.3448536057816,-6.13245845073776,
-2.72261955097264));
#22844=CARTESIAN_POINT('Ctrl Pts',(-48.3481589393823,-6.04366518477749,
-1.32104552345038));
#22845=CARTESIAN_POINT('Ctrl Pts',(-48.3539879394112,-6.01733942146287,
-0.619658817789202));
#22846=CARTESIAN_POINT('Ctrl Pts',(-48.353987706665,-6.00666333723547,0.0824317919588709));
#22847=CARTESIAN_POINT('Ctrl Pts',(-48.353987706665,-6.00666333723547,0.0824317919588709));
#22848=CARTESIAN_POINT('Ctrl Pts',(-48.3539875902912,-6.00132529512179,
-0.268613512915427));
#22849=CARTESIAN_POINT('Ctrl Pts',(-48.3525301621487,-5.99973567328071,
-0.61971075554883));
#22850=CARTESIAN_POINT('Ctrl Pts',(-48.3427993418052,-5.99820579736973,
-1.32203631868417));
#22851=CARTESIAN_POINT('Ctrl Pts',(-48.3345259496042,-5.99826554329983,
-1.67326463918611));
#22852=CARTESIAN_POINT('Ctrl Pts',(-48.2936298161322,-5.99214762358588,
-2.72718702102022));
#22853=CARTESIAN_POINT('Ctrl Pts',(-48.2504292399901,-5.99475664078831,
-3.42843979396698));
#22854=CARTESIAN_POINT('Ctrl Pts',(-48.1943732865555,-6.00705144710501,
-4.12954958707863));
#22855=CARTESIAN_POINT('Ctrl Pts',(-48.3539878230381,-6.01200137934917,
-0.268613512915165));
#22856=CARTESIAN_POINT('Ctrl Pts',(-48.353045974614,-6.00879525432293,-0.541629932872173));
#22857=CARTESIAN_POINT('Ctrl Pts',(-48.3509583174043,-6.00835114797862,
-0.832717795175944));
#22858=CARTESIAN_POINT('Ctrl Pts',(-48.3410826227118,-6.00829173506032,
-1.44781988530405));
#22859=CARTESIAN_POINT('Ctrl Pts',(-48.3332754509119,-6.00864450579782,
-1.77183914806596));
#22860=CARTESIAN_POINT('Ctrl Pts',(-48.2931970947834,-6.00381665756611,
-2.78846829166608));
#22861=CARTESIAN_POINT('Ctrl Pts',(-48.2516773068029,-6.00697011627401,
-3.46541553672362));
#22862=CARTESIAN_POINT('Ctrl Pts',(-48.1993391601324,-6.01900581052064,
-4.12960227429863));
#22863=CARTESIAN_POINT('Ctrl Pts',(-48.3525306312174,-6.02125184123468,
-0.619482841767479));
#22864=CARTESIAN_POINT('Ctrl Pts',(-48.3513305951669,-6.01828947675528,
-0.832372601140253));
#22865=CARTESIAN_POINT('Ctrl Pts',(-48.3489425213176,-6.01789996842498,
-1.07740316093052));
#22866=CARTESIAN_POINT('Ctrl Pts',(-48.3390430002211,-6.01814206511767,
-1.6217484591999));
#22867=CARTESIAN_POINT('Ctrl Pts',(-48.3315028514982,-6.0187257861079,-1.92107075008537));
#22868=CARTESIAN_POINT('Ctrl Pts',(-48.2925867091325,-6.01569196512697,
-2.8854776362454));
#22869=CARTESIAN_POINT('Ctrl Pts',(-48.2530217284169,-6.02014444454683,
-3.52759295130783));
#22870=CARTESIAN_POINT('Ctrl Pts',(-48.2060243727241,-6.0312811715619,-4.12973535553853));
#22871=CARTESIAN_POINT('Ctrl Pts',(-48.3492030226894,-6.04818290219387,
-1.32089560047537));
#22872=CARTESIAN_POINT('Ctrl Pts',(-48.3474462842631,-6.04432658406742,
-1.44625764078141));
#22873=CARTESIAN_POINT('Ctrl Pts',(-48.3443564160926,-6.04289085428131,
-1.62044191118949));
#22874=CARTESIAN_POINT('Ctrl Pts',(-48.3339923325724,-6.04173521007275,
-2.04438575562572));
#22875=CARTESIAN_POINT('Ctrl Pts',(-48.3266822403782,-6.04195544060936,
-2.2941547701618));
#22876=CARTESIAN_POINT('Ctrl Pts',(-48.2905861997417,-6.04033961883411,
-3.12373338268601));
#22877=CARTESIAN_POINT('Ctrl Pts',(-48.2556497470813,-6.04594588203863,
-3.6727550861618));
#22878=CARTESIAN_POINT('Ctrl Pts',(-48.2204933169654,-6.05467770199135,
-4.13029598569448));
#22879=CARTESIAN_POINT('Ctrl Pts',(-48.3473326059821,-6.06586350126756,
-1.67143903033095));
#22880=CARTESIAN_POINT('Ctrl Pts',(-48.3452802018275,-6.06089216511434,
-1.76939839258765));
#22881=CARTESIAN_POINT('Ctrl Pts',(-48.3417903804858,-6.05836696394193,
-1.91879286634364));
#22882=CARTESIAN_POINT('Ctrl Pts',(-48.330986629329,-6.0555205802838,-2.29309144146787));
#22883=CARTESIAN_POINT('Ctrl Pts',(-48.3236392144589,-6.05514353309318,
-2.51800435397685));
#22884=CARTESIAN_POINT('Ctrl Pts',(-48.2891989250228,-6.0531346611475,-3.26497816498047));
#22885=CARTESIAN_POINT('Ctrl Pts',(-48.2569333441317,-6.05857299125762,
-3.75573980643155));
#22886=CARTESIAN_POINT('Ctrl Pts',(-48.2282770486149,-6.06579887137955,
-4.13072353461054));
#22887=CARTESIAN_POINT('Ctrl Pts',(-48.3448536057816,-6.13245845073776,
-2.72261955097264));
#22888=CARTESIAN_POINT('Ctrl Pts',(-48.3416407743715,-6.12571278892215,
-2.78284525790236));
#22889=CARTESIAN_POINT('Ctrl Pts',(-48.336607865393,-6.11975101509667,-2.87982117794571));
#22890=CARTESIAN_POINT('Ctrl Pts',(-48.3235830578589,-6.109355998997,-3.11912188340943));
#22891=CARTESIAN_POINT('Ctrl Pts',(-48.3155720249862,-6.10489083403431,
-3.26145170376736));
#22892=CARTESIAN_POINT('Ctrl Pts',(-48.285129064075,-6.09364276612035,-3.71424370742436));
#22893=CARTESIAN_POINT('Ctrl Pts',(-48.2603125971885,-6.09193010339171,
-3.99151086881468));
#22894=CARTESIAN_POINT('Ctrl Pts',(-48.2497657836928,-6.09473681170808,
-4.1326484023275));
#22895=CARTESIAN_POINT('Ctrl Pts',(-48.3401597427964,-6.17306838542386,
-3.42489190599315));
#22896=CARTESIAN_POINT('Ctrl Pts',(-48.3361613302899,-6.16367997399771,
-3.46086303011612));
#22897=CARTESIAN_POINT('Ctrl Pts',(-48.3302694595612,-6.15479195321228,
-3.52283172259502));
#22898=CARTESIAN_POINT('Ctrl Pts',(-48.3160467255223,-6.13882811012296,
-3.66842757813698));
#22899=CARTESIAN_POINT('Ctrl Pts',(-48.307715862212,-6.13175228781906,-3.75205474120005));
#22900=CARTESIAN_POINT('Ctrl Pts',(-48.2810866692031,-6.11446024442978,
-3.98991893707404));
#22901=CARTESIAN_POINT('Ctrl Pts',(-48.2619367151003,-6.10813589078396,
-4.13111411250191));
#22902=CARTESIAN_POINT('Ctrl Pts',(-48.2616083272502,-6.10812801481237,
-4.13478794209722));
#22903=CARTESIAN_POINT('Ctrl Pts',(-48.3299590819564,-6.20946968446904,
-4.12660735477694));
#22904=CARTESIAN_POINT('Ctrl Pts',(-48.3249609987342,-6.1974794740721,-4.12726570197174));
#22905=CARTESIAN_POINT('Ctrl Pts',(-48.3188308025825,-6.18527410478074,
-4.12793443793977));
#22906=CARTESIAN_POINT('Ctrl Pts',(-48.3054305681492,-6.16205725105381,
-4.12937020672336));
#22907=CARTESIAN_POINT('Ctrl Pts',(-48.2981605298677,-6.15104576661825,
-4.13013723953891));
#22908=CARTESIAN_POINT('Ctrl Pts',(-48.2763272274221,-6.12223844456225,
-4.13270206220845));
#22909=CARTESIAN_POINT('Ctrl Pts',(-48.2619179788887,-6.10843369230012,
-4.13475573974244));
#22910=CARTESIAN_POINT('Ctrl Pts',(-48.2616069550931,-6.10843371318471,
-4.13831849503753));
#22911=CARTESIAN_POINT('Ctrl Pts',(-48.3299590819564,-6.20946968446903,
-4.12660735477694));
#22912=CARTESIAN_POINT('Ctrl Pts',(-48.319962915512,-6.18548926367518,-4.12792404916654));
#22913=CARTESIAN_POINT('Ctrl Pts',(-48.3054382973496,-6.16064820730356,
-4.12928229864908));
#22914=CARTESIAN_POINT('Ctrl Pts',(-48.2763272274221,-6.12223844456225,
-4.13270206220845));
#22915=CARTESIAN_POINT('Ctrl Pts',(-48.2619179788887,-6.10843369230012,
-4.13475573974244));
#22916=CARTESIAN_POINT('Ctrl Pts',(-48.2616069550931,-6.10843371318472,
-4.13831849503754));
#22917=CARTESIAN_POINT('',(-48.1943732865555,-6.00705144710502,-4.12954958707863));
#22918=CARTESIAN_POINT('Ctrl Pts',(-48.2616069550931,-6.10843371318472,
-4.13831849503754));
#22919=CARTESIAN_POINT('Ctrl Pts',(-48.2616096994074,-6.10782231644003,
-4.1312573891569));
#22920=CARTESIAN_POINT('Ctrl Pts',(-48.2142367808633,-6.05486890076757,
-4.12976033595866));
#22921=CARTESIAN_POINT('Ctrl Pts',(-48.1943732865555,-6.00705144710502,
-4.12954958707863));
#22922=CARTESIAN_POINT('Ctrl Pts',(-48.1943732865555,-6.00705144710502,
-4.12954958707863));
#22923=CARTESIAN_POINT('Ctrl Pts',(-48.2504292399901,-5.99475664078831,
-3.42843979396698));
#22924=CARTESIAN_POINT('Ctrl Pts',(-48.2936298161323,-5.99214762358588,
-2.72718702102021));
#22925=CARTESIAN_POINT('Ctrl Pts',(-48.3481579940948,-6.00030484987115,
-1.32195717857475));
#22926=CARTESIAN_POINT('Ctrl Pts',(-48.3539874739176,-5.99598725300811,
-0.619658817789722));
#22927=CARTESIAN_POINT('Ctrl Pts',(-48.353987706665,-6.00666333723547,0.0824317919588709));
#22928=CARTESIAN_POINT('Ctrl Pts',(-48.353987706665,-6.00666333723547,0.0824317919588709));
#22929=CARTESIAN_POINT('Ctrl Pts',(-48.3539872411712,-5.9853111687807,0.0824317919583475));
#22930=CARTESIAN_POINT('Ctrl Pts',(-48.353628932479,-5.96223275463528,0.0824317919477567));
#22931=CARTESIAN_POINT('Ctrl Pts',(-48.3495242804801,-5.92795641804994,
0.0824317919456884));
#22932=CARTESIAN_POINT('Ctrl Pts',(-48.3539734316379,-5.90583775506839,
0.0824317919453202));
#22933=CARTESIAN_POINT('Ctrl Pts',(-48.3539734316379,-5.88746284406389,
0.0824317919393457));
#22934=CARTESIAN_POINT('Ctrl Pts',(-48.3539875902912,-6.00132529512179,
-0.268613512915427));
#22935=CARTESIAN_POINT('Ctrl Pts',(-48.3539275501301,-5.98270666392102,
-0.190757692317236));
#22936=CARTESIAN_POINT('Ctrl Pts',(-48.3536632315908,-5.96240686080377,
-0.173571652624935));
#22937=CARTESIAN_POINT('Ctrl Pts',(-48.3495016480342,-5.92787973562318,
-0.195374050181301));
#22938=CARTESIAN_POINT('Ctrl Pts',(-48.353973431638,-5.90583775506839,-0.234362487437545));
#22939=CARTESIAN_POINT('Ctrl Pts',(-48.3539734316379,-5.88746284406389,
-0.26885562075853));
#22940=CARTESIAN_POINT('Ctrl Pts',(-48.3525301621487,-5.99973567328071,
-0.61971075554883));
#22941=CARTESIAN_POINT('Ctrl Pts',(-48.352733527773,-5.98152768121118,-0.48634291779545));
#22942=CARTESIAN_POINT('Ctrl Pts',(-48.3522992264081,-5.96239709811723,
-0.46057610468301));
#22943=CARTESIAN_POINT('Ctrl Pts',(-48.3473885441251,-5.92723732580308,
-0.501601281232533));
#22944=CARTESIAN_POINT('Ctrl Pts',(-48.3508557705022,-5.90562906540036,
-0.568393270900862));
#22945=CARTESIAN_POINT('Ctrl Pts',(-48.3501520759131,-5.88746284406389,
-0.620143038727584));
#22946=CARTESIAN_POINT('Ctrl Pts',(-48.3427993418052,-5.99820579736973,
-1.32203631868417));
#22947=CARTESIAN_POINT('Ctrl Pts',(-48.3443675175985,-5.97907559060215,
-1.12899680959845));
#22948=CARTESIAN_POINT('Ctrl Pts',(-48.3432090309159,-5.96099214798805,
-1.09680529223567));
#22949=CARTESIAN_POINT('Ctrl Pts',(-48.3361366892894,-5.9251130175414,-1.16128319669793));
#22950=CARTESIAN_POINT('Ctrl Pts',(-48.3366948692374,-5.9049506781467,-1.25795261852717));
#22951=CARTESIAN_POINT('Ctrl Pts',(-48.3348648315385,-5.8874628440639,-1.32263498783777));
#22952=CARTESIAN_POINT('Ctrl Pts',(-48.3345259496042,-5.99826554329983,
-1.67326463918611));
#22953=CARTESIAN_POINT('Ctrl Pts',(-48.3370692580606,-5.9777471823027,-1.47607399037158));
#22954=CARTESIAN_POINT('Ctrl Pts',(-48.3353565172368,-5.95954166014514,
-1.44603650619017));
#22955=CARTESIAN_POINT('Ctrl Pts',(-48.3269346991117,-5.9236034688997,-1.51473806899513));
#22956=CARTESIAN_POINT('Ctrl Pts',(-48.3256515256245,-5.90448098056108,
-1.61347711598476));
#22957=CARTESIAN_POINT('Ctrl Pts',(-48.3233989425165,-5.8874628440639,-1.67383952952183));
#22958=CARTESIAN_POINT('Ctrl Pts',(-48.3072618606229,-5.99418693015719,
-2.37587956040885));
#22959=CARTESIAN_POINT('Ctrl Pts',(-48.3087333779557,-5.97194742955361,
-2.2284105390898));
#22960=CARTESIAN_POINT('Ctrl Pts',(-48.3062335055684,-5.95413393118536,
-2.2069034605042));
#22961=CARTESIAN_POINT('Ctrl Pts',(-48.2977571519412,-5.91998502842413,
-2.25918163584876));
#22962=CARTESIAN_POINT('Ctrl Pts',(-48.295070923821,-5.90343694889075,-2.33296688978062));
#22963=CARTESIAN_POINT('Ctrl Pts',(-48.2928171719614,-5.8874628440639,-2.37608253350143));
#22964=CARTESIAN_POINT('Ctrl Pts',(-48.289645694342,-5.99381953117215,-2.72684648395123));
#22965=CARTESIAN_POINT('Ctrl Pts',(-48.2899913250448,-5.9708180255258,-2.60397205002056));
#22966=CARTESIAN_POINT('Ctrl Pts',(-48.2869150459205,-5.95257589046839,
-2.58894422957247));
#22967=CARTESIAN_POINT('Ctrl Pts',(-48.2785859525854,-5.91860436677926,
-2.63542225668577));
#22968=CARTESIAN_POINT('Ctrl Pts',(-48.2755338718776,-5.90286261480602,
-2.69692810424823));
#22969=CARTESIAN_POINT('Ctrl Pts',(-48.2737012896825,-5.8874628440639,-2.72712100634181));
#22970=CARTESIAN_POINT('Ctrl Pts',(-48.247215395667,-5.99717808806688,-3.4284040490082));
#22971=CARTESIAN_POINT('Ctrl Pts',(-48.2437182975085,-5.97321241327166,
-3.36074991074874));
#22972=CARTESIAN_POINT('Ctrl Pts',(-48.2392225168896,-5.95314193699471,
-3.35655320341621));
#22973=CARTESIAN_POINT('Ctrl Pts',(-48.2313449268639,-5.91737158402251,
-3.38631956483236));
#22974=CARTESIAN_POINT('Ctrl Pts',(-48.2285187244,-5.90176568155596,-3.42028263358126));
#22975=CARTESIAN_POINT('Ctrl Pts',(-48.2278104516838,-5.8874628440639,-3.42894804748533));
#22976=CARTESIAN_POINT('Ctrl Pts',(-48.2224012632728,-6.00090404394666,
-3.77899469052281));
#22977=CARTESIAN_POINT('Ctrl Pts',(-48.2161873228831,-5.97673620504532,
-3.74196626054616));
#22978=CARTESIAN_POINT('Ctrl Pts',(-48.2108487060109,-5.95526602423799,
-3.74211938381146));
#22979=CARTESIAN_POINT('Ctrl Pts',(-48.2032756172259,-5.91751946291063,
-3.76097220601848));
#22980=CARTESIAN_POINT('Ctrl Pts',(-48.2010411453131,-5.90124308239061,
-3.77967190496021));
#22981=CARTESIAN_POINT('Ctrl Pts',(-48.2010354948423,-5.8874628440639,-3.77973662633642));
#22982=CARTESIAN_POINT('Ctrl Pts',(-48.1943732865555,-6.00705144710501,
-4.12954958707863));
#22983=CARTESIAN_POINT('Ctrl Pts',(-48.1844415394016,-5.98314272027373,
-4.12944421263861));
#22984=CARTESIAN_POINT('Ctrl Pts',(-48.178454383799,-5.9599264156786,-4.12964628233308));
#22985=CARTESIAN_POINT('Ctrl Pts',(-48.1714459461707,-5.91876732373883,
-4.13010310894204));
#22986=CARTESIAN_POINT('Ctrl Pts',(-48.170424664145,-5.90082453639419,-4.13035786585651));
#22987=CARTESIAN_POINT('Ctrl Pts',(-48.170424664145,-5.8874628440639,-4.13035786585651));
#22988=CARTESIAN_POINT('Ctrl Pts',(-48.1943732865555,-6.00705144710502,
-4.12954958707862));
#22989=CARTESIAN_POINT('Ctrl Pts',(-48.1899403654158,-5.99638006180393,
-4.129502554409));
#22990=CARTESIAN_POINT('Ctrl Pts',(-48.1862445826294,-5.9858106003976,-4.1295124996258));
#22991=CARTESIAN_POINT('Ctrl Pts',(-48.1832154572887,-5.97555360442599,
-4.12955963932632));
#22992=CARTESIAN_POINT('Ctrl Pts',(-48.1799757201013,-5.96458345048952,
-4.12961005659982));
#22993=CARTESIAN_POINT('Ctrl Pts',(-48.1774980373401,-5.95397176603297,
-4.12970297530113));
#22994=CARTESIAN_POINT('Ctrl Pts',(-48.1756402817456,-5.94395259925277,
-4.12980930460529));
#22995=CARTESIAN_POINT('Ctrl Pts',(-48.1736701824512,-5.93332754531064,
-4.1299220639412));
#22996=CARTESIAN_POINT('Ctrl Pts',(-48.1723957131875,-5.92336957191581,
-4.13004977115199));
#22997=CARTESIAN_POINT('Ctrl Pts',(-48.1716028722098,-5.91431731008252,
-4.13015382200399));
#22998=CARTESIAN_POINT('Ctrl Pts',(-48.1707100966236,-5.90412404486024,
-4.1302709880726));
#22999=CARTESIAN_POINT('Ctrl Pts',(-48.170424664145,-5.89507967138156,-4.13035786585652));
#23000=CARTESIAN_POINT('Ctrl Pts',(-48.170424664145,-5.8874628440639,-4.13035786585652));
#23001=CARTESIAN_POINT('Ctrl Pts',(-48.3539734316379,-5.88746284406389,
0.0824317919393457));
#23002=CARTESIAN_POINT('Ctrl Pts',(-48.3539734316379,-5.90583775506839,
0.0824317919453202));
#23003=CARTESIAN_POINT('Ctrl Pts',(-48.3495242804801,-5.92795641804994,
0.0824317919456884));
#23004=CARTESIAN_POINT('Ctrl Pts',(-48.353628932479,-5.96223275463528,0.0824317919477567));
#23005=CARTESIAN_POINT('Ctrl Pts',(-48.3539872411712,-5.9853111687807,0.0824317919583475));
#23006=CARTESIAN_POINT('Ctrl Pts',(-48.353987706665,-6.00666333723547,0.0824317919588709));
#23007=CARTESIAN_POINT('Ctrl Pts',(-48.353987706665,-6.00666333723547,0.0824317919588709));
#23008=CARTESIAN_POINT('Ctrl Pts',(-48.3539875902919,-6.00132529512177,
0.433477096832907));
#23009=CARTESIAN_POINT('Ctrl Pts',(-48.3525301621497,-5.99973567328063,
0.784574339470114));
#23010=CARTESIAN_POINT('Ctrl Pts',(-48.3427993418055,-5.9982057973697,1.48689990262106));
#23011=CARTESIAN_POINT('Ctrl Pts',(-48.3345259496034,-5.9982655432999,1.8381282231348));
#23012=CARTESIAN_POINT('Ctrl Pts',(-48.3072618606178,-5.99418693015788,
2.540743144389));
#23013=CARTESIAN_POINT('Ctrl Pts',(-48.2896456943372,-5.99381953117289,
2.89171006791637));
#23014=CARTESIAN_POINT('Ctrl Pts',(-48.2472153956642,-5.99717808806743,
3.59326763292906));
#23015=CARTESIAN_POINT('Ctrl Pts',(-48.2224012632718,-6.00090404394695,
3.94385827441437));
#23016=CARTESIAN_POINT('Ctrl Pts',(-48.1943732865555,-6.00705144710499,
4.29441317095732));
#23017=CARTESIAN_POINT('Ctrl Pts',(-48.3539872411712,-5.9853111687807,0.0824317919583475));
#23018=CARTESIAN_POINT('Ctrl Pts',(-48.3539275501302,-5.98270666392057,
0.355621276231302));
#23019=CARTESIAN_POINT('Ctrl Pts',(-48.3527335277731,-5.98152768121041,
0.651206501710543));
#23020=CARTESIAN_POINT('Ctrl Pts',(-48.3443675175979,-5.97907559060113,
1.2938603935253));
#23021=CARTESIAN_POINT('Ctrl Pts',(-48.3370692580592,-5.97774718230175,
1.64093757430917));
#23022=CARTESIAN_POINT('Ctrl Pts',(-48.3087333779502,-5.97194742955337,
2.39327412306098));
#23023=CARTESIAN_POINT('Ctrl Pts',(-48.2899913250396,-5.97081802552575,
2.76883563397861));
#23024=CARTESIAN_POINT('Ctrl Pts',(-48.2437182975056,-5.97321241327176,
3.52561349466635));
#23025=CARTESIAN_POINT('Ctrl Pts',(-48.216187322882,-5.9767362050454,3.90682984443646));
#23026=CARTESIAN_POINT('Ctrl Pts',(-48.1844415394016,-5.98314272027372,
4.29430779651733));
#23027=CARTESIAN_POINT('Ctrl Pts',(-48.353628932479,-5.96223275463528,0.0824317919477567));
#23028=CARTESIAN_POINT('Ctrl Pts',(-48.3536632315906,-5.96240686080333,
0.338435236520447));
#23029=CARTESIAN_POINT('Ctrl Pts',(-48.3522992264079,-5.96239709811649,
0.625439688580834));
#23030=CARTESIAN_POINT('Ctrl Pts',(-48.3432090309151,-5.96099214798705,
1.26166887614506));
#23031=CARTESIAN_POINT('Ctrl Pts',(-48.3353565172354,-5.95954166014419,
1.61090009010881));
#23032=CARTESIAN_POINT('Ctrl Pts',(-48.306233505564,-5.95413393118495,2.37176704445063));
#23033=CARTESIAN_POINT('Ctrl Pts',(-48.2869150459164,-5.95257589046815,
2.75380781351011));
#23034=CARTESIAN_POINT('Ctrl Pts',(-48.2392225168873,-5.95314193699467,
3.52141678732466));
#23035=CARTESIAN_POINT('Ctrl Pts',(-48.21084870601,-5.95526602423798,3.90698296769951));
#23036=CARTESIAN_POINT('Ctrl Pts',(-48.178454383799,-5.95992641567858,4.29450986621179));
#23037=CARTESIAN_POINT('Ctrl Pts',(-48.3495242804801,-5.92795641804994,
0.0824317919456884));
#23038=CARTESIAN_POINT('Ctrl Pts',(-48.349501648034,-5.92787973562296,0.360237634072677));
#23039=CARTESIAN_POINT('Ctrl Pts',(-48.3473885441248,-5.92723732580272,
0.666464865124364));
#23040=CARTESIAN_POINT('Ctrl Pts',(-48.3361366892888,-5.92511301754091,
1.32614678059277));
#23041=CARTESIAN_POINT('Ctrl Pts',(-48.3269346991108,-5.92360346889921,
1.67960165289253));
#23042=CARTESIAN_POINT('Ctrl Pts',(-48.2977571519393,-5.91998502842383,
2.42404521975457));
#23043=CARTESIAN_POINT('Ctrl Pts',(-48.2785859525836,-5.91860436677904,
2.80028584058811));
#23044=CARTESIAN_POINT('Ctrl Pts',(-48.2313449268628,-5.91737158402241,
3.55118314872339));
#23045=CARTESIAN_POINT('Ctrl Pts',(-48.2032756172255,-5.91751946291058,
3.92583578990169));
#23046=CARTESIAN_POINT('Ctrl Pts',(-48.1714459461707,-5.91876732373881,
4.29496669282072));
#23047=CARTESIAN_POINT('Ctrl Pts',(-48.3539734316379,-5.90583775506839,
0.0824317919453202));
#23048=CARTESIAN_POINT('Ctrl Pts',(-48.3539734316379,-5.90583775506839,
0.399226071328185));
#23049=CARTESIAN_POINT('Ctrl Pts',(-48.350855770502,-5.90562906540036,0.733256854791239));
#23050=CARTESIAN_POINT('Ctrl Pts',(-48.3366948692371,-5.90495067814671,
1.42281620241652));
#23051=CARTESIAN_POINT('Ctrl Pts',(-48.3256515256241,-5.90448098056108,
1.77834069987334));
#23052=CARTESIAN_POINT('Ctrl Pts',(-48.2950709238206,-5.90343694889074,
2.49783047366717));
#23053=CARTESIAN_POINT('Ctrl Pts',(-48.2755338718772,-5.90286261480601,
2.86179168813353));
#23054=CARTESIAN_POINT('Ctrl Pts',(-48.2285187243997,-5.90176568155594,
3.58514621746359));
#23055=CARTESIAN_POINT('Ctrl Pts',(-48.201041145313,-5.90124308239059,3.94453548884082));
#23056=CARTESIAN_POINT('Ctrl Pts',(-48.170424664145,-5.90082453639417,4.29522144973519));
#23057=CARTESIAN_POINT('Ctrl Pts',(-48.3539734316379,-5.88746284406389,
0.0824317919393457));
#23058=CARTESIAN_POINT('Ctrl Pts',(-48.3539734316379,-5.88746284406389,
0.433719204637221));
#23059=CARTESIAN_POINT('Ctrl Pts',(-48.3501520759131,-5.88746284406389,
0.785006622606274));
#23060=CARTESIAN_POINT('Ctrl Pts',(-48.3348648315386,-5.88746284406389,
1.48749857171645));
#23061=CARTESIAN_POINT('Ctrl Pts',(-48.3233989425165,-5.88746284406389,
1.83870311340052));
#23062=CARTESIAN_POINT('Ctrl Pts',(-48.2928171719614,-5.88746284406389,
2.5409461173801));
#23063=CARTESIAN_POINT('Ctrl Pts',(-48.2737012896826,-5.88746284406389,
2.89198459022049));
#23064=CARTESIAN_POINT('Ctrl Pts',(-48.2278104516838,-5.88746284406388,
3.593811631364));
#23065=CARTESIAN_POINT('Ctrl Pts',(-48.2010354948423,-5.88746284406388,
3.94460021021509));
#23066=CARTESIAN_POINT('Ctrl Pts',(-48.170424664145,-5.88746284406388,4.29522144973519));
#23067=CARTESIAN_POINT('',(-48.1943732865555,-6.007051447105,4.29441317095728));
#23068=CARTESIAN_POINT('Origin',(-48.4830242383024,-5.88723161925863,4.32103607292913));
#23069=CARTESIAN_POINT('Ctrl Pts',(-48.1943732865555,-6.007051447105,4.29441317095728));
#23070=CARTESIAN_POINT('Ctrl Pts',(-48.2504292399881,-5.99475664078891,
3.59330337787145));
#23071=CARTESIAN_POINT('Ctrl Pts',(-48.293629816125,-5.99214762358688,2.89205060501605));
#23072=CARTESIAN_POINT('Ctrl Pts',(-48.3481579940962,-6.00030484987091,
1.48682076250771));
#23073=CARTESIAN_POINT('Ctrl Pts',(-48.3539874739188,-5.99598725300808,
0.784522401706929));
#23074=CARTESIAN_POINT('Ctrl Pts',(-48.353987706665,-6.00666333723547,0.0824317919588709));
#23075=CARTESIAN_POINT('Ctrl Pts',(48.5210408433891,-6.00666333723546,0.0824317919201338));
#23076=CARTESIAN_POINT('Ctrl Pts',(48.5210407270157,-6.00132529512171,-0.268613512953911));
#23077=CARTESIAN_POINT('Ctrl Pts',(48.5195832988733,-5.99973567328055,-0.61971075559112));
#23078=CARTESIAN_POINT('Ctrl Pts',(48.5098524785288,-5.99820579736961,-1.32203631874206));
#23079=CARTESIAN_POINT('Ctrl Pts',(48.5015790863268,-5.99826554329984,-1.67326463925579));
#23080=CARTESIAN_POINT('Ctrl Pts',(48.4743149973416,-5.99418693015786,-2.37587956050997));
#23081=CARTESIAN_POINT('Ctrl Pts',(48.4566988310611,-5.99381953117288,-2.72684648403734));
#23082=CARTESIAN_POINT('Ctrl Pts',(48.4142685323882,-5.99717808806743,-3.42840404905));
#23083=CARTESIAN_POINT('Ctrl Pts',(48.3894543999959,-6.00090404394696,-3.77899469053528));
#23084=CARTESIAN_POINT('Ctrl Pts',(48.3614264232796,-6.00705144710499,-4.12954958707821));
#23085=CARTESIAN_POINT('Ctrl Pts',(48.5210403778953,-5.9853111687807,0.0824317919206602));
#23086=CARTESIAN_POINT('Ctrl Pts',(48.5209806868542,-5.98270666392053,-0.190757692352299));
#23087=CARTESIAN_POINT('Ctrl Pts',(48.5197866644968,-5.98152768121036,-0.48634291783155));
#23088=CARTESIAN_POINT('Ctrl Pts',(48.5114206543214,-5.97907559060105,-1.12899680964633));
#23089=CARTESIAN_POINT('Ctrl Pts',(48.5041223947826,-5.97774718230167,-1.4760739904302));
#23090=CARTESIAN_POINT('Ctrl Pts',(48.475786514674,-5.97194742955333,-2.22841053918201));
#23091=CARTESIAN_POINT('Ctrl Pts',(48.4570444617636,-5.97081802552572,-2.60397205009964));
#23092=CARTESIAN_POINT('Ctrl Pts',(48.4107714342297,-5.97321241327177,-3.36074991078733));
#23093=CARTESIAN_POINT('Ctrl Pts',(48.3832404596062,-5.97673620504541,-3.7419662605574));
#23094=CARTESIAN_POINT('Ctrl Pts',(48.3514946761257,-5.98314272027372,-4.12944421263819));
#23095=CARTESIAN_POINT('Ctrl Pts',(48.5206820692032,-5.96223275463527,0.0824317919312382));
#23096=CARTESIAN_POINT('Ctrl Pts',(48.5207163683146,-5.96240686080331,-0.173571652641453));
#23097=CARTESIAN_POINT('Ctrl Pts',(48.5193523631318,-5.96239709811646,-0.46057610470184));
#23098=CARTESIAN_POINT('Ctrl Pts',(48.5102621676387,-5.96099214798699,-1.09680529226608));
#23099=CARTESIAN_POINT('Ctrl Pts',(48.5024096539591,-5.95954166014412,-1.44603650622985));
#23100=CARTESIAN_POINT('Ctrl Pts',(48.473286642288,-5.95413393118491,-2.20690346057166));
#23101=CARTESIAN_POINT('Ctrl Pts',(48.4539681826404,-5.95257589046813,-2.58894422963113));
#23102=CARTESIAN_POINT('Ctrl Pts',(48.4062756536114,-5.95314193699467,-3.35655320344563));
#23103=CARTESIAN_POINT('Ctrl Pts',(48.3779018427341,-5.95526602423799,-3.74211938382045));
#23104=CARTESIAN_POINT('Ctrl Pts',(48.3455075205231,-5.95992641567859,-4.12964628233266));
#23105=CARTESIAN_POINT('Ctrl Pts',(48.5165774172042,-5.92795641804992,0.0824317919333195));
#23106=CARTESIAN_POINT('Ctrl Pts',(48.516554784758,-5.92787973562295,-0.195374050193665));
#23107=CARTESIAN_POINT('Ctrl Pts',(48.5144416808488,-5.9272373258027,-0.501601281245333));
#23108=CARTESIAN_POINT('Ctrl Pts',(48.5031898260128,-5.92511301754087,-1.16128319671373));
#23109=CARTESIAN_POINT('Ctrl Pts',(48.4939878358348,-5.92360346889917,-1.51473806901351));
#23110=CARTESIAN_POINT('Ctrl Pts',(48.4648102886634,-5.9199850284238,-2.25918163587555));
#23111=CARTESIAN_POINT('Ctrl Pts',(48.4456390893077,-5.91860436677902,-2.63542225670908));
#23112=CARTESIAN_POINT('Ctrl Pts',(48.3983980635869,-5.91737158402241,-3.38631956484433));
#23113=CARTESIAN_POINT('Ctrl Pts',(48.3703287539496,-5.91751946291058,-3.76097220602262));
#23114=CARTESIAN_POINT('Ctrl Pts',(48.3384990828948,-5.91876732373882,-4.13010310894162));
#23115=CARTESIAN_POINT('Ctrl Pts',(48.521026568362,-5.90583775506839,0.0824317919337002));
#23116=CARTESIAN_POINT('Ctrl Pts',(48.521026568362,-5.90583775506839,-0.23436248744916));
#23117=CARTESIAN_POINT('Ctrl Pts',(48.5179089072261,-5.90562906540036,-0.568393270912183));
#23118=CARTESIAN_POINT('Ctrl Pts',(48.5037480059612,-5.90495067814671,-1.25795261853744));
#23119=CARTESIAN_POINT('Ctrl Pts',(48.4927046623482,-5.90448098056109,-1.61347711599428));
#23120=CARTESIAN_POINT('Ctrl Pts',(48.4621240605447,-5.90343694889074,-2.3329668897881));
#23121=CARTESIAN_POINT('Ctrl Pts',(48.4425870086013,-5.90286261480601,-2.69692810425446));
#23122=CARTESIAN_POINT('Ctrl Pts',(48.3955718611238,-5.90176568155594,-3.4202826335845));
#23123=CARTESIAN_POINT('Ctrl Pts',(48.3680942820371,-5.90124308239059,-3.77967190496174));
#23124=CARTESIAN_POINT('Ctrl Pts',(48.3374778008691,-5.90082453639417,-4.1303578658561));
#23125=CARTESIAN_POINT('Ctrl Pts',(48.521026568362,-5.88746284406389,0.082431791939678));
#23126=CARTESIAN_POINT('Ctrl Pts',(48.521026568362,-5.88746284406389,-0.268855620758191));
#23127=CARTESIAN_POINT('Ctrl Pts',(48.5172052126372,-5.88746284406389,-0.620143038727212));
#23128=CARTESIAN_POINT('Ctrl Pts',(48.5019179682627,-5.88746284406389,-1.32263498783737));
#23129=CARTESIAN_POINT('Ctrl Pts',(48.4904520792406,-5.88746284406389,-1.67383952952145));
#23130=CARTESIAN_POINT('Ctrl Pts',(48.4598703086855,-5.88746284406389,-2.37608253350103));
#23131=CARTESIAN_POINT('Ctrl Pts',(48.4407544264067,-5.88746284406388,-2.7271210063414));
#23132=CARTESIAN_POINT('Ctrl Pts',(48.3948635884079,-5.88746284406388,-3.42894804748491));
#23133=CARTESIAN_POINT('Ctrl Pts',(48.3680886315664,-5.88746284406389,-3.77973662633601));
#23134=CARTESIAN_POINT('Ctrl Pts',(48.3374778008691,-5.88746284406389,-4.1303578658561));
#23135=CARTESIAN_POINT('',(48.5210408433891,-6.00666333723546,0.0824317919201338));
#23136=CARTESIAN_POINT('Ctrl Pts',(48.5210265683621,-5.88746284406389,0.082431791939678));
#23137=CARTESIAN_POINT('Ctrl Pts',(48.521026568362,-5.90583775506839,0.0824317919337002));
#23138=CARTESIAN_POINT('Ctrl Pts',(48.5165774172042,-5.92795641804992,0.0824317919333195));
#23139=CARTESIAN_POINT('Ctrl Pts',(48.5206820692032,-5.96223275463527,0.0824317919312382));
#23140=CARTESIAN_POINT('Ctrl Pts',(48.5210403778953,-5.9853111687807,0.0824317919206602));
#23141=CARTESIAN_POINT('Ctrl Pts',(48.5210408433891,-6.00666333723546,0.0824317919201338));
#23142=CARTESIAN_POINT('',(48.3614264232796,-6.00705144710501,-4.12954958707822));
#23143=CARTESIAN_POINT('Ctrl Pts',(48.3374778008691,-5.88746284406389,-4.1303578658561));
#23144=CARTESIAN_POINT('Ctrl Pts',(48.3374778008691,-5.89466520940775,-4.13035786585611));
#23145=CARTESIAN_POINT('Ctrl Pts',(48.3377330767287,-5.90314351486559,-4.13028019061201));
#23146=CARTESIAN_POINT('Ctrl Pts',(48.3385156183452,-5.91266355145352,-4.13017267066886));
#23147=CARTESIAN_POINT('Ctrl Pts',(48.3392385198517,-5.92145803425844,-4.13007334517968));
#23148=CARTESIAN_POINT('Ctrl Pts',(48.3404137627567,-5.93114147445238,-4.12994875887528));
#23149=CARTESIAN_POINT('Ctrl Pts',(48.342246929742,-5.94148964487018,-4.12983582017077));
#23150=CARTESIAN_POINT('Ctrl Pts',(48.344019574647,-5.95149617003371,-4.12972661014203));
#23151=CARTESIAN_POINT('Ctrl Pts',(48.3464089871042,-5.96212379582484,-4.12962842768266));
#23152=CARTESIAN_POINT('Ctrl Pts',(48.3495648080625,-5.97313476325663,-4.12957145846139));
#23153=CARTESIAN_POINT('Ctrl Pts',(48.3524876731452,-5.98333292489419,-4.12951869458479));
#23154=CARTESIAN_POINT('Ctrl Pts',(48.3560684105317,-5.99385899411776,-4.12950132106585));
#23155=CARTESIAN_POINT('Ctrl Pts',(48.3603813000572,-6.00450404015464,-4.12953941874855));
#23156=CARTESIAN_POINT('Ctrl Pts',(48.3607250425592,-6.005352463175,-4.12954245517985));
#23157=CARTESIAN_POINT('Ctrl Pts',(48.3610734091784,-6.00620163512511,-4.12954584164827));
#23158=CARTESIAN_POINT('Ctrl Pts',(48.3614264232796,-6.00705144710501,-4.12954958707822));
#23159=CARTESIAN_POINT('Ctrl Pts',(48.3614264232796,-6.00705144710501,-4.12954958707822));
#23160=CARTESIAN_POINT('Ctrl Pts',(48.4174823767122,-5.99475664078892,-3.42843979399236));
#23161=CARTESIAN_POINT('Ctrl Pts',(48.460682952849,-5.99214762358688,-2.72718702113706));
#23162=CARTESIAN_POINT('Ctrl Pts',(48.5152111308193,-6.00030484987083,-1.3219571786287));
#23163=CARTESIAN_POINT('Ctrl Pts',(48.5210406106424,-5.99598725300796,-0.619658817827956));
#23164=CARTESIAN_POINT('Ctrl Pts',(48.5210408433891,-6.00666333723546,0.0824317919201338));
#23165=CARTESIAN_POINT('Ctrl Pts',(48.5210408433891,-6.00666333723546,0.0824317919201338));
#23166=CARTESIAN_POINT('Ctrl Pts',(48.5210409597626,-6.01200137934909,-0.268613512954174));
#23167=CARTESIAN_POINT('Ctrl Pts',(48.5195837679427,-6.02125184123585,-0.619482841813776));
#23168=CARTESIAN_POINT('Ctrl Pts',(48.5162561594161,-6.04818290219915,-1.32089560055031));
#23169=CARTESIAN_POINT('Ctrl Pts',(48.5143857427094,-6.06586350127569,-1.67143903042725));
#23170=CARTESIAN_POINT('Ctrl Pts',(48.5119067425097,-6.1324584507553,-2.72261955115417));
#23171=CARTESIAN_POINT('Ctrl Pts',(48.5072128795234,-6.17306838545284,-3.42489190632274));
#23172=CARTESIAN_POINT('Ctrl Pts',(48.4970122186805,-6.20946968450871,-4.12660735523292));
#23173=CARTESIAN_POINT('Ctrl Pts',(48.5210407270157,-6.00132529512171,-0.268613512953911));
#23174=CARTESIAN_POINT('Ctrl Pts',(48.5200991113388,-6.00879525432309,-0.541629932914882));
#23175=CARTESIAN_POINT('Ctrl Pts',(48.5183837318925,-6.01828947675668,-0.832372601189314));
#23176=CARTESIAN_POINT('Ctrl Pts',(48.5144994209904,-6.04432658407318,-1.44625764085795));
#23177=CARTESIAN_POINT('Ctrl Pts',(48.5123333385556,-6.06089216512316,-1.76939839268532));
#23178=CARTESIAN_POINT('Ctrl Pts',(48.508693911101,-6.12571278894254,-2.78284525810139));
#23179=CARTESIAN_POINT('Ctrl Pts',(48.5032144670184,-6.16367997403221,-3.46086303049164));
#23180=CARTESIAN_POINT('Ctrl Pts',(48.4920141354583,-6.19747947412215,-4.12726570254766));
#23181=CARTESIAN_POINT('Ctrl Pts',(48.5195832988733,-5.99973567328055,-0.61971075559112));
#23182=CARTESIAN_POINT('Ctrl Pts',(48.5180114541292,-6.00835114797888,-0.832717795223906));
#23183=CARTESIAN_POINT('Ctrl Pts',(48.5159956580433,-6.01789996842705,-1.077403160991));
#23184=CARTESIAN_POINT('Ctrl Pts',(48.5114095528202,-6.04289085428948,-1.62044191129696));
#23185=CARTESIAN_POINT('Ctrl Pts',(48.5088435172146,-6.05836696395436,-1.91879286648555));
#23186=CARTESIAN_POINT('Ctrl Pts',(48.5036610021237,-6.11975101512501,-2.8798211782362));
#23187=CARTESIAN_POINT('Ctrl Pts',(48.497322596291,-6.15479195325803,-3.52283172309684));
#23188=CARTESIAN_POINT('Ctrl Pts',(48.4858839393065,-6.18527410484421,-4.12793443867102));
#23189=CARTESIAN_POINT('Ctrl Pts',(48.5098524785288,-5.99820579736961,-1.32203631874206));
#23190=CARTESIAN_POINT('Ctrl Pts',(48.5081357594357,-6.0082917350608,-1.44781988536826));
#23191=CARTESIAN_POINT('Ctrl Pts',(48.5060961369459,-6.0181420651212,-1.62174845929102));
#23192=CARTESIAN_POINT('Ctrl Pts',(48.5010454692996,-6.04173521008612,-2.04438575580717));
#23193=CARTESIAN_POINT('Ctrl Pts',(48.4980397660576,-6.05552058030391,-2.29309144171275));
#23194=CARTESIAN_POINT('Ctrl Pts',(48.4906361945903,-6.10935599904101,-3.11912188389239));
#23195=CARTESIAN_POINT('Ctrl Pts',(48.4830998622531,-6.13882811018934,-3.66842757888082));
#23196=CARTESIAN_POINT('Ctrl Pts',(48.4724837048732,-6.1620572511385,-4.12937020770049));
#23197=CARTESIAN_POINT('Ctrl Pts',(48.5015790863268,-5.99826554329984,-1.67326463925579));
#23198=CARTESIAN_POINT('Ctrl Pts',(48.5003285876348,-6.00864450579842,-1.77183914814116));
#23199=CARTESIAN_POINT('Ctrl Pts',(48.498555988222,-6.01872578611223,-1.92107075019569));
#23200=CARTESIAN_POINT('Ctrl Pts',(48.4937353771045,-6.0419554406255,-2.29415477038631));
#23201=CARTESIAN_POINT('Ctrl Pts',(48.4906923511867,-6.05514353311736,-2.51800435428045));
#23202=CARTESIAN_POINT('Ctrl Pts',(48.4826251617171,-6.10489083408601,-3.26145170435135));
#23203=CARTESIAN_POINT('Ctrl Pts',(48.4747689989427,-6.13175228789483,-3.75205474205961));
#23204=CARTESIAN_POINT('Ctrl Pts',(48.4652136665916,-6.15104576671075,-4.13013724060659));
#23205=CARTESIAN_POINT('Ctrl Pts',(48.460682952849,-5.99214762358688,-2.72718702113706));
#23206=CARTESIAN_POINT('Ctrl Pts',(48.4602502315003,-6.00381665756758,-2.78846829178684));
#23207=CARTESIAN_POINT('Ctrl Pts',(48.4596398458504,-6.01569196513298,-2.88547763641065));
#23208=CARTESIAN_POINT('Ctrl Pts',(48.457639336462,-6.04033961885395,-3.12373338298816));
#23209=CARTESIAN_POINT('Ctrl Pts',(48.4562520617447,-6.05313466117661,-3.26497816537503));
#23210=CARTESIAN_POINT('Ctrl Pts',(48.4521822008009,-6.09364276617912,-3.7142437081182));
#23211=CARTESIAN_POINT('Ctrl Pts',(48.4481398059304,-6.11446024451103,-3.98991893800781));
#23212=CARTESIAN_POINT('Ctrl Pts',(48.4433803641459,-6.12223844465216,-4.13270206324732));
#23213=CARTESIAN_POINT('Ctrl Pts',(48.4174823767122,-5.99475664078892,-3.42843979399236));
#23214=CARTESIAN_POINT('Ctrl Pts',(48.418730443525,-6.00697011627484,-3.46541553675024));
#23215=CARTESIAN_POINT('Ctrl Pts',(48.4200748651391,-6.02014444454773,-3.52759295133352));
#23216=CARTESIAN_POINT('Ctrl Pts',(48.422702883804,-6.0459458820395,-3.67275508618324));
#23217=CARTESIAN_POINT('Ctrl Pts',(48.4239864808546,-6.05857299125839,-3.75573980644969));
#23218=CARTESIAN_POINT('Ctrl Pts',(48.4273657339121,-6.09193010339208,-3.99151086882235));
#23219=CARTESIAN_POINT('Ctrl Pts',(48.4289898518245,-6.10813589078396,-4.13111411250188));
#23220=CARTESIAN_POINT('Ctrl Pts',(48.4289711156128,-6.10843369230009,-4.13475573974202));
#23221=CARTESIAN_POINT('Ctrl Pts',(48.3614264232796,-6.00705144710499,-4.12954958707821));
#23222=CARTESIAN_POINT('Ctrl Pts',(48.3663922968565,-6.01900581052063,-4.12960227429821));
#23223=CARTESIAN_POINT('Ctrl Pts',(48.3730775094482,-6.03128117156189,-4.12973535553811));
#23224=CARTESIAN_POINT('Ctrl Pts',(48.3875464536895,-6.05467770199134,-4.13029598569406));
#23225=CARTESIAN_POINT('Ctrl Pts',(48.395330185339,-6.06579887137953,-4.13072353461011));
#23226=CARTESIAN_POINT('Ctrl Pts',(48.4168189204169,-6.09473681170807,-4.13264840232708));
#23227=CARTESIAN_POINT('Ctrl Pts',(48.4286614639744,-6.10812801481235,-4.1347879420968));
#23228=CARTESIAN_POINT('Ctrl Pts',(48.4286600918172,-6.10843371318468,-4.13831849503711));
#23229=CARTESIAN_POINT('Ctrl Pts',(48.3614264232796,-6.00705144710501,-4.12954958707822));
#23230=CARTESIAN_POINT('Ctrl Pts',(48.3812898236076,-6.05486867452979,-4.1297603349611));
#23231=CARTESIAN_POINT('Ctrl Pts',(48.4286623878632,-6.1078218153655,-4.13125737499063));
#23232=CARTESIAN_POINT('Ctrl Pts',(48.428660091853,-6.1084337045031,-4.1383183948133));
#23233=CARTESIAN_POINT('',(48.4970119975844,-6.2094697762355,-4.1266073472585));
#23234=CARTESIAN_POINT('Ctrl Pts',(48.4286601057169,-6.10843371319293,-4.13831833592522));
#23235=CARTESIAN_POINT('Ctrl Pts',(48.4289715446248,-6.1084341033154,-4.13475567859721));
#23236=CARTESIAN_POINT('Ctrl Pts',(48.4433805808296,-6.12223873054926,-4.13270203779284));
#23237=CARTESIAN_POINT('Ctrl Pts',(48.4724914340735,-6.16064820739694,-4.12928229972635));
#23238=CARTESIAN_POINT('Ctrl Pts',(48.4870160522361,-6.18548926373558,-4.12792404986242));
#23239=CARTESIAN_POINT('Ctrl Pts',(48.4970122186805,-6.2094696845087,-4.12660735523292));
#23240=CARTESIAN_POINT('Ctrl Pts',(48.4970122186805,-6.2094696845087,-4.12660735523292));
#23241=CARTESIAN_POINT('Ctrl Pts',(48.5072128795234,-6.17306838545284,-3.42489190632274));
#23242=CARTESIAN_POINT('Ctrl Pts',(48.5119067425097,-6.1324584507553,-2.72261955115417));
#23243=CARTESIAN_POINT('Ctrl Pts',(48.5152120761093,-6.04366518478249,-1.32104552351828));
#23244=CARTESIAN_POINT('Ctrl Pts',(48.5210410761362,-6.01733942146272,-0.619658817828478));
#23245=CARTESIAN_POINT('Ctrl Pts',(48.5210408433891,-6.00666333723546,0.0824317919201338));
#23246=CARTESIAN_POINT('Ctrl Pts',(48.5210408433891,-6.00666333723546,0.0824317919201338));
#23247=CARTESIAN_POINT('Ctrl Pts',(48.5210413088828,-6.02801550569023,0.0824317919196075));
#23248=CARTESIAN_POINT('Ctrl Pts',(48.5206840668932,-6.05386667280683,0.0824317919099577));
#23249=CARTESIAN_POINT('Ctrl Pts',(48.5224494671407,-6.10694539169997,0.0824317919266097));
#23250=CARTESIAN_POINT('Ctrl Pts',(48.521026568362,-6.1214884958821,0.0824317919326452));
#23251=CARTESIAN_POINT('Ctrl Pts',(48.521026568362,-6.14692278878552,0.0824317919396692));
#23252=CARTESIAN_POINT('Ctrl Pts',(48.5210409597626,-6.01200137934909,-0.268613512954174));
#23253=CARTESIAN_POINT('Ctrl Pts',(48.5209817377068,-6.03090918789886,-0.190411563724606));
#23254=CARTESIAN_POINT('Ctrl Pts',(48.5206817360457,-6.05382055712372,-0.190198224106269));
#23255=CARTESIAN_POINT('Ctrl Pts',(48.5224506909739,-6.10695822375808,-0.228911446012096));
#23256=CARTESIAN_POINT('Ctrl Pts',(48.521026568362,-6.12148849588209,-0.267838007555758));
#23257=CARTESIAN_POINT('Ctrl Pts',(48.521026568362,-6.14692278878552,-0.267915860671833));
#23258=CARTESIAN_POINT('Ctrl Pts',(48.5195837679427,-6.02125184123585,-0.619482841813776));
#23259=CARTESIAN_POINT('Ctrl Pts',(48.5206699839277,-6.03698783585497,-0.48601517812655));
#23260=CARTESIAN_POINT('Ctrl Pts',(48.5207850195095,-6.05830967273443,-0.4856519792755));
#23261=CARTESIAN_POINT('Ctrl Pts',(48.5225859377164,-6.11145963930962,-0.551717780117302));
#23262=CARTESIAN_POINT('Ctrl Pts',(48.5210265683614,-6.12687873284895,-0.618146779828));
#23263=CARTESIAN_POINT('Ctrl Pts',(48.5210265683614,-6.15072449281718,-0.618263513283336));
#23264=CARTESIAN_POINT('Ctrl Pts',(48.5162561594161,-6.04818290219915,-1.32089560055031));
#23265=CARTESIAN_POINT('Ctrl Pts',(48.5194060549133,-6.05935112779908,-1.12857563447696));
#23266=CARTESIAN_POINT('Ctrl Pts',(48.5204407823906,-6.07865710025979,-1.12801608352039));
#23267=CARTESIAN_POINT('Ctrl Pts',(48.5225314340435,-6.12977840933563,-1.22311169348749));
#23268=CARTESIAN_POINT('Ctrl Pts',(48.5210265683597,-6.1464337020842,-1.31876685442492));
#23269=CARTESIAN_POINT('Ctrl Pts',(48.5210265683599,-6.16593130894384,-1.31887631215337));
#23270=CARTESIAN_POINT('Ctrl Pts',(48.5143857427094,-6.06586350127569,-1.67143903042725));
#23271=CARTESIAN_POINT('Ctrl Pts',(48.5184689188876,-6.07568031733621,-1.47552932160173));
#23272=CARTESIAN_POINT('Ctrl Pts',(48.5200083010177,-6.09455995772354,-1.47492327777235));
#23273=CARTESIAN_POINT('Ctrl Pts',(48.5223492032329,-6.14361803658467,-1.57169769534062));
#23274=CARTESIAN_POINT('Ctrl Pts',(48.5210265683587,-6.16059843435258,-1.6690781567496));
#23275=CARTESIAN_POINT('Ctrl Pts',(48.5210265683589,-6.17733642103885,-1.6691414584119));
#23276=CARTESIAN_POINT('Ctrl Pts',(48.5119067425097,-6.1324584507553,-2.72261955115417));
#23277=CARTESIAN_POINT('Ctrl Pts',(48.5182994308559,-6.14582978514634,-2.60217795499973));
#23278=CARTESIAN_POINT('Ctrl Pts',(48.5205482384313,-6.16286923349053,-2.60155209044579));
#23279=CARTESIAN_POINT('Ctrl Pts',(48.5223287689013,-6.19966838879307,-2.6604144807085));
#23280=CARTESIAN_POINT('Ctrl Pts',(48.5210265683567,-6.21324540616173,-2.71990273552945));
#23281=CARTESIAN_POINT('Ctrl Pts',(48.521026568357,-6.22295686941884,-2.71968937812859));
#23282=CARTESIAN_POINT('Ctrl Pts',(48.5072128795234,-6.17306838545284,-3.42489190632274));
#23283=CARTESIAN_POINT('Ctrl Pts',(48.5152097045332,-6.19184520829409,-3.35294965798495));
#23284=CARTESIAN_POINT('Ctrl Pts',(48.5186631267415,-6.21237399283441,-3.35194886516752));
#23285=CARTESIAN_POINT('Ctrl Pts',(48.5215715586532,-6.2473915990406,-3.38562737807026));
#23286=CARTESIAN_POINT('Ctrl Pts',(48.5210265683567,-6.26188042070647,-3.42030668379043));
#23287=CARTESIAN_POINT('Ctrl Pts',(48.521026568357,-6.26857731779883,-3.41972463252783));
#23288=CARTESIAN_POINT('Ctrl Pts',(48.4970122186805,-6.20946968450871,-4.12660735523292));
#23289=CARTESIAN_POINT('Ctrl Pts',(48.507008385125,-6.23345010528183,-4.12529066060343));
#23290=CARTESIAN_POINT('Ctrl Pts',(48.5130119725454,-6.25674581560881,-4.1239954623018));
#23291=CARTESIAN_POINT('Ctrl Pts',(48.5200210641639,-6.29803503999843,-4.12148173153252));
#23292=CARTESIAN_POINT('Ctrl Pts',(48.5210265683621,-6.31602855406107,-4.12026319906486));
#23293=CARTESIAN_POINT('Ctrl Pts',(48.5210265683621,-6.3294045823055,-4.1190998361033));
#23294=CARTESIAN_POINT('Ctrl Pts',(48.4970115553921,-6.20946995968909,-4.12660733130967));
#23295=CARTESIAN_POINT('Ctrl Pts',(48.5011279178742,-6.21934480701995,-4.12606513380734));
#23296=CARTESIAN_POINT('Ctrl Pts',(48.5046178396385,-6.22915570483188,-4.12552208566969));
#23297=CARTESIAN_POINT('Ctrl Pts',(48.5075257383419,-6.2387140812738,-4.12498377433694));
#23298=CARTESIAN_POINT('Ctrl Pts',(48.5106110815886,-6.24885572484965,-4.1244126144017));
#23299=CARTESIAN_POINT('Ctrl Pts',(48.5130419072292,-6.25871184341287,-4.12384689551928));
#23300=CARTESIAN_POINT('Ctrl Pts',(48.5149245180109,-6.26808527594666,-4.12329088894307));
#23301=CARTESIAN_POINT('Ctrl Pts',(48.5168931544651,-6.2778870263491,-4.12270947571344));
#23302=CARTESIAN_POINT('Ctrl Pts',(48.5182638775358,-6.2871603096056,-4.12213874113348));
#23303=CARTESIAN_POINT('Ctrl Pts',(48.5191966343059,-6.29572520171223,-4.12157964242301));
#23304=CARTESIAN_POINT('Ctrl Pts',(48.520210635235,-6.30503610551135,-4.12097184558885));
#23305=CARTESIAN_POINT('Ctrl Pts',(48.5207092754634,-6.31350977078186,-4.1203778077907));
#23306=CARTESIAN_POINT('Ctrl Pts',(48.520912047233,-6.32097498479566,-4.11979356060943));
#23307=CARTESIAN_POINT('Ctrl Pts',(48.5209927725262,-6.32394695466906,-4.11956096647104));
#23308=CARTESIAN_POINT('Ctrl Pts',(48.5210265564937,-6.32675971428292,-4.11932987011934));
#23309=CARTESIAN_POINT('Ctrl Pts',(48.5210265683589,-6.32940458230548,-4.1190998361033));
#23310=CARTESIAN_POINT('Ctrl Pts',(48.5210265683621,-6.14692278878556,0.0824317919396692));
#23311=CARTESIAN_POINT('Ctrl Pts',(48.521026568362,-6.1214884958821,0.0824317919326452));
#23312=CARTESIAN_POINT('Ctrl Pts',(48.5224494671407,-6.10694539169997,0.0824317919266097));
#23313=CARTESIAN_POINT('Ctrl Pts',(48.5206840668932,-6.05386667280683,0.0824317919099577));
#23314=CARTESIAN_POINT('Ctrl Pts',(48.5210413088828,-6.02801550569023,0.0824317919196075));
#23315=CARTESIAN_POINT('Ctrl Pts',(48.5210408433891,-6.00666333723546,0.0824317919201338));
#23316=CARTESIAN_POINT('Ctrl Pts',(48.5210408433891,-6.00666333723546,0.0824317919201338));
#23317=CARTESIAN_POINT('Ctrl Pts',(48.5210409597624,-6.01200137934921,0.433477096794178));
#23318=CARTESIAN_POINT('Ctrl Pts',(48.519583767942,-6.02125184123474,0.784346425646489));
#23319=CARTESIAN_POINT('Ctrl Pts',(48.5162561594143,-6.04818290219394,1.48575918435436));
#23320=CARTESIAN_POINT('Ctrl Pts',(48.514385742707,-6.06586350126761,1.83630261420992));
#23321=CARTESIAN_POINT('Ctrl Pts',(48.5119067425057,-6.13245845073776,2.88748313485153));
#23322=CARTESIAN_POINT('Ctrl Pts',(48.5072128795205,-6.17306838542385,3.58975548987207));
#23323=CARTESIAN_POINT('Ctrl Pts',(48.4970122186805,-6.20946968446903,4.29147093865584));
#23324=CARTESIAN_POINT('Ctrl Pts',(48.5210413088828,-6.02801550569023,0.0824317919196075));
#23325=CARTESIAN_POINT('Ctrl Pts',(48.5209817377062,-6.03090918789795,0.355275147562284));
#23326=CARTESIAN_POINT('Ctrl Pts',(48.520669983927,-6.03698783585279,0.650878761955212));
#23327=CARTESIAN_POINT('Ctrl Pts',(48.5194060549125,-6.05935112779395,1.29343921827952));
#23328=CARTESIAN_POINT('Ctrl Pts',(48.5184689188868,-6.07568031732942,1.64039290538721));
#23329=CARTESIAN_POINT('Ctrl Pts',(48.5182994308548,-6.14582978513442,2.76704153873217));
#23330=CARTESIAN_POINT('Ctrl Pts',(48.5152097045334,-6.19184520827617,3.51781324162618));
#23331=CARTESIAN_POINT('Ctrl Pts',(48.5070083851249,-6.23345010526291,4.29015424426622));
#23332=CARTESIAN_POINT('Ctrl Pts',(48.5206840668932,-6.05386667280683,0.0824317919099577));
#23333=CARTESIAN_POINT('Ctrl Pts',(48.5206817360452,-6.05382055712278,0.355061807926185));
#23334=CARTESIAN_POINT('Ctrl Pts',(48.5207850195089,-6.05830967273254,0.650515563090774));
#23335=CARTESIAN_POINT('Ctrl Pts',(48.5204407823903,-6.07865710025595,1.29287966732272));
#23336=CARTESIAN_POINT('Ctrl Pts',(48.5200083010175,-6.09455995771876,1.63978686156639));
#23337=CARTESIAN_POINT('Ctrl Pts',(48.5205482384312,-6.162869233483,2.76641567421791));
#23338=CARTESIAN_POINT('Ctrl Pts',(48.5186631267424,-6.21237399282373,3.51681244889125));
#23339=CARTESIAN_POINT('Ctrl Pts',(48.5130119725453,-6.25674581559981,4.2888590460787));
#23340=CARTESIAN_POINT('Ctrl Pts',(48.5224494671407,-6.10694539169997,0.0824317919266097));
#23341=CARTESIAN_POINT('Ctrl Pts',(48.5224506909736,-6.1069582237576,0.393775029865316));
#23342=CARTESIAN_POINT('Ctrl Pts',(48.5225859377162,-6.11145963930881,0.716581363969174));
#23343=CARTESIAN_POINT('Ctrl Pts',(48.5225314340435,-6.12977840933438,1.3879752773367));
#23344=CARTESIAN_POINT('Ctrl Pts',(48.522349203233,-6.14361803658331,1.73656127918852));
#23345=CARTESIAN_POINT('Ctrl Pts',(48.5223287689018,-6.1996683887915,2.82527806455661));
#23346=CARTESIAN_POINT('Ctrl Pts',(48.5215715586541,-6.24739159903889,3.55049096191302));
#23347=CARTESIAN_POINT('Ctrl Pts',(48.5200210641639,-6.29803503999888,4.28634531541769));
#23348=CARTESIAN_POINT('Ctrl Pts',(48.521026568362,-6.1214884958821,0.0824317919326452));
#23349=CARTESIAN_POINT('Ctrl Pts',(48.521026568362,-6.1214884958821,0.432701591421048));
#23350=CARTESIAN_POINT('Ctrl Pts',(48.5210265683614,-6.12687873284896,0.783010363694165));
#23351=CARTESIAN_POINT('Ctrl Pts',(48.5210265683597,-6.14643370208421,1.48363043829371));
#23352=CARTESIAN_POINT('Ctrl Pts',(48.5210265683587,-6.1605984343526,1.83394174062015));
#23353=CARTESIAN_POINT('Ctrl Pts',(48.5210265683567,-6.21324540616174,2.88476631940526));
#23354=CARTESIAN_POINT('Ctrl Pts',(48.5210265683567,-6.26188042070648,3.58517026766974));
#23355=CARTESIAN_POINT('Ctrl Pts',(48.521026568362,-6.31602855406106,4.2851267829442));
#23356=CARTESIAN_POINT('Ctrl Pts',(48.521026568362,-6.14692278878552,0.0824317919396692));
#23357=CARTESIAN_POINT('Ctrl Pts',(48.521026568362,-6.14692278878553,0.432779444551172));
#23358=CARTESIAN_POINT('Ctrl Pts',(48.5210265683614,-6.15072449281719,0.783127097162674));
#23359=CARTESIAN_POINT('Ctrl Pts',(48.5210265683598,-6.16593130894386,1.48373989603271));
#23360=CARTESIAN_POINT('Ctrl Pts',(48.5210265683589,-6.17733642103886,1.83400504229124));
#23361=CARTESIAN_POINT('Ctrl Pts',(48.521026568357,-6.22295686941886,2.88455296200792));
#23362=CARTESIAN_POINT('Ctrl Pts',(48.521026568357,-6.26857731779886,3.58458821640716));
#23363=CARTESIAN_POINT('Ctrl Pts',(48.521026568362,-6.32940458230552,4.28396341998264));
#23364=CARTESIAN_POINT('',(48.4970120083066,-6.20946977174738,4.29147093106825));
#23365=CARTESIAN_POINT('Ctrl Pts',(48.5210265683593,-6.32940458230551,4.28396341998264));
#23366=CARTESIAN_POINT('Ctrl Pts',(48.5210265403013,-6.32271656818346,4.2845451014634));
#23367=CARTESIAN_POINT('Ctrl Pts',(48.5208120050159,-6.31495176722323,4.28513385994596));
#23368=CARTESIAN_POINT('Ctrl Pts',(48.5201635803604,-6.30626433210881,4.28573553175603));
#23369=CARTESIAN_POINT('Ctrl Pts',(48.5195712981029,-6.29832907912766,4.28628510915853));
#23370=CARTESIAN_POINT('Ctrl Pts',(48.5186151096696,-6.28962376481004,4.28684548308324));
#23371=CARTESIAN_POINT('Ctrl Pts',(48.5171272023472,-6.28030805427429,4.28741743373515));
#23372=CARTESIAN_POINT('Ctrl Pts',(48.5157114991037,-6.27144440972979,4.28796162918391));
#23373=CARTESIAN_POINT('Ctrl Pts',(48.5138129998971,-6.26202846118944,4.2885162789801));
#23374=CARTESIAN_POINT('Ctrl Pts',(48.511309655777,-6.25223759022023,4.28907860942712));
#23375=CARTESIAN_POINT('Ctrl Pts',(48.5089253111837,-6.24291214028634,4.28961420880806));
#23376=CARTESIAN_POINT('Ctrl Pts',(48.5059913516873,-6.23324739180496,4.29015670363398));
#23377=CARTESIAN_POINT('Ctrl Pts',(48.5024397868646,-6.22342541541284,4.29070122155964));
#23378=CARTESIAN_POINT('Ctrl Pts',(48.5007677320116,-6.21880128939719,4.29095757724668));
#23379=CARTESIAN_POINT('Ctrl Pts',(48.4989594246657,-6.21414266599999,4.29121435123722));
#23380=CARTESIAN_POINT('Ctrl Pts',(48.4970115875589,-6.20946994630411,4.29147091589307));
#23381=CARTESIAN_POINT('Ctrl Pts',(48.4970122186805,-6.20946968446902,4.29147093865584));
#23382=CARTESIAN_POINT('Ctrl Pts',(48.5072128795205,-6.17306838542385,3.58975548987207));
#23383=CARTESIAN_POINT('Ctrl Pts',(48.5119067425057,-6.13245845073776,2.88748313485153));
#23384=CARTESIAN_POINT('Ctrl Pts',(48.5152120761074,-6.04366518477756,1.48590910732938));
#23385=CARTESIAN_POINT('Ctrl Pts',(48.5210410761359,-6.01733942146297,0.784522401668223));
#23386=CARTESIAN_POINT('Ctrl Pts',(48.5210408433891,-6.00666333723546,0.0824317919201338));
#23387=CARTESIAN_POINT('Ctrl Pts',(48.5210408433891,-6.00666333723546,0.0824317919201338));
#23388=CARTESIAN_POINT('Ctrl Pts',(48.5210407270156,-6.00132529512183,0.433477096794441));
#23389=CARTESIAN_POINT('Ctrl Pts',(48.5195832988733,-5.99973567328077,0.784574339427845));
#23390=CARTESIAN_POINT('Ctrl Pts',(48.5098524785301,-5.9982057973698,1.48689990256317));
#23391=CARTESIAN_POINT('Ctrl Pts',(48.5015790863291,-5.99826554329988,1.83812822306509));
#23392=CARTESIAN_POINT('Ctrl Pts',(48.4606829528563,-5.99214762358588,2.8920506048991));
#23393=CARTESIAN_POINT('Ctrl Pts',(48.4174823767142,-5.99475664078831,3.59330337784589));
#23394=CARTESIAN_POINT('Ctrl Pts',(48.3614264232796,-6.007051447105,4.29441317095755));
#23395=CARTESIAN_POINT('Ctrl Pts',(48.5210409597624,-6.01200137934921,0.433477096794178));
#23396=CARTESIAN_POINT('Ctrl Pts',(48.5200991113386,-6.008795254323,0.706493516751188));
#23397=CARTESIAN_POINT('Ctrl Pts',(48.5180114541291,-6.0083511479787,0.997581379054961));
#23398=CARTESIAN_POINT('Ctrl Pts',(48.5081357594368,-6.0082917350604,1.61268346918306));
#23399=CARTESIAN_POINT('Ctrl Pts',(48.5003285876369,-6.00864450579789,1.93670273194495));
#23400=CARTESIAN_POINT('Ctrl Pts',(48.4602502315076,-6.00381665756613,2.95333187554498));
#23401=CARTESIAN_POINT('Ctrl Pts',(48.418730443527,-6.00697011627401,3.63027912060255));
#23402=CARTESIAN_POINT('Ctrl Pts',(48.3663922968565,-6.01900581052064,4.29446585817755));
#23403=CARTESIAN_POINT('Ctrl Pts',(48.519583767942,-6.02125184123474,0.784346425646489));
#23404=CARTESIAN_POINT('Ctrl Pts',(48.5183837318917,-6.01828947675535,0.997236185019257));
#23405=CARTESIAN_POINT('Ctrl Pts',(48.5159956580425,-6.01789996842507,1.24226674480952));
#23406=CARTESIAN_POINT('Ctrl Pts',(48.5060961369461,-6.01814206511776,1.7866120430789));
#23407=CARTESIAN_POINT('Ctrl Pts',(48.4985559882231,-6.01872578610798,2.08593433396436));
#23408=CARTESIAN_POINT('Ctrl Pts',(48.4596398458567,-6.015691965127,3.05034122012432));
#23409=CARTESIAN_POINT('Ctrl Pts',(48.420074865141,-6.02014444454683,3.69245653518678));
#23410=CARTESIAN_POINT('Ctrl Pts',(48.3730775094482,-6.0312811715619,4.29459893941745));
#23411=CARTESIAN_POINT('Ctrl Pts',(48.5162561594143,-6.04818290219394,1.48575918435436));
#23412=CARTESIAN_POINT('Ctrl Pts',(48.5144994209881,-6.0443265840675,1.61112122466037));
#23413=CARTESIAN_POINT('Ctrl Pts',(48.5114095528176,-6.0428908542814,1.78530549506845));
#23414=CARTESIAN_POINT('Ctrl Pts',(48.5010454692974,-6.04173521007285,2.20924933950468));
#23415=CARTESIAN_POINT('Ctrl Pts',(48.4937353771031,-6.04195544060946,2.45901835404076));
#23416=CARTESIAN_POINT('Ctrl Pts',(48.4576393364659,-6.04033961883415,3.28859696656493));
#23417=CARTESIAN_POINT('Ctrl Pts',(48.4227028838054,-6.04594588203863,3.83761867004076));
#23418=CARTESIAN_POINT('Ctrl Pts',(48.3875464536895,-6.05467770199135,4.29515956957339));
#23419=CARTESIAN_POINT('Ctrl Pts',(48.514385742707,-6.06586350126761,1.83630261420992));
#23420=CARTESIAN_POINT('Ctrl Pts',(48.5123333385524,-6.06089216511441,1.93426197646659));
#23421=CARTESIAN_POINT('Ctrl Pts',(48.5088435172107,-6.05836696394202,2.08365645022257));
#23422=CARTESIAN_POINT('Ctrl Pts',(48.4980397660539,-6.0555205802839,2.4579550253468));
#23423=CARTESIAN_POINT('Ctrl Pts',(48.4906923511837,-6.05514353309329,2.68286793785579));
#23424=CARTESIAN_POINT('Ctrl Pts',(48.456252061747,-6.05313466114754,3.42984174885938));
#23425=CARTESIAN_POINT('Ctrl Pts',(48.4239864808558,-6.05857299125761,3.92060339031051));
#23426=CARTESIAN_POINT('Ctrl Pts',(48.395330185339,-6.06579887137954,4.29558711848945));
#23427=CARTESIAN_POINT('Ctrl Pts',(48.5119067425057,-6.13245845073776,2.88748313485153));
#23428=CARTESIAN_POINT('Ctrl Pts',(48.5086939110956,-6.12571278892215,2.94770884178122));
#23429=CARTESIAN_POINT('Ctrl Pts',(48.5036610021172,-6.11975101509668,3.04468476182455));
#23430=CARTESIAN_POINT('Ctrl Pts',(48.4906361945831,-6.10935599899704,3.28398546728826));
#23431=CARTESIAN_POINT('Ctrl Pts',(48.4826251617104,-6.10489083403436,3.42631528764621));
#23432=CARTESIAN_POINT('Ctrl Pts',(48.4521822007991,-6.09364276612037,3.87910729130324));
#23433=CARTESIAN_POINT('Ctrl Pts',(48.4273657339126,-6.0919301033917,4.15637445269361));
#23434=CARTESIAN_POINT('Ctrl Pts',(48.4168189204168,-6.09473681170808,4.29751198620641));
#23435=CARTESIAN_POINT('Ctrl Pts',(48.5072128795205,-6.17306838542385,3.58975548987207));
#23436=CARTESIAN_POINT('Ctrl Pts',(48.503214467014,-6.16367997399769,3.62572661399501));
#23437=CARTESIAN_POINT('Ctrl Pts',(48.4973225962853,-6.15479195321227,3.68769530647388));
#23438=CARTESIAN_POINT('Ctrl Pts',(48.4830998622463,-6.13882811012295,3.83329116201583));
#23439=CARTESIAN_POINT('Ctrl Pts',(48.4747689989361,-6.13175228781906,3.9169183250789));
#23440=CARTESIAN_POINT('Ctrl Pts',(48.4481398059271,-6.11446024442977,4.15478252095291));
#23441=CARTESIAN_POINT('Ctrl Pts',(48.4289898518244,-6.10813589078395,4.29597769638082));
#23442=CARTESIAN_POINT('Ctrl Pts',(48.4286614639743,-6.10812801481236,4.29965152597613));
#23443=CARTESIAN_POINT('Ctrl Pts',(48.4970122186805,-6.20946968446903,4.29147093865584));
#23444=CARTESIAN_POINT('Ctrl Pts',(48.4920141354583,-6.19747947407209,4.29212928585064));
#23445=CARTESIAN_POINT('Ctrl Pts',(48.4858839393066,-6.18527410478073,4.29279802181868));
#23446=CARTESIAN_POINT('Ctrl Pts',(48.4724837048733,-6.16205725105381,4.29423379060227));
#23447=CARTESIAN_POINT('Ctrl Pts',(48.4652136665918,-6.15104576661825,4.29500082341782));
#23448=CARTESIAN_POINT('Ctrl Pts',(48.4433803641462,-6.12223844456224,4.29756564608736));
#23449=CARTESIAN_POINT('Ctrl Pts',(48.4289711156128,-6.10843369230011,4.29961932362136));
#23450=CARTESIAN_POINT('Ctrl Pts',(48.4286600918172,-6.1084337131847,4.30318207891644));
#23451=CARTESIAN_POINT('Ctrl Pts',(48.4970122186805,-6.20946968446902,4.29147093865584));
#23452=CARTESIAN_POINT('Ctrl Pts',(48.4870160522361,-6.18548926367516,4.29278763304545));
#23453=CARTESIAN_POINT('Ctrl Pts',(48.4724914340736,-6.16064820730357,4.29414588252798));
#23454=CARTESIAN_POINT('Ctrl Pts',(48.4433803641462,-6.12223844456224,4.29756564608736));
#23455=CARTESIAN_POINT('Ctrl Pts',(48.4289711156128,-6.10843369230011,4.29961932362136));
#23456=CARTESIAN_POINT('Ctrl Pts',(48.4286600918172,-6.10843371318471,4.30318207891645));
#23457=CARTESIAN_POINT('',(48.3614264232796,-6.00705144710501,4.29441317095755));
#23458=CARTESIAN_POINT('Ctrl Pts',(48.3614264232796,-6.00705144710501,4.29441317095755));
#23459=CARTESIAN_POINT('Ctrl Pts',(48.3635409992397,-6.01214187260733,4.29443560631099));
#23460=CARTESIAN_POINT('Ctrl Pts',(48.3658956083523,-6.01712837927263,4.29447185537051));
#23461=CARTESIAN_POINT('Ctrl Pts',(48.3684077092534,-6.02202472097697,4.29452495588205));
#23462=CARTESIAN_POINT('Ctrl Pts',(48.371521187098,-6.02809320787936,4.29459076823304));
#23463=CARTESIAN_POINT('Ctrl Pts',(48.3748781145008,-6.03402508126499,4.29468221557362));
#23464=CARTESIAN_POINT('Ctrl Pts',(48.3783993459457,-6.03985134429203,4.29480804388813));
#23465=CARTESIAN_POINT('Ctrl Pts',(48.3790315660535,-6.04089742169324,4.29483063575458));
#23466=CARTESIAN_POINT('Ctrl Pts',(48.3796692141087,-6.04194007079459,4.29485434909697));
#23467=CARTESIAN_POINT('Ctrl Pts',(48.3803119815688,-6.04297943677662,4.29487925449542));
#23468=CARTESIAN_POINT('Ctrl Pts',(48.3843513079875,-6.04951109671614,4.29503576682709));
#23469=CARTESIAN_POINT('Ctrl Pts',(48.3885900320879,-6.05591441295341,4.29523764776086));
#23470=CARTESIAN_POINT('Ctrl Pts',(48.3929742996562,-6.06221542044989,4.29551276627763));
#23471=CARTESIAN_POINT('Ctrl Pts',(48.3960776511973,-6.06667551350295,4.29570750564051));
#23472=CARTESIAN_POINT('Ctrl Pts',(48.3992541326303,-6.07108307969412,4.29593860867427));
#23473=CARTESIAN_POINT('Ctrl Pts',(48.4024930970316,-6.07544485148906,4.29622874106177));
#23474=CARTESIAN_POINT('Ctrl Pts',(48.4052050793963,-6.07909695960793,4.29647166868333));
#23475=CARTESIAN_POINT('Ctrl Pts',(48.4079603485602,-6.08271598873198,4.29675485663422));
#23476=CARTESIAN_POINT('Ctrl Pts',(48.4107527583317,-6.08630203841479,4.29711043443884));
#23477=CARTESIAN_POINT('Ctrl Pts',(48.4127529501023,-6.08887071122852,4.29736513337519));
#23478=CARTESIAN_POINT('Ctrl Pts',(48.4147730680574,-6.09142345508024,4.2976561771177));
#23479=CARTESIAN_POINT('Ctrl Pts',(48.4168100839244,-6.09395875854621,4.29801585661109));
#23480=CARTESIAN_POINT('Ctrl Pts',(48.418234877991,-6.09573208068565,4.29826743501868));
#23481=CARTESIAN_POINT('Ctrl Pts',(48.4196681079838,-6.09749699613462,4.29855158068182));
#23482=CARTESIAN_POINT('Ctrl Pts',(48.4211080201929,-6.09925274341038,4.2989009079552));
#23483=CARTESIAN_POINT('Ctrl Pts',(48.4220746454017,-6.10043139136287,4.29913541429971));
#23484=CARTESIAN_POINT('Ctrl Pts',(48.4230445410963,-6.10160612835187,4.29939833468633));
#23485=CARTESIAN_POINT('Ctrl Pts',(48.4240147544947,-6.10277497406914,4.29972059174042));
#23486=CARTESIAN_POINT('Ctrl Pts',(48.4246007385427,-6.10348092695132,4.29991522674895));
#23487=CARTESIAN_POINT('Ctrl Pts',(48.4251874240369,-6.10418538595768,4.30013130395329));
#23488=CARTESIAN_POINT('Ctrl Pts',(48.4257707705672,-6.10488492040487,4.30038975841948));
#23489=CARTESIAN_POINT('Ctrl Pts',(48.4261752550347,-6.10536996797714,4.3005689671945));
#23490=CARTESIAN_POINT('Ctrl Pts',(48.4265807298491,-6.10585567764595,4.30076899482023));
#23491=CARTESIAN_POINT('Ctrl Pts',(48.4269781707174,-6.10633304315556,4.30100976460741));
#23492=CARTESIAN_POINT('Ctrl Pts',(48.4272533213187,-6.10666352604623,4.30117645091727));
#23493=CARTESIAN_POINT('Ctrl Pts',(48.4275278798357,-6.1069938323219,4.30136389578696));
#23494=CARTESIAN_POINT('Ctrl Pts',(48.4277875302301,-6.10730907399672,4.30159035252877));
#23495=CARTESIAN_POINT('Ctrl Pts',(48.4279029314537,-6.10744918268042,4.30169100088381));
#23496=CARTESIAN_POINT('Ctrl Pts',(48.4280156595997,-6.10758666990988,4.30179985197504));
#23497=CARTESIAN_POINT('Ctrl Pts',(48.4281226651196,-6.10771844494382,4.30192110165643));
#23498=CARTESIAN_POINT('Ctrl Pts',(48.4281945740975,-6.10780699932883,4.30200258287975));
#23499=CARTESIAN_POINT('Ctrl Pts',(48.4282626359345,-6.10789132123128,4.30208695977842));
#23500=CARTESIAN_POINT('Ctrl Pts',(48.4283341793758,-6.10798127288354,4.30219267071245));
#23501=CARTESIAN_POINT('Ctrl Pts',(48.4283699510964,-6.10802624870967,4.30224552617946));
#23502=CARTESIAN_POINT('Ctrl Pts',(48.4284054731147,-6.1080710493202,4.30229992515555));
#23503=CARTESIAN_POINT('Ctrl Pts',(48.4284536139635,-6.10813310869685,4.30239026699659));
#23504=CARTESIAN_POINT('Ctrl Pts',(48.4284776843793,-6.10816413837406,4.30243543790092));
#23505=CARTESIAN_POINT('Ctrl Pts',(48.4285124648215,-6.10820885152106,4.30249946297644));
#23506=CARTESIAN_POINT('Ctrl Pts',(48.4285567328635,-6.10826888896255,4.30261832089737));
#23507=CARTESIAN_POINT('Ctrl Pts',(48.4285893193314,-6.10831308355696,4.30270581425947));
#23508=CARTESIAN_POINT('Ctrl Pts',(48.4286274756883,-6.10836602282788,4.30282297533157));
#23509=CARTESIAN_POINT('Ctrl Pts',(48.4286479760914,-6.10840319283353,4.30298683407108));
#23510=CARTESIAN_POINT('Ctrl Pts',(48.4286553250614,-6.10841651751098,4.30304557403661));
#23511=CARTESIAN_POINT('Ctrl Pts',(48.428660119669,-6.1084275022391,4.30311034818538));
#23512=CARTESIAN_POINT('Ctrl Pts',(48.4286600918174,-6.1084337131341,4.3031820783319));
#23513=CARTESIAN_POINT('Ctrl Pts',(48.3614264232796,-6.00705144710501,4.29441317095755));
#23514=CARTESIAN_POINT('Ctrl Pts',(48.4174823767142,-5.99475664078831,3.59330337784589));
#23515=CARTESIAN_POINT('Ctrl Pts',(48.4606829528563,-5.99214762358588,2.8920506048991));
#23516=CARTESIAN_POINT('Ctrl Pts',(48.51521113082,-6.00030484987122,1.48682076245375));
#23517=CARTESIAN_POINT('Ctrl Pts',(48.521040610642,-5.99598725300821,0.78452240166875));
#23518=CARTESIAN_POINT('Ctrl Pts',(48.5210408433891,-6.00666333723546,0.0824317919201338));
#23519=CARTESIAN_POINT('Ctrl Pts',(0.0835265683425695,-6.00666333723547,
-48.3550824830876));
#23520=CARTESIAN_POINT('Ctrl Pts',(0.083526568342042,-6.02801550569023,
-48.3550829485813));
#23521=CARTESIAN_POINT('Ctrl Pts',(0.0835265683323826,-6.05386667280684,
-48.3547257065917));
#23522=CARTESIAN_POINT('Ctrl Pts',(0.0835265683490379,-6.10694539169998,
-48.3564911068392));
#23523=CARTESIAN_POINT('Ctrl Pts',(0.083526568355074,-6.12148849588211,
-48.3550682080606));
#23524=CARTESIAN_POINT('Ctrl Pts',(0.0835265683620966,-6.14692278878554,
-48.3550682080606));
#23525=CARTESIAN_POINT('Ctrl Pts',(-0.26751873653172,-6.01200137934907,
-48.3550825994612));
#23526=CARTESIAN_POINT('Ctrl Pts',(-0.189316787302164,-6.03090918789885,
-48.3550233774054));
#23527=CARTESIAN_POINT('Ctrl Pts',(-0.189103447683842,-6.05382055712372,
-48.3547233757443));
#23528=CARTESIAN_POINT('Ctrl Pts',(-0.227816669589675,-6.1069582237581,
-48.3564923306724));
#23529=CARTESIAN_POINT('Ctrl Pts',(-0.266743231133337,-6.12148849588211,
-48.3550682080606));
#23530=CARTESIAN_POINT('Ctrl Pts',(-0.266821084249414,-6.14692278878554,
-48.3550682080606));
#23531=CARTESIAN_POINT('Ctrl Pts',(-0.618388065391316,-6.02125184123581,
-48.3536254076414));
#23532=CARTESIAN_POINT('Ctrl Pts',(-0.484920401704102,-6.03698783585495,
-48.3547116236264));
#23533=CARTESIAN_POINT('Ctrl Pts',(-0.48455720285307,-6.05830967273443,
-48.3548266592081));
#23534=CARTESIAN_POINT('Ctrl Pts',(-0.550623003694885,-6.11145963930963,
-48.356627577415));
#23535=CARTESIAN_POINT('Ctrl Pts',(-0.617052003405587,-6.12687873284897,
-48.3550682080599));
#23536=CARTESIAN_POINT('Ctrl Pts',(-0.617168736860925,-6.15072449281721,
-48.35506820806));
#23537=CARTESIAN_POINT('Ctrl Pts',(-1.31980082412786,-6.04818290219911,
-48.350297799115));
#23538=CARTESIAN_POINT('Ctrl Pts',(-1.12748085805452,-6.05935112779907,
-48.3534476946121));
#23539=CARTESIAN_POINT('Ctrl Pts',(-1.12692130709796,-6.07865710025978,
-48.3544824220894));
#23540=CARTESIAN_POINT('Ctrl Pts',(-1.22201691706508,-6.12977840933565,
-48.3565730737421));
#23541=CARTESIAN_POINT('Ctrl Pts',(-1.31767207800253,-6.14643370208422,
-48.3550682080582));
#23542=CARTESIAN_POINT('Ctrl Pts',(-1.31778153573098,-6.16593130894387,
-48.3550682080584));
#23543=CARTESIAN_POINT('Ctrl Pts',(-1.67034425400482,-6.06586350127566,
-48.3484273824083));
#23544=CARTESIAN_POINT('Ctrl Pts',(-1.47443454517931,-6.0756803173362,-48.3525105585865));
#23545=CARTESIAN_POINT('Ctrl Pts',(-1.47382850134994,-6.09455995772354,
-48.3540499407165));
#23546=CARTESIAN_POINT('Ctrl Pts',(-1.57060291891823,-6.14361803658469,
-48.3563908429315));
#23547=CARTESIAN_POINT('Ctrl Pts',(-1.66798338032722,-6.16059843435261,
-48.3550682080572));
#23548=CARTESIAN_POINT('Ctrl Pts',(-1.66804668198952,-6.17733642103887,
-48.3550682080574));
#23549=CARTESIAN_POINT('Ctrl Pts',(-2.72152477473183,-6.1324584507553,-48.3459483822083));
#23550=CARTESIAN_POINT('Ctrl Pts',(-2.60108317857739,-6.14582978514635,
-48.3523410705545));
#23551=CARTESIAN_POINT('Ctrl Pts',(-2.60045731402345,-6.16286923349055,
-48.3545898781298));
#23552=CARTESIAN_POINT('Ctrl Pts',(-2.65931970428615,-6.19966838879309,
-48.3563704085999));
#23553=CARTESIAN_POINT('Ctrl Pts',(-2.71880795910709,-6.21324540616175,
-48.3550682080552));
#23554=CARTESIAN_POINT('Ctrl Pts',(-2.71859460170623,-6.22295686941886,
-48.3550682080555));
#23555=CARTESIAN_POINT('Ctrl Pts',(-3.4237971299004,-6.17306838545285,-48.3412545192219));
#23556=CARTESIAN_POINT('Ctrl Pts',(-3.3518548815626,-6.1918452082941,-48.3492513442317));
#23557=CARTESIAN_POINT('Ctrl Pts',(-3.35085408874517,-6.21237399283442,
-48.35270476644));
#23558=CARTESIAN_POINT('Ctrl Pts',(-3.38453260164791,-6.24739159904062,
-48.3556131983518));
#23559=CARTESIAN_POINT('Ctrl Pts',(-3.41921190736808,-6.26188042070649,
-48.3550682080552));
#23560=CARTESIAN_POINT('Ctrl Pts',(-3.41862985610548,-6.26857731779886,
-48.3550682080555));
#23561=CARTESIAN_POINT('Ctrl Pts',(-4.1255125788106,-6.20946968450873,-48.331053858379));
#23562=CARTESIAN_POINT('Ctrl Pts',(-4.12419588418111,-6.23345010528185,
-48.3410500248235));
#23563=CARTESIAN_POINT('Ctrl Pts',(-4.12290068587948,-6.25674581560883,
-48.3470536122439));
#23564=CARTESIAN_POINT('Ctrl Pts',(-4.1203869551102,-6.29803503999845,-48.3540627038624));
#23565=CARTESIAN_POINT('Ctrl Pts',(-4.11916842264253,-6.31602855406109,
-48.3550682080606));
#23566=CARTESIAN_POINT('Ctrl Pts',(-4.11800505968097,-6.32940458230552,
-48.3550682080606));
#23567=CARTESIAN_POINT('',(-4.12551257083619,-6.20946977623546,-48.331053637283));
#23568=CARTESIAN_POINT('',(0.0835265683425695,-6.00666333723547,-48.3550824830876));
#23569=CARTESIAN_POINT('Ctrl Pts',(-4.1255125788106,-6.20946968450871,-48.331053858379));
#23570=CARTESIAN_POINT('Ctrl Pts',(-3.4237971299004,-6.17306838545285,-48.3412545192219));
#23571=CARTESIAN_POINT('Ctrl Pts',(-2.72152477473183,-6.1324584507553,-48.3459483822083));
#23572=CARTESIAN_POINT('Ctrl Pts',(-1.31995074709581,-6.04366518478245,
-48.3492537158084));
#23573=CARTESIAN_POINT('Ctrl Pts',(-0.618564041406008,-6.01733942146266,
-48.355082715835));
#23574=CARTESIAN_POINT('Ctrl Pts',(0.0835265683425695,-6.00666333723547,
-48.3550824830876));
#23575=CARTESIAN_POINT('Ctrl Pts',(-4.12551255488737,-6.20946995968897,
-48.331053195091));
#23576=CARTESIAN_POINT('Ctrl Pts',(-4.12497035738504,-6.21934480701976,
-48.335169557573));
#23577=CARTESIAN_POINT('Ctrl Pts',(-4.12442730924739,-6.22915570483163,
-48.3386594793373));
#23578=CARTESIAN_POINT('Ctrl Pts',(-4.12388899791465,-6.23871408127349,
-48.3415673780406));
#23579=CARTESIAN_POINT('Ctrl Pts',(-4.12331783797941,-6.24885572484929,
-48.3446527212873));
#23580=CARTESIAN_POINT('Ctrl Pts',(-4.12275211909699,-6.25871184341249,
-48.3470835469279));
#23581=CARTESIAN_POINT('Ctrl Pts',(-4.12219611252078,-6.26808527594625,
-48.3489661577096));
#23582=CARTESIAN_POINT('Ctrl Pts',(-4.12161469929116,-6.27788702634866,
-48.3509347941638));
#23583=CARTESIAN_POINT('Ctrl Pts',(-4.12104396471119,-6.28716030960515,
-48.3523055172344));
#23584=CARTESIAN_POINT('Ctrl Pts',(-4.12048486600072,-6.29572520171176,
-48.3532382740045));
#23585=CARTESIAN_POINT('Ctrl Pts',(-4.11987706916655,-6.3050361055109,-48.3542522749337));
#23586=CARTESIAN_POINT('Ctrl Pts',(-4.11928303136841,-6.31350977078143,
-48.3547509151621));
#23587=CARTESIAN_POINT('Ctrl Pts',(-4.11869878418713,-6.32097498479525,
-48.3549536869316));
#23588=CARTESIAN_POINT('Ctrl Pts',(-4.11846619004874,-6.32394695466881,
-48.3550344122248));
#23589=CARTESIAN_POINT('Ctrl Pts',(-4.11823509369702,-6.32675971428282,
-48.3550681961923));
#23590=CARTESIAN_POINT('Ctrl Pts',(-4.11800505968097,-6.32940458230551,
-48.3550682080575));
#23591=CARTESIAN_POINT('Ctrl Pts',(0.0835265683620966,-6.14692278878557,
-48.3550682080606));
#23592=CARTESIAN_POINT('Ctrl Pts',(0.083526568355074,-6.12148849588211,
-48.3550682080606));
#23593=CARTESIAN_POINT('Ctrl Pts',(0.0835265683490379,-6.10694539169998,
-48.3564911068392));
#23594=CARTESIAN_POINT('Ctrl Pts',(0.0835265683323826,-6.05386667280684,
-48.3547257065917));
#23595=CARTESIAN_POINT('Ctrl Pts',(0.083526568342042,-6.02801550569023,
-48.3550829485813));
#23596=CARTESIAN_POINT('Ctrl Pts',(0.0835265683425695,-6.00666333723547,
-48.3550824830876));
#23597=CARTESIAN_POINT('Ctrl Pts',(0.0835265683425695,-6.00666333723547,
-48.3550824830876));
#23598=CARTESIAN_POINT('Ctrl Pts',(0.434571873216595,-6.01200137934925,
-48.3550825994608));
#23599=CARTESIAN_POINT('Ctrl Pts',(0.785441202068902,-6.02125184123479,
-48.3536254076403));
#23600=CARTESIAN_POINT('Ctrl Pts',(1.48685396077679,-6.04818290219399,-48.3502977991125));
#23601=CARTESIAN_POINT('Ctrl Pts',(1.83739739063237,-6.06586350126766,-48.3484273824051));
#23602=CARTESIAN_POINT('Ctrl Pts',(2.88857791127407,-6.13245845073778,-48.3459483822043));
#23603=CARTESIAN_POINT('Ctrl Pts',(3.59085026629458,-6.17306838542386,-48.341254519219));
#23604=CARTESIAN_POINT('Ctrl Pts',(4.29256571507838,-6.20946968446905,-48.331053858379));
#23605=CARTESIAN_POINT('Ctrl Pts',(0.083526568342042,-6.02801550569023,
-48.3550829485813));
#23606=CARTESIAN_POINT('Ctrl Pts',(0.356369923984709,-6.03090918789797,
-48.3550233774046));
#23607=CARTESIAN_POINT('Ctrl Pts',(0.651973538377631,-6.03698783585282,
-48.3547116236253));
#23608=CARTESIAN_POINT('Ctrl Pts',(1.29453399470195,-6.05935112779398,-48.3534476946107));
#23609=CARTESIAN_POINT('Ctrl Pts',(1.64148768180965,-6.07568031732944,-48.352510558585));
#23610=CARTESIAN_POINT('Ctrl Pts',(2.76813631515469,-6.14582978513442,-48.3523410705534));
#23611=CARTESIAN_POINT('Ctrl Pts',(3.51890801804868,-6.19184520827618,-48.349251344232));
#23612=CARTESIAN_POINT('Ctrl Pts',(4.29124902068876,-6.23345010526292,-48.3410500248235));
#23613=CARTESIAN_POINT('Ctrl Pts',(0.0835265683323826,-6.05386667280684,
-48.3547257065917));
#23614=CARTESIAN_POINT('Ctrl Pts',(0.356156584348608,-6.0538205571228,-48.3547233757437));
#23615=CARTESIAN_POINT('Ctrl Pts',(0.651610339513195,-6.05830967273256,
-48.3548266592073));
#23616=CARTESIAN_POINT('Ctrl Pts',(1.29397444374515,-6.07865710025598,-48.3544824220886));
#23617=CARTESIAN_POINT('Ctrl Pts',(1.64088163798883,-6.09455995771877,-48.3540499407158));
#23618=CARTESIAN_POINT('Ctrl Pts',(2.76751045064042,-6.16286923348299,-48.3545898781298));
#23619=CARTESIAN_POINT('Ctrl Pts',(3.51790722531375,-6.21237399282374,-48.352704766441));
#23620=CARTESIAN_POINT('Ctrl Pts',(4.28995382250124,-6.25674581559981,-48.3470536122438));
#23621=CARTESIAN_POINT('Ctrl Pts',(0.0835265683490379,-6.10694539169998,
-48.3564911068392));
#23622=CARTESIAN_POINT('Ctrl Pts',(0.39486980628775,-6.10695822375761,-48.3564923306722));
#23623=CARTESIAN_POINT('Ctrl Pts',(0.717676140391613,-6.11145963930883,
-48.3566275774147));
#23624=CARTESIAN_POINT('Ctrl Pts',(1.38907005375915,-6.12977840933439,-48.356573073742));
#23625=CARTESIAN_POINT('Ctrl Pts',(1.73765605561098,-6.14361803658331,-48.3563908429315));
#23626=CARTESIAN_POINT('Ctrl Pts',(2.8263728409791,-6.1996683887915,-48.3563704086003));
#23627=CARTESIAN_POINT('Ctrl Pts',(3.55158573833553,-6.24739159903889,-48.3556131983526));
#23628=CARTESIAN_POINT('Ctrl Pts',(4.28744009184022,-6.29803503999889,-48.3540627038624));
#23629=CARTESIAN_POINT('Ctrl Pts',(0.083526568355074,-6.12148849588211,
-48.3550682080606));
#23630=CARTESIAN_POINT('Ctrl Pts',(0.433796367843485,-6.12148849588211,
-48.3550682080606));
#23631=CARTESIAN_POINT('Ctrl Pts',(0.784105140116609,-6.12687873284897,
-48.3550682080599));
#23632=CARTESIAN_POINT('Ctrl Pts',(1.48472521471617,-6.14643370208422,-48.3550682080582));
#23633=CARTESIAN_POINT('Ctrl Pts',(1.83503651704262,-6.1605984343526,-48.3550682080572));
#23634=CARTESIAN_POINT('Ctrl Pts',(2.88586109582775,-6.21324540616174,-48.3550682080552));
#23635=CARTESIAN_POINT('Ctrl Pts',(3.58626504409225,-6.26188042070648,-48.3550682080552));
#23636=CARTESIAN_POINT('Ctrl Pts',(4.28622155936672,-6.31602855406106,-48.3550682080606));
#23637=CARTESIAN_POINT('Ctrl Pts',(0.0835265683620966,-6.14692278878554,
-48.3550682080606));
#23638=CARTESIAN_POINT('Ctrl Pts',(0.433874220973607,-6.14692278878554,
-48.3550682080606));
#23639=CARTESIAN_POINT('Ctrl Pts',(0.784221873585118,-6.15072449281721,
-48.35506820806));
#23640=CARTESIAN_POINT('Ctrl Pts',(1.48483467245517,-6.16593130894387,-48.3550682080584));
#23641=CARTESIAN_POINT('Ctrl Pts',(1.83509981871371,-6.17733642103887,-48.3550682080574));
#23642=CARTESIAN_POINT('Ctrl Pts',(2.88564773843042,-6.22295686941886,-48.3550682080555));
#23643=CARTESIAN_POINT('Ctrl Pts',(3.58568299282967,-6.26857731779886,-48.3550682080555));
#23644=CARTESIAN_POINT('Ctrl Pts',(4.28505819640516,-6.32940458230553,-48.3550682080606));
#23645=CARTESIAN_POINT('',(4.29256570749077,-6.20946977174739,-48.3310536480052));
#23646=CARTESIAN_POINT('Ctrl Pts',(4.28505819640516,-6.32940458230551,-48.3550682080579));
#23647=CARTESIAN_POINT('Ctrl Pts',(4.28563987788593,-6.32271656818346,-48.3550681799999));
#23648=CARTESIAN_POINT('Ctrl Pts',(4.28622863636849,-6.31495176722324,-48.3548536447145));
#23649=CARTESIAN_POINT('Ctrl Pts',(4.28683030817856,-6.30626433210882,-48.3542052200589));
#23650=CARTESIAN_POINT('Ctrl Pts',(4.28737988558105,-6.29832907912768,-48.3536129378015));
#23651=CARTESIAN_POINT('Ctrl Pts',(4.28794025950575,-6.28962376481006,-48.3526567493682));
#23652=CARTESIAN_POINT('Ctrl Pts',(4.28851221015767,-6.28030805427432,-48.3511688420458));
#23653=CARTESIAN_POINT('Ctrl Pts',(4.28905640560643,-6.27144440972983,-48.3497531388023));
#23654=CARTESIAN_POINT('Ctrl Pts',(4.28961105540263,-6.2620284611895,-48.3478546395958));
#23655=CARTESIAN_POINT('Ctrl Pts',(4.29017338584965,-6.2522375902203,-48.3453512954757));
#23656=CARTESIAN_POINT('Ctrl Pts',(4.29070898523059,-6.24291214028641,-48.3429669508824));
#23657=CARTESIAN_POINT('Ctrl Pts',(4.29125148005651,-6.23324739180503,-48.3400329913859));
#23658=CARTESIAN_POINT('Ctrl Pts',(4.29179599798217,-6.2234254154129,-48.3364814265633));
#23659=CARTESIAN_POINT('Ctrl Pts',(4.29205235366921,-6.21880128939723,-48.3348093717102));
#23660=CARTESIAN_POINT('Ctrl Pts',(4.29230912765975,-6.214142666,-48.3330010643644));
#23661=CARTESIAN_POINT('Ctrl Pts',(4.2925656923156,-6.20946994630409,-48.3310532272575));
#23662=CARTESIAN_POINT('Ctrl Pts',(4.29256571507836,-6.20946968446903,-48.331053858379));
#23663=CARTESIAN_POINT('Ctrl Pts',(3.59085026629458,-6.17306838542386,-48.341254519219));
#23664=CARTESIAN_POINT('Ctrl Pts',(2.88857791127407,-6.13245845073778,-48.3459483822043));
#23665=CARTESIAN_POINT('Ctrl Pts',(1.4870038837518,-6.04366518477762,-48.3492537158055));
#23666=CARTESIAN_POINT('Ctrl Pts',(0.785617178090622,-6.01733942146302,
-48.3550827158341));
#23667=CARTESIAN_POINT('Ctrl Pts',(0.0835265683425695,-6.00666333723547,
-48.3550824830876));
#23668=CARTESIAN_POINT('Ctrl Pts',(0.0835265683425695,-6.00666333723547,
-48.3550824830876));
#23669=CARTESIAN_POINT('Ctrl Pts',(0.434571873216859,-6.00132529512187,
-48.3550823667139));
#23670=CARTESIAN_POINT('Ctrl Pts',(0.785669115850259,-5.99973567328082,
-48.3536249385716));
#23671=CARTESIAN_POINT('Ctrl Pts',(1.4879946789856,-5.99820579736985,-48.3438941182282));
#23672=CARTESIAN_POINT('Ctrl Pts',(1.83922299948754,-5.99826554329993,-48.3356207260272));
#23673=CARTESIAN_POINT('Ctrl Pts',(2.89314538132166,-5.99214762358589,-48.2947245925549));
#23674=CARTESIAN_POINT('Ctrl Pts',(3.59439815426843,-5.99475664078831,-48.2515240164127));
#23675=CARTESIAN_POINT('Ctrl Pts',(4.29550794738009,-6.007051447105,-48.1954680629781));
#23676=CARTESIAN_POINT('Ctrl Pts',(0.434571873216595,-6.01200137934925,
-48.3550825994608));
#23677=CARTESIAN_POINT('Ctrl Pts',(0.707588293173598,-6.00879525432306,
-48.3541407510368));
#23678=CARTESIAN_POINT('Ctrl Pts',(0.998676155477369,-6.00835114797876,
-48.3520530938273));
#23679=CARTESIAN_POINT('Ctrl Pts',(1.61377824560549,-6.00829173506045,-48.3421773991349));
#23680=CARTESIAN_POINT('Ctrl Pts',(1.9377975083674,-6.00864450579793,-48.334370227335));
#23681=CARTESIAN_POINT('Ctrl Pts',(2.95442665196754,-6.00381665756613,-48.294291871206));
#23682=CARTESIAN_POINT('Ctrl Pts',(3.63137389702508,-6.00697011627401,-48.2527720832255));
#23683=CARTESIAN_POINT('Ctrl Pts',(4.2955606346001,-6.01900581052064,-48.200433936555));
#23684=CARTESIAN_POINT('Ctrl Pts',(0.785441202068902,-6.02125184123479,
-48.3536254076403));
#23685=CARTESIAN_POINT('Ctrl Pts',(0.998330961441668,-6.01828947675541,
-48.3524253715899));
#23686=CARTESIAN_POINT('Ctrl Pts',(1.24336152123193,-6.01789996842513,-48.3500372977406));
#23687=CARTESIAN_POINT('Ctrl Pts',(1.78770681950133,-6.01814206511781,-48.3401377766442));
#23688=CARTESIAN_POINT('Ctrl Pts',(2.08702911038681,-6.01872578610802,-48.3325976279212));
#23689=CARTESIAN_POINT('Ctrl Pts',(3.05143599654687,-6.01569196512699,-48.2936814855552));
#23690=CARTESIAN_POINT('Ctrl Pts',(3.6935513116093,-6.02014444454682,-48.2541165048395));
#23691=CARTESIAN_POINT('Ctrl Pts',(4.29569371583999,-6.0312811715619,-48.2071191491467));
#23692=CARTESIAN_POINT('Ctrl Pts',(1.48685396077679,-6.04818290219399,-48.3502977991125));
#23693=CARTESIAN_POINT('Ctrl Pts',(1.61221600108281,-6.04432658406756,-48.3485410606862));
#23694=CARTESIAN_POINT('Ctrl Pts',(1.78640027149089,-6.04289085428145,-48.3454511925156));
#23695=CARTESIAN_POINT('Ctrl Pts',(2.21034411592712,-6.04173521007289,-48.3350871089954));
#23696=CARTESIAN_POINT('Ctrl Pts',(2.46011313046322,-6.04195544060948,-48.3277770168012));
#23697=CARTESIAN_POINT('Ctrl Pts',(3.28969174298747,-6.04033961883414,-48.2916809761644));
#23698=CARTESIAN_POINT('Ctrl Pts',(3.83871344646328,-6.04594588203862,-48.2567445235039));
#23699=CARTESIAN_POINT('Ctrl Pts',(4.29625434599593,-6.05467770199135,-48.221588093388));
#23700=CARTESIAN_POINT('Ctrl Pts',(1.83739739063237,-6.06586350126766,-48.3484273824051));
#23701=CARTESIAN_POINT('Ctrl Pts',(1.93535675288904,-6.06089216511445,-48.3463749782505));
#23702=CARTESIAN_POINT('Ctrl Pts',(2.08475122664503,-6.05836696394206,-48.3428851569089));
#23703=CARTESIAN_POINT('Ctrl Pts',(2.45904980176926,-6.05552058028392,-48.332081405752));
#23704=CARTESIAN_POINT('Ctrl Pts',(2.68396271427826,-6.0551435330933,-48.3247339908818));
#23705=CARTESIAN_POINT('Ctrl Pts',(3.43093652528192,-6.05313466114753,-48.2902937014455));
#23706=CARTESIAN_POINT('Ctrl Pts',(3.92169816673303,-6.0585729912576,-48.2580281205544));
#23707=CARTESIAN_POINT('Ctrl Pts',(4.29668189491198,-6.06579887137954,-48.2293718250375));
#23708=CARTESIAN_POINT('Ctrl Pts',(2.88857791127407,-6.13245845073778,-48.3459483822043));
#23709=CARTESIAN_POINT('Ctrl Pts',(2.94880361820377,-6.12571278892217,-48.3427355507941));
#23710=CARTESIAN_POINT('Ctrl Pts',(3.0457795382471,-6.11975101509669,-48.3377026418157));
#23711=CARTESIAN_POINT('Ctrl Pts',(3.28508024371081,-6.10935599899704,-48.3246778342816));
#23712=CARTESIAN_POINT('Ctrl Pts',(3.42741006406875,-6.10489083403435,-48.3166668014089));
#23713=CARTESIAN_POINT('Ctrl Pts',(3.88020206772579,-6.09364276612036,-48.2862238404977));
#23714=CARTESIAN_POINT('Ctrl Pts',(4.15746922911613,-6.0919301033917,-48.2614073736111));
#23715=CARTESIAN_POINT('Ctrl Pts',(4.29860676262894,-6.09473681170807,-48.2508605601154));
#23716=CARTESIAN_POINT('Ctrl Pts',(3.59085026629458,-6.17306838542386,-48.341254519219));
#23717=CARTESIAN_POINT('Ctrl Pts',(3.62682139041753,-6.16367997399771,-48.3372561067125));
#23718=CARTESIAN_POINT('Ctrl Pts',(3.6887900828964,-6.15479195321228,-48.3313642359839));
#23719=CARTESIAN_POINT('Ctrl Pts',(3.83438593843836,-6.13882811012295,-48.3171415019449));
#23720=CARTESIAN_POINT('Ctrl Pts',(3.91801310150143,-6.13175228781906,-48.3088106386346));
#23721=CARTESIAN_POINT('Ctrl Pts',(4.15587729737545,-6.11446024442977,-48.2821814456257));
#23722=CARTESIAN_POINT('Ctrl Pts',(4.29707247280335,-6.10813589078395,-48.263031491523));
#23723=CARTESIAN_POINT('Ctrl Pts',(4.30074630239866,-6.10812801481237,-48.2627031036729));
#23724=CARTESIAN_POINT('Ctrl Pts',(4.29256571507838,-6.20946968446905,-48.331053858379));
#23725=CARTESIAN_POINT('Ctrl Pts',(4.29322406227318,-6.1974794740721,-48.3260557751568));
#23726=CARTESIAN_POINT('Ctrl Pts',(4.29389279824122,-6.18527410478074,-48.3199255790051));
#23727=CARTESIAN_POINT('Ctrl Pts',(4.29532856702481,-6.16205725105381,-48.3065253445719));
#23728=CARTESIAN_POINT('Ctrl Pts',(4.29609559984036,-6.15104576661825,-48.2992553062903));
#23729=CARTESIAN_POINT('Ctrl Pts',(4.2986604225099,-6.12223844456225,-48.2774220038447));
#23730=CARTESIAN_POINT('Ctrl Pts',(4.30071410004389,-6.10843369230011,-48.2630127553113));
#23731=CARTESIAN_POINT('Ctrl Pts',(4.30427685533897,-6.1084337131847,-48.2627017315157));
#23732=CARTESIAN_POINT('Ctrl Pts',(4.29256571507836,-6.20946968446903,-48.331053858379));
#23733=CARTESIAN_POINT('Ctrl Pts',(4.29388240946801,-6.18548926367518,-48.3210576919346));
#23734=CARTESIAN_POINT('Ctrl Pts',(4.29524065895049,-6.16064820730358,-48.3065330737723));
#23735=CARTESIAN_POINT('Ctrl Pts',(4.2986604225099,-6.12223844456225,-48.2774220038447));
#23736=CARTESIAN_POINT('Ctrl Pts',(4.30071410004389,-6.10843369230011,-48.2630127553113));
#23737=CARTESIAN_POINT('Ctrl Pts',(4.30427685533897,-6.10843371318471,-48.2627017315157));
#23738=CARTESIAN_POINT('',(4.29550794738007,-6.00705144710501,-48.1954680629781));
#23739=CARTESIAN_POINT('Ctrl Pts',(4.30427685533897,-6.10843371318471,-48.2627017315157));
#23740=CARTESIAN_POINT('Ctrl Pts',(4.29721574945835,-6.10782231644002,-48.26270447583));
#23741=CARTESIAN_POINT('Ctrl Pts',(4.29571869626011,-6.05486890076755,-48.2153315572858));
#23742=CARTESIAN_POINT('Ctrl Pts',(4.29550794738007,-6.00705144710501,-48.1954680629781));
#23743=CARTESIAN_POINT('Ctrl Pts',(4.29550794738007,-6.00705144710501,-48.1954680629781));
#23744=CARTESIAN_POINT('Ctrl Pts',(3.59439815426845,-5.9947566407883,-48.2515240164127));
#23745=CARTESIAN_POINT('Ctrl Pts',(2.89314538132164,-5.99214762358589,-48.2947245925549));
#23746=CARTESIAN_POINT('Ctrl Pts',(1.48791553887618,-6.00030484987127,-48.349252770518));
#23747=CARTESIAN_POINT('Ctrl Pts',(0.785617178091139,-5.99598725300827,
-48.3550822503403));
#23748=CARTESIAN_POINT('Ctrl Pts',(0.0835265683425695,-6.00666333723547,
-48.3550824830876));
#23749=CARTESIAN_POINT('Ctrl Pts',(0.0835265683425695,-6.00666333723547,
-48.3550824830876));
#23750=CARTESIAN_POINT('Ctrl Pts',(0.0835265683430974,-5.9853111687807,
-48.3550820175939));
#23751=CARTESIAN_POINT('Ctrl Pts',(0.0835265683536855,-5.96223275463528,
-48.3547237089017));
#23752=CARTESIAN_POINT('Ctrl Pts',(0.0835265683557651,-5.92795641804993,
-48.3506190569028));
#23753=CARTESIAN_POINT('Ctrl Pts',(0.0835265683561427,-5.90583775506839,
-48.3550682080606));
#23754=CARTESIAN_POINT('Ctrl Pts',(0.0835265683621219,-5.88746284406389,
-48.3550682080606));
#23755=CARTESIAN_POINT('Ctrl Pts',(0.434571873216859,-6.00132529512187,
-48.3550823667139));
#23756=CARTESIAN_POINT('Ctrl Pts',(0.356716052618675,-5.98270666392106,
-48.3550223265529));
#23757=CARTESIAN_POINT('Ctrl Pts',(0.339530012926373,-5.96240686080379,
-48.3547580080134));
#23758=CARTESIAN_POINT('Ctrl Pts',(0.361332410482752,-5.92787973562318,
-48.3505964244568));
#23759=CARTESIAN_POINT('Ctrl Pts',(0.400320847739005,-5.90583775506839,
-48.3550682080606));
#23760=CARTESIAN_POINT('Ctrl Pts',(0.434813981059995,-5.88746284406389,
-48.3550682080606));
#23761=CARTESIAN_POINT('Ctrl Pts',(0.785669115850259,-5.99973567328082,
-48.3536249385716));
#23762=CARTESIAN_POINT('Ctrl Pts',(0.652301278096881,-5.98152768121126,
-48.3538283041958));
#23763=CARTESIAN_POINT('Ctrl Pts',(0.626534464984441,-5.96239709811728,
-48.3533940028309));
#23764=CARTESIAN_POINT('Ctrl Pts',(0.667559641533983,-5.92723732580308,
-48.3484833205478));
#23765=CARTESIAN_POINT('Ctrl Pts',(0.734351631202325,-5.90562906540035,
-48.3519505469248));
#23766=CARTESIAN_POINT('Ctrl Pts',(0.786101399029053,-5.88746284406389,
-48.3512468523357));
#23767=CARTESIAN_POINT('Ctrl Pts',(1.4879946789856,-5.99820579736985,-48.3438941182282));
#23768=CARTESIAN_POINT('Ctrl Pts',(1.29495516989986,-5.97907559060224,-48.3454622940215));
#23769=CARTESIAN_POINT('Ctrl Pts',(1.26276365253708,-5.96099214798812,-48.3443038073388));
#23770=CARTESIAN_POINT('Ctrl Pts',(1.32724155699937,-5.92511301754141,-48.3372314657121));
#23771=CARTESIAN_POINT('Ctrl Pts',(1.42391097882863,-5.9049506781467,-48.33778964566));
#23772=CARTESIAN_POINT('Ctrl Pts',(1.48859334813923,-5.88746284406389,-48.3359596079612));
#23773=CARTESIAN_POINT('Ctrl Pts',(1.83922299948754,-5.99826554329993,-48.3356207260272));
#23774=CARTESIAN_POINT('Ctrl Pts',(1.64203235067299,-5.9777471823028,-48.3381640344836));
#23775=CARTESIAN_POINT('Ctrl Pts',(1.61199486649158,-5.95954166014522,-48.3364512936597));
#23776=CARTESIAN_POINT('Ctrl Pts',(1.68069642929659,-5.92360346889971,-48.3280294755344));
#23777=CARTESIAN_POINT('Ctrl Pts',(1.77943547628625,-5.90448098056108,-48.3267463020471));
#23778=CARTESIAN_POINT('Ctrl Pts',(1.83979788982333,-5.88746284406389,-48.3244937189391));
#23779=CARTESIAN_POINT('Ctrl Pts',(2.54183792071029,-5.99418693015723,-48.3083566370457));
#23780=CARTESIAN_POINT('Ctrl Pts',(2.3943688993912,-5.97194742955366,-48.3098281543785));
#23781=CARTESIAN_POINT('Ctrl Pts',(2.37286182080562,-5.9541339311854,-48.3073282819912));
#23782=CARTESIAN_POINT('Ctrl Pts',(2.42513999615023,-5.91998502842413,-48.2988519283639));
#23783=CARTESIAN_POINT('Ctrl Pts',(2.49892525008213,-5.90343694889074,-48.2961657002436));
#23784=CARTESIAN_POINT('Ctrl Pts',(2.54204089380294,-5.88746284406389,-48.293911948384));
#23785=CARTESIAN_POINT('Ctrl Pts',(2.89280484425267,-5.99381953117216,-48.2907404707647));
#23786=CARTESIAN_POINT('Ctrl Pts',(2.76993041032196,-5.97081802552583,-48.2910861014675));
#23787=CARTESIAN_POINT('Ctrl Pts',(2.75490258987387,-5.95257589046841,-48.2880098223432));
#23788=CARTESIAN_POINT('Ctrl Pts',(2.8013806169872,-5.91860436677926,-48.279680729008));
#23789=CARTESIAN_POINT('Ctrl Pts',(2.86288646454969,-5.90286261480602,-48.2766286483002));
#23790=CARTESIAN_POINT('Ctrl Pts',(2.89307936664327,-5.88746284406389,-48.2747960661052));
#23791=CARTESIAN_POINT('Ctrl Pts',(3.59436240930965,-5.99717808806687,-48.2483101720896));
#23792=CARTESIAN_POINT('Ctrl Pts',(3.52670827105016,-5.97321241327166,-48.2448130739311));
#23793=CARTESIAN_POINT('Ctrl Pts',(3.52251156371763,-5.95314193699471,-48.2403172933123));
#23794=CARTESIAN_POINT('Ctrl Pts',(3.55227792513379,-5.91737158402251,-48.2324397032865));
#23795=CARTESIAN_POINT('Ctrl Pts',(3.58624099388271,-5.90176568155595,-48.2296135008226));
#23796=CARTESIAN_POINT('Ctrl Pts',(3.59490640778678,-5.8874628440639,-48.2289052281065));
#23797=CARTESIAN_POINT('Ctrl Pts',(3.94495305082426,-6.00090404394666,-48.2234960396954));
#23798=CARTESIAN_POINT('Ctrl Pts',(3.9079246208476,-5.97673620504532,-48.2172820993057));
#23799=CARTESIAN_POINT('Ctrl Pts',(3.9080777441129,-5.95526602423799,-48.2119434824335));
#23800=CARTESIAN_POINT('Ctrl Pts',(3.92693056631993,-5.91751946291063,-48.2043703936485));
#23801=CARTESIAN_POINT('Ctrl Pts',(3.94563026526167,-5.9012430823906,-48.2021359217358));
#23802=CARTESIAN_POINT('Ctrl Pts',(3.94569498663788,-5.8874628440639,-48.2021302712649));
#23803=CARTESIAN_POINT('Ctrl Pts',(4.29550794738009,-6.007051447105,-48.1954680629781));
#23804=CARTESIAN_POINT('Ctrl Pts',(4.29540257294009,-5.98314272027373,-48.1855363158242));
#23805=CARTESIAN_POINT('Ctrl Pts',(4.29560464263456,-5.9599264156786,-48.1795491602216));
#23806=CARTESIAN_POINT('Ctrl Pts',(4.2960614692435,-5.91876732373882,-48.1725407225933));
#23807=CARTESIAN_POINT('Ctrl Pts',(4.29631622615797,-5.90082453639418,-48.1715194405676));
#23808=CARTESIAN_POINT('Ctrl Pts',(4.29631622615797,-5.88746284406389,-48.1715194405676));
#23809=CARTESIAN_POINT('Ctrl Pts',(4.29550794738007,-6.00705144710502,-48.1954680629781));
#23810=CARTESIAN_POINT('Ctrl Pts',(4.29546091471046,-5.99638006180393,-48.1910351418385));
#23811=CARTESIAN_POINT('Ctrl Pts',(4.2954708599273,-5.9858106003976,-48.187339359052));
#23812=CARTESIAN_POINT('Ctrl Pts',(4.29551799962782,-5.975553604426,-48.1843102337114));
#23813=CARTESIAN_POINT('Ctrl Pts',(4.29556841690132,-5.96458345048953,-48.1810704965239));
#23814=CARTESIAN_POINT('Ctrl Pts',(4.29566133560256,-5.95397176603299,-48.1785928137628));
#23815=CARTESIAN_POINT('Ctrl Pts',(4.29576766490672,-5.94395259925279,-48.1767350581682));
#23816=CARTESIAN_POINT('Ctrl Pts',(4.29588042424262,-5.93332754531067,-48.1747649588739));
#23817=CARTESIAN_POINT('Ctrl Pts',(4.29600813145345,-5.92336957191585,-48.1734904896102));
#23818=CARTESIAN_POINT('Ctrl Pts',(4.29611218230544,-5.91431731008256,-48.1726976486325));
#23819=CARTESIAN_POINT('Ctrl Pts',(4.29622934837405,-5.90412404486025,-48.1718048730462));
#23820=CARTESIAN_POINT('Ctrl Pts',(4.29631622615796,-5.89507967138156,-48.1715194405676));
#23821=CARTESIAN_POINT('Ctrl Pts',(4.29631622615797,-5.88746284406389,-48.1715194405676));
#23822=CARTESIAN_POINT('Ctrl Pts',(0.0835265683620358,-5.88746284406389,
-48.3550682080606));
#23823=CARTESIAN_POINT('Ctrl Pts',(0.0835265683561427,-5.90583775506839,
-48.3550682080606));
#23824=CARTESIAN_POINT('Ctrl Pts',(0.0835265683557651,-5.92795641804993,
-48.3506190569028));
#23825=CARTESIAN_POINT('Ctrl Pts',(0.0835265683536855,-5.96223275463528,
-48.3547237089017));
#23826=CARTESIAN_POINT('Ctrl Pts',(0.0835265683430974,-5.9853111687807,
-48.3550820175939));
#23827=CARTESIAN_POINT('Ctrl Pts',(0.0835265683425695,-6.00666333723547,
-48.3550824830876));
#23828=CARTESIAN_POINT('Ctrl Pts',(0.0835265683425695,-6.00666333723547,
-48.3550824830876));
#23829=CARTESIAN_POINT('Ctrl Pts',(-0.267518736531456,-6.00132529512168,
-48.3550823667144));
#23830=CARTESIAN_POINT('Ctrl Pts',(-0.618615979168657,-5.99973567328051,
-48.3536249385721));
#23831=CARTESIAN_POINT('Ctrl Pts',(-1.3209415423196,-5.99820579736957,-48.3438941182277));
#23832=CARTESIAN_POINT('Ctrl Pts',(-1.67216986283335,-5.9982655432998,-48.3356207260257));
#23833=CARTESIAN_POINT('Ctrl Pts',(-2.37478478408758,-5.99418693015785,
-48.3083566370402));
#23834=CARTESIAN_POINT('Ctrl Pts',(-2.72575170761495,-5.99381953117288,
-48.2907404707597));
#23835=CARTESIAN_POINT('Ctrl Pts',(-3.42730927262762,-5.99717808806743,
-48.2483101720868));
#23836=CARTESIAN_POINT('Ctrl Pts',(-3.77789991411291,-6.00090404394696,
-48.2234960396944));
#23837=CARTESIAN_POINT('Ctrl Pts',(-4.12845481065586,-6.007051447105,-48.1954680629781));
#23838=CARTESIAN_POINT('Ctrl Pts',(0.0835265683430974,-5.9853111687807,
-48.3550820175939));
#23839=CARTESIAN_POINT('Ctrl Pts',(-0.189662915929852,-5.98270666392052,
-48.3550223265528));
#23840=CARTESIAN_POINT('Ctrl Pts',(-0.485248141409092,-5.98152768121033,
-48.3538283041956));
#23841=CARTESIAN_POINT('Ctrl Pts',(-1.12790203322386,-5.97907559060103,
-48.3454622940202));
#23842=CARTESIAN_POINT('Ctrl Pts',(-1.47497921400774,-5.97774718230166,
-48.3381640344815));
#23843=CARTESIAN_POINT('Ctrl Pts',(-2.22731576275959,-5.97194742955333,
-48.3098281543727));
#23844=CARTESIAN_POINT('Ctrl Pts',(-2.60287727367722,-5.97081802552573,
-48.2910861014622));
#23845=CARTESIAN_POINT('Ctrl Pts',(-3.35965513436493,-5.97321241327177,
-48.2448130739282));
#23846=CARTESIAN_POINT('Ctrl Pts',(-3.74087148413501,-5.97673620504541,
-48.2172820993047));
#23847=CARTESIAN_POINT('Ctrl Pts',(-4.12834943621584,-5.98314272027373,
-48.1855363158243));
#23848=CARTESIAN_POINT('Ctrl Pts',(0.0835265683536855,-5.96223275463528,
-48.3547237089017));
#23849=CARTESIAN_POINT('Ctrl Pts',(-0.172476876219001,-5.9624068608033,
-48.3547580080132));
#23850=CARTESIAN_POINT('Ctrl Pts',(-0.459481328279409,-5.96239709811644,
-48.3533940028304));
#23851=CARTESIAN_POINT('Ctrl Pts',(-1.09571051584365,-5.96099214798698,
-48.3443038073375));
#23852=CARTESIAN_POINT('Ctrl Pts',(-1.44494172980739,-5.95954166014412,
-48.3364512936579));
#23853=CARTESIAN_POINT('Ctrl Pts',(-2.20580868414923,-5.95413393118492,
-48.3073282819866));
#23854=CARTESIAN_POINT('Ctrl Pts',(-2.58784945320871,-5.95257589046814,
-48.288009822339));
#23855=CARTESIAN_POINT('Ctrl Pts',(-3.35545842702323,-5.95314193699468,
-48.2403172933099));
#23856=CARTESIAN_POINT('Ctrl Pts',(-3.74102460739806,-5.955266024238,-48.2119434824327));
#23857=CARTESIAN_POINT('Ctrl Pts',(-4.12855150591032,-5.95992641567859,
-48.1795491602216));
#23858=CARTESIAN_POINT('Ctrl Pts',(0.0835265683557651,-5.92795641804993,
-48.3506190569028));
#23859=CARTESIAN_POINT('Ctrl Pts',(-0.194279273771221,-5.92787973562296,
-48.3505964244566));
#23860=CARTESIAN_POINT('Ctrl Pts',(-0.500506504822973,-5.92723732580271,
-48.3484833205473));
#23861=CARTESIAN_POINT('Ctrl Pts',(-1.16018842029139,-5.92511301754088,
-48.3372314657113));
#23862=CARTESIAN_POINT('Ctrl Pts',(-1.51364329259108,-5.92360346889918,
-48.3280294755334));
#23863=CARTESIAN_POINT('Ctrl Pts',(-2.25808685945314,-5.91998502842382,
-48.2988519283619));
#23864=CARTESIAN_POINT('Ctrl Pts',(-2.63432748028667,-5.91860436677903,
-48.2796807290063));
#23865=CARTESIAN_POINT('Ctrl Pts',(-3.38522478842194,-5.91737158402242,
-48.2324397032854));
#23866=CARTESIAN_POINT('Ctrl Pts',(-3.75987742960026,-5.91751946291059,
-48.2043703936481));
#23867=CARTESIAN_POINT('Ctrl Pts',(-4.12900833251928,-5.91876732373882,
-48.1725407225933));
#23868=CARTESIAN_POINT('Ctrl Pts',(0.0835265683561427,-5.90583775506839,
-48.3550682080606));
#23869=CARTESIAN_POINT('Ctrl Pts',(-0.233267711026719,-5.9058377550684,
-48.3550682080605));
#23870=CARTESIAN_POINT('Ctrl Pts',(-0.567298494489859,-5.90562906540037,
-48.3519505469246));
#23871=CARTESIAN_POINT('Ctrl Pts',(-1.25685784211514,-5.90495067814671,
-48.3377896456597));
#23872=CARTESIAN_POINT('Ctrl Pts',(-1.61238233957187,-5.90448098056109,
-48.3267463020468));
#23873=CARTESIAN_POINT('Ctrl Pts',(-2.33187211336571,-5.90343694889075,
-48.2961657002432));
#23874=CARTESIAN_POINT('Ctrl Pts',(-2.69583332783207,-5.90286261480602,
-48.2766286482999));
#23875=CARTESIAN_POINT('Ctrl Pts',(-3.41918785716212,-5.90176568155595,
-48.2296135008224));
#23876=CARTESIAN_POINT('Ctrl Pts',(-3.77857712853939,-5.9012430823906,-48.2021359217356));
#23877=CARTESIAN_POINT('Ctrl Pts',(-4.12926308943376,-5.90082453639418,
-48.1715194405676));
#23878=CARTESIAN_POINT('Ctrl Pts',(0.0835265683621219,-5.88746284406389,
-48.3550682080606));
#23879=CARTESIAN_POINT('Ctrl Pts',(-0.267760844335752,-5.88746284406389,
-48.3550682080606));
#23880=CARTESIAN_POINT('Ctrl Pts',(-0.619048262304891,-5.88746284406389,
-48.3512468523357));
#23881=CARTESIAN_POINT('Ctrl Pts',(-1.32154021141508,-5.88746284406389,
-48.3359596079612));
#23882=CARTESIAN_POINT('Ctrl Pts',(-1.67274475309905,-5.88746284406389,
-48.3244937189391));
#23883=CARTESIAN_POINT('Ctrl Pts',(-2.37498775707864,-5.88746284406389,
-48.2939119483841));
#23884=CARTESIAN_POINT('Ctrl Pts',(-2.72602622991902,-5.88746284406389,
-48.2747960661052));
#23885=CARTESIAN_POINT('Ctrl Pts',(-3.42785327106253,-5.88746284406389,
-48.2289052281065));
#23886=CARTESIAN_POINT('Ctrl Pts',(-3.77864184991366,-5.88746284406389,
-48.2021302712649));
#23887=CARTESIAN_POINT('Ctrl Pts',(-4.12926308943376,-5.88746284406389,
-48.1715194405676));
#23888=CARTESIAN_POINT('',(-4.12845481065586,-6.00705144710501,-48.1954680629781));
#23889=CARTESIAN_POINT('Origin',(-4.15507771262898,-5.88723161925855,-48.4841190147253));
#23890=CARTESIAN_POINT('Ctrl Pts',(-4.12845481065586,-6.00705144710501,
-48.1954680629781));
#23891=CARTESIAN_POINT('Ctrl Pts',(-3.42734501756996,-5.99475664078892,
-48.2515240164107));
#23892=CARTESIAN_POINT('Ctrl Pts',(-2.72609224471469,-5.99214762358689,
-48.2947245925476));
#23893=CARTESIAN_POINT('Ctrl Pts',(-1.32086240220623,-6.00030484987077,
-48.3492527705183));
#23894=CARTESIAN_POINT('Ctrl Pts',(-0.618564041405483,-5.99598725300791,
-48.3550822503411));
#23895=CARTESIAN_POINT('Ctrl Pts',(0.0835265683425695,-6.00666333723547,
-48.3550824830876));
#23896=CARTESIAN_POINT('Ctrl Pts',(27.6169432000905,-6.28105857414854,-39.6589503071862));
#23897=CARTESIAN_POINT('Ctrl Pts',(27.6725217924464,-6.09633085020215,-39.8274976919832));
#23898=CARTESIAN_POINT('Ctrl Pts',(27.4448729346656,-6.06008770502774,-39.939229356356));
#23899=CARTESIAN_POINT('Ctrl Pts',(28.3333834524819,-8.4789807742448,-41.8316237374642));
#23900=CARTESIAN_POINT('Ctrl Pts',(28.3922756330097,-8.30110493969029,-42.0102198945798));
#23901=CARTESIAN_POINT('Ctrl Pts',(28.1589136994597,-8.25800948638859,-42.1135427213873));
#23902=CARTESIAN_POINT('Ctrl Pts',(29.0478992516726,-10.6833293750564,-43.998461079774));
#23903=CARTESIAN_POINT('Ctrl Pts',(29.1067545955585,-10.5025148294077,-44.1769455263626));
#23904=CARTESIAN_POINT('Ctrl Pts',(28.8713287464266,-10.4623581523703,-44.2817497435117));
#23905=CARTESIAN_POINT('Ctrl Pts',(29.7611081292079,-12.8919045823054,-46.1613350574533));
#23906=CARTESIAN_POINT('Ctrl Pts',(29.8183400962187,-12.7034528674627,-46.3348964586614));
#23907=CARTESIAN_POINT('Ctrl Pts',(29.5826474545624,-12.6709337131846,-46.4458225157374));
#23908=CARTESIAN_POINT('Ctrl Pts',(27.4605785366061,-6.10843371318469,-39.9870540284924));
#23909=CARTESIAN_POINT('Ctrl Pts',(27.465458387645,-6.10756827058305,-39.982671765503));
#23910=CARTESIAN_POINT('Ctrl Pts',(27.470433835024,-6.10708538385355,-39.9783580051385));
#23911=CARTESIAN_POINT('Ctrl Pts',(27.475474250485,-6.10700426240367,-39.9741447883131));
#23912=CARTESIAN_POINT('Ctrl Pts',(27.4830348736764,-6.10688258022884,-39.967824963075));
#23913=CARTESIAN_POINT('Ctrl Pts',(27.4907409943993,-6.10766522922468,-39.9617312210474));
#23914=CARTESIAN_POINT('Ctrl Pts',(27.4984985962217,-6.10940561367496,-39.955980126062));
#23915=CARTESIAN_POINT('Ctrl Pts',(27.5023773971328,-6.11027580590009,-39.9531045785694));
#23916=CARTESIAN_POINT('Ctrl Pts',(27.5062692657206,-6.11138525201715,-39.9503148097033));
#23917=CARTESIAN_POINT('Ctrl Pts',(27.5101637009479,-6.1127398416781,-39.9476257773117));
#23918=CARTESIAN_POINT('Ctrl Pts',(27.5111373097547,-6.11307848909333,-39.9469535192137));
#23919=CARTESIAN_POINT('Ctrl Pts',(27.5121110832077,-6.11343245632765,-39.9462875574448));
#23920=CARTESIAN_POINT('Ctrl Pts',(27.5130848657175,-6.11380183251764,-39.9456281258756));
#23921=CARTESIAN_POINT('Ctrl Pts',(27.5145455394822,-6.11435589680261,-39.9446389785216));
#23922=CARTESIAN_POINT('Ctrl Pts',(27.5160062328241,-6.11494463135669,-39.9436645242677));
#23923=CARTESIAN_POINT('Ctrl Pts',(27.5174664350244,-6.11556833384706,-39.942705550843));
#23924=CARTESIAN_POINT('Ctrl Pts',(27.5189266372247,-6.11619203633743,-39.9417465774182));
#23925=CARTESIAN_POINT('Ctrl Pts',(27.5203863482847,-6.11685070666529,-39.9408030849329));
#23926=CARTESIAN_POINT('Ctrl Pts',(27.5218450747583,-6.11754464002833,-39.9398758577402));
#23927=CARTESIAN_POINT('Ctrl Pts',(27.5297560792404,-6.12130799802896,-39.9348472943937));
#23928=CARTESIAN_POINT('Ctrl Pts',(27.5374062985722,-6.12597258662812,-39.930411392287));
#23929=CARTESIAN_POINT('Ctrl Pts',(27.5447641973967,-6.13138771967645,-39.9265070394851));
#23930=CARTESIAN_POINT('Ctrl Pts',(27.5470542145033,-6.13307308497037,-39.9252918780757));
#23931=CARTESIAN_POINT('Ctrl Pts',(27.5493160954356,-6.13483149128261,-39.9241281566109));
#23932=CARTESIAN_POINT('Ctrl Pts',(27.5515493057335,-6.13665930617706,-39.9230139068561));
#23933=CARTESIAN_POINT('Ctrl Pts',(27.5527253791102,-6.13762188656503,-39.9224271105867));
#23934=CARTESIAN_POINT('Ctrl Pts',(27.5538933581835,-6.13860357319269,-39.9218540549599));
#23935=CARTESIAN_POINT('Ctrl Pts',(27.5550530642264,-6.13960373328463,-39.9212944500448));
#23936=CARTESIAN_POINT('Ctrl Pts',(27.5555765385631,-6.1400551909139,-39.9210418525753));
#23937=CARTESIAN_POINT('Ctrl Pts',(27.5560983353807,-6.14051040725671,-39.9207919716895));
#23938=CARTESIAN_POINT('Ctrl Pts',(27.5566184179837,-6.14096936706301,-39.9205448870854));
#23939=CARTESIAN_POINT('Ctrl Pts',(27.5571065033715,-6.14140009013226,-39.9203130039497));
#23940=CARTESIAN_POINT('Ctrl Pts',(27.557593149706,-6.14183402342711,-39.9200834930602));
#23941=CARTESIAN_POINT('Ctrl Pts',(27.5580783374539,-6.14227112540981,-39.9198564005236));
#23942=CARTESIAN_POINT('Ctrl Pts',(27.5650936167147,-6.14859113758576,-39.91657289312));
#23943=CARTESIAN_POINT('Ctrl Pts',(27.5718055899689,-6.15557322588934,-39.9137930036632));
#23944=CARTESIAN_POINT('Ctrl Pts',(27.5782114177422,-6.1630485902823,-39.9114693381554));
#23945=CARTESIAN_POINT('Ctrl Pts',(27.5839675375493,-6.16976576947769,-39.9093813492914));
#23946=CARTESIAN_POINT('Ctrl Pts',(27.5894017151405,-6.17677030338733,-39.9076507714992));
#23947=CARTESIAN_POINT('Ctrl Pts',(27.5945623304161,-6.18399336848785,-39.906237064347));
#23948=CARTESIAN_POINT('Ctrl Pts',(27.5969029162795,-6.18726937399527,-39.9055958805349));
#23949=CARTESIAN_POINT('Ctrl Pts',(27.599187113212,-6.19059093207268,-39.9050203362105));
#23950=CARTESIAN_POINT('Ctrl Pts',(27.6014189311488,-6.19395424178567,-39.9045087946084));
#23951=CARTESIAN_POINT('Ctrl Pts',(27.6041011626861,-6.19799631673864,-39.9038940164068));
#23952=CARTESIAN_POINT('Ctrl Pts',(27.6067075951069,-6.20209746439247,-39.9033697450797));
#23953=CARTESIAN_POINT('Ctrl Pts',(27.6092439514794,-6.20624978925052,-39.9029293953656));
#23954=CARTESIAN_POINT('Ctrl Pts',(27.6114632633054,-6.20988307350132,-39.9025440893657));
#23955=CARTESIAN_POINT('Ctrl Pts',(27.6136289069462,-6.21355555791224,-39.9022230232443));
#23956=CARTESIAN_POINT('Ctrl Pts',(27.6157440919799,-6.21726235805581,-39.9019615796143));
#23957=CARTESIAN_POINT('Ctrl Pts',(27.6219750132014,-6.22818186595202,-39.9011914178383));
#23958=CARTESIAN_POINT('Ctrl Pts',(27.6277878380593,-6.23942896207809,-39.9009317259755));
#23959=CARTESIAN_POINT('Ctrl Pts',(27.6332066390285,-6.25083884461389,-39.9010765586603));
#23960=CARTESIAN_POINT('Ctrl Pts',(27.6343122708321,-6.25316687420542,-39.9011061097775));
#23961=CARTESIAN_POINT('Ctrl Pts',(27.6354014986682,-6.2555018522693,-39.9011525316285));
#23962=CARTESIAN_POINT('Ctrl Pts',(27.6364745204553,-6.25784263179033,-39.9012149693086));
#23963=CARTESIAN_POINT('Ctrl Pts',(27.6426392228307,-6.27129082943956,-39.9015736849657));
#23964=CARTESIAN_POINT('Ctrl Pts',(27.6483061366112,-6.28489536287214,-39.9024185375791));
#23965=CARTESIAN_POINT('Ctrl Pts',(27.6535535090021,-6.2985815443386,-39.903595289237));
#23966=CARTESIAN_POINT('Ctrl Pts',(27.6574502388027,-6.30874498371449,-39.9044691519842));
#23967=CARTESIAN_POINT('Ctrl Pts',(27.6611206154207,-6.31897515336467,-39.9055604607672));
#23968=CARTESIAN_POINT('Ctrl Pts',(27.6645917831624,-6.32926010582614,-39.9068416997379));
#23969=CARTESIAN_POINT('Ctrl Pts',(27.670418092268,-6.34652326238773,-39.9089922423901));
#23970=CARTESIAN_POINT('Ctrl Pts',(27.675680571127,-6.36392973947355,-39.9116755677516));
#23971=CARTESIAN_POINT('Ctrl Pts',(27.6804674646178,-6.38139910649553,-39.9147853711119));
#23972=CARTESIAN_POINT('Ctrl Pts',(27.6857545369784,-6.40069383442647,-39.9182201154663));
#23973=CARTESIAN_POINT('Ctrl Pts',(27.690461568716,-6.42006561689591,-39.9221751468457));
#23974=CARTESIAN_POINT('Ctrl Pts',(27.6946812503251,-6.43945161623791,-39.9265477081944));
#23975=CARTESIAN_POINT('Ctrl Pts',(27.6991993449422,-6.46020858024372,-39.9312294941022));
#23976=CARTESIAN_POINT('Ctrl Pts',(27.7031587031065,-6.48098271066482,-39.9363903152504));
#23977=CARTESIAN_POINT('Ctrl Pts',(27.7066438148032,-6.50173650935267,-39.9419447801428));
#23978=CARTESIAN_POINT('Ctrl Pts',(27.7105819510236,-6.52518806368856,-39.9482212617253));
#23979=CARTESIAN_POINT('Ctrl Pts',(27.7139148163436,-6.54861499428405,-39.9550006703093));
#23980=CARTESIAN_POINT('Ctrl Pts',(27.7167256519374,-6.57199467982627,-39.9622052700919));
#23981=CARTESIAN_POINT('Ctrl Pts',(27.7176622649425,-6.57978514525988,-39.9646059518919));
#23982=CARTESIAN_POINT('Ctrl Pts',(27.7185406109312,-6.58757049922583,-39.9670541566905));
#23983=CARTESIAN_POINT('Ctrl Pts',(27.7193629006997,-6.59535009141639,-39.9695478224821));
#23984=CARTESIAN_POINT('Origin',(29.4643271522699,-12.8919045823054,-46.2591987469795));
#23985=CARTESIAN_POINT('Ctrl Pts',(30.3297286714007,-13.2959337131847,-46.7096495545262));
#23986=CARTESIAN_POINT('Ctrl Pts',(30.2800412871707,-13.2044045823055,-46.63278118881));
#23987=CARTESIAN_POINT('Ctrl Pts',(30.2097727145138,-13.2044045823055,-46.5240729034967));
#23988=CARTESIAN_POINT('Ctrl Pts',(30.2480070382537,-13.2959337183949,-46.7624740763582));
#23989=CARTESIAN_POINT('Ctrl Pts',(30.2237821295074,-13.2092798238967,-46.6749519433113));
#23990=CARTESIAN_POINT('Ctrl Pts',(30.1727791352342,-13.2044045823055,-46.5621348913443));
#23991=CARTESIAN_POINT('Ctrl Pts',(30.1557802945293,-13.2734166054796,-46.7949451596591));
#23992=CARTESIAN_POINT('Ctrl Pts',(30.1567362919807,-13.1931723515309,-46.698954204891));
#23993=CARTESIAN_POINT('Ctrl Pts',(30.1272434959976,-13.1931460297457,-46.5790211908226));
#23994=CARTESIAN_POINT('Ctrl Pts',(29.9810497702099,-13.1901047283842,-46.8078019025926));
#23995=CARTESIAN_POINT('Ctrl Pts',(30.0332579895645,-13.1260474868728,-46.6985032563468));
#23996=CARTESIAN_POINT('Ctrl Pts',(30.0334560808361,-13.1514900886123,-46.5650271793139));
#23997=CARTESIAN_POINT('Ctrl Pts',(29.9021671260579,-13.1321577745916,-46.7892918780939));
#23998=CARTESIAN_POINT('Ctrl Pts',(29.9785578442827,-13.0767072102091,-46.6749582903023));
#23999=CARTESIAN_POINT('Ctrl Pts',(29.9874804360701,-13.1225166214135,-46.535607917148));
#24000=CARTESIAN_POINT('Ctrl Pts',(29.7068169519706,-12.9456232578403,-46.6923959077902));
#24001=CARTESIAN_POINT('Ctrl Pts',(29.850736282044,-12.917759331099,-46.5682098335491));
#24002=CARTESIAN_POINT('Ctrl Pts',(29.8659898138072,-13.0292493378241,-46.4142407544751));
#24003=CARTESIAN_POINT('Ctrl Pts',(29.6248993528429,-12.802121823431,-46.5743671996335));
#24004=CARTESIAN_POINT('Ctrl Pts',(29.8160663686883,-12.7965826300651,-46.4467809431966));
#24005=CARTESIAN_POINT('Ctrl Pts',(29.8034597078097,-12.957479090352,-46.2897702608793));
#24006=CARTESIAN_POINT('Ctrl Pts',(29.5826474545624,-12.6709337131846,-46.4458225157374));
#24007=CARTESIAN_POINT('Ctrl Pts',(29.8183400962187,-12.7034528674627,-46.3348964586614));
#24008=CARTESIAN_POINT('Ctrl Pts',(29.7611081292079,-12.8919045823054,-46.1613350574533));
#24009=CARTESIAN_POINT('Origin',(30.2097727145137,-13.5169045823054,-46.5240729034966));
#24010=CARTESIAN_POINT('Ctrl Pts',(29.7611081292079,-12.8919045823054,-46.1613350574533));
#24011=CARTESIAN_POINT('Ctrl Pts',(29.7689446056648,-12.9040380872524,-46.1850999200892));
#24012=CARTESIAN_POINT('Ctrl Pts',(29.7774029552135,-12.9162817766924,-46.2085325222876));
#24013=CARTESIAN_POINT('Ctrl Pts',(29.7865325971137,-12.9286427508496,-46.2316011837146));
#24014=CARTESIAN_POINT('Ctrl Pts',(29.7946239763792,-12.9395979811959,-46.2520463765046));
#24015=CARTESIAN_POINT('Ctrl Pts',(29.803243400554,-12.9506462200838,-46.2722072543535));
#24016=CARTESIAN_POINT('Ctrl Pts',(29.8124568466866,-12.9617976021851,-46.2920436345019));
#24017=CARTESIAN_POINT('Ctrl Pts',(29.820976079617,-12.972108751808,-46.3103853863879));
#24018=CARTESIAN_POINT('Ctrl Pts',(29.8300034908812,-12.9825085406178,-46.3284505844458));
#24019=CARTESIAN_POINT('Ctrl Pts',(29.8396134313692,-12.9930011868745,-46.3461752269231));
#24020=CARTESIAN_POINT('Ctrl Pts',(29.8486149610157,-13.0028295376813,-46.3627777121238));
#24021=CARTESIAN_POINT('Ctrl Pts',(29.8581277574155,-13.0127396637205,-46.3790820278025));
#24022=CARTESIAN_POINT('Ctrl Pts',(29.8682301303537,-13.0227264646583,-46.3949958588203));
#24023=CARTESIAN_POINT('Ctrl Pts',(29.8775297079321,-13.031919654283,-46.4096450810401));
#24024=CARTESIAN_POINT('Ctrl Pts',(29.8873290303633,-13.0411779829383,-46.4239636984746));
#24025=CARTESIAN_POINT('Ctrl Pts',(29.8977020867377,-13.0504868885806,-46.4378390387971));
#24026=CARTESIAN_POINT('Ctrl Pts',(29.9030617551183,-13.0552967194953,-46.4450083069581));
#24027=CARTESIAN_POINT('Ctrl Pts',(29.9085747980936,-13.0601198606037,-46.4520585243));
#24028=CARTESIAN_POINT('Ctrl Pts',(29.9142527689337,-13.0649528255951,-46.4589689296633));
#24029=CARTESIAN_POINT('Ctrl Pts',(29.9228757513932,-13.0722925202715,-46.4694635774722));
#24030=CARTESIAN_POINT('Ctrl Pts',(29.9318251137018,-13.0796093213738,-46.4795773572471));
#24031=CARTESIAN_POINT('Ctrl Pts',(29.9411925883594,-13.086931462929,-46.4892853924893));
#24032=CARTESIAN_POINT('Ctrl Pts',(29.9431045819531,-13.0884259839454,-46.4912668978437));
#24033=CARTESIAN_POINT('Ctrl Pts',(29.9450340495387,-13.0899206854315,-46.4932313419366));
#24034=CARTESIAN_POINT('Ctrl Pts',(29.9469818564132,-13.0914157380931,-46.4951782578757));
#24035=CARTESIAN_POINT('Ctrl Pts',(29.9549256601176,-13.0975130596637,-46.5031184280495));
#24036=CARTESIAN_POINT('Ctrl Pts',(29.9632075915649,-13.1036283475447,-46.5107647600667));
#24037=CARTESIAN_POINT('Ctrl Pts',(29.9718588309488,-13.109735216012,-46.518012937061));
#24038=CARTESIAN_POINT('Ctrl Pts',(29.980031801798,-13.11550447701,-46.5248604113539));
#24039=CARTESIAN_POINT('Ctrl Pts',(29.9885346137173,-13.1212664690673,-46.5313529626109));
#24040=CARTESIAN_POINT('Ctrl Pts',(29.9973930117943,-13.1269828032032,-46.5373614305493));
#24041=CARTESIAN_POINT('Ctrl Pts',(30.0055746904732,-13.1322624495583,-46.5429108937362));
#24042=CARTESIAN_POINT('Ctrl Pts',(30.0140598659004,-13.1375032622592,-46.548047569981));
#24043=CARTESIAN_POINT('Ctrl Pts',(30.0228656315125,-13.1426584957574,-46.5526298236939));
#24044=CARTESIAN_POINT('Ctrl Pts',(30.0295253896781,-13.1465573740489,-46.5560953601305));
#24045=CARTESIAN_POINT('Ctrl Pts',(30.0363684855418,-13.1504070236379,-46.5592430884801));
#24046=CARTESIAN_POINT('Ctrl Pts',(30.0434000451071,-13.1541794056116,-46.5619934529432));
#24047=CARTESIAN_POINT('Ctrl Pts',(30.0550572816468,-13.1604334305654,-46.5665531311794));
#24048=CARTESIAN_POINT('Ctrl Pts',(30.0674459465525,-13.1665823184279,-46.570124885838));
#24049=CARTESIAN_POINT('Ctrl Pts',(30.0803549315343,-13.1723138052614,-46.572067420129));
#24050=CARTESIAN_POINT('Ctrl Pts',(30.089601156449,-13.1764190557078,-46.5734587850569));
#24051=CARTESIAN_POINT('Ctrl Pts',(30.0990247132506,-13.180252986557,-46.5739543522569));
#24052=CARTESIAN_POINT('Ctrl Pts',(30.1084980236264,-13.1837286680714,-46.5734464756373));
#24053=CARTESIAN_POINT('Ctrl Pts',(30.115560834798,-13.186319956782,-46.573067829048));
#24054=CARTESIAN_POINT('Ctrl Pts',(30.122650932996,-13.1887123032027,-46.5721323870867));
#24055=CARTESIAN_POINT('Ctrl Pts',(30.1297115805048,-13.1908748315003,-46.5706133212394));
#24056=CARTESIAN_POINT('Ctrl Pts',(30.1379679083212,-13.1934035716073,-46.5688370102715));
#24057=CARTESIAN_POINT('Ctrl Pts',(30.1461053622757,-13.1955933528871,-46.5662741485632));
#24058=CARTESIAN_POINT('Ctrl Pts',(30.1540188210239,-13.1974205800258,-46.5629748938067));
#24059=CARTESIAN_POINT('Ctrl Pts',(30.1619718333917,-13.1992569401429,-46.5596591484774));
#24060=CARTESIAN_POINT('Ctrl Pts',(30.1696981454544,-13.2007270768473,-46.5555998526813));
#24061=CARTESIAN_POINT('Ctrl Pts',(30.1771066956215,-13.2018302796858,-46.5508928619014));
#24062=CARTESIAN_POINT('Ctrl Pts',(30.1846349929034,-13.2029513139965,-46.5461097903023));
#24063=CARTESIAN_POINT('Ctrl Pts',(30.1918347533013,-13.2036934504427,-46.5406581808445));
#24064=CARTESIAN_POINT('Ctrl Pts',(30.1986333530818,-13.2040802847478,-46.5346813319021));
#24065=CARTESIAN_POINT('Ctrl Pts',(30.2024773666742,-13.204299005716,-46.531301946541));
#24066=CARTESIAN_POINT('Ctrl Pts',(30.2061935878781,-13.2044045823055,-46.5277553985989));
#24067=CARTESIAN_POINT('Ctrl Pts',(30.2097727145138,-13.2044045823055,-46.5240729034967));
#24068=CARTESIAN_POINT('Ctrl Pts',(27.4605785366061,-6.10843371318469,-39.9870540284924));
#24069=CARTESIAN_POINT('Ctrl Pts',(27.4089435087152,-6.01690458230549,-39.9114801858336));
#24070=CARTESIAN_POINT('Ctrl Pts',(27.4089435087152,-5.8874628440639,-39.9114801858336));
#24071=CARTESIAN_POINT('Ctrl Pts',(27.4926254958792,-6.10275018345573,-39.9582748359069));
#24072=CARTESIAN_POINT('Ctrl Pts',(27.457094436975,-6.01222811249993,-39.8785815735222));
#24073=CARTESIAN_POINT('Ctrl Pts',(27.4761172860278,-5.88746285448466,-39.8655844136585));
#24074=CARTESIAN_POINT('Ctrl Pts',(27.5262766366667,-6.11419577460873,-39.9349635041551));
#24075=CARTESIAN_POINT('Ctrl Pts',(27.5056815629761,-6.02882146164738,-39.8452613916108));
#24076=CARTESIAN_POINT('Ctrl Pts',(27.5432762945934,-5.91065570868296,-39.8194267690275));
#24077=CARTESIAN_POINT('Ctrl Pts',(27.5869602346596,-6.16774318631796,-39.9061265671302));
#24078=CARTESIAN_POINT('Ctrl Pts',(27.583668943987,-6.09780352750744,-39.7916619276919));
#24079=CARTESIAN_POINT('Ctrl Pts',(27.6568986769456,-5.99623773973461,-39.7409950094831));
#24080=CARTESIAN_POINT('Ctrl Pts',(27.6142659702345,-6.20950986590629,-39.9002511491957));
#24081=CARTESIAN_POINT('Ctrl Pts',(27.6140401210967,-6.15046547604275,-39.7707310218534));
#24082=CARTESIAN_POINT('Ctrl Pts',(27.7041874632732,-6.05824038173977,-39.7081745064884));
#24083=CARTESIAN_POINT('Ctrl Pts',(27.6808991139987,-6.3546301407073,-39.9034964109337));
#24084=CARTESIAN_POINT('Ctrl Pts',(27.6737052370323,-6.32861804115438,-39.7296612449018));
#24085=CARTESIAN_POINT('Ctrl Pts',(27.8101683547685,-6.26685602924678,-39.6344682377825));
#24086=CARTESIAN_POINT('Ctrl Pts',(27.7067660427821,-6.47617237885483,-39.9313466488163));
#24087=CARTESIAN_POINT('Ctrl Pts',(27.6709846760168,-6.47276044373897,-39.7316943091956));
#24088=CARTESIAN_POINT('Ctrl Pts',(27.8370886911753,-6.43425950785912,-39.61556810409));
#24089=CARTESIAN_POINT('Ctrl Pts',(27.7193629372986,-6.59535043767467,-39.9695479334715));
#24090=CARTESIAN_POINT('Ctrl Pts',(27.6465610575461,-6.59535043767467,-39.7487692861459));
#24091=CARTESIAN_POINT('Ctrl Pts',(27.83708867484,-6.59535043767467,-39.6155681155102));
#24092=CARTESIAN_POINT('Origin',(27.5852365212336,-5.88746284406389,-40.1695054243999));
#24093=CARTESIAN_POINT('Origin',(28.0161439142367,-6.59535043767467,-39.8716842439453));
#24094=CARTESIAN_POINT('Origin',(0.0835265683620477,-13.5169045823054,0.0824317919394229));
#24095=CARTESIAN_POINT('Origin',(31.5582959274376,-13.5169045823054,-45.624196617704));
#24096=CARTESIAN_POINT('Origin',(13.3939389642122,-12.8919045823054,4.47154756213422));
#24097=CARTESIAN_POINT('Origin',(28.0161439142367,-12.8919045823054,-39.8716842439453));
#24098=CARTESIAN_POINT('Origin',(28.0161439142367,-14.7669045823054,-39.8716842439453));
#24099=CARTESIAN_POINT('Origin',(28.0161439142367,-12.8919045823054,-39.8716842439453));
#24100=CARTESIAN_POINT('Origin',(0.0835265683620477,-5.88746284406389,0.0824317919394229));
#24101=CARTESIAN_POINT('Ctrl Pts',(30.5401339447129,-14.9741386829693,-48.3550682080606));
#24102=CARTESIAN_POINT('Ctrl Pts',(30.6141174651452,-14.8357920829899,-48.3550682080606));
#24103=CARTESIAN_POINT('Ctrl Pts',(30.6583146466958,-14.7531448966913,-48.229253285411));
#24104=CARTESIAN_POINT('Ctrl Pts',(28.492829280589,-13.8793029116944,-48.3550682080606));
#24105=CARTESIAN_POINT('Ctrl Pts',(28.5700753356058,-13.7458678866727,-48.3550682080606));
#24106=CARTESIAN_POINT('Ctrl Pts',(28.6053355619279,-13.6583075326732,-48.232843582883));
#24107=CARTESIAN_POINT('Ctrl Pts',(26.4097780451804,-12.8434482903031,-48.3550682080606));
#24108=CARTESIAN_POINT('Ctrl Pts',(26.4826847058204,-12.7103751542466,-48.3550682080606));
#24109=CARTESIAN_POINT('Ctrl Pts',(26.5160221214703,-12.6224528665269,-48.2364507688974));
#24110=CARTESIAN_POINT('Ctrl Pts',(23.213550958804,-11.4077451872907,-48.3550682080606));
#24111=CARTESIAN_POINT('Ctrl Pts',(23.2738757441258,-11.2735898053145,-48.3550682080606));
#24112=CARTESIAN_POINT('Ctrl Pts',(23.3093293343021,-11.1867499400307,-48.2417141569431));
#24113=CARTESIAN_POINT('Ctrl Pts',(22.1361415983178,-10.9489604127289,-48.3550682080606));
#24114=CARTESIAN_POINT('Ctrl Pts',(22.1939919164413,-10.8151504288131,-48.3550682080606));
#24115=CARTESIAN_POINT('Ctrl Pts',(22.2282518962435,-10.7279650272959,-48.2434431037797));
#24116=CARTESIAN_POINT('Ctrl Pts',(19.9534411816293,-10.0773547210516,-48.3550682080606));
#24117=CARTESIAN_POINT('Ctrl Pts',(20.0062495694822,-9.94441815656816,-48.3550682080606));
#24118=CARTESIAN_POINT('Ctrl Pts',(20.0378275778654,-9.85635900888071,-48.2468078474917));
#24119=CARTESIAN_POINT('Ctrl Pts',(18.8490684843153,-9.66512413195019,-48.3550682080606));
#24120=CARTESIAN_POINT('Ctrl Pts',(18.8991406427071,-9.5324655645878,-48.3550682080606));
#24121=CARTESIAN_POINT('Ctrl Pts',(18.9294012091805,-9.44412830208801,-48.2484415699068));
#24122=CARTESIAN_POINT('Ctrl Pts',(13.3105934045374,-7.75733423685904,-48.3550682080606));
#24123=CARTESIAN_POINT('Ctrl Pts',(13.3719143129995,-7.63508483860106,-48.3550682080606));
#24124=CARTESIAN_POINT('Ctrl Pts',(13.3698756070365,-7.53633525782184,-48.2561639741704));
#24125=CARTESIAN_POINT('Ctrl Pts',(8.78203978180937,-6.70462823795841,-48.3550682080606));
#24126=CARTESIAN_POINT('Ctrl Pts',(8.81311496927653,-6.57519149763133,-48.3550682080606));
#24127=CARTESIAN_POINT('Ctrl Pts',(8.82176014815773,-6.48363668556399,-48.2609639163927));
#24128=CARTESIAN_POINT('Ctrl Pts',(4.11624754821277,-6.31501530004509,-48.3550682080606));
#24129=CARTESIAN_POINT('Ctrl Pts',(4.12707394707883,-6.18536424665212,-48.3550682080606));
#24130=CARTESIAN_POINT('Ctrl Pts',(4.13470171397579,-6.09401826675045,-48.2627408790281));
#24131=CARTESIAN_POINT('Ctrl Pts',(30.5121796307589,-14.6753754514262,-48.2295435588551));
#24132=CARTESIAN_POINT('Ctrl Pts',(30.4851371197009,-14.6690808662602,-48.2391368684286));
#24133=CARTESIAN_POINT('Ctrl Pts',(30.4577982704948,-14.6627210376773,-48.2478016524146));
#24134=CARTESIAN_POINT('Ctrl Pts',(30.4302713467175,-14.6563210590023,-48.2557044117279));
#24135=CARTESIAN_POINT('Ctrl Pts',(30.4010697645148,-14.6495317241356,-48.2640879520604));
#24136=CARTESIAN_POINT('Ctrl Pts',(30.3716560750817,-14.6426970987334,-48.2716137426758));
#24137=CARTESIAN_POINT('Ctrl Pts',(30.3421145822481,-14.6358367158202,-48.2784438176708));
#24138=CARTESIAN_POINT('Ctrl Pts',(30.3092090732797,-14.6281951117635,-48.2860516625169));
#24139=CARTESIAN_POINT('Ctrl Pts',(30.2761445940227,-14.6205214533656,-48.292796328517));
#24140=CARTESIAN_POINT('Ctrl Pts',(30.2429899455176,-14.6128317093194,-48.2988585238745));
#24141=CARTESIAN_POINT('Ctrl Pts',(30.2062238617915,-14.6043043447963,-48.3055810557705));
#24142=CARTESIAN_POINT('Ctrl Pts',(30.1693457982678,-14.5957569385231,-48.3114640731145));
#24143=CARTESIAN_POINT('Ctrl Pts',(30.1324060630064,-14.587201298653,-48.3167055873355));
#24144=CARTESIAN_POINT('Ctrl Pts',(30.1041689095605,-14.5806612703033,-48.3207122603747));
#24145=CARTESIAN_POINT('Ctrl Pts',(30.0758945614216,-14.5741161640292,-48.3243429309501));
#24146=CARTESIAN_POINT('Ctrl Pts',(30.0475982203807,-14.5675696486119,-48.3276721877859));
#24147=CARTESIAN_POINT('Ctrl Pts',(30.0447146594573,-14.5669025208015,-48.3280114583263));
#24148=CARTESIAN_POINT('Ctrl Pts',(30.0418299490014,-14.5662351623918,-48.3283473948448));
#24149=CARTESIAN_POINT('Ctrl Pts',(30.0389439896954,-14.5655675503514,-48.3286800185805));
#24150=CARTESIAN_POINT('Ctrl Pts',(29.9436377737461,-14.5435202618948,-48.3396646189221));
#24151=CARTESIAN_POINT('Ctrl Pts',(29.8480280991363,-14.5214458554098,-48.3469207097561));
#24152=CARTESIAN_POINT('Ctrl Pts',(29.7521618054431,-14.4993564117025,-48.3509992918687));
#24153=CARTESIAN_POINT('Ctrl Pts',(29.6871620963625,-14.4843792246285,-48.3537646710292));
#24154=CARTESIAN_POINT('Ctrl Pts',(29.622044134505,-14.4693950374107,-48.3550680832409));
#24155=CARTESIAN_POINT('Ctrl Pts',(29.5568194237311,-14.454406734056,-48.3550682080516));
#24156=CARTESIAN_POINT('Ctrl Pts',(-30.4912134104872,-14.7531486984911,
-48.2292882301095));
#24157=CARTESIAN_POINT('Ctrl Pts',(-30.4470156710373,-14.8357969973015,
-48.3550682080606));
#24158=CARTESIAN_POINT('Ctrl Pts',(-30.373045062923,-14.9741195676119,-48.3550682080606));
#24159=CARTESIAN_POINT('Ctrl Pts',(-28.4387348231413,-13.6585793127108,
-48.2328767825385));
#24160=CARTESIAN_POINT('Ctrl Pts',(-28.4034671513468,-13.7461362596467,
-48.3550682080606));
#24161=CARTESIAN_POINT('Ctrl Pts',(-28.3262370698434,-13.8795503180506,
-48.3550682080606));
#24162=CARTESIAN_POINT('Ctrl Pts',(-26.3501996831797,-12.6231097579334,
-48.2364817168271));
#24163=CARTESIAN_POINT('Ctrl Pts',(-26.3168499742945,-12.7110265271844,
-48.3550682080606));
#24164=CARTESIAN_POINT('Ctrl Pts',(-26.243961294676,-12.8440806269501,-48.3550682080606));
#24165=CARTESIAN_POINT('Ctrl Pts',(-23.145314529641,-11.1881005852606,-48.2417410418288));
#24166=CARTESIAN_POINT('Ctrl Pts',(-23.1098551901269,-11.2749369501014,
-48.3550682080606));
#24167=CARTESIAN_POINT('Ctrl Pts',(-23.0495359459671,-11.4090714544335,
-48.3550682080606));
#24168=CARTESIAN_POINT('Ctrl Pts',(-22.0649478906704,-10.7295656511252,
-48.2434685231326));
#24169=CARTESIAN_POINT('Ctrl Pts',(-22.0306807474001,-10.8167469967119,
-48.3550682080606));
#24170=CARTESIAN_POINT('Ctrl Pts',(-21.9728343771648,-10.9505365201866,
-48.3550682080606));
#24171=CARTESIAN_POINT('Ctrl Pts',(-19.8762142444861,-9.85847188921458,
-48.246830209952));
#24172=CARTESIAN_POINT('Ctrl Pts',(-19.844626683273,-9.94652588376056,-48.3550682080606));
#24173=CARTESIAN_POINT('Ctrl Pts',(-19.7918171438271,-10.0794427583948,
-48.3550682080606));
#24174=CARTESIAN_POINT('Ctrl Pts',(-18.7666798697007,-9.44570717935272,
-48.2484654765336));
#24175=CARTESIAN_POINT('Ctrl Pts',(-18.7364165373226,-9.53404162556794,
-48.3550682080606));
#24176=CARTESIAN_POINT('Ctrl Pts',(-18.6863395540866,-9.66667804843006,
-48.3550682080606));
#24177=CARTESIAN_POINT('Ctrl Pts',(-13.2023926152288,-7.53595817693426,
-48.2561934845101));
#24178=CARTESIAN_POINT('Ctrl Pts',(-13.2044686097622,-7.63471881015605,
-48.3550682080606));
#24179=CARTESIAN_POINT('Ctrl Pts',(-13.1431103220519,-7.7569290462289,-48.3550682080606));
#24180=CARTESIAN_POINT('Ctrl Pts',(-8.6526970032033,-6.4835029201157,-48.2609915525571));
#24181=CARTESIAN_POINT('Ctrl Pts',(-8.64404384437381,-6.57505277908091,
-48.3550682080606));
#24182=CARTESIAN_POINT('Ctrl Pts',(-8.61298834195424,-6.70446830382948,
-48.3550682080606));
#24183=CARTESIAN_POINT('Ctrl Pts',(-3.96771901147946,-6.09405046754031,
-48.2627672936114));
#24184=CARTESIAN_POINT('Ctrl Pts',(-3.96009147509235,-6.18539206100947,
-48.3550682080606));
#24185=CARTESIAN_POINT('Ctrl Pts',(-3.94926670206929,-6.31502133666111,
-48.3550682080606));
#24186=CARTESIAN_POINT('Ctrl Pts',(-29.3897661934246,-14.4544067125512,
-48.3550682080518));
#24187=CARTESIAN_POINT('Ctrl Pts',(-29.4762602452486,-14.474282601133,-48.3550680438326));
#24188=CARTESIAN_POINT('Ctrl Pts',(-29.5625289546745,-14.4941426280479,
-48.3527732539111));
#24189=CARTESIAN_POINT('Ctrl Pts',(-29.6485434749624,-14.5139794995301,
-48.3478250805349));
#24190=CARTESIAN_POINT('Ctrl Pts',(-29.7231251977381,-14.5311797122927,
-48.3435346038368));
#24191=CARTESIAN_POINT('Ctrl Pts',(-29.7975156566768,-14.548362486812,-48.3372488058751));
#24192=CARTESIAN_POINT('Ctrl Pts',(-29.8716853835464,-14.5655203189317,
-48.3287039250806));
#24193=CARTESIAN_POINT('Ctrl Pts',(-29.8750081603114,-14.566288983565,-48.3283211175314));
#24194=CARTESIAN_POINT('Ctrl Pts',(-29.8783295511836,-14.5670573738946,
-48.3279338770541));
#24195=CARTESIAN_POINT('Ctrl Pts',(-29.8816496610406,-14.5678255143184,
-48.3275421732212));
#24196=CARTESIAN_POINT('Ctrl Pts',(-29.921364211269,-14.5770138703543,-48.3228566832171));
#24197=CARTESIAN_POINT('Ctrl Pts',(-29.961084755409,-14.5862107044419,-48.3175899444853));
#24198=CARTESIAN_POINT('Ctrl Pts',(-30.0007382034786,-14.5953989044396,
-48.3115102233366));
#24199=CARTESIAN_POINT('Ctrl Pts',(-30.0367071665706,-14.6037333631736,
-48.3059954124878));
#24200=CARTESIAN_POINT('Ctrl Pts',(-30.0726218123948,-14.6120609299876,
-48.2998121059003));
#24201=CARTESIAN_POINT('Ctrl Pts',(-30.108407457618,-14.6203642532744,-48.2927569262129));
#24202=CARTESIAN_POINT('Ctrl Pts',(-30.1417601067399,-14.6281030498338,
-48.2861814144082));
#24203=CARTESIAN_POINT('Ctrl Pts',(-30.175001269215,-14.6358209223577,-48.2788488663937));
#24204=CARTESIAN_POINT('Ctrl Pts',(-30.2080423754229,-14.6434973280408,
-48.2705618313201));
#24205=CARTESIAN_POINT('Ctrl Pts',(-30.2384940192198,-14.6505721266275,
-48.2629242589397));
#24206=CARTESIAN_POINT('Ctrl Pts',(-30.2687760027118,-14.6576117669138,
-48.2544760489632));
#24207=CARTESIAN_POINT('Ctrl Pts',(-30.2987888272563,-14.6645931621405,
-48.2450311446474));
#24208=CARTESIAN_POINT('Ctrl Pts',(-30.3143131643305,-14.6682043361767,
-48.2401457038248));
#24209=CARTESIAN_POINT('Ctrl Pts',(-30.3297649549302,-14.6717998028493,
-48.2349930527964));
#24210=CARTESIAN_POINT('Ctrl Pts',(-30.3451264940351,-14.6753754514261,
-48.2295435588555));
#24211=CARTESIAN_POINT('Ctrl Pts',(-4.13722355950312,-6.10843371319295,
-48.2627017454154));
#24212=CARTESIAN_POINT('Ctrl Pts',(-4.13366090217496,-6.10843410331483,
-48.2630131843227));
#24213=CARTESIAN_POINT('Ctrl Pts',(-4.13160726137051,-6.12223873054887,
-48.2774222205278));
#24214=CARTESIAN_POINT('Ctrl Pts',(-4.12818752330401,-6.16064820739695,
-48.306533073772));
#24215=CARTESIAN_POINT('Ctrl Pts',(-4.12682927344009,-6.1854892637356,-48.3210576919346));
#24216=CARTESIAN_POINT('Ctrl Pts',(-4.1255125788106,-6.20946968450871,-48.331053858379));
#24217=CARTESIAN_POINT('Origin',(-44.291473431638,-14.4544045823054,-48.6675682080606));
#24218=CARTESIAN_POINT('Origin',(-29.3897569232175,-14.4544045823054,-48.6675682080606));
#24219=CARTESIAN_POINT('Origin',(29.5568100599416,-14.4544045823054,-48.6675682080606));
#24220=CARTESIAN_POINT('Ctrl Pts',(29.5568100599416,-14.7669045823054,-48.6675682080606));
#24221=CARTESIAN_POINT('Ctrl Pts',(29.5568100599416,-14.7669045823054,-48.3550682080606));
#24222=CARTESIAN_POINT('Ctrl Pts',(29.5568100599416,-14.4544045823054,-48.3550682080606));
#24223=CARTESIAN_POINT('Ctrl Pts',(29.7424051118639,-14.7669045823054,-48.6675682065036));
#24224=CARTESIAN_POINT('Ctrl Pts',(29.7130820249225,-14.7669045823054,-48.3909786805563));
#24225=CARTESIAN_POINT('Ctrl Pts',(29.7225178757419,-14.4924833818637,-48.3550682080606));
#24226=CARTESIAN_POINT('Ctrl Pts',(29.9261186112019,-14.7669045823054,-48.65073395611));
#24227=CARTESIAN_POINT('Ctrl Pts',(29.885222340593,-14.7669045823054,-48.4094018403383));
#24228=CARTESIAN_POINT('Ctrl Pts',(29.88629202078,-14.5302495546685,-48.3466510766381));
#24229=CARTESIAN_POINT('Ctrl Pts',(30.2885287859832,-14.7669045823054,-48.5748131378707));
#24230=CARTESIAN_POINT('Ctrl Pts',(30.2267587801975,-14.7669045823054,-48.3980269109194));
#24231=CARTESIAN_POINT('Ctrl Pts',(30.2089038710123,-14.6048828507185,-48.3086906784128));
#24232=CARTESIAN_POINT('Ctrl Pts',(30.4709665311741,-14.7669045823054,-48.5166482630913));
#24233=CARTESIAN_POINT('Ctrl Pts',(30.4029958016937,-14.7669045823061,-48.373227132016));
#24234=CARTESIAN_POINT('Ctrl Pts',(30.3706213015912,-14.6424253938168,-48.279761206536));
#24235=CARTESIAN_POINT('Ctrl Pts',(30.6299435607004,-14.7669045823054,-48.4165189096496));
#24236=CARTESIAN_POINT('Ctrl Pts',(30.560959047699,-14.7669045823054,-48.3069912849837));
#24237=CARTESIAN_POINT('Ctrl Pts',(30.5121796307589,-14.6753754514262,-48.2295435588551));
#24238=CARTESIAN_POINT('Origin',(30.6299435607004,-14.4544045823054,-48.4165189096496));
#24239=CARTESIAN_POINT('Origin',(31.5582959274376,-13.5169045823054,-45.624196617704));
#24240=CARTESIAN_POINT('Origin',(31.5582959274376,-13.5169045823054,-45.624196617704));
#24241=CARTESIAN_POINT('Origin',(31.5582959274376,-13.5169045823054,-45.624196617704));
#24242=CARTESIAN_POINT('Ctrl Pts',(38.7441826758856,-12.5761796977905,-39.0327738807645));
#24243=CARTESIAN_POINT('Ctrl Pts',(38.3485196429793,-12.4966730216635,-39.3120862649867));
#24244=CARTESIAN_POINT('Ctrl Pts',(38.2952452485764,-12.8445798972111,-38.9722437240839));
#24245=CARTESIAN_POINT('Ctrl Pts',(38.8327231904435,-12.7679658886682,-39.2148934728689));
#24246=CARTESIAN_POINT('Ctrl Pts',(38.4835044759548,-12.6138199372454,-39.3425594757914));
#24247=CARTESIAN_POINT('Ctrl Pts',(38.3710663661159,-12.9405865508053,-39.1587051318414));
#24248=CARTESIAN_POINT('Ctrl Pts',(38.8505926378097,-12.947799979713,-39.4500192046968));
#24249=CARTESIAN_POINT('Ctrl Pts',(38.5841849711601,-12.8036087634365,-39.5090831497147));
#24250=CARTESIAN_POINT('Ctrl Pts',(38.4159465000987,-13.0304169137549,-39.3844915465615));
#24251=CARTESIAN_POINT('Ctrl Pts',(38.7807028232922,-13.1418528526575,-39.7888775131573));
#24252=CARTESIAN_POINT('Ctrl Pts',(38.5946371067972,-13.0167291165572,-39.7950416036854));
#24253=CARTESIAN_POINT('Ctrl Pts',(38.4282877533204,-13.1274080636027,-39.6957098010915));
#24254=CARTESIAN_POINT('Ctrl Pts',(38.7479587227422,-13.1924895597094,-39.8911589997829));
#24255=CARTESIAN_POINT('Ctrl Pts',(38.5857601078203,-13.0721360087908,-39.8805420027495));
#24256=CARTESIAN_POINT('Ctrl Pts',(38.4256296765948,-13.1527155106485,-39.7878990938785));
#24257=CARTESIAN_POINT('Ctrl Pts',(38.6303501830799,-13.2848578326186,-40.1327590777328));
#24258=CARTESIAN_POINT('Ctrl Pts',(38.5262233426554,-13.1766908654362,-40.0825873356879));
#24259=CARTESIAN_POINT('Ctrl Pts',(38.397287636017,-13.1988763557092,-39.9996108902579));
#24260=CARTESIAN_POINT('Ctrl Pts',(38.5301204732258,-13.3151873395653,-40.2706150387653));
#24261=CARTESIAN_POINT('Ctrl Pts',(38.4618886750501,-13.2202535090901,-40.2043352524455));
#24262=CARTESIAN_POINT('Ctrl Pts',(38.3631207749851,-13.2140287022009,-40.1151439306369));
#24263=CARTESIAN_POINT('Ctrl Pts',(38.3844295904368,-13.2823030560806,-40.3632398375542));
#24264=CARTESIAN_POINT('Ctrl Pts',(38.3547920390607,-13.2034487358314,-40.2827072051125));
#24265=CARTESIAN_POINT('Ctrl Pts',(38.2967798358718,-13.1975864244366,-40.1818251675064));
#24266=CARTESIAN_POINT('Origin',(38.3461436957037,-13.5169045823054,-40.1137013224621));
#24267=CARTESIAN_POINT('Origin',(38.6273587102144,-12.8919045823054,-38.970752044692));
#24268=CARTESIAN_POINT('Ctrl Pts',(38.3461436957037,-13.2044045823054,-40.1137013224621));
#24269=CARTESIAN_POINT('Ctrl Pts',(38.3527349505192,-13.2044045823054,-40.1014642897562));
#24270=CARTESIAN_POINT('Ctrl Pts',(38.3586506936916,-13.2039200465849,-40.0889643259692));
#24271=CARTESIAN_POINT('Ctrl Pts',(38.3639906945034,-13.2030865921358,-40.07627240884));
#24272=CARTESIAN_POINT('Ctrl Pts',(38.3695508553509,-13.2022187756393,-40.0630572234514));
#24273=CARTESIAN_POINT('Ctrl Pts',(38.3744876033222,-13.2009724747263,-40.0496336726696));
#24274=CARTESIAN_POINT('Ctrl Pts',(38.3789315603931,-13.199446062585,-40.0360759455575));
#24275=CARTESIAN_POINT('Ctrl Pts',(38.3836173393714,-13.1978365893588,-40.0217804625719));
#24276=CARTESIAN_POINT('Ctrl Pts',(38.3877559277068,-13.1959155151287,-40.0073355755147));
#24277=CARTESIAN_POINT('Ctrl Pts',(38.3915083691255,-13.1937414656795,-39.9928256451289));
#24278=CARTESIAN_POINT('Ctrl Pts',(38.3923482654788,-13.1932548554968,-39.9895779361689));
#24279=CARTESIAN_POINT('Ctrl Pts',(38.3931688235478,-13.1927553638524,-39.9863269663215));
#24280=CARTESIAN_POINT('Ctrl Pts',(38.3939718492354,-13.1922433006301,-39.9830736815322));
#24281=CARTESIAN_POINT('Ctrl Pts',(38.3985388456595,-13.1893310763501,-39.96457148387));
#24282=CARTESIAN_POINT('Ctrl Pts',(38.4024620375392,-13.1860397456251,-39.9460233830121));
#24283=CARTESIAN_POINT('Ctrl Pts',(38.4058467955392,-13.1824628010599,-39.9274371587315));
#24284=CARTESIAN_POINT('Ctrl Pts',(38.4094080083047,-13.1786993826273,-39.9078819943239));
#24285=CARTESIAN_POINT('Ctrl Pts',(38.412373936463,-13.1746195596086,-39.8882843799791));
#24286=CARTESIAN_POINT('Ctrl Pts',(38.4148685466348,-13.1702746943006,-39.8686529670812));
#24287=CARTESIAN_POINT('Ctrl Pts',(38.4157454344845,-13.1687474177584,-39.861752270677));
#24288=CARTESIAN_POINT('Ctrl Pts',(38.416564043558,-13.1671869117775,-39.8548474119525));
#24289=CARTESIAN_POINT('Ctrl Pts',(38.4173295455032,-13.1655939279677,-39.8479388367875));
#24290=CARTESIAN_POINT('Ctrl Pts',(38.4202095417174,-13.1596007526788,-39.8219471715217));
#24291=CARTESIAN_POINT('Ctrl Pts',(38.4223252371397,-13.1531817886309,-39.796040194814));
#24292=CARTESIAN_POINT('Ctrl Pts',(38.423772695553,-13.1464435609449,-39.770219526676));
#24293=CARTESIAN_POINT('Ctrl Pts',(38.4252700922353,-13.1394728599642,-39.743508028475));
#24294=CARTESIAN_POINT('Ctrl Pts',(38.4260531947707,-13.1321600180536,-39.7168886175193));
#24295=CARTESIAN_POINT('Ctrl Pts',(38.4262243221591,-13.1245659628583,-39.6903644177419));
#24296=CARTESIAN_POINT('Ctrl Pts',(38.4264026290774,-13.1166533043878,-39.6627274137112));
#24297=CARTESIAN_POINT('Ctrl Pts',(38.4259173417366,-13.1084348255796,-39.6351935110303));
#24298=CARTESIAN_POINT('Ctrl Pts',(38.4248669041159,-13.0999262547332,-39.6077719485728));
#24299=CARTESIAN_POINT('Ctrl Pts',(38.4245074060405,-13.0970143113834,-39.5983872895176));
#24300=CARTESIAN_POINT('Ctrl Pts',(38.4240815153899,-13.094067983939,-39.5890158539865));
#24301=CARTESIAN_POINT('Ctrl Pts',(38.4235924932819,-13.0910867263844,-39.5796582381904));
#24302=CARTESIAN_POINT('Ctrl Pts',(38.4217908661768,-13.0801033488869,-39.5451834486482));
#24303=CARTESIAN_POINT('Ctrl Pts',(38.4190961268959,-13.0686901791307,-39.5108890101577));
#24304=CARTESIAN_POINT('Ctrl Pts',(38.4155748665864,-13.0568974025755,-39.47679947463));
#24305=CARTESIAN_POINT('Ctrl Pts',(38.4119452755458,-13.0447418240704,-39.4416611826959));
#24306=CARTESIAN_POINT('Ctrl Pts',(38.4074384431895,-13.0321818870426,-39.406740292716));
#24307=CARTESIAN_POINT('Ctrl Pts',(38.4020915182394,-13.0192318837648,-39.3720754913156));
#24308=CARTESIAN_POINT('Ctrl Pts',(38.3968155709718,-13.0064537851295,-39.3378708473499));
#24309=CARTESIAN_POINT('Ctrl Pts',(38.390722128783,-12.9932945861615,-39.3039153924143));
#24310=CARTESIAN_POINT('Ctrl Pts',(38.3838028214921,-12.9797471343051,-39.2702608213597));
#24311=CARTESIAN_POINT('Ctrl Pts',(38.3767438853237,-12.9659263002422,-39.2359271144062));
#24312=CARTESIAN_POINT('Ctrl Pts',(38.3688259942699,-12.9516999140197,-39.201906366769));
#24313=CARTESIAN_POINT('Ctrl Pts',(38.3599859968467,-12.9370593466235,-39.1682713601004));
#24314=CARTESIAN_POINT('Ctrl Pts',(38.3518796591162,-12.923633846796,-39.1374278303379));
#24315=CARTESIAN_POINT('Ctrl Pts',(38.3429974054472,-12.9098590019422,-39.1069088406553));
#24316=CARTESIAN_POINT('Ctrl Pts',(38.3332466950008,-12.8957449858576,-39.0767849714504));
#24317=CARTESIAN_POINT('Ctrl Pts',(38.3323642122487,-12.894467604499,-39.0740586270322));
#24318=CARTESIAN_POINT('Ctrl Pts',(38.3314745869667,-12.8931874634454,-39.0713355286148));
#24319=CARTESIAN_POINT('Ctrl Pts',(38.3305777332763,-12.8919045823054,-39.0686157342182));
#24320=CARTESIAN_POINT('Origin',(28.0161439142367,-12.8919045823054,-39.8716842439453));
#24321=CARTESIAN_POINT('Origin',(28.0161439142367,-12.8919045823054,-39.8716842439453));
#24322=CARTESIAN_POINT('Ctrl Pts',(0.0835265683425695,-6.00666333723547,
-48.3550824830876));
#24323=CARTESIAN_POINT('Ctrl Pts',(-0.26751873653172,-6.01200137934907,
-48.3550825994612));
#24324=CARTESIAN_POINT('Ctrl Pts',(-0.618388065391316,-6.02125184123581,
-48.3536254076414));
#24325=CARTESIAN_POINT('Ctrl Pts',(-1.31980082412786,-6.04818290219911,
-48.350297799115));
#24326=CARTESIAN_POINT('Ctrl Pts',(-1.67034425400482,-6.06586350127566,
-48.3484273824083));
#24327=CARTESIAN_POINT('Ctrl Pts',(-2.72152477473183,-6.1324584507553,-48.3459483822083));
#24328=CARTESIAN_POINT('Ctrl Pts',(-3.4237971299004,-6.17306838545285,-48.3412545192219));
#24329=CARTESIAN_POINT('Ctrl Pts',(-4.1255125788106,-6.20946968450873,-48.331053858379));
#24330=CARTESIAN_POINT('Ctrl Pts',(-0.267518736531456,-6.00132529512168,
-48.3550823667144));
#24331=CARTESIAN_POINT('Ctrl Pts',(-0.540535156492418,-6.00879525432304,
-48.3541407510376));
#24332=CARTESIAN_POINT('Ctrl Pts',(-0.831277824766847,-6.01828947675663,
-48.3524253715914));
#24333=CARTESIAN_POINT('Ctrl Pts',(-1.4451628644355,-6.04432658407313,-48.3485410606893));
#24334=CARTESIAN_POINT('Ctrl Pts',(-1.76830361626289,-6.06089216512314,
-48.3463749782546));
#24335=CARTESIAN_POINT('Ctrl Pts',(-2.78175048167905,-6.12571278894255,
-48.3427355507996));
#24336=CARTESIAN_POINT('Ctrl Pts',(-3.45976825406929,-6.16367997403223,
-48.3372561067169));
#24337=CARTESIAN_POINT('Ctrl Pts',(-4.12617092612534,-6.19747947412217,
-48.3260557751568));
#24338=CARTESIAN_POINT('Ctrl Pts',(-0.618615979168657,-5.99973567328051,
-48.3536249385721));
#24339=CARTESIAN_POINT('Ctrl Pts',(-0.83162301880144,-6.00835114797883,
-48.352053093828));
#24340=CARTESIAN_POINT('Ctrl Pts',(-1.07630838456854,-6.01789996842699,
-48.3500372977422));
#24341=CARTESIAN_POINT('Ctrl Pts',(-1.6193471348745,-6.04289085428944,-48.3454511925192));
#24342=CARTESIAN_POINT('Ctrl Pts',(-1.91769809006312,-6.05836696395434,
-48.3428851569135));
#24343=CARTESIAN_POINT('Ctrl Pts',(-2.87872640181385,-6.11975101512502,
-48.3377026418223));
#24344=CARTESIAN_POINT('Ctrl Pts',(-3.52173694667449,-6.15479195325804,
-48.3313642359895));
#24345=CARTESIAN_POINT('Ctrl Pts',(-4.1268396622487,-6.18527410484422,-48.3199255790051));
#24346=CARTESIAN_POINT('Ctrl Pts',(-1.3209415423196,-5.99820579736957,-48.3438941182277));
#24347=CARTESIAN_POINT('Ctrl Pts',(-1.44672510894581,-6.00829173506076,
-48.3421773991346));
#24348=CARTESIAN_POINT('Ctrl Pts',(-1.62065368286856,-6.01814206512116,
-48.3401377766449));
#24349=CARTESIAN_POINT('Ctrl Pts',(-2.04329097938473,-6.04173521008609,
-48.3350871089986));
#24350=CARTESIAN_POINT('Ctrl Pts',(-2.29199666529032,-6.0555205803039,-48.3320814057566));
#24351=CARTESIAN_POINT('Ctrl Pts',(-3.11802710747004,-6.10935599904102,
-48.3246778342889));
#24352=CARTESIAN_POINT('Ctrl Pts',(-3.66733280245846,-6.13882811018935,
-48.3171415019516));
#24353=CARTESIAN_POINT('Ctrl Pts',(-4.12827543127815,-6.16205725113852,
-48.3065253445717));
#24354=CARTESIAN_POINT('Ctrl Pts',(-1.67216986283335,-5.9982655432998,-48.3356207260257));
#24355=CARTESIAN_POINT('Ctrl Pts',(-1.77074437171872,-6.00864450579839,
-48.3343702273337));
#24356=CARTESIAN_POINT('Ctrl Pts',(-1.91997597377325,-6.0187257861122,-48.3325976279209));
#24357=CARTESIAN_POINT('Ctrl Pts',(-2.29305999396389,-6.04195544062549,
-48.3277770168035));
#24358=CARTESIAN_POINT('Ctrl Pts',(-2.51690957785804,-6.05514353311736,
-48.3247339908856));
#24359=CARTESIAN_POINT('Ctrl Pts',(-3.26035692792899,-6.10489083408603,
-48.3166668014157));
#24360=CARTESIAN_POINT('Ctrl Pts',(-3.75095996563724,-6.13175228789484,
-48.3088106386412));
#24361=CARTESIAN_POINT('Ctrl Pts',(-4.12904246418424,-6.15104576671076,
-48.2992553062901));
#24362=CARTESIAN_POINT('Ctrl Pts',(-2.72609224471469,-5.99214762358687,
-48.2947245925476));
#24363=CARTESIAN_POINT('Ctrl Pts',(-2.78737351536448,-6.00381665756758,
-48.2942918711989));
#24364=CARTESIAN_POINT('Ctrl Pts',(-2.8843828599883,-6.01569196513299,-48.293681485549));
#24365=CARTESIAN_POINT('Ctrl Pts',(-3.12263860656582,-6.04033961885396,
-48.2916809761606));
#24366=CARTESIAN_POINT('Ctrl Pts',(-3.26388338895268,-6.05313466117662,
-48.2902937014433));
#24367=CARTESIAN_POINT('Ctrl Pts',(-3.71314893169586,-6.09364276617914,
-48.2862238404994));
#24368=CARTESIAN_POINT('Ctrl Pts',(-3.98882416158545,-6.11446024451105,
-48.2821814456289));
#24369=CARTESIAN_POINT('Ctrl Pts',(-4.13160728682495,-6.12223844465218,
-48.2774220038444));
#24370=CARTESIAN_POINT('Ctrl Pts',(-3.42734501756996,-5.99475664078893,
-48.2515240164107));
#24371=CARTESIAN_POINT('Ctrl Pts',(-3.46432076032786,-6.00697011627485,
-48.2527720832235));
#24372=CARTESIAN_POINT('Ctrl Pts',(-3.52649817491115,-6.02014444454774,
-48.2541165048377));
#24373=CARTESIAN_POINT('Ctrl Pts',(-3.67166030976089,-6.04594588203951,
-48.2567445235025));
#24374=CARTESIAN_POINT('Ctrl Pts',(-3.75464503002734,-6.05857299125839,
-48.2580281205531));
#24375=CARTESIAN_POINT('Ctrl Pts',(-3.99041609240001,-6.0919301033921,-48.2614073736106));
#24376=CARTESIAN_POINT('Ctrl Pts',(-4.13001933607955,-6.10813589078397,
-48.263031491523));
#24377=CARTESIAN_POINT('Ctrl Pts',(-4.13366096331968,-6.1084336923001,-48.2630127553113));
#24378=CARTESIAN_POINT('Ctrl Pts',(-4.12845481065586,-6.007051447105,-48.1954680629781));
#24379=CARTESIAN_POINT('Ctrl Pts',(-4.12850749787586,-6.01900581052064,
-48.200433936555));
#24380=CARTESIAN_POINT('Ctrl Pts',(-4.12864057911576,-6.03128117156189,
-48.2071191491468));
#24381=CARTESIAN_POINT('Ctrl Pts',(-4.12920120927171,-6.05467770199135,
-48.221588093388));
#24382=CARTESIAN_POINT('Ctrl Pts',(-4.12962875818777,-6.06579887137954,
-48.2293718250376));
#24383=CARTESIAN_POINT('Ctrl Pts',(-4.13155362590474,-6.09473681170807,
-48.2508605601154));
#24384=CARTESIAN_POINT('Ctrl Pts',(-4.13369316567446,-6.10812801481236,
-48.2627031036729));
#24385=CARTESIAN_POINT('Ctrl Pts',(-4.13722371861477,-6.1084337131847,-48.2627017315157));
#24386=CARTESIAN_POINT('Ctrl Pts',(-4.13722361839104,-6.10843370450313,
-48.2627017315515));
#24387=CARTESIAN_POINT('Ctrl Pts',(-4.13701407672473,-6.10841554618144,
-48.2627017996875));
#24388=CARTESIAN_POINT('Ctrl Pts',(-4.13685790799886,-6.10835892240998,
-48.262663281257));
#24389=CARTESIAN_POINT('Ctrl Pts',(-4.13674169752953,-6.10830758140055,
-48.2626265177434));
#24390=CARTESIAN_POINT('Ctrl Pts',(-4.13662522520969,-6.10825612470732,
-48.2625896713927));
#24391=CARTESIAN_POINT('Ctrl Pts',(-4.13654900508533,-6.10820886405876,
-48.2625535279384));
#24392=CARTESIAN_POINT('Ctrl Pts',(-4.13650271508106,-6.10817971723551,
-48.2625311962608));
#24393=CARTESIAN_POINT('Ctrl Pts',(-4.1364102317774,-6.10812148447991,-48.2624865795588));
#24394=CARTESIAN_POINT('Ctrl Pts',(-4.13635999437262,-6.10808254421846,
-48.2624559072796));
#24395=CARTESIAN_POINT('Ctrl Pts',(-4.13631216026214,-6.10804496697942,
-48.2624262729228));
#24396=CARTESIAN_POINT('Ctrl Pts',(-4.13621649204119,-6.10796981250135,
-48.2623670042092));
#24397=CARTESIAN_POINT('Ctrl Pts',(-4.13614678177369,-6.10790555146429,
-48.2623154903795));
#24398=CARTESIAN_POINT('Ctrl Pts',(-4.13607861507656,-6.10783843371639,
-48.262261395266));
#24399=CARTESIAN_POINT('Ctrl Pts',(-4.13584716396225,-6.10761054417216,
-48.2620777223754));
#24400=CARTESIAN_POINT('Ctrl Pts',(-4.13565789362604,-6.10735799473039,
-48.2618699174502));
#24401=CARTESIAN_POINT('Ctrl Pts',(-4.13549318405383,-6.10710655540123,
-48.2616620276179));
#24402=CARTESIAN_POINT('Ctrl Pts',(-4.13530295146511,-6.10681615361189,
-48.2614219236552));
#24403=CARTESIAN_POINT('Ctrl Pts',(-4.13514554673403,-6.10652655415251,
-48.2611810107393));
#24404=CARTESIAN_POINT('Ctrl Pts',(-4.13499914832338,-6.10622795083367,
-48.2609322939333));
#24405=CARTESIAN_POINT('Ctrl Pts',(-4.13499063034215,-6.10621057702851,
-48.2609178227032));
#24406=CARTESIAN_POINT('Ctrl Pts',(-4.13498215077319,-6.10619316218202,
-48.2609033158664));
#24407=CARTESIAN_POINT('Ctrl Pts',(-4.13497370572295,-6.10617570066421,
-48.2608887688412));
#24408=CARTESIAN_POINT('Ctrl Pts',(-4.13474598139209,-6.10570484349367,
-48.2604965021883));
#24409=CARTESIAN_POINT('Ctrl Pts',(-4.13455475664386,-6.10522791969297,
-48.2600983887895));
#24410=CARTESIAN_POINT('Ctrl Pts',(-4.13438266923931,-6.10475153053746,
-48.2597011835133));
#24411=CARTESIAN_POINT('Ctrl Pts',(-4.13411895040737,-6.10402147831793,
-48.2590924782348));
#24412=CARTESIAN_POINT('Ctrl Pts',(-4.13389862072628,-6.10328536512368,
-48.2584796979253));
#24413=CARTESIAN_POINT('Ctrl Pts',(-4.13370045808856,-6.10254802979483,
-48.2578680802102));
#24414=CARTESIAN_POINT('Ctrl Pts',(-4.13333556021568,-6.10119029608581,
-48.2567418436712));
#24415=CARTESIAN_POINT('Ctrl Pts',(-4.13304559573053,-6.0998260029529,-48.255617420827));
#24416=CARTESIAN_POINT('Ctrl Pts',(-4.1327886833905,-6.09845605313882,-48.2544972544273));
#24417=CARTESIAN_POINT('Ctrl Pts',(-4.13238882388217,-6.09632385715694,
-48.2527538224623));
#24418=CARTESIAN_POINT('Ctrl Pts',(-4.13207291555085,-6.09417845354371,
-48.2510208352385));
#24419=CARTESIAN_POINT('Ctrl Pts',(-4.1317961782277,-6.09202099947451,-48.2493008362025));
#24420=CARTESIAN_POINT('Ctrl Pts',(-4.13138155083735,-6.08878854950964,
-48.2467238122451));
#24421=CARTESIAN_POINT('Ctrl Pts',(-4.13105831741888,-6.0855286414402,-48.244175351545));
#24422=CARTESIAN_POINT('Ctrl Pts',(-4.13078034438517,-6.08224206853585,
-48.2416599697016));
#24423=CARTESIAN_POINT('Ctrl Pts',(-4.13058977880351,-6.07998894466698,
-48.239935539106));
#24424=CARTESIAN_POINT('Ctrl Pts',(-4.13042195826053,-6.07772362660907,
-48.2382269095075));
#24425=CARTESIAN_POINT('Ctrl Pts',(-4.13027038076009,-6.07544485148905,
-48.2365347367302));
#24426=CARTESIAN_POINT('Ctrl Pts',(-4.12989286227413,-6.06976934073926,
-48.2323202160853));
#24427=CARTESIAN_POINT('Ctrl Pts',(-4.12961378163258,-6.06401605346406,
-48.2282106199239));
#24428=CARTESIAN_POINT('Ctrl Pts',(-4.12938833601404,-6.05817109637975,
-48.2242324211879));
#24429=CARTESIAN_POINT('Ctrl Pts',(-4.12919574641795,-6.05317797240012,
-48.2208339976892));
#24430=CARTESIAN_POINT('Ctrl Pts',(-4.12904403874395,-6.04811857384527,
-48.2175317800084));
#24431=CARTESIAN_POINT('Ctrl Pts',(-4.12892089419374,-6.04297943677662,
-48.2143536212674));
#24432=CARTESIAN_POINT('Ctrl Pts',(-4.12878312414699,-6.03722994032761,
-48.2107980024637));
#24433=CARTESIAN_POINT('Ctrl Pts',(-4.12868136839902,-6.03138079133467,
-48.2073956831987));
#24434=CARTESIAN_POINT('Ctrl Pts',(-4.1286061408438,-6.02540321593081,-48.204215112076));
#24435=CARTESIAN_POINT('Ctrl Pts',(-4.12854502676884,-6.0205470965177,-48.2016312495348));
#24436=CARTESIAN_POINT('Ctrl Pts',(-4.12850159802488,-6.01560535413783,
-48.1991929077068));
#24437=CARTESIAN_POINT('Ctrl Pts',(-4.12847260770142,-6.01056187471018,
-48.1969709327471));
#24438=CARTESIAN_POINT('Ctrl Pts',(-4.12846591277299,-6.00939715042373,
-48.1964577972745));
#24439=CARTESIAN_POINT('Ctrl Pts',(-4.12845999189732,-6.0082270347227,-48.1959564051244));
#24440=CARTESIAN_POINT('Ctrl Pts',(-4.12845481065586,-6.00705144710501,
-48.1954680629781));
#24441=CARTESIAN_POINT('Ctrl Pts',(-29.2891959206732,-14.4313124010515,
-48.3540540388567));
#24442=CARTESIAN_POINT('Ctrl Pts',(-29.2899746397388,-14.7671408702645,
-48.3291878272403));
#24443=CARTESIAN_POINT('Ctrl Pts',(-29.2771538582069,-14.7669045053135,
-48.6657591384501));
#24444=CARTESIAN_POINT('Ctrl Pts',(-29.4909783664048,-14.4776157931207,
-48.3580817390519));
#24445=CARTESIAN_POINT('Ctrl Pts',(-29.4738070695996,-14.7670932226239,
-48.3824331547409));
#24446=CARTESIAN_POINT('Ctrl Pts',(-29.5030413152524,-14.766904515933,-48.6738002220355));
#24447=CARTESIAN_POINT('Ctrl Pts',(-29.6888652328203,-14.5232222287052,
-48.3502871282448));
#24448=CARTESIAN_POINT('Ctrl Pts',(-29.6826141588837,-14.7670538266072,
-48.4107537194043));
#24449=CARTESIAN_POINT('Ctrl Pts',(-29.7249751299964,-14.7669045263941,
-48.6581913870529));
#24450=CARTESIAN_POINT('Ctrl Pts',(-30.0744334835308,-14.6124212350924,
-48.3047943346257));
#24451=CARTESIAN_POINT('Ctrl Pts',(-30.0911805469422,-14.7669897766034,
-48.3969112259716));
#24452=CARTESIAN_POINT('Ctrl Pts',(-30.1581350349744,-14.7669045468573,
-48.5671620693194));
#24453=CARTESIAN_POINT('Ctrl Pts',(-30.266548451205,-14.657050343384,-48.26838676292));
#24454=CARTESIAN_POINT('Ctrl Pts',(-30.3019621750083,-14.7669625172305,
-48.3638427252435));
#24455=CARTESIAN_POINT('Ctrl Pts',(-30.3752125459255,-14.766904557097,-48.4937819709548));
#24456=CARTESIAN_POINT('Ctrl Pts',(-30.4284642980806,-14.6947854519677,
-48.1964235659436));
#24457=CARTESIAN_POINT('Ctrl Pts',(-30.4842634718295,-14.7669413153223,
-48.2634723170081));
#24458=CARTESIAN_POINT('Ctrl Pts',(-30.5563486668935,-14.7669045657556,
-48.3506792970572));
#24459=CARTESIAN_POINT('Origin',(-30.4628904239763,-14.4544045823054,-48.4165189096496));
#24460=CARTESIAN_POINT('Origin',(0.0835265683620477,-14.4544045823054,0.0824317919394229));
#24461=CARTESIAN_POINT('Origin',(32.2559828833067,-14.4544045823054,-47.3534709072605));
#24462=CARTESIAN_POINT('Ctrl Pts',(32.1346390008072,-14.6836564585996,-47.1787761295051));
#24463=CARTESIAN_POINT('Ctrl Pts',(32.3631522226839,-14.7195047625521,-47.0671198130351));
#24464=CARTESIAN_POINT('Ctrl Pts',(32.3073948493568,-14.9046273277204,-46.8980302578828));
#24465=CARTESIAN_POINT('Ctrl Pts',(31.9843639648594,-14.2208393515122,-46.7214805263384));
#24466=CARTESIAN_POINT('Ctrl Pts',(32.2124425821686,-14.2572370951355,-46.6100784470017));
#24467=CARTESIAN_POINT('Ctrl Pts',(32.1566961228079,-14.4418102212117,-46.441021989494));
#24468=CARTESIAN_POINT('Ctrl Pts',(31.8340251513167,-13.7582547217141,-46.2639539460438));
#24469=CARTESIAN_POINT('Ctrl Pts',(32.0615622174417,-13.7949155819462,-46.1525193435408));
#24470=CARTESIAN_POINT('Ctrl Pts',(32.0059240732351,-13.9792255914462,-45.9837913620383));
#24471=CARTESIAN_POINT('Ctrl Pts',(31.6836214013763,-13.2959337131846,-45.8061901631445));
#24472=CARTESIAN_POINT('Ctrl Pts',(31.9104948844699,-13.3325299785125,-45.6943932409652));
#24473=CARTESIAN_POINT('Ctrl Pts',(31.8550769043756,-13.5169045823054,-45.5263329281778));
#24474=CARTESIAN_POINT('Ctrl Pts',(32.1607495589358,-14.4544045595331,-46.4533144213431));
#24475=CARTESIAN_POINT('Ctrl Pts',(32.1704524589662,-14.464589809121,-46.4827393915657));
#24476=CARTESIAN_POINT('Ctrl Pts',(32.1792350499887,-14.4747854410079,-46.5124192299058));
#24477=CARTESIAN_POINT('Ctrl Pts',(32.1870746530974,-14.4849571274431,-46.5423134022322));
#24478=CARTESIAN_POINT('Ctrl Pts',(32.1943891325094,-14.4944474791847,-46.5702051596324));
#24479=CARTESIAN_POINT('Ctrl Pts',(32.200883324293,-14.5039154723654,-46.5982848321975));
#24480=CARTESIAN_POINT('Ctrl Pts',(32.2064963987694,-14.5133279314553,-46.6265388357118));
#24481=CARTESIAN_POINT('Ctrl Pts',(32.2118478660973,-14.522301706435,-46.6534760120001));
#24482=CARTESIAN_POINT('Ctrl Pts',(32.2163984055497,-14.5312237762477,-46.6805728996695));
#24483=CARTESIAN_POINT('Ctrl Pts',(32.2200515628477,-14.5400795913951,-46.7078177704894));
#24484=CARTESIAN_POINT('Ctrl Pts',(32.2234471358259,-14.5483109825347,-46.7331416039858));
#24485=CARTESIAN_POINT('Ctrl Pts',(32.2260667128419,-14.5564843935868,-46.7585942678845));
#24486=CARTESIAN_POINT('Ctrl Pts',(32.2277998636429,-14.5646141114394,-46.7841509175346));
#24487=CARTESIAN_POINT('Ctrl Pts',(32.2285348731612,-14.5680618322026,-46.7949892016216));
#24488=CARTESIAN_POINT('Ctrl Pts',(32.2291100930038,-14.5715020908807,-46.8058459067609));
#24489=CARTESIAN_POINT('Ctrl Pts',(32.2295157094557,-14.5749379971499,-46.8167175507953));
#24490=CARTESIAN_POINT('Ctrl Pts',(32.2302341780251,-14.5810240191791,-46.835974497843));
#24491=CARTESIAN_POINT('Ctrl Pts',(32.2304309663889,-14.5871115455618,-46.8552737733236));
#24492=CARTESIAN_POINT('Ctrl Pts',(32.2299898035979,-14.593121590845,-46.8745857273906));
#24493=CARTESIAN_POINT('Ctrl Pts',(32.2295649448931,-14.5989095224365,-46.893183968131));
#24494=CARTESIAN_POINT('Ctrl Pts',(32.2285476864384,-14.6046251025894,-46.9117947067213));
#24495=CARTESIAN_POINT('Ctrl Pts',(32.226808708919,-14.6102297042048,-46.9303675333675));
#24496=CARTESIAN_POINT('Ctrl Pts',(32.2251621322189,-14.6155365045113,-46.947953490212));
#24497=CARTESIAN_POINT('Ctrl Pts',(32.222867550472,-14.6207436431622,-46.9655059347368));
#24498=CARTESIAN_POINT('Ctrl Pts',(32.2198039300316,-14.6258519573891,-46.9829517238513));
#24499=CARTESIAN_POINT('Ctrl Pts',(32.2186440659339,-14.62778592747,-46.9895565709079));
#24500=CARTESIAN_POINT('Ctrl Pts',(32.2173739277389,-14.6297061021636,-46.9961457718268));
#24501=CARTESIAN_POINT('Ctrl Pts',(32.2159869766137,-14.6316139267949,-47.0027139299464));
#24502=CARTESIAN_POINT('Ctrl Pts',(32.2132964611226,-14.6353148731598,-47.0154553530929));
#24503=CARTESIAN_POINT('Ctrl Pts',(32.2102245596925,-14.6390800656586,-47.0281862151157));
#24504=CARTESIAN_POINT('Ctrl Pts',(32.2066063719569,-14.6427512671794,-47.0408006165906));
#24505=CARTESIAN_POINT('Ctrl Pts',(32.2031615521097,-14.6462465606208,-47.0528105905711));
#24506=CARTESIAN_POINT('Ctrl Pts',(32.1992207015494,-14.649656542816,-47.0647153880478));
#24507=CARTESIAN_POINT('Ctrl Pts',(32.1946310810407,-14.6528783603918,-47.0763929094605));
#24508=CARTESIAN_POINT('Ctrl Pts',(32.1902432135721,-14.6559585515544,-47.0875571040216));
#24509=CARTESIAN_POINT('Ctrl Pts',(32.1852614610874,-14.6588667966843,-47.0985138216531));
#24510=CARTESIAN_POINT('Ctrl Pts',(32.1795549189995,-14.6615453756132,-47.1091229500894));
#24511=CARTESIAN_POINT('Ctrl Pts',(32.1740290872121,-14.6641391314047,-47.1193961169648));
#24512=CARTESIAN_POINT('Ctrl Pts',(32.1678226434197,-14.6665177507396,-47.1293434730558));
#24513=CARTESIAN_POINT('Ctrl Pts',(32.1608329021082,-14.6686579758318,-47.1388029396664));
#24514=CARTESIAN_POINT('Ctrl Pts',(32.1541159295901,-14.6707146804345,-47.1478932585248));
#24515=CARTESIAN_POINT('Ctrl Pts',(32.146674683016,-14.6725517512568,-47.1565328027866));
#24516=CARTESIAN_POINT('Ctrl Pts',(32.1384470677752,-14.6741705573068,-47.1645458719539));
#24517=CARTESIAN_POINT('Ctrl Pts',(32.1363333475157,-14.6745864376128,-47.1666044741302));
#24518=CARTESIAN_POINT('Ctrl Pts',(32.1341679203907,-14.6749880046772,-47.1686215712106));
#24519=CARTESIAN_POINT('Ctrl Pts',(32.13195017295,-14.6753754514101,-47.1705938672733));
#24520=CARTESIAN_POINT('Origin',(14.8778438489026,-13.5169045823054,4.96086600976507));
#24521=CARTESIAN_POINT('Origin',(29.344152791651,-13.5169045823054,-38.9095962781799));
#24522=CARTESIAN_POINT('Origin',(0.0835265683620477,-12.8919045823054,0.0824317919394229));
#24523=CARTESIAN_POINT('Ctrl Pts',(29.326104774044,-12.8919045823054,-38.5318534679819));
#24524=CARTESIAN_POINT('Ctrl Pts',(29.326104774044,-12.9139187960401,-38.5318534679819));
#24525=CARTESIAN_POINT('Ctrl Pts',(29.3262379991816,-12.9356278245235,-38.534839371807));
#24526=CARTESIAN_POINT('Ctrl Pts',(29.3264870838848,-12.9566097073251,-38.5403603727184));
#24527=CARTESIAN_POINT('Ctrl Pts',(29.3267304618257,-12.9771108756647,-38.5457548823607));
#24528=CARTESIAN_POINT('Ctrl Pts',(29.3270844381453,-12.9969176625798,-38.5535693851653));
#24529=CARTESIAN_POINT('Ctrl Pts',(29.3275331992697,-13.0156824718681,-38.5633972432341));
#24530=CARTESIAN_POINT('Ctrl Pts',(29.327995837035,-13.0350275286559,-38.5735289994125));
#24531=CARTESIAN_POINT('Ctrl Pts',(29.3285591963311,-13.0532645768243,-38.5858001371315));
#24532=CARTESIAN_POINT('Ctrl Pts',(29.3292065902322,-13.0700686738468,-38.5997854381345));
#24533=CARTESIAN_POINT('Ctrl Pts',(29.329811080222,-13.0857591343542,-38.6128439091002));
#24534=CARTESIAN_POINT('Ctrl Pts',(29.3304888352246,-13.1002006435729,-38.6273968808538));
#24535=CARTESIAN_POINT('Ctrl Pts',(29.3312269160076,-13.1131767225615,-38.6431179310376));
#24536=CARTESIAN_POINT('Ctrl Pts',(29.3312793015773,-13.1140977047963,-38.6442337386668));
#24537=CARTESIAN_POINT('Ctrl Pts',(29.331331991325,-13.1150113249639,-38.6453554392112));
#24538=CARTESIAN_POINT('Ctrl Pts',(29.3313849807581,-13.1159175149051,-38.6464829200197));
#24539=CARTESIAN_POINT('Ctrl Pts',(29.33152105734,-13.1182446058459,-38.6493782847288));
#24540=CARTESIAN_POINT('Ctrl Pts',(29.3316591563938,-13.1205242789863,-38.6523112691164));
#24541=CARTESIAN_POINT('Ctrl Pts',(29.3317991613583,-13.1227565895721,-38.6552792745761));
#24542=CARTESIAN_POINT('Ctrl Pts',(29.3324793477165,-13.1336018279018,-38.6696987405676));
#24543=CARTESIAN_POINT('Ctrl Pts',(29.3332010329856,-13.1433259542997,-38.6849362776199));
#24544=CARTESIAN_POINT('Ctrl Pts',(29.3339549946389,-13.1519718239002,-38.7007769154678));
#24545=CARTESIAN_POINT('Ctrl Pts',(29.3347774710834,-13.161403369998,-38.7180570403117));
#24546=CARTESIAN_POINT('Ctrl Pts',(29.3356383745261,-13.1695524259128,-38.736055450668));
#24547=CARTESIAN_POINT('Ctrl Pts',(29.3365286964844,-13.1764446443693,-38.7545492977395));
#24548=CARTESIAN_POINT('Ctrl Pts',(29.3374556677569,-13.1836205748887,-38.7738044276311));
#24549=CARTESIAN_POINT('Ctrl Pts',(29.3384145864597,-13.1894346380349,-38.7935979691783));
#24550=CARTESIAN_POINT('Ctrl Pts',(29.3393977354577,-13.1938753423343,-38.8137207235506));
#24551=CARTESIAN_POINT('Ctrl Pts',(29.340386391301,-13.1983409200474,-38.8339561901333));
#24552=CARTESIAN_POINT('Ctrl Pts',(29.3413996267514,-13.2014181302613,-38.8545262160037));
#24553=CARTESIAN_POINT('Ctrl Pts',(29.3424309768835,-13.2030479859161,-38.8752367598351));
#24554=CARTESIAN_POINT('Ctrl Pts',(29.342999734741,-13.2039468011501,-38.8866579873821));
#24555=CARTESIAN_POINT('Ctrl Pts',(29.3435740193766,-13.2044045823054,-38.8981221352879));
#24556=CARTESIAN_POINT('Ctrl Pts',(29.344152791651,-13.2044045823054,-38.9095962781799));
#24557=CARTESIAN_POINT('Ctrl Pts',(38.5478788395692,-13.5144022989996,-39.7276020745818));
#24558=CARTESIAN_POINT('Ctrl Pts',(38.6381834185545,-13.1933434847834,-40.0014593274924));
#24559=CARTESIAN_POINT('Ctrl Pts',(38.9993997115465,-13.2935409838962,-39.7876377918258));
#24560=CARTESIAN_POINT('Ctrl Pts',(37.6321471688162,-10.8876754024414,-36.9505584011307));
#24561=CARTESIAN_POINT('Ctrl Pts',(37.7135976841852,-10.5315615565335,-37.197564861227));
#24562=CARTESIAN_POINT('Ctrl Pts',(38.0873367198682,-10.6668492065293,-37.0070442715679));
#24563=CARTESIAN_POINT('Ctrl Pts',(36.7092038782167,-8.28316551512454,-34.1516448023406));
#24564=CARTESIAN_POINT('Ctrl Pts',(36.7875685005852,-7.90880841569709,-34.3892929975985));
#24565=CARTESIAN_POINT('Ctrl Pts',(37.1684809904989,-8.06235637916793,-34.2039263650138));
#24566=CARTESIAN_POINT('Ctrl Pts',(35.7758342203384,-5.72100917799142,-31.3211122498619));
#24567=CARTESIAN_POINT('Ctrl Pts',(35.8691121688728,-5.37442442506644,-31.6039865296246));
#24568=CARTESIAN_POINT('Ctrl Pts',(36.2397262089015,-5.50017070394688,-31.3680265018349));
#24569=CARTESIAN_POINT('Ctrl Pts',(36.2681294096903,-7.07886051013668,-32.8140443877542));
#24570=CARTESIAN_POINT('Ctrl Pts',(36.2569664163808,-6.97591157388989,-32.7801889939238));
#24571=CARTESIAN_POINT('Ctrl Pts',(36.2554727333015,-6.87711064623287,-32.7339348504581));
#24572=CARTESIAN_POINT('Ctrl Pts',(36.2630467530083,-6.68740381001557,-32.6293153550853));
#24573=CARTESIAN_POINT('Ctrl Pts',(36.2724147441973,-6.59673597566758,-32.570618363652));
#24574=CARTESIAN_POINT('Ctrl Pts',(36.30162041965,-6.42451466437639,-32.4414153041646));
#24575=CARTESIAN_POINT('Ctrl Pts',(36.321062466775,-6.34396835910598,-32.3720253866706));
#24576=CARTESIAN_POINT('Ctrl Pts',(36.361286826097,-6.23614184370369,-32.256689531614));
#24577=CARTESIAN_POINT('Ctrl Pts',(36.3765528768977,-6.2025085626214,-32.216414958201));
#24578=CARTESIAN_POINT('Ctrl Pts',(36.4125915840679,-6.14483638321709,-32.1317287552063));
#24579=CARTESIAN_POINT('Ctrl Pts',(36.4332088055153,-6.11985717446073,-32.0871018700298));
#24580=CARTESIAN_POINT('Ctrl Pts',(36.459401450406,-6.10843371318468,-32.0401832160515));
#24581=CARTESIAN_POINT('Origin',(35.9713494567465,-14.7669045823054,-32.9119111827578));
#24582=CARTESIAN_POINT('Origin',(35.9713494567465,-12.8919045823054,-32.9119111827578));
#24583=CARTESIAN_POINT('Origin',(35.9713494567465,-7.07886995352309,-32.9119111827578));
#24584=CARTESIAN_POINT('Origin',(22.6388808156566,-12.8919045823054,7.52007219592841));
#24585=CARTESIAN_POINT('Origin',(35.9713494567465,-12.8919045823054,-32.9119111827578));
#24586=CARTESIAN_POINT('Origin',(0.0835265683620477,-13.5169045823054,0.0824317919394229));
#24587=CARTESIAN_POINT('Origin',(37.084741276154,-13.5169045823054,-41.2777797274919));
#24588=CARTESIAN_POINT('Ctrl Pts',(36.2784254248408,-7.15534954851098,-32.836829591711));
#24589=CARTESIAN_POINT('Ctrl Pts',(36.1434013184732,-7.11664814656864,-32.2629428084027));
#24590=CARTESIAN_POINT('Ctrl Pts',(35.7454348445936,-7.18677502471099,-32.6959179419936));
#24591=CARTESIAN_POINT('Ctrl Pts',(36.2588919622279,-7.03238137414826,-32.8057216385754));
#24592=CARTESIAN_POINT('Ctrl Pts',(36.0761096691241,-7.08021162576623,-32.3364442437081));
#24593=CARTESIAN_POINT('Ctrl Pts',(35.7317594193323,-7.01162141076107,-32.7107648798629));
#24594=CARTESIAN_POINT('Ctrl Pts',(36.2544224233627,-6.9007862514849,-32.7478923847614));
#24595=CARTESIAN_POINT('Ctrl Pts',(36.0343634050485,-6.94927177594153,-32.3814124480413));
#24596=CARTESIAN_POINT('Ctrl Pts',(35.7530195024256,-6.83269992253369,-32.6877129958713));
#24597=CARTESIAN_POINT('Ctrl Pts',(36.2640203102083,-6.67697195553546,-32.6234372773615));
#24598=CARTESIAN_POINT('Ctrl Pts',(36.0276939617195,-6.69622936404188,-32.3874954073924));
#24599=CARTESIAN_POINT('Ctrl Pts',(35.8268903954434,-6.53795985193932,-32.6071031454275));
#24600=CARTESIAN_POINT('Ctrl Pts',(36.2744837959597,-6.58104909157633,-32.5604598516983));
#24601=CARTESIAN_POINT('Ctrl Pts',(36.0416953029314,-6.57996991861108,-32.371645126971));
#24602=CARTESIAN_POINT('Ctrl Pts',(35.8724674696584,-6.41511471179818,-32.5572714061768));
#24603=CARTESIAN_POINT('Ctrl Pts',(36.3068728829042,-6.40173475569586,-32.4227465017006));
#24604=CARTESIAN_POINT('Ctrl Pts',(36.100847967489,-6.36383534698761,-32.3054510953759));
#24605=CARTESIAN_POINT('Ctrl Pts',(35.9858853058558,-6.19278444406274,-32.4324748322831));
#24606=CARTESIAN_POINT('Ctrl Pts',(36.3281094141996,-6.32050524456542,-32.3501393983736));
#24607=CARTESIAN_POINT('Ctrl Pts',(36.1424453507782,-6.2630776214194,-32.2590472164985));
#24608=CARTESIAN_POINT('Ctrl Pts',(36.0517003472671,-6.09580032219768,-32.3597580486369));
#24609=CARTESIAN_POINT('Ctrl Pts',(36.3918485606395,-6.16373114058233,-32.1739515607077));
#24610=CARTESIAN_POINT('Ctrl Pts',(36.2655421565245,-6.07811517883126,-32.1210623649169));
#24611=CARTESIAN_POINT('Ctrl Pts',(36.2288436140461,-5.92198390393177,-32.1624016484031));
#24612=CARTESIAN_POINT('Ctrl Pts',(36.4367840484078,-6.09886182619368,-32.071567005352));
#24613=CARTESIAN_POINT('Ctrl Pts',(36.3533716225856,-6.00005797767508,-32.0222299156167));
#24614=CARTESIAN_POINT('Ctrl Pts',(36.343660429214,-5.86097989280999,-32.0334346821493));
#24615=CARTESIAN_POINT('Ctrl Pts',(36.4922864453313,-6.10268725739347,-31.9855710438836));
#24616=CARTESIAN_POINT('Ctrl Pts',(36.4460471988281,-6.01584203961169,-31.9169227992496));
#24617=CARTESIAN_POINT('Ctrl Pts',(36.4638571848965,-5.89881153279529,-31.896661392609));
#24618=CARTESIAN_POINT('Origin',(36.625034450523,-5.88746284406389,-32.186449528893));
#24619=CARTESIAN_POINT('Origin',(0.0835265683620477,-5.88746284406389,0.0824317919394229));
#24620=CARTESIAN_POINT('Origin',(-32.1853547524705,-5.88746284406389,-36.4590760902215));
#24621=CARTESIAN_POINT('Ctrl Pts',(-39.7265072775759,-13.5144022795305,
-38.3819204724802));
#24622=CARTESIAN_POINT('Ctrl Pts',(-40.0003645304861,-13.1933434652888,
-38.4722250514726));
#24623=CARTESIAN_POINT('Ctrl Pts',(-39.7865429947924,-13.2935409644279,
-38.8334413444868));
#24624=CARTESIAN_POINT('Ctrl Pts',(-36.9494636177385,-10.8876753960648,
-37.4661888062163));
#24625=CARTESIAN_POINT('Ctrl Pts',(-37.196470078124,-10.5315615503784,-37.5476393216535));
#24626=CARTESIAN_POINT('Ctrl Pts',(-37.0059494882058,-10.6668492001279,
-37.921378357208));
#24627=CARTESIAN_POINT('Ctrl Pts',(-34.150550032778,-8.28316552163412,-36.5432455201772));
#24628=CARTESIAN_POINT('Ctrl Pts',(-34.3881982285108,-7.90880842257625,
-36.621610142688));
#24629=CARTESIAN_POINT('Ctrl Pts',(-34.2028315954194,-8.06235638571299,
-37.0025226324655));
#24630=CARTESIAN_POINT('Ctrl Pts',(-31.3200174944135,-5.72100919698887,
-35.609875866953));
#24631=CARTESIAN_POINT('Ctrl Pts',(-31.602891774127,-5.37442444417786,-35.7031538154752));
#24632=CARTESIAN_POINT('Ctrl Pts',(-31.3669317464438,-5.50017072293065,
-36.0737678554641));
#24633=CARTESIAN_POINT('Origin',(-38.9696572682695,-12.8919045823054,-38.4614003499128));
#24634=CARTESIAN_POINT('Ctrl Pts',(-32.8129496113305,-7.07886051013307,
-36.1021710493883));
#24635=CARTESIAN_POINT('Ctrl Pts',(-32.7790942175002,-6.97591157388758,
-36.0910080560792));
#24636=CARTESIAN_POINT('Ctrl Pts',(-32.732840074035,-6.87711064623175,-36.089514373));
#24637=CARTESIAN_POINT('Ctrl Pts',(-32.6282205786628,-6.68740381001556,
-36.0970883927067));
#24638=CARTESIAN_POINT('Ctrl Pts',(-32.5695235872295,-6.59673597566758,
-36.1064563838958));
#24639=CARTESIAN_POINT('Ctrl Pts',(-32.4403205277421,-6.42451466437638,
-36.1356620593484));
#24640=CARTESIAN_POINT('Ctrl Pts',(-32.3709306102481,-6.34396835910597,
-36.1551041064734));
#24641=CARTESIAN_POINT('Ctrl Pts',(-32.2555947551915,-6.23614184370368,
-36.1953284657954));
#24642=CARTESIAN_POINT('Ctrl Pts',(-32.2153201817785,-6.2025085626214,-36.2105945165962));
#24643=CARTESIAN_POINT('Ctrl Pts',(-32.1306339787838,-6.1448363832171,-36.2466332237663));
#24644=CARTESIAN_POINT('Ctrl Pts',(-32.0860070936073,-6.11985717446073,
-36.2672504452137));
#24645=CARTESIAN_POINT('Ctrl Pts',(-32.0390884396291,-6.10843371318469,
-36.2934430901044));
#24646=CARTESIAN_POINT('Origin',(0.0835265683620477,-14.4544045823054,0.0824317919394229));
#24647=CARTESIAN_POINT('Origin',(-43.0351235939456,-14.4544045823054,-37.6801663496809));
#24648=CARTESIAN_POINT('Origin',(-46.3845835303221,-14.4544045823054,-37.9450121028891));
#24649=CARTESIAN_POINT('Origin',(6.83612114566778,-14.4544045823054,-20.3954556167886));
#24650=CARTESIAN_POINT('Origin',(-42.442236506563,-14.4544045823054,-36.6450210147876));
#24651=CARTESIAN_POINT('Ctrl Pts',(32.1333443923172,-14.4267018210609,-46.3767934681345));
#24652=CARTESIAN_POINT('Ctrl Pts',(32.1052213194306,-14.7669045823054,-46.3888540627253));
#24653=CARTESIAN_POINT('Ctrl Pts',(32.4199640389762,-14.7669045823054,-46.2552612894439));
#24654=CARTESIAN_POINT('Ctrl Pts',(32.1917878197712,-14.4797609665066,-46.5273115522008));
#24655=CARTESIAN_POINT('Ctrl Pts',(32.2108318123702,-14.7669045823054,-46.4982492296413));
#24656=CARTESIAN_POINT('Ctrl Pts',(32.5026074478398,-14.7669045823054,-46.4513285344375));
#24657=CARTESIAN_POINT('Ctrl Pts',(32.229426473191,-14.5360769750833,-46.6948057129722));
#24658=CARTESIAN_POINT('Ctrl Pts',(32.2987356959689,-14.7669045823054,-46.6757640436418));
#24659=CARTESIAN_POINT('Ctrl Pts',(32.5416287263888,-14.7669045823054,-46.6753447743204));
#24660=CARTESIAN_POINT('Ctrl Pts',(32.2303679539465,-14.6333609973512,-47.0050021456081));
#24661=CARTESIAN_POINT('Ctrl Pts',(32.3251131331188,-14.7669045823054,-47.028208228159));
#24662=CARTESIAN_POINT('Ctrl Pts',(32.4805743442183,-14.7669045823054,-47.1044264916346));
#24663=CARTESIAN_POINT('Ctrl Pts',(32.1934182263391,-14.6768299128517,-47.1557619332086));
#24664=CARTESIAN_POINT('Ctrl Pts',(32.2752623675051,-14.7669045823054,-47.222653288913));
#24665=CARTESIAN_POINT('Ctrl Pts',(32.3777047498528,-14.7669045823054,-47.3212251413928));
#24666=CARTESIAN_POINT('Ctrl Pts',(32.0821172043475,-14.6796363815827,-47.2014099893353));
#24667=CARTESIAN_POINT('Ctrl Pts',(32.1108290781635,-14.7669045823054,-47.2879256345056));
#24668=CARTESIAN_POINT('Ctrl Pts',(32.1539578388482,-14.7669045823054,-47.4064123788888));
#24669=CARTESIAN_POINT('Origin',(32.4575305290195,-14.4544045823054,-46.3554507110303));
#24670=CARTESIAN_POINT('Ctrl Pts',(29.4342239561067,-12.8919045823054,-38.184865357424));
#24671=CARTESIAN_POINT('Ctrl Pts',(29.5041756346414,-12.8919045823054,-38.3970004975819));
#24672=CARTESIAN_POINT('Ctrl Pts',(29.326104774044,-12.8919045823054,-38.5318534679819));
#24673=CARTESIAN_POINT('Ctrl Pts',(29.4342239819946,-13.0608832998917,-38.1848654359315));
#24674=CARTESIAN_POINT('Ctrl Pts',(29.5041756540699,-12.9975414109167,-38.397000556497));
#24675=CARTESIAN_POINT('Ctrl Pts',(29.3261047525712,-12.9763939382004,-38.5318534842432));
#24676=CARTESIAN_POINT('Ctrl Pts',(29.4582227637604,-13.226389889153,-38.2576440316728));
#24677=CARTESIAN_POINT('Ctrl Pts',(29.5231089112903,-13.1003236725302,-38.4544174656888));
#24678=CARTESIAN_POINT('Ctrl Pts',(29.3280674855906,-13.0591472399313,-38.5758498536463));
#24679=CARTESIAN_POINT('Ctrl Pts',(29.5354545666183,-13.4534586900123,-38.4918568435322));
#24680=CARTESIAN_POINT('Ctrl Pts',(29.5773853840454,-13.2166231342364,-38.6190160485472));
#24681=CARTESIAN_POINT('Ctrl Pts',(29.3346698006211,-13.1726816319567,-38.7171327311836));
#24682=CARTESIAN_POINT('Ctrl Pts',(29.5885432101734,-13.5169045492971,-38.6528532209924));
#24683=CARTESIAN_POINT('Ctrl Pts',(29.6131548298068,-13.22877512521,-38.7274903060458));
#24684=CARTESIAN_POINT('Ctrl Pts',(29.3393370685557,-13.2044045823054,-38.8141247129866));
#24685=CARTESIAN_POINT('Ctrl Pts',(29.6409337685891,-13.5169045823054,-38.8117325886538));
#24686=CARTESIAN_POINT('Ctrl Pts',(29.6409337685891,-13.2044045823054,-38.8117325886538));
#24687=CARTESIAN_POINT('Ctrl Pts',(29.344152791651,-13.2044045823054,-38.9095962781799));
#24688=CARTESIAN_POINT('Origin',(29.1374429791686,-12.8919045823054,-38.2827290469501));
#24689=CARTESIAN_POINT('Origin',(35.9713494567465,-12.8919045823054,-32.9119111827578));
#24690=CARTESIAN_POINT('Origin',(35.9713494567465,-12.8919045823054,-32.9119111827578));
#24691=CARTESIAN_POINT('Origin',(37.084741276154,-13.5169045823054,-41.2777797274919));
#24692=CARTESIAN_POINT('Origin',(37.084741276154,-13.5169045823054,-41.2777797274919));
#24693=CARTESIAN_POINT('Origin',(37.084741276154,-13.5169045823054,-41.2777797274919));
#24694=CARTESIAN_POINT('Ctrl Pts',(48.5200123991582,-14.4313124010524,-29.2902906970955));
#24695=CARTESIAN_POINT('Ctrl Pts',(48.4951461875456,-14.7671408702692,-29.2910694161602));
#24696=CARTESIAN_POINT('Ctrl Pts',(48.8317174987565,-14.7669045053135,-29.2782486346292));
#24697=CARTESIAN_POINT('Ctrl Pts',(48.5240400993535,-14.4776157931193,-29.4920731428274));
#24698=CARTESIAN_POINT('Ctrl Pts',(48.5483915150367,-14.767093222629,-29.4749018460235));
#24699=CARTESIAN_POINT('Ctrl Pts',(48.839758582342,-14.766904515933,-29.5041360916753));
#24700=CARTESIAN_POINT('Ctrl Pts',(48.5162454885462,-14.523222228705,-29.6899600092429));
#24701=CARTESIAN_POINT('Ctrl Pts',(48.5767120797059,-14.7670538266106,-29.6837089353061));
#24702=CARTESIAN_POINT('Ctrl Pts',(48.8241497473579,-14.7669045263941,-29.7260699064196));
#24703=CARTESIAN_POINT('Ctrl Pts',(48.4707526949274,-14.6124212350926,-30.0755282599531));
#24704=CARTESIAN_POINT('Ctrl Pts',(48.562869586275,-14.7669897766053,-30.0922753233648));
#24705=CARTESIAN_POINT('Ctrl Pts',(48.733120429625,-14.7669045468573,-30.1592298113981));
#24706=CARTESIAN_POINT('Ctrl Pts',(48.4343451232206,-14.657050343383,-30.2676432276275));
#24707=CARTESIAN_POINT('Ctrl Pts',(48.5298010855454,-14.7669625172313,-30.3030569514312));
#24708=CARTESIAN_POINT('Ctrl Pts',(48.6597403312579,-14.766904557097,-30.3763073223494));
#24709=CARTESIAN_POINT('Ctrl Pts',(48.3623819262458,-14.6947854519682,-30.4295590745031));
#24710=CARTESIAN_POINT('Ctrl Pts',(48.4294306773109,-14.7669413153234,-30.4853582482525));
#24711=CARTESIAN_POINT('Ctrl Pts',(48.5166376573611,-14.7669045657556,-30.5574434433174));
#24712=CARTESIAN_POINT('Origin',(48.5824772699512,-14.4544045823054,-30.4639852003988));
#24713=CARTESIAN_POINT('Origin',(48.8335265683622,-14.4544045823054,-29.39085169964));
#24714=CARTESIAN_POINT('Ctrl Pts',(48.3955019191571,-14.6753754514261,-30.3462212704575));
#24715=CARTESIAN_POINT('Ctrl Pts',(48.4059549771833,-14.6685167481301,-30.3167552206967));
#24716=CARTESIAN_POINT('Ctrl Pts',(48.4153181071138,-14.6615856670197,-30.2869594234401));
#24717=CARTESIAN_POINT('Ctrl Pts',(48.4237914685547,-14.6546090802607,-30.2569496411699));
#24718=CARTESIAN_POINT('Ctrl Pts',(48.4330908949959,-14.646952348534,-30.2240142158746));
#24719=CARTESIAN_POINT('Ctrl Pts',(48.4413185922837,-14.6392407575335,-30.1908208469554));
#24720=CARTESIAN_POINT('Ctrl Pts',(48.448693282195,-14.6314992383765,-30.157477015652));
#24721=CARTESIAN_POINT('Ctrl Pts',(48.4565789660921,-14.6232213075498,-30.1218227824927));
#24722=CARTESIAN_POINT('Ctrl Pts',(48.4634889654078,-14.6149090026934,-30.0859958597154));
#24723=CARTESIAN_POINT('Ctrl Pts',(48.4696439731935,-14.6065829337798,-30.0500850635473));
#24724=CARTESIAN_POINT('Ctrl Pts',(48.4767477541929,-14.5969734300704,-30.0086387420524));
#24725=CARTESIAN_POINT('Ctrl Pts',(48.4828456977915,-14.5873453832268,-29.9670798327071));
#24726=CARTESIAN_POINT('Ctrl Pts',(48.4882202022897,-14.5777205278782,-29.9255015399208));
#24727=CARTESIAN_POINT('Ctrl Pts',(48.4900623043444,-14.5744216254734,-29.9112506524953));
#24728=CARTESIAN_POINT('Ctrl Pts',(48.4918190010901,-14.5711230389451,-29.8969972272884));
#24729=CARTESIAN_POINT('Ctrl Pts',(48.4935005335227,-14.5678255143183,-29.882744437463));
#24730=CARTESIAN_POINT('Ctrl Pts',(48.4938922373557,-14.5670573738945,-29.8794243276061));
#24731=CARTESIAN_POINT('Ctrl Pts',(48.4942794778329,-14.5662889835649,-29.8761029367338));
#24732=CARTESIAN_POINT('Ctrl Pts',(48.4946622853821,-14.5655203189316,-29.8727801599688));
#24733=CARTESIAN_POINT('Ctrl Pts',(48.5045170298835,-14.5457323247156,-29.7872407913554));
#24734=CARTESIAN_POINT('Ctrl Pts',(48.5113680830515,-14.5259112556565,-29.7014082137169));
#24735=CARTESIAN_POINT('Ctrl Pts',(48.5156165893993,-14.5060682995342,-29.615326399795));
#24736=CARTESIAN_POINT('Ctrl Pts',(48.5193003967565,-14.4888628108826,-29.5406863278512));
#24737=CARTESIAN_POINT('Ctrl Pts',(48.5210264259617,-14.4716407563751,-29.4658584862374));
#24738=CARTESIAN_POINT('Ctrl Pts',(48.5210265683534,-14.454406712551,-29.390860969846));
#24739=CARTESIAN_POINT('Origin',(48.8335265683622,-14.4544045823054,-44.2925682080603));
#24740=CARTESIAN_POINT('Origin',(48.8335265683619,-14.4544045823054,29.5557152835192));
#24741=CARTESIAN_POINT('Ctrl Pts',(48.5210265683619,-14.9741386829693,30.5390391682904));
#24742=CARTESIAN_POINT('Ctrl Pts',(48.521026568362,-14.8357920829888,30.6130226887234));
#24743=CARTESIAN_POINT('Ctrl Pts',(48.3952116457107,-14.7531448966902,30.657219870274));
#24744=CARTESIAN_POINT('Ctrl Pts',(48.5210265683619,-13.8793029117135,28.4917345041611));
#24745=CARTESIAN_POINT('Ctrl Pts',(48.521026568362,-13.7458678867053,28.5689805591673));
#24746=CARTESIAN_POINT('Ctrl Pts',(48.398801943192,-13.65830753268,28.6042407855062));
#24747=CARTESIAN_POINT('Ctrl Pts',(48.521026568362,-12.8434482902991,26.4086832687539));
#24748=CARTESIAN_POINT('Ctrl Pts',(48.521026568362,-12.7103751542363,26.4815899293964));
#24749=CARTESIAN_POINT('Ctrl Pts',(48.4024091291961,-12.6224528665228,26.5149273450437));
#24750=CARTESIAN_POINT('Ctrl Pts',(48.521026568362,-11.4077451872927,23.2124561823835));
#24751=CARTESIAN_POINT('Ctrl Pts',(48.521026568362,-11.2735898053172,23.2727809677033));
#24752=CARTESIAN_POINT('Ctrl Pts',(48.4076725172434,-11.186749940031,23.3082345578824));
#24753=CARTESIAN_POINT('Ctrl Pts',(48.521026568362,-10.9489604127228,22.1350468218994));
#24754=CARTESIAN_POINT('Ctrl Pts',(48.521026568362,-10.8151504288079,22.1928971400193));
#24755=CARTESIAN_POINT('Ctrl Pts',(48.4094014640764,-10.727965027292,22.2271571198222));
#24756=CARTESIAN_POINT('Ctrl Pts',(48.521026568362,-10.0773547210577,19.9523464052027));
#24757=CARTESIAN_POINT('Ctrl Pts',(48.521026568362,-9.94441815657111,20.0051547930602));
#24758=CARTESIAN_POINT('Ctrl Pts',(48.4127662077947,-9.85635900888213,20.0367328014427));
#24759=CARTESIAN_POINT('Ctrl Pts',(48.521026568362,-9.6651241319502,18.8479737078929));
#24760=CARTESIAN_POINT('Ctrl Pts',(48.521026568362,-9.53246556458668,18.898045866283));
#24761=CARTESIAN_POINT('Ctrl Pts',(48.4143999302067,-9.4441283020868,18.9283064327585));
#24762=CARTESIAN_POINT('Ctrl Pts',(48.521026568362,-7.75733423685905,13.3094986281149));
#24763=CARTESIAN_POINT('Ctrl Pts',(48.521026568362,-7.63508483859962,13.3708195365843));
#24764=CARTESIAN_POINT('Ctrl Pts',(48.4221223344704,-7.53633525782046,13.368780830614));
#24765=CARTESIAN_POINT('Ctrl Pts',(48.521026568362,-6.70462823796833,8.78094500538595));
#24766=CARTESIAN_POINT('Ctrl Pts',(48.521026568362,-6.57519149763907,8.81202019284637));
#24767=CARTESIAN_POINT('Ctrl Pts',(48.4269222766975,-6.48363668556734,8.82066537173487));
#24768=CARTESIAN_POINT('Ctrl Pts',(48.521026568362,-6.31501530004508,4.11515277179024));
#24769=CARTESIAN_POINT('Ctrl Pts',(48.5210265683621,-6.18536424665105,4.12597917065639));
#24770=CARTESIAN_POINT('Ctrl Pts',(48.4286992393282,-6.09401826674915,4.13360693755336));
#24771=CARTESIAN_POINT('Ctrl Pts',(48.3955019191565,-14.6753754514262,30.5110848543364));
#24772=CARTESIAN_POINT('Ctrl Pts',(48.4052064423862,-14.6690078941722,30.4837288439063));
#24773=CARTESIAN_POINT('Ctrl Pts',(48.4139628772557,-14.6625738073748,30.4560706196742));
#24774=CARTESIAN_POINT('Ctrl Pts',(48.4219415507532,-14.6560985772181,30.4282197016506));
#24775=CARTESIAN_POINT('Ctrl Pts',(48.4304079610655,-14.649227515833,30.3986662552492));
#24776=CARTESIAN_POINT('Ctrl Pts',(48.437998422541,-14.642310020426,30.3688953829949));
#24777=CARTESIAN_POINT('Ctrl Pts',(48.4448791359127,-14.6353661273908,30.3389935466465));
#24778=CARTESIAN_POINT('Ctrl Pts',(48.4525470064664,-14.6276278493874,30.3056709246955));
#24779=CARTESIAN_POINT('Ctrl Pts',(48.459333447508,-14.6198566891109,30.2721852455818));
#24780=CARTESIAN_POINT('Ctrl Pts',(48.4654246307801,-14.6120695184222,30.238609179989));
#24781=CARTESIAN_POINT('Ctrl Pts',(48.4722050743052,-14.6034011745691,30.2012337462881));
#24782=CARTESIAN_POINT('Ctrl Pts',(48.4781237366281,-14.5947127249934,30.1637451913772));
#24783=CARTESIAN_POINT('Ctrl Pts',(48.4833879588141,-14.586017636216,30.126200917409));
#24784=CARTESIAN_POINT('Ctrl Pts',(48.4871194262825,-14.5798542487752,30.0995882038902));
#24785=CARTESIAN_POINT('Ctrl Pts',(48.4905209582135,-14.5736872964226,30.0729464959421));
#24786=CARTESIAN_POINT('Ctrl Pts',(48.4936555202531,-14.5675203997113,30.0462908924709));
#24787=CARTESIAN_POINT('Ctrl Pts',(48.4939882725562,-14.5668657471449,30.0434612424802));
#24788=CARTESIAN_POINT('Ctrl Pts',(48.4943178162041,-14.5662108690007,30.0406304700051));
#24789=CARTESIAN_POINT('Ctrl Pts',(48.494644170793,-14.5655557443929,30.037798484972));
#24790=CARTESIAN_POINT('Ctrl Pts',(48.5055255724454,-14.5437124051737,29.9433736854619));
#24791=CARTESIAN_POINT('Ctrl Pts',(48.5127481549386,-14.5218400677965,29.8486407866783));
#24792=CARTESIAN_POINT('Ctrl Pts',(48.5168466348194,-14.4999508808714,29.7536469513485));
#24793=CARTESIAN_POINT('Ctrl Pts',(48.5196878200913,-14.48477666084,29.6877944661076));
#24794=CARTESIAN_POINT('Ctrl Pts',(48.5210264418471,-14.4695942532302,29.6218162870134));
#24795=CARTESIAN_POINT('Ctrl Pts',(48.521026568353,-14.4544067340556,29.555724647307));
#24796=CARTESIAN_POINT('Ctrl Pts',(48.3952465904111,-14.7531486984911,-30.4923081869096));
#24797=CARTESIAN_POINT('Ctrl Pts',(48.5210265683622,-14.8357969973015,-30.4481104474598));
#24798=CARTESIAN_POINT('Ctrl Pts',(48.5210265683622,-14.9741195676119,-30.3741398393454));
#24799=CARTESIAN_POINT('Ctrl Pts',(48.3988351428458,-13.6585793127145,-28.4398295995618));
#24800=CARTESIAN_POINT('Ctrl Pts',(48.5210265683622,-13.7461362596315,-28.40456192777));
#24801=CARTESIAN_POINT('Ctrl Pts',(48.5210265683622,-13.879550318061,-28.3273318462602));
#24802=CARTESIAN_POINT('Ctrl Pts',(48.4024400771286,-12.6231097579334,-26.3512944596022));
#24803=CARTESIAN_POINT('Ctrl Pts',(48.521026568354,-12.7110265271815,-26.3179447507229));
#24804=CARTESIAN_POINT('Ctrl Pts',(48.5210265683621,-12.8440806269501,-26.2450560710985));
#24805=CARTESIAN_POINT('Ctrl Pts',(48.4076994021303,-11.1881005852606,-23.1464093060635));
#24806=CARTESIAN_POINT('Ctrl Pts',(48.5210265683662,-11.2749369501022,-23.1109499665448));
#24807=CARTESIAN_POINT('Ctrl Pts',(48.5210265683621,-11.4090714544335,-23.0506307223895));
#24808=CARTESIAN_POINT('Ctrl Pts',(48.4094268834328,-10.7295656511245,-22.0660426670943));
#24809=CARTESIAN_POINT('Ctrl Pts',(48.5210265683621,-10.8167469967087,-22.0317755238263));
#24810=CARTESIAN_POINT('Ctrl Pts',(48.5210265683621,-10.9505365201845,-21.9739291535892));
#24811=CARTESIAN_POINT('Ctrl Pts',(48.4127885702549,-9.85847188921516,-19.877309020907));
#24812=CARTESIAN_POINT('Ctrl Pts',(48.5210265683621,-9.94652588376348,-19.8457214596911));
#24813=CARTESIAN_POINT('Ctrl Pts',(48.5210265683621,-10.0794427583968,-19.7929119202474));
#24814=CARTESIAN_POINT('Ctrl Pts',(48.4144238368348,-9.44570717935303,-18.767774646125));
#24815=CARTESIAN_POINT('Ctrl Pts',(48.5210265683621,-9.53404162556802,-18.7375113137474));
#24816=CARTESIAN_POINT('Ctrl Pts',(48.5210265683621,-9.66667804843002,-18.687434330509));
#24817=CARTESIAN_POINT('Ctrl Pts',(48.4221518448129,-7.53595817693283,-13.2034873916435));
#24818=CARTESIAN_POINT('Ctrl Pts',(48.5210265683621,-7.63471881015773,-13.2055633861815));
#24819=CARTESIAN_POINT('Ctrl Pts',(48.5210265683621,-7.75692904622885,-13.1442050984742));
#24820=CARTESIAN_POINT('Ctrl Pts',(48.4269499128865,-6.48350292014371,-8.65379177962918));
#24821=CARTESIAN_POINT('Ctrl Pts',(48.5210265683621,-6.57505277912449,-8.64513862080266));
#24822=CARTESIAN_POINT('Ctrl Pts',(48.5210265683621,-6.7044683038842,-8.61408311837201));
#24823=CARTESIAN_POINT('Ctrl Pts',(48.4287256539129,-6.0940504675403,-3.96881378790178));
#24824=CARTESIAN_POINT('Ctrl Pts',(48.5210265683621,-6.18539206100946,-3.96118625151467));
#24825=CARTESIAN_POINT('Ctrl Pts',(48.5210265683621,-6.3150213366611,-3.95036147849161));
#24826=CARTESIAN_POINT('Origin',(0.0835265683620477,-5.88746284406389,0.0824317919394229));
#24827=CARTESIAN_POINT('Ctrl Pts',(-32.8357348152455,-7.15534954835,-36.112467064513));
#24828=CARTESIAN_POINT('Ctrl Pts',(-32.2618480320884,-7.11664814651665,
-35.9774429580661));
#24829=CARTESIAN_POINT('Ctrl Pts',(-32.6948231655917,-7.18677502448105,
-35.579476484273));
#24830=CARTESIAN_POINT('Ctrl Pts',(-32.8046268621034,-7.03238137403248,
-36.0929336019227));
#24831=CARTESIAN_POINT('Ctrl Pts',(-32.335349467333,-7.08021162563639,-35.9101513087856));
#24832=CARTESIAN_POINT('Ctrl Pts',(-32.7096701034189,-7.01162141060435,
-35.5658010590506));
#24833=CARTESIAN_POINT('Ctrl Pts',(-32.7467976083082,-6.90078625143033,
-36.0884640630633));
#24834=CARTESIAN_POINT('Ctrl Pts',(-32.3803176716213,-6.94927177586967,
-35.868405044745));
#24835=CARTESIAN_POINT('Ctrl Pts',(-32.6866182194288,-6.83269992246191,
-35.5870611421423));
#24836=CARTESIAN_POINT('Ctrl Pts',(-32.6223425009383,-6.67697195553557,
-36.0980619499061));
#24837=CARTESIAN_POINT('Ctrl Pts',(-32.3864006309704,-6.69622936404148,
-35.8617356014171));
#24838=CARTESIAN_POINT('Ctrl Pts',(-32.6060083690053,-6.53795985193926,
-35.6609320351416));
#24839=CARTESIAN_POINT('Ctrl Pts',(-32.5593650752754,-6.58104909157614,
-36.1085254356579));
#24840=CARTESIAN_POINT('Ctrl Pts',(-32.3705503505499,-6.57996991861,-35.8757369426306));
#24841=CARTESIAN_POINT('Ctrl Pts',(-32.5561766297544,-6.41511471179757,
-35.7065091093568));
#24842=CARTESIAN_POINT('Ctrl Pts',(-32.4216517252779,-6.40173475569596,
-36.1409145226018));
#24843=CARTESIAN_POINT('Ctrl Pts',(-32.3043563189527,-6.36383534698789,
-35.9348896071862));
#24844=CARTESIAN_POINT('Ctrl Pts',(-32.4313800558606,-6.19278444406334,
-35.8199269455543));
#24845=CARTESIAN_POINT('Ctrl Pts',(-32.3490446219505,-6.32050524456491,
-36.1621510538971));
#24846=CARTESIAN_POINT('Ctrl Pts',(-32.2579524400761,-6.26307762141883,
-35.9764869904755));
#24847=CARTESIAN_POINT('Ctrl Pts',(-32.3586632722149,-6.09580032219761,
-35.885741986965));
#24848=CARTESIAN_POINT('Ctrl Pts',(-32.1728567843285,-6.16373114062077,
-36.2258902003226));
#24849=CARTESIAN_POINT('Ctrl Pts',(-32.1199675885256,-6.07811517887309,
-36.0995837961962));
#24850=CARTESIAN_POINT('Ctrl Pts',(-32.1613068720281,-5.92198390397422,
-36.0628852537019));
#24851=CARTESIAN_POINT('Ctrl Pts',(-32.0704722290187,-6.09886182625026,
-36.2708256880667));
#24852=CARTESIAN_POINT('Ctrl Pts',(-32.0211351392778,-6.00005797774296,
-36.1874132622081));
#24853=CARTESIAN_POINT('Ctrl Pts',(-32.0323399058407,-5.8609798928657,-36.1777020688111));
#24854=CARTESIAN_POINT('Ctrl Pts',(-31.984476267574,-6.10268725738808,-36.3263280849565));
#24855=CARTESIAN_POINT('Ctrl Pts',(-31.9158280229635,-6.01584203958953,
-36.2800888384076));
#24856=CARTESIAN_POINT('Ctrl Pts',(-31.8955666163655,-5.89881153274382,
-36.2978988244376));
#24857=CARTESIAN_POINT('Origin',(-32.9108164063353,-7.07886995352309,-35.8053910964449));
#24858=CARTESIAN_POINT('Ctrl Pts',(-39.0316791043431,-12.5761796977906,
-38.5782243155831));
#24859=CARTESIAN_POINT('Ctrl Pts',(-39.3109914885678,-12.4966730216632,
-38.1825612826739));
#24860=CARTESIAN_POINT('Ctrl Pts',(-38.971148947661,-12.8445798972116,-38.1292868882747));
#24861=CARTESIAN_POINT('Ctrl Pts',(-39.2137986964445,-12.7679658886679,
-38.6667648301433));
#24862=CARTESIAN_POINT('Ctrl Pts',(-39.3414646993651,-12.6138199372453,
-38.3175461156564));
#24863=CARTESIAN_POINT('Ctrl Pts',(-39.1576103554185,-12.9405865508059,
-38.2051080058143));
#24864=CARTESIAN_POINT('Ctrl Pts',(-39.4489244282751,-12.9477999797135,
-38.6846342775079));
#24865=CARTESIAN_POINT('Ctrl Pts',(-39.5079883732932,-12.8036087634352,
-38.4182266108569));
#24866=CARTESIAN_POINT('Ctrl Pts',(-39.3833967701386,-13.030416913756,-38.2499881397961));
#24867=CARTESIAN_POINT('Ctrl Pts',(-39.7877827367345,-13.1418528526573,
-38.6147444629907));
#24868=CARTESIAN_POINT('Ctrl Pts',(-39.7939468272625,-13.0167291165573,
-38.4286787464956));
#24869=CARTESIAN_POINT('Ctrl Pts',(-39.6946150246688,-13.1274080636027,
-38.2623293930186));
#24870=CARTESIAN_POINT('Ctrl Pts',(-39.8900642233608,-13.1924895597097,
-38.5820003624405));
#24871=CARTESIAN_POINT('Ctrl Pts',(-39.8794472263271,-13.0721360087909,
-38.4198017475188));
#24872=CARTESIAN_POINT('Ctrl Pts',(-39.7868043174562,-13.1527155106486,
-38.2596713162932));
#24873=CARTESIAN_POINT('Ctrl Pts',(-40.1316643013097,-13.2848578326182,
-38.4643918227783));
#24874=CARTESIAN_POINT('Ctrl Pts',(-40.0814925592654,-13.1766908654357,
-38.3602649823531));
#24875=CARTESIAN_POINT('Ctrl Pts',(-39.9985161138346,-13.1988763557094,
-38.2313292757146));
#24876=CARTESIAN_POINT('Ctrl Pts',(-40.2695202623444,-13.3151873395668,
-38.3641621129247));
#24877=CARTESIAN_POINT('Ctrl Pts',(-40.2032404760251,-13.2202535090907,
-38.2959303147521));
#24878=CARTESIAN_POINT('Ctrl Pts',(-40.1140491542167,-13.2140287022007,
-38.1971624146867));
#24879=CARTESIAN_POINT('Ctrl Pts',(-40.36214506113,-13.282303056079,-38.2184712301346));
#24880=CARTESIAN_POINT('Ctrl Pts',(-40.2816124286873,-13.2034487358305,
-38.1888336787549));
#24881=CARTESIAN_POINT('Ctrl Pts',(-40.180730391081,-13.1975864244367,-38.1308214755661));
#24882=CARTESIAN_POINT('Ctrl Pts',(-40.1126065460396,-13.2044045823054,
-38.1801853354021));
#24883=CARTESIAN_POINT('Ctrl Pts',(-40.1003695133337,-13.2044045823054,
-38.1867765902176));
#24884=CARTESIAN_POINT('Ctrl Pts',(-40.0878695495467,-13.2039200465849,
-38.19269233339));
#24885=CARTESIAN_POINT('Ctrl Pts',(-40.0751776324174,-13.2030865921358,
-38.1980323342018));
#24886=CARTESIAN_POINT('Ctrl Pts',(-40.0619624470289,-13.2022187756393,
-38.2035924950493));
#24887=CARTESIAN_POINT('Ctrl Pts',(-40.048538896247,-13.2009724747263,-38.2085292430206));
#24888=CARTESIAN_POINT('Ctrl Pts',(-40.034981169135,-13.199446062585,-38.2129732000915));
#24889=CARTESIAN_POINT('Ctrl Pts',(-40.0206856861494,-13.1978365893588,
-38.2176589790698));
#24890=CARTESIAN_POINT('Ctrl Pts',(-40.0062407990922,-13.1959155151287,
-38.2217975674052));
#24891=CARTESIAN_POINT('Ctrl Pts',(-39.9917308687064,-13.1937414656795,
-38.2255500088239));
#24892=CARTESIAN_POINT('Ctrl Pts',(-39.9884831597464,-13.1932548554968,
-38.2263899051772));
#24893=CARTESIAN_POINT('Ctrl Pts',(-39.985232189899,-13.1927553638524,-38.2272104632462));
#24894=CARTESIAN_POINT('Ctrl Pts',(-39.9819789051098,-13.1922433006301,
-38.2280134889338));
#24895=CARTESIAN_POINT('Ctrl Pts',(-39.9634767074475,-13.1893310763501,
-38.2325804853579));
#24896=CARTESIAN_POINT('Ctrl Pts',(-39.9449286065895,-13.1860397456251,
-38.2365036772376));
#24897=CARTESIAN_POINT('Ctrl Pts',(-39.9263423823089,-13.1824628010599,
-38.2398884352376));
#24898=CARTESIAN_POINT('Ctrl Pts',(-39.9067872179013,-13.1786993826273,
-38.2434496480031));
#24899=CARTESIAN_POINT('Ctrl Pts',(-39.8871896035564,-13.1746195596086,
-38.2464155761614));
#24900=CARTESIAN_POINT('Ctrl Pts',(-39.8675581906585,-13.1702746943005,
-38.2489101863332));
#24901=CARTESIAN_POINT('Ctrl Pts',(-39.8606574942543,-13.1687474177584,
-38.2497870741829));
#24902=CARTESIAN_POINT('Ctrl Pts',(-39.8537526355299,-13.1671869117775,
-38.2506056832564));
#24903=CARTESIAN_POINT('Ctrl Pts',(-39.846844060365,-13.1655939279677,-38.2513711852016));
#24904=CARTESIAN_POINT('Ctrl Pts',(-39.8208523950992,-13.1596007526788,
-38.2542511814158));
#24905=CARTESIAN_POINT('Ctrl Pts',(-39.7949454183915,-13.1531817886309,
-38.2563668768381));
#24906=CARTESIAN_POINT('Ctrl Pts',(-39.7691247502535,-13.1464435609449,
-38.2578143352514));
#24907=CARTESIAN_POINT('Ctrl Pts',(-39.7424132520525,-13.1394728599642,
-38.2593117319337));
#24908=CARTESIAN_POINT('Ctrl Pts',(-39.7157938410967,-13.1321600180536,
-38.2600948344691));
#24909=CARTESIAN_POINT('Ctrl Pts',(-39.6892696413194,-13.1245659628583,
-38.2602659618575));
#24910=CARTESIAN_POINT('Ctrl Pts',(-39.6616326372886,-13.1166533043878,
-38.2604442687758));
#24911=CARTESIAN_POINT('Ctrl Pts',(-39.6340987346077,-13.1084348255795,
-38.259958981435));
#24912=CARTESIAN_POINT('Ctrl Pts',(-39.6066771721502,-13.0999262547332,
-38.2589085438143));
#24913=CARTESIAN_POINT('Ctrl Pts',(-39.5972925130951,-13.0970143113834,
-38.2585490457389));
#24914=CARTESIAN_POINT('Ctrl Pts',(-39.587921077564,-13.094067983939,-38.2581231550883));
#24915=CARTESIAN_POINT('Ctrl Pts',(-39.5785634617679,-13.0910867263844,
-38.2576341329803));
#24916=CARTESIAN_POINT('Ctrl Pts',(-39.5440886722257,-13.0801033488869,
-38.2558325058752));
#24917=CARTESIAN_POINT('Ctrl Pts',(-39.5097942337352,-13.0686901791307,
-38.2531377665943));
#24918=CARTESIAN_POINT('Ctrl Pts',(-39.4757046982075,-13.0568974025755,
-38.2496165062848));
#24919=CARTESIAN_POINT('Ctrl Pts',(-39.4405664062734,-13.0447418240704,
-38.2459869152442));
#24920=CARTESIAN_POINT('Ctrl Pts',(-39.4056455162936,-13.0321818870426,
-38.2414800828879));
#24921=CARTESIAN_POINT('Ctrl Pts',(-39.3709807148931,-13.0192318837648,
-38.2361331579378));
#24922=CARTESIAN_POINT('Ctrl Pts',(-39.3367760709274,-13.0064537851295,
-38.2308572106702));
#24923=CARTESIAN_POINT('Ctrl Pts',(-39.3028206159918,-12.9932945861615,
-38.2247637684813));
#24924=CARTESIAN_POINT('Ctrl Pts',(-39.2691660449372,-12.9797471343051,
-38.2178444611905));
#24925=CARTESIAN_POINT('Ctrl Pts',(-39.2348323379837,-12.9659263002422,
-38.2107855250221));
#24926=CARTESIAN_POINT('Ctrl Pts',(-39.2008115903465,-12.9516999140197,
-38.2028676339683));
#24927=CARTESIAN_POINT('Ctrl Pts',(-39.1671765836779,-12.9370593466235,
-38.1940276365451));
#24928=CARTESIAN_POINT('Ctrl Pts',(-39.1363330539154,-12.923633846796,-38.1859212988146));
#24929=CARTESIAN_POINT('Ctrl Pts',(-39.1058140642328,-12.9098590019422,
-38.1770390451456));
#24930=CARTESIAN_POINT('Ctrl Pts',(-39.0756901950279,-12.8957449858576,
-38.1672883346991));
#24931=CARTESIAN_POINT('Ctrl Pts',(-39.0729638506097,-12.894467604499,-38.1664058519471));
#24932=CARTESIAN_POINT('Ctrl Pts',(-39.0702407521924,-12.8931874634454,
-38.1655162266651));
#24933=CARTESIAN_POINT('Ctrl Pts',(-39.0675209577957,-12.8919045823054,
-38.1646193729747));
#24934=CARTESIAN_POINT('Origin',(-40.1126065460396,-13.5169045823054,-38.1801853354021));
#24935=CARTESIAN_POINT('Ctrl Pts',(-42.7963830377277,-14.6563598281152,
-37.572732204214));
#24936=CARTESIAN_POINT('Ctrl Pts',(-42.8482224231091,-14.7669045823027,
-37.64926336932));
#24937=CARTESIAN_POINT('Ctrl Pts',(-42.9289078842538,-14.7669045823054,
-37.769437584449));
#24938=CARTESIAN_POINT('Ctrl Pts',(-42.858102552525,-14.6732979129424,-37.5515771497065));
#24939=CARTESIAN_POINT('Ctrl Pts',(-42.9221643671718,-14.7669045823064,
-37.6214949477829));
#24940=CARTESIAN_POINT('Ctrl Pts',(-43.0171700719925,-14.7669045823054,
-37.7163455316033));
#24941=CARTESIAN_POINT('Ctrl Pts',(-42.9046371348531,-14.6836226395017,
-37.511596293802));
#24942=CARTESIAN_POINT('Ctrl Pts',(-42.9828541398335,-14.7669045823055,
-37.5612377434468));
#24943=CARTESIAN_POINT('Ctrl Pts',(-43.0894948610397,-14.7669045823054,
-37.6289001478671));
#24944=CARTESIAN_POINT('Ctrl Pts',(-42.930578525807,-14.6837071744118,-37.4337545567665));
#24945=CARTESIAN_POINT('Ctrl Pts',(-43.0197879756039,-14.7669045823053,
-37.4502266440492));
#24946=CARTESIAN_POINT('Ctrl Pts',(-43.1413666883037,-14.7669045823054,
-37.4726705102553));
#24947=CARTESIAN_POINT('Ctrl Pts',(-42.9305937454166,-14.6805726740673,
-37.4030029435815));
#24948=CARTESIAN_POINT('Ctrl Pts',(-43.0218035062137,-14.7669045823054,
-37.4068468927024));
#24949=CARTESIAN_POINT('Ctrl Pts',(-43.1478444705321,-14.7669045823054,
-37.4130984790331));
#24950=CARTESIAN_POINT('Ctrl Pts',(-42.9062631519066,-14.6635276241068,
-37.3097719517883));
#24951=CARTESIAN_POINT('Ctrl Pts',(-42.9975785139956,-14.7669045823054,
-37.2792440170877));
#24952=CARTESIAN_POINT('Ctrl Pts',(-43.134092223999,-14.7669045823054,-37.2376557184966));
#24953=CARTESIAN_POINT('Ctrl Pts',(-42.8588599809403,-14.6424796666932,
-37.2472449190099));
#24954=CARTESIAN_POINT('Ctrl Pts',(-42.9410778224509,-14.7669045823058,
-37.1988871414035));
#24955=CARTESIAN_POINT('Ctrl Pts',(-43.082276268341,-14.7669045823054,-37.1265846080327));
#24956=CARTESIAN_POINT('Ctrl Pts',(-42.6561292830181,-14.560778522968,-37.0605332449033));
#24957=CARTESIAN_POINT('Ctrl Pts',(-42.6929533769163,-14.7669045823044,
-36.9765311644006));
#24958=CARTESIAN_POINT('Ctrl Pts',(-42.8437843379004,-14.7669045823054,
-36.808037040221));
#24959=CARTESIAN_POINT('Ctrl Pts',(-42.4452340977281,-14.485990546607,-36.9651610952557));
#24960=CARTESIAN_POINT('Ctrl Pts',(-42.4208805578758,-14.7669045823061,
-36.9206538390427));
#24961=CARTESIAN_POINT('Ctrl Pts',(-42.5749664504047,-14.7669045823054,
-36.6685486138914));
#24962=CARTESIAN_POINT('Ctrl Pts',(-42.2429004856065,-14.4183787521208,
-36.9115565886974));
#24963=CARTESIAN_POINT('Ctrl Pts',(-42.23469723594,-14.7669045823051,-36.9519162686243));
#24964=CARTESIAN_POINT('Ctrl Pts',(-42.3098537353251,-14.7669045823054,
-36.6082395787205));
#24965=CARTESIAN_POINT('Ctrl Pts',(-42.3443728681154,-14.4544045238107,
-36.9418020085688));
#24966=CARTESIAN_POINT('Ctrl Pts',(-42.3737106494897,-14.4643868520267,
-36.9514761580288));
#24967=CARTESIAN_POINT('Ctrl Pts',(-42.4027641035859,-14.4744011867389,
-36.9619828372566));
#24968=CARTESIAN_POINT('Ctrl Pts',(-42.4314670014265,-14.4844099197098,
-36.9733072590746));
#24969=CARTESIAN_POINT('Ctrl Pts',(-42.4596712580304,-14.4942447759171,
-36.9844349473177));
#24970=CARTESIAN_POINT('Ctrl Pts',(-42.4875385896839,-14.5040728389242,
-36.996351552873));
#24971=CARTESIAN_POINT('Ctrl Pts',(-42.5150050555123,-14.5138432176011,
-37.0090909967157));
#24972=CARTESIAN_POINT('Ctrl Pts',(-42.5401900236358,-14.5228020212953,
-37.0207722406403));
#24973=CARTESIAN_POINT('Ctrl Pts',(-42.5650389656366,-14.5317110776815,
-37.0331459059695));
#24974=CARTESIAN_POINT('Ctrl Pts',(-42.5894839867309,-14.5405368969068,
-37.0462776461334));
#24975=CARTESIAN_POINT('Ctrl Pts',(-42.6126265157218,-14.5488924543229,
-37.0587096942085));
#24976=CARTESIAN_POINT('Ctrl Pts',(-42.6354077244154,-14.5571724059617,
-37.0718219993755));
#24977=CARTESIAN_POINT('Ctrl Pts',(-42.6577407274503,-14.5653692837009,
-37.0856974585248));
#24978=CARTESIAN_POINT('Ctrl Pts',(-42.6784000406813,-14.5729518673985,
-37.0985330568696));
#24979=CARTESIAN_POINT('Ctrl Pts',(-42.6986760027707,-14.5804628051684,
-37.1120227658321));
#24980=CARTESIAN_POINT('Ctrl Pts',(-42.7184682792969,-14.587925101972,-37.1262428650811));
#24981=CARTESIAN_POINT('Ctrl Pts',(-42.728622039289,-14.5917533816866,-37.1335380074387));
#24982=CARTESIAN_POINT('Ctrl Pts',(-42.7386479513117,-14.5955693937988,
-37.1410254719861));
#24983=CARTESIAN_POINT('Ctrl Pts',(-42.7485287260783,-14.5993802185557,
-37.1487152165534));
#24984=CARTESIAN_POINT('Ctrl Pts',(-42.7616540438129,-14.604442401122,-37.1589300370636));
#24985=CARTESIAN_POINT('Ctrl Pts',(-42.7745538904303,-14.6095732512804,
-37.1694686330813));
#24986=CARTESIAN_POINT('Ctrl Pts',(-42.7871269159706,-14.6146451518332,
-37.1804202089125));
#24987=CARTESIAN_POINT('Ctrl Pts',(-42.7989080093126,-14.6193975905872,
-37.1906819821584));
#24988=CARTESIAN_POINT('Ctrl Pts',(-42.8104022403622,-14.6240978916553,
-37.2013072124028));
#24989=CARTESIAN_POINT('Ctrl Pts',(-42.8214944105973,-14.6286695523063,
-37.2123820369564));
#24990=CARTESIAN_POINT('Ctrl Pts',(-42.8321400773418,-14.6330571856305,
-37.2230110562515));
#24991=CARTESIAN_POINT('Ctrl Pts',(-42.8424154792447,-14.6373259480378,
-37.2340550798162));
#24992=CARTESIAN_POINT('Ctrl Pts',(-42.8521871210052,-14.6414408657886,
-37.2455902226561));
#24993=CARTESIAN_POINT('Ctrl Pts',(-42.8616851363247,-14.6454405572215,
-37.2568023573302));
#24994=CARTESIAN_POINT('Ctrl Pts',(-42.8707071510317,-14.6492945993135,
-37.2684795517426));
#24995=CARTESIAN_POINT('Ctrl Pts',(-42.8790997295204,-14.6530074411931,
-37.2806776882817));
#24996=CARTESIAN_POINT('Ctrl Pts',(-42.8869655548277,-14.6564872496522,
-37.2921102189659));
#24997=CARTESIAN_POINT('Ctrl Pts',(-42.8942780129941,-14.6598432010016,
-37.3040012433705));
#24998=CARTESIAN_POINT('Ctrl Pts',(-42.9008873385451,-14.6631120254244,
-37.3163705916822));
#24999=CARTESIAN_POINT('Ctrl Pts',(-42.9013299473147,-14.663330929811,-37.317198933696));
#25000=CARTESIAN_POINT('Ctrl Pts',(-42.9017693952537,-14.6635494557761,
-37.3180294074842));
#25001=CARTESIAN_POINT('Ctrl Pts',(-42.9022056342624,-14.6637676196428,
-37.3188620128984));
#25002=CARTESIAN_POINT('Ctrl Pts',(-42.9080335625763,-14.6666821764586,
-37.3299851920969));
#25003=CARTESIAN_POINT('Ctrl Pts',(-42.9132544517344,-14.6694736866497,
-37.3415545631474));
#25004=CARTESIAN_POINT('Ctrl Pts',(-42.9175148584672,-14.6719975663698,
-37.3534879002389));
#25005=CARTESIAN_POINT('Ctrl Pts',(-42.921639999208,-14.6744413140473,-37.3650423592606));
#25006=CARTESIAN_POINT('Ctrl Pts',(-42.9248639641694,-14.6766346712663,
-37.3769386888275));
#25007=CARTESIAN_POINT('Ctrl Pts',(-42.926860530905,-14.6784666962725,-37.3890588177022));
#25008=CARTESIAN_POINT('Ctrl Pts',(-42.9287803512802,-14.6802282997652,
-37.4007130589293));
#25009=CARTESIAN_POINT('Ctrl Pts',(-42.9295645080495,-14.6816565741043,
-37.4125744533077));
#25010=CARTESIAN_POINT('Ctrl Pts',(-42.9289290029343,-14.6826626743678,
-37.4244909451429));
#25011=CARTESIAN_POINT('Ctrl Pts',(-42.9287732308293,-14.6829092850591,
-37.4274118610765));
#25012=CARTESIAN_POINT('Ctrl Pts',(-42.9285322257575,-14.6831305465446,
-37.4303358517388));
#25013=CARTESIAN_POINT('Ctrl Pts',(-42.9282019541629,-14.6833251552392,
-37.4332602126666));
#25014=CARTESIAN_POINT('Ctrl Pts',(-42.9271345709019,-14.6839540984074,
-37.4427112643312));
#25015=CARTESIAN_POINT('Ctrl Pts',(-42.925040039123,-14.6841943737355,-37.4519923607426));
#25016=CARTESIAN_POINT('Ctrl Pts',(-42.9220297208895,-14.6841331258666,
-37.4609600273967));
#25017=CARTESIAN_POINT('Ctrl Pts',(-42.9189684247695,-14.6840708408026,
-37.4700795559664));
#25018=CARTESIAN_POINT('Ctrl Pts',(-42.9149605958391,-14.6836965195603,
-37.4788739643186));
#25019=CARTESIAN_POINT('Ctrl Pts',(-42.9101526120369,-14.6830632794738,
-37.4872169821896));
#25020=CARTESIAN_POINT('Ctrl Pts',(-42.9052560717732,-14.6824183759742,
-37.495713666997));
#25021=CARTESIAN_POINT('Ctrl Pts',(-42.8995304118283,-14.6815043446903,
-37.5037415250777));
#25022=CARTESIAN_POINT('Ctrl Pts',(-42.8931501145775,-14.6803438374132,
-37.5112053503256));
#25023=CARTESIAN_POINT('Ctrl Pts',(-42.8865120039902,-14.67913643667,-37.5189707718181));
#25024=CARTESIAN_POINT('Ctrl Pts',(-42.8791661545134,-14.6776614503338,
-37.5261253320786));
#25025=CARTESIAN_POINT('Ctrl Pts',(-42.871317367589,-14.675919147448,-37.5326108693554));
#25026=CARTESIAN_POINT('Ctrl Pts',(-42.8705136526921,-14.6757407358287,
-37.533274987642));
#25027=CARTESIAN_POINT('Ctrl Pts',(-42.8697046643841,-14.6755595065434,
-37.5339321330287));
#25028=CARTESIAN_POINT('Ctrl Pts',(-42.8688906217797,-14.6753754510085,
-37.5345822715346));
#25029=CARTESIAN_POINT('Origin',(0.0835265683620477,-14.4544045823054,0.0824317919394229));
#25030=CARTESIAN_POINT('Origin',(15.4714058027788,-14.4544045823054,5.15659338881741));
#25031=CARTESIAN_POINT('Origin',(29.1374429791686,-14.7669045823054,-38.2827290469501));
#25032=CARTESIAN_POINT('Origin',(29.1374429791686,-11.3294045823054,-38.2827290469501));
#25033=CARTESIAN_POINT('Origin',(0.0835265683620477,-12.8919045823054,0.0824317919394229));
#25034=CARTESIAN_POINT('Ctrl Pts',(34.7488729746945,-13.2044045823054,-34.1940362076806));
#25035=CARTESIAN_POINT('Ctrl Pts',(34.7490067374541,-13.2044045823054,-34.1691350833616));
#25036=CARTESIAN_POINT('Ctrl Pts',(34.749145716179,-13.2030022087213,-34.1445008166353));
#25037=CARTESIAN_POINT('Ctrl Pts',(34.7492919647972,-13.2001447338014,-34.1200426226309));
#25038=CARTESIAN_POINT('Ctrl Pts',(34.7494355478613,-13.1973393397408,-34.0960302081331));
#25039=CARTESIAN_POINT('Ctrl Pts',(34.749586164608,-13.1931314656534,-34.0721874632317));
#25040=CARTESIAN_POINT('Ctrl Pts',(34.7497462547033,-13.187422036285,-34.0484389068724));
#25041=CARTESIAN_POINT('Ctrl Pts',(34.7497860634588,-13.1860023027459,-34.042533479238));
#25042=CARTESIAN_POINT('Ctrl Pts',(34.7498264593483,-13.1844894768732,-34.0366339287836));
#25043=CARTESIAN_POINT('Ctrl Pts',(34.7498674817982,-13.1828815404475,-34.0307392028842));
#25044=CARTESIAN_POINT('Ctrl Pts',(34.7500209276666,-13.1768669995856,-34.0086897802678));
#25045=CARTESIAN_POINT('Ctrl Pts',(34.7501794108001,-13.1696750914266,-33.9872331665337));
#25046=CARTESIAN_POINT('Ctrl Pts',(34.7503432418475,-13.1611455958502,-33.9663916514025));
#25047=CARTESIAN_POINT('Ctrl Pts',(34.7505070728949,-13.1526161002738,-33.9455501362714));
#25048=CARTESIAN_POINT('Ctrl Pts',(34.7506762764637,-13.1427495299604,-33.9253233735306));
#25049=CARTESIAN_POINT('Ctrl Pts',(34.7508505176857,-13.1313389816383,-33.9057667392102));
#25050=CARTESIAN_POINT('Ctrl Pts',(34.7509093060885,-13.1274891009823,-33.8991683965153));
#25051=CARTESIAN_POINT('Ctrl Pts',(34.7509669071891,-13.1234784566375,-33.8926739099407));
#25052=CARTESIAN_POINT('Ctrl Pts',(34.7510237261945,-13.1192883941035,-33.8862654556767));
#25053=CARTESIAN_POINT('Ctrl Pts',(34.7511184667809,-13.1123018412986,-33.8755799339813));
#25054=CARTESIAN_POINT('Ctrl Pts',(34.7512095940135,-13.1049166125579,-33.8652988342736));
#25055=CARTESIAN_POINT('Ctrl Pts',(34.7512983550753,-13.0970443878841,-33.8553996398422));
#25056=CARTESIAN_POINT('Ctrl Pts',(34.7513313938886,-13.0941141732644,-33.8517149426379));
#25057=CARTESIAN_POINT('Ctrl Pts',(34.7513641008242,-13.0911162306688,-33.848083590736));
#25058=CARTESIAN_POINT('Ctrl Pts',(34.7513965235091,-13.088045086031,-33.8445060658395));
#25059=CARTESIAN_POINT('Ctrl Pts',(34.751482407832,-13.0799099430592,-33.8350295741887));
#25060=CARTESIAN_POINT('Ctrl Pts',(34.7515659307597,-13.0712950250751,-33.8259697968496));
#25061=CARTESIAN_POINT('Ctrl Pts',(34.7516435388463,-13.0621639241565,-33.81741373038));
#25062=CARTESIAN_POINT('Ctrl Pts',(34.7517211469329,-13.053032823238,-33.8088576639104));
#25063=CARTESIAN_POINT('Ctrl Pts',(34.7517917066434,-13.0433849467636,-33.8008061504376));
#25064=CARTESIAN_POINT('Ctrl Pts',(34.7518655550335,-13.0331862397833,-33.7933487163968));
#25065=CARTESIAN_POINT('Ctrl Pts',(34.7519013947382,-13.0282366579926,-33.7897295144916));
#25066=CARTESIAN_POINT('Ctrl Pts',(34.7519360091844,-13.0231465710756,-33.7862448865609));
#25067=CARTESIAN_POINT('Ctrl Pts',(34.7519691779118,-13.0179182754031,-33.7829138711544));
#25068=CARTESIAN_POINT('Ctrl Pts',(34.7520437167405,-13.0061689239916,-33.7754282060314));
#25069=CARTESIAN_POINT('Ctrl Pts',(34.7521095322082,-12.9939049176378,-33.7688513062993));
#25070=CARTESIAN_POINT('Ctrl Pts',(34.7521646053494,-12.9812267133693,-33.7633720134592));
#25071=CARTESIAN_POINT('Ctrl Pts',(34.7522184025857,-12.9688422309163,-33.7580196619277));
#25072=CARTESIAN_POINT('Ctrl Pts',(34.7522619420059,-12.9560629035372,-33.7537150431855));
#25073=CARTESIAN_POINT('Ctrl Pts',(34.7522936929901,-12.943000609226,-33.7505884810027));
#25074=CARTESIAN_POINT('Ctrl Pts',(34.7523245873487,-12.9302907290149,-33.7475462718877));
#25075=CARTESIAN_POINT('Ctrl Pts',(34.7523443148449,-12.9173133257173,-33.7456196262415));
#25076=CARTESIAN_POINT('Ctrl Pts',(34.7523518990928,-12.9041833323999,-33.7448804669025));
#25077=CARTESIAN_POINT('Ctrl Pts',(34.7523542554978,-12.9001038795416,-33.7446508121261));
#25078=CARTESIAN_POINT('Ctrl Pts',(34.7523554432478,-12.8960097626116,-33.7445354190578));
#25079=CARTESIAN_POINT('Ctrl Pts',(34.7523554432478,-12.8919045823054,-33.7445354190578));
#25080=CARTESIAN_POINT('Origin',(21.1549759309662,-13.5169045823054,7.03075374829756));
#25081=CARTESIAN_POINT('Origin',(34.7488729746945,-13.5169045823054,-34.1940362076806));
#25082=CARTESIAN_POINT('Ctrl Pts',(37.2673094055704,-14.9232028613467,-42.8293153229833));
#25083=CARTESIAN_POINT('Ctrl Pts',(37.3552899674095,-14.6181128259927,-43.0961247721324));
#25084=CARTESIAN_POINT('Ctrl Pts',(37.7096412180108,-14.7022319922259,-42.8977137135733));
#25085=CARTESIAN_POINT('Ctrl Pts',(37.1076947869938,-14.453862129984,-42.345268761239));
#25086=CARTESIAN_POINT('Ctrl Pts',(37.1955707280038,-14.1470746072355,-42.6117609377653));
#25087=CARTESIAN_POINT('Ctrl Pts',(37.550607296294,-14.2328912595893,-42.4131587905921));
#25088=CARTESIAN_POINT('Ctrl Pts',(36.9479116082779,-13.9850662226643,-41.8607110247875));
#25089=CARTESIAN_POINT('Ctrl Pts',(37.0359221508734,-13.6772499732423,-42.1276113934436));
#25090=CARTESIAN_POINT('Ctrl Pts',(37.3914171317387,-13.7640953522116,-41.9280765487537));
#25091=CARTESIAN_POINT('Ctrl Pts',(36.7879602992159,-13.5169045823054,-41.3756434170181));
#25092=CARTESIAN_POINT('Ctrl Pts',(36.8763881414603,-13.2088427643879,-41.6438092866772));
#25093=CARTESIAN_POINT('Ctrl Pts',(37.2320718162657,-13.2959337131846,-41.4424668154812));
#25094=CARTESIAN_POINT('Ctrl Pts',(37.7005406318363,-14.6753754510085,-42.8699853982021));
#25095=CARTESIAN_POINT('Ctrl Pts',(37.6942941487563,-14.6771438430879,-42.8778066598394));
#25096=CARTESIAN_POINT('Ctrl Pts',(37.6873971139536,-14.6786525232815,-42.8851614290357));
#25097=CARTESIAN_POINT('Ctrl Pts',(37.6798997497709,-14.6799030932779,-42.8918545698488));
#25098=CARTESIAN_POINT('Ctrl Pts',(37.6726072486374,-14.681119491854,-42.898364822756));
#25099=CARTESIAN_POINT('Ctrl Pts',(37.6647469214214,-14.6820924420367,-42.9042483364246));
#25100=CARTESIAN_POINT('Ctrl Pts',(37.6564075056867,-14.6828029998435,-42.9093313166295));
#25101=CARTESIAN_POINT('Ctrl Pts',(37.648225521828,-14.6835001437071,-42.914318340099));
#25102=CARTESIAN_POINT('Ctrl Pts',(37.6395829273532,-14.6839452832804,-42.9185340273081));
#25103=CARTESIAN_POINT('Ctrl Pts',(37.6305998593746,-14.6840907481788,-42.921831148677));
#25104=CARTESIAN_POINT('Ctrl Pts',(37.6217179108511,-14.6842345756264,-42.9250911554302));
#25105=CARTESIAN_POINT('Ctrl Pts',(37.6125039938892,-14.6840857258449,-42.9274525885272));
#25106=CARTESIAN_POINT('Ctrl Pts',(37.6030993276363,-14.6835622048232,-42.9287997028454));
#25107=CARTESIAN_POINT('Ctrl Pts',(37.6018091775119,-14.6834903872071,-42.9289845025669));
#25108=CARTESIAN_POINT('Ctrl Pts',(37.6005154638893,-14.6834114599928,-42.9291502622653));
#25109=CARTESIAN_POINT('Ctrl Pts',(37.5992185729682,-14.6833251552392,-42.9292967305854));
#25110=CARTESIAN_POINT('Ctrl Pts',(37.5871874867119,-14.682524517408,-42.9306554978992));
#25111=CARTESIAN_POINT('Ctrl Pts',(37.5751667988684,-14.6812727698323,-42.9305019908788));
#25112=CARTESIAN_POINT('Ctrl Pts',(37.5633248420647,-14.679660389819,-42.9291239695466));
#25113=CARTESIAN_POINT('Ctrl Pts',(37.5511660377452,-14.6780048684052,-42.9277090773963));
#25114=CARTESIAN_POINT('Ctrl Pts',(37.5391953985779,-14.6759682812647,-42.9250042042342));
#25115=CARTESIAN_POINT('Ctrl Pts',(37.5275408602363,-14.6736566051529,-42.921330936022));
#25116=CARTESIAN_POINT('Ctrl Pts',(37.5153677286545,-14.6712420661416,-42.9174942180009));
#25117=CARTESIAN_POINT('Ctrl Pts',(37.5035388927731,-14.6685267231679,-42.9126018607288));
#25118=CARTESIAN_POINT('Ctrl Pts',(37.4921479858276,-14.6656525103353,-42.9070169658405));
#25119=CARTESIAN_POINT('Ctrl Pts',(37.4896849080212,-14.665031013744,-42.9058093332335));
#25120=CARTESIAN_POINT('Ctrl Pts',(37.4872421403176,-14.6644021844318,-42.9045692821918));
#25121=CARTESIAN_POINT('Ctrl Pts',(37.4848203732001,-14.663767619643,-42.9033004106846));
#25122=CARTESIAN_POINT('Ctrl Pts',(37.4722830144273,-14.6604825116887,-42.8967315307926));
#25123=CARTESIAN_POINT('Ctrl Pts',(37.4602321609586,-14.6571124630586,-42.8894367548376));
#25124=CARTESIAN_POINT('Ctrl Pts',(37.4486497152673,-14.6536176840784,-42.8815709768372));
#25125=CARTESIAN_POINT('Ctrl Pts',(37.4365571014837,-14.6499689717431,-42.8733587375569));
#25126=CARTESIAN_POINT('Ctrl Pts',(37.4249739677492,-14.6461842219902,-42.8645245242179));
#25127=CARTESIAN_POINT('Ctrl Pts',(37.4138479847458,-14.6422568272874,-42.8552175604044));
#25128=CARTESIAN_POINT('Ctrl Pts',(37.4019517120116,-14.6380575256611,-42.8452662437594));
#25129=CARTESIAN_POINT('Ctrl Pts',(37.3905769669797,-14.6336952044168,-42.8347747585113));
#25130=CARTESIAN_POINT('Ctrl Pts',(37.3796421032092,-14.6292054571928,-42.8238889904825));
#25131=CARTESIAN_POINT('Ctrl Pts',(37.367941220124,-14.6244011899927,-42.8122406424399));
#25132=CARTESIAN_POINT('Ctrl Pts',(37.3567428099825,-14.6194513461054,-42.8001409114864));
#25133=CARTESIAN_POINT('Ctrl Pts',(37.3459461922268,-14.6144447802764,-42.7877248805979));
#25134=CARTESIAN_POINT('Ctrl Pts',(37.3351495744711,-14.6094382144474,-42.7753088497095));
#25135=CARTESIAN_POINT('Ctrl Pts',(37.3247539006079,-14.6043757482481,-42.7625760014678));
#25136=CARTESIAN_POINT('Ctrl Pts',(37.314673576856,-14.5993802185558,-42.7496235025004));
#25137=CARTESIAN_POINT('Ctrl Pts',(37.2996591606931,-14.591939489111,-42.7303310457666));
#25138=CARTESIAN_POINT('Ctrl Pts',(37.2854163404317,-14.5844764296232,-42.7104876092804));
#25139=CARTESIAN_POINT('Ctrl Pts',(37.271869192699,-14.5769485180956,-42.6902126068496));
#25140=CARTESIAN_POINT('Ctrl Pts',(37.2575210202359,-14.5689754912257,-42.6687387706364));
#25141=CARTESIAN_POINT('Ctrl Pts',(37.2439518403639,-14.5609303686272,-42.6467806455568));
#25142=CARTESIAN_POINT('Ctrl Pts',(37.231074974359,-14.5528049305378,-42.6244379172628));
#25143=CARTESIAN_POINT('Ctrl Pts',(37.216955372675,-14.5438953131443,-42.5999389107556));
#25144=CARTESIAN_POINT('Ctrl Pts',(37.2036667293897,-14.5348900830946,-42.5749770310613));
#25145=CARTESIAN_POINT('Ctrl Pts',(37.1911225229489,-14.5258150805519,-42.5496389875043));
#25146=CARTESIAN_POINT('Ctrl Pts',(37.1780215140351,-14.5163372638589,-42.5231762585891));
#25147=CARTESIAN_POINT('Ctrl Pts',(37.1657318069736,-14.5067848826414,-42.4963019660966));
#25148=CARTESIAN_POINT('Ctrl Pts',(37.1542009804941,-14.4972049637149,-42.4690826148663));
#25149=CARTESIAN_POINT('Ctrl Pts',(37.1421820564311,-14.4872195287323,-42.4407110739313));
#25150=CARTESIAN_POINT('Ctrl Pts',(37.1309877266823,-14.4772057790309,-42.4119630555272));
#25151=CARTESIAN_POINT('Ctrl Pts',(37.1206126001907,-14.4672106594482,-42.3829021690193));
#25152=CARTESIAN_POINT('Ctrl Pts',(37.1161774871905,-14.4629379901138,-42.3704793503043));
#25153=CARTESIAN_POINT('Ctrl Pts',(37.1118927098178,-14.4586685042085,-42.3579993627814));
#25154=CARTESIAN_POINT('Ctrl Pts',(37.1077603688698,-14.4544045238129,-42.3454676445359));
#25155=CARTESIAN_POINT('Origin',(0.0835265683620477,-14.4544045823054,0.0824317919394229));
#25156=CARTESIAN_POINT('Origin',(37.8461247099825,-14.4544045823054,-43.0362183703681));
#25157=CARTESIAN_POINT('Ctrl Pts',(48.833526568362,-14.7669045823054,29.5557152835192));
#25158=CARTESIAN_POINT('Ctrl Pts',(48.521026568362,-14.7669045823054,29.5557152835192));
#25159=CARTESIAN_POINT('Ctrl Pts',(48.521026568362,-14.4544045823054,29.5557152835192));
#25160=CARTESIAN_POINT('Ctrl Pts',(48.8335265666929,-14.7669045823054,29.7413197449171));
#25161=CARTESIAN_POINT('Ctrl Pts',(48.5569389176245,-14.7669045823054,29.7119954162173));
#25162=CARTESIAN_POINT('Ctrl Pts',(48.521026568362,-14.4924853132395,29.7214315040358));
#25163=CARTESIAN_POINT('Ctrl Pts',(48.8166857802236,-14.7669045823054,29.9249596309445));
#25164=CARTESIAN_POINT('Ctrl Pts',(48.5753407341527,-14.7669045823059,29.8840840848071));
#25165=CARTESIAN_POINT('Ctrl Pts',(48.5126061688921,-14.5302363915369,29.8851398847485));
#25166=CARTESIAN_POINT('Ctrl Pts',(48.7408780450792,-14.7669045823054,30.287020683478));
#25167=CARTESIAN_POINT('Ctrl Pts',(48.5640170046697,-14.7669045823049,30.2252857066681));
#25168=CARTESIAN_POINT('Ctrl Pts',(48.4747023121212,-14.6047976733282,30.2074413642911));
#25169=CARTESIAN_POINT('Ctrl Pts',(48.6828517369698,-14.7669045823054,30.4694825866923));
#25170=CARTESIAN_POINT('Ctrl Pts',(48.5393566233762,-14.7669045823071,30.4014929051335));
#25171=CARTESIAN_POINT('Ctrl Pts',(48.4458475996025,-14.6423413865141,30.3691656155262));
#25172=CARTESIAN_POINT('Ctrl Pts',(48.582477269951,-14.7669045823054,30.6288487842779));
#25173=CARTESIAN_POINT('Ctrl Pts',(48.472949645285,-14.7669045823054,30.5598642712766));
#25174=CARTESIAN_POINT('Ctrl Pts',(48.3955019191565,-14.6753754514262,30.5110848543364));
#25175=CARTESIAN_POINT('Origin',(48.582477269951,-14.4544045823054,30.6288487842779));
#25176=CARTESIAN_POINT('Ctrl Pts',(48.5210408433891,-6.00666333723546,0.0824317919201338));
#25177=CARTESIAN_POINT('Ctrl Pts',(48.5210403778953,-5.9853111687807,0.0824317919206602));
#25178=CARTESIAN_POINT('Ctrl Pts',(48.5206820692032,-5.96223275463527,0.0824317919312382));
#25179=CARTESIAN_POINT('Ctrl Pts',(48.5165774172042,-5.92795641804992,0.0824317919333195));
#25180=CARTESIAN_POINT('Ctrl Pts',(48.521026568362,-5.90583775506839,0.0824317919337002));
#25181=CARTESIAN_POINT('Ctrl Pts',(48.521026568362,-5.88746284406389,0.082431791939678));
#25182=CARTESIAN_POINT('Ctrl Pts',(48.5210407270156,-6.00132529512183,0.433477096794441));
#25183=CARTESIAN_POINT('Ctrl Pts',(48.5209806868545,-5.98270666392103,0.355621276196246));
#25184=CARTESIAN_POINT('Ctrl Pts',(48.520716368315,-5.96240686080378,0.33843523650393));
#25185=CARTESIAN_POINT('Ctrl Pts',(48.5165547847583,-5.92787973562316,0.360237634060305));
#25186=CARTESIAN_POINT('Ctrl Pts',(48.5210265683621,-5.90583775506839,0.39922607131656));
#25187=CARTESIAN_POINT('Ctrl Pts',(48.521026568362,-5.88746284406389,0.433719204637548));
#25188=CARTESIAN_POINT('Ctrl Pts',(48.5195832988733,-5.99973567328077,0.784574339427845));
#25189=CARTESIAN_POINT('Ctrl Pts',(48.5197866644975,-5.98152768121122,0.651206501674453));
#25190=CARTESIAN_POINT('Ctrl Pts',(48.5193523631325,-5.96239709811727,0.625439688561988));
#25191=CARTESIAN_POINT('Ctrl Pts',(48.5144416808493,-5.92723732580307,0.666464865111502));
#25192=CARTESIAN_POINT('Ctrl Pts',(48.5179089072263,-5.90562906540035,0.733256854779834));
#25193=CARTESIAN_POINT('Ctrl Pts',(48.5172052126372,-5.88746284406389,0.785006622606558));
#25194=CARTESIAN_POINT('Ctrl Pts',(48.5098524785301,-5.9982057973698,1.48689990256317));
#25195=CARTESIAN_POINT('Ctrl Pts',(48.5114206543233,-5.97907559060222,1.29386039347741));
#25196=CARTESIAN_POINT('Ctrl Pts',(48.5102621676405,-5.9609921479881,1.26166887611461));
#25197=CARTESIAN_POINT('Ctrl Pts',(48.5031898260137,-5.9251130175414,1.32614678057686));
#25198=CARTESIAN_POINT('Ctrl Pts',(48.5037480059615,-5.9049506781467,1.42281620240611));
#25199=CARTESIAN_POINT('Ctrl Pts',(48.5019179682626,-5.88746284406389,1.48749857171671));
#25200=CARTESIAN_POINT('Ctrl Pts',(48.5015790863291,-5.99826554329988,1.83812822306509));
#25201=CARTESIAN_POINT('Ctrl Pts',(48.5041223947854,-5.97774718230277,1.64093757425052));
#25202=CARTESIAN_POINT('Ctrl Pts',(48.5024096539615,-5.95954166014521,1.6109000900691));
#25203=CARTESIAN_POINT('Ctrl Pts',(48.4939878358359,-5.9236034688997,1.67960165287408));
#25204=CARTESIAN_POINT('Ctrl Pts',(48.4927046623486,-5.90448098056108,1.77834069986374));
#25205=CARTESIAN_POINT('Ctrl Pts',(48.4904520792406,-5.88746284406389,1.83870311340082));
#25206=CARTESIAN_POINT('Ctrl Pts',(48.4743149973473,-5.99418693015721,2.54074314428776));
#25207=CARTESIAN_POINT('Ctrl Pts',(48.4757865146801,-5.97194742955365,2.39327412296866));
#25208=CARTESIAN_POINT('Ctrl Pts',(48.4732866422927,-5.9541339311854,2.37176704438306));
#25209=CARTESIAN_POINT('Ctrl Pts',(48.4648102886654,-5.91998502842413,2.42404521972768));
#25210=CARTESIAN_POINT('Ctrl Pts',(48.4621240605451,-5.90343694889074,2.49783047365958));
#25211=CARTESIAN_POINT('Ctrl Pts',(48.4598703086855,-5.88746284406389,2.54094611738039));
#25212=CARTESIAN_POINT('Ctrl Pts',(48.4566988310663,-5.99381953117216,2.89171006783013));
#25213=CARTESIAN_POINT('Ctrl Pts',(48.457044461769,-5.97081802552582,2.7688356338994));
#25214=CARTESIAN_POINT('Ctrl Pts',(48.4539681826447,-5.95257589046842,2.75380781345132));
#25215=CARTESIAN_POINT('Ctrl Pts',(48.4456390893095,-5.91860436677926,2.80028584056467));
#25216=CARTESIAN_POINT('Ctrl Pts',(48.4425870086017,-5.90286261480602,2.86179168812718));
#25217=CARTESIAN_POINT('Ctrl Pts',(48.4407544264066,-5.88746284406389,2.89198459022076));
#25218=CARTESIAN_POINT('Ctrl Pts',(48.4142685323911,-5.99717808806687,3.5932676328871));
#25219=CARTESIAN_POINT('Ctrl Pts',(48.4107714342326,-5.97321241327166,3.5256134946276));
#25220=CARTESIAN_POINT('Ctrl Pts',(48.4062756536138,-5.95314193699471,3.52141678729507));
#25221=CARTESIAN_POINT('Ctrl Pts',(48.3983980635879,-5.91737158402251,3.55118314871125));
#25222=CARTESIAN_POINT('Ctrl Pts',(48.3955718611241,-5.90176568155595,3.58514621746019));
#25223=CARTESIAN_POINT('Ctrl Pts',(48.3948635884079,-5.8874628440639,3.59381163136426));
#25224=CARTESIAN_POINT('Ctrl Pts',(48.3894543999969,-6.00090404394666,3.94385827440172));
#25225=CARTESIAN_POINT('Ctrl Pts',(48.3832404596072,-5.97673620504532,3.90682984442505));
#25226=CARTESIAN_POINT('Ctrl Pts',(48.3779018427349,-5.95526602423799,3.90698296769036));
#25227=CARTESIAN_POINT('Ctrl Pts',(48.37032875395,-5.91751946291063,3.9258357898974));
#25228=CARTESIAN_POINT('Ctrl Pts',(48.3680942820372,-5.90124308239061,3.94453548883914));
#25229=CARTESIAN_POINT('Ctrl Pts',(48.3680886315664,-5.8874628440639,3.94460021021535));
#25230=CARTESIAN_POINT('Ctrl Pts',(48.3614264232796,-6.007051447105,4.29441317095755));
#25231=CARTESIAN_POINT('Ctrl Pts',(48.3514946761257,-5.98314272027373,4.29430779651755));
#25232=CARTESIAN_POINT('Ctrl Pts',(48.3455075205231,-5.9599264156786,4.29450986621202));
#25233=CARTESIAN_POINT('Ctrl Pts',(48.3384990828948,-5.91876732373883,4.29496669282097));
#25234=CARTESIAN_POINT('Ctrl Pts',(48.3374778008691,-5.90082453639418,4.29522144973544));
#25235=CARTESIAN_POINT('Ctrl Pts',(48.3374778008691,-5.88746284406389,4.29522144973544));
#25236=CARTESIAN_POINT('Origin',(48.6500773750269,-5.88723161925852,4.32103607293));
#25237=CARTESIAN_POINT('Origin',(-32.9108164063353,-14.7669045823054,-35.8053910964449));
#25238=CARTESIAN_POINT('Origin',(-32.9108164063353,-12.8919045823054,-35.8053910964449));
#25239=CARTESIAN_POINT('Origin',(7.52116697235096,-12.8919045823054,-22.4729224553552));
#25240=CARTESIAN_POINT('Origin',(-32.9108164063353,-12.8919045823054,-35.8053910964449));
#25241=CARTESIAN_POINT('Origin',(0.0835265683620477,-13.5169045823054,0.0824317919394229));
#25242=CARTESIAN_POINT('Origin',(-41.2766849510695,-13.5169045823054,-36.9187829158523));
#25243=CARTESIAN_POINT('Ctrl Pts',(-42.8282205465608,-14.9232028613467,
-37.1013510452688));
#25244=CARTESIAN_POINT('Ctrl Pts',(-43.0950299957099,-14.6181128259927,
-37.1893316071079));
#25245=CARTESIAN_POINT('Ctrl Pts',(-42.8966189371508,-14.7022319922259,
-37.5436828577092));
#25246=CARTESIAN_POINT('Ctrl Pts',(-42.3441739848189,-14.453862129981,-36.941736426693));
#25247=CARTESIAN_POINT('Ctrl Pts',(-42.6106661613464,-14.1470746072311,
-37.0296123677042));
#25248=CARTESIAN_POINT('Ctrl Pts',(-42.4120640141707,-14.2328912595888,
-37.3846489359903));
#25249=CARTESIAN_POINT('Ctrl Pts',(-41.8596162483688,-13.9850662226602,
-36.7819532479775));
#25250=CARTESIAN_POINT('Ctrl Pts',(-42.1265166170242,-13.6772499732382,
-36.8699637905753));
#25251=CARTESIAN_POINT('Ctrl Pts',(-41.926981772331,-13.7640953522118,-37.2254587714377));
#25252=CARTESIAN_POINT('Ctrl Pts',(-41.3745486405956,-13.5169045823054,
-36.6220019389142));
#25253=CARTESIAN_POINT('Ctrl Pts',(-41.6427145102547,-13.2088427643879,
-36.7104297811587));
#25254=CARTESIAN_POINT('Ctrl Pts',(-41.4413720390587,-13.2959337131846,
-37.0661134559641));
#25255=CARTESIAN_POINT('Origin',(-41.2766849510695,-13.5169045823054,-36.9187829158523));
#25256=CARTESIAN_POINT('Ctrl Pts',(29.326104774044,-11.3294045823054,-38.5318534679819));
#25257=CARTESIAN_POINT('Ctrl Pts',(29.5041756346414,-11.3294045823054,-38.3970004975819));
#25258=CARTESIAN_POINT('Ctrl Pts',(29.4342239561067,-11.3294045823054,-38.184865357424));
#25259=CARTESIAN_POINT('Ctrl Pts',(29.3261048404642,-11.1601003758276,-38.5318534176819));
#25260=CARTESIAN_POINT('Ctrl Pts',(29.5041756838974,-11.2236230318997,-38.3970004597999));
#25261=CARTESIAN_POINT('Ctrl Pts',(29.4342239477177,-11.2447524820091,-38.1848653319834));
#25262=CARTESIAN_POINT('Ctrl Pts',(29.3879020055527,-10.9943058431437,-38.4851778011785));
#25263=CARTESIAN_POINT('Ctrl Pts',(29.5522467105556,-11.120480985332,-38.3601666095093));
#25264=CARTESIAN_POINT('Ctrl Pts',(29.4610377908797,-11.1618552084332,-38.1498951506615));
#25265=CARTESIAN_POINT('Ctrl Pts',(29.5859222979822,-10.7673610427475,-38.3339133713355));
#25266=CARTESIAN_POINT('Ctrl Pts',(29.6910051070021,-11.0035905561212,-38.2530870172994));
#25267=CARTESIAN_POINT('Ctrl Pts',(29.5467078428248,-11.0483828168177,-38.0362328980616));
#25268=CARTESIAN_POINT('Ctrl Pts',(29.7215756454094,-10.7044046130696,-38.2295231964381));
#25269=CARTESIAN_POINT('Ctrl Pts',(29.7830216375393,-10.9913613137645,-38.1816458099468));
#25270=CARTESIAN_POINT('Ctrl Pts',(29.6052696128604,-11.0169045823054,-37.9576620938899));
#25271=CARTESIAN_POINT('Ctrl Pts',(29.8546073333508,-10.7044045823054,-38.1258677820342));
#25272=CARTESIAN_POINT('Ctrl Pts',(29.8546073333508,-11.0169045823054,-38.1258677820342));
#25273=CARTESIAN_POINT('Ctrl Pts',(29.6625358445444,-11.0169045823054,-37.8793626234925));
#25274=CARTESIAN_POINT('Ctrl Pts',(29.6625358445444,-11.0169045823054,-37.8793626234925));
#25275=CARTESIAN_POINT('Ctrl Pts',(29.6486851738549,-11.0169045823054,-37.8983004889245));
#25276=CARTESIAN_POINT('Ctrl Pts',(29.6347995539505,-11.018741507632,-37.9172194534708));
#25277=CARTESIAN_POINT('Ctrl Pts',(29.6210644235878,-11.0223262069025,-37.9358685771032));
#25278=CARTESIAN_POINT('Ctrl Pts',(29.6079659337868,-11.0257447508548,-37.9536532904075));
#25279=CARTESIAN_POINT('Ctrl Pts',(29.5950033242865,-11.0307535195304,-37.9711937956057));
#25280=CARTESIAN_POINT('Ctrl Pts',(29.5823447885438,-11.0373176231359,-37.9882626371803));
#25281=CARTESIAN_POINT('Ctrl Pts',(29.5716026040572,-11.0428879997855,-38.0027474598245));
#25282=CARTESIAN_POINT('Ctrl Pts',(29.5610692588669,-11.0495814926586,-38.0168965067492));
#25283=CARTESIAN_POINT('Ctrl Pts',(29.5508418916121,-11.0574216164539,-38.0305775227158));
#25284=CARTESIAN_POINT('Ctrl Pts',(29.5487244956887,-11.059044775743,-38.0334099356637));
#25285=CARTESIAN_POINT('Ctrl Pts',(29.5466202962154,-11.0607171987456,-38.036222182028));
#25286=CARTESIAN_POINT('Ctrl Pts',(29.5445302949047,-11.0624392724585,-38.0390129068931));
#25287=CARTESIAN_POINT('Ctrl Pts',(29.5350786849189,-11.0702270039863,-38.0516333980223));
#25288=CARTESIAN_POINT('Ctrl Pts',(29.5259128880755,-11.0790298901569,-38.0638160310099));
#25289=CARTESIAN_POINT('Ctrl Pts',(29.5171571849087,-11.0888942095813,-38.07544538592));
#25290=CARTESIAN_POINT('Ctrl Pts',(29.514625005418,-11.0917470047092,-38.0788086353851));
#25291=CARTESIAN_POINT('Ctrl Pts',(29.5121272694726,-11.0946887229266,-38.0821253594875));
#25292=CARTESIAN_POINT('Ctrl Pts',(29.5096673709869,-11.0977208509785,-38.0853921096116));
#25293=CARTESIAN_POINT('Ctrl Pts',(29.5077130397355,-11.1001298051058,-38.0879874654343));
#25294=CARTESIAN_POINT('Ctrl Pts',(29.5057827559271,-11.1025951245287,-38.0905492193572));
#25295=CARTESIAN_POINT('Ctrl Pts',(29.5038785684965,-11.1051169477604,-38.0930746719112));
#25296=CARTESIAN_POINT('Ctrl Pts',(29.4943883336226,-11.1176854031531,-38.1056612153982));
#25297=CARTESIAN_POINT('Ctrl Pts',(29.4855598341066,-11.1317057213307,-38.1173411611829));
#25298=CARTESIAN_POINT('Ctrl Pts',(29.4775886595648,-11.1469740767486,-38.1278665693324));
#25299=CARTESIAN_POINT('Ctrl Pts',(29.4693767293853,-11.1627035866208,-38.1387098793592));
#25300=CARTESIAN_POINT('Ctrl Pts',(29.4620748017894,-11.179757668146,-38.1483277159914));
#25301=CARTESIAN_POINT('Ctrl Pts',(29.4559087086157,-11.1978608317579,-38.1564354879713));
#25302=CARTESIAN_POINT('Ctrl Pts',(29.4495980788777,-11.2163883433315,-38.1647333105184));
#25303=CARTESIAN_POINT('Ctrl Pts',(29.4444773334721,-11.236014539749,-38.1714492216813));
#25304=CARTESIAN_POINT('Ctrl Pts',(29.4407987204571,-11.2563909917773,-38.1762670359295));
#25305=CARTESIAN_POINT('Ctrl Pts',(29.4369636562796,-11.2776340529315,-38.1812897514916));
#25306=CARTESIAN_POINT('Ctrl Pts',(29.4346962366054,-11.299692404456,-38.1842491853732));
#25307=CARTESIAN_POINT('Ctrl Pts',(29.4342900459812,-11.3221161967402,-38.1847791414454));
#25308=CARTESIAN_POINT('Ctrl Pts',(29.434246110956,-11.3245416340106,-38.1848364633824));
#25309=CARTESIAN_POINT('Ctrl Pts',(29.4342239561067,-11.3269712973085,-38.184865357424));
#25310=CARTESIAN_POINT('Ctrl Pts',(29.4342239561067,-11.3294045823054,-38.184865357424));
#25311=CARTESIAN_POINT('Origin',(29.6625358445444,-10.7044045823054,-37.8793626234925));
#25312=CARTESIAN_POINT('Ctrl Pts',(34.4520919977564,-13.5169045823054,-34.2918998972067));
#25313=CARTESIAN_POINT('Ctrl Pts',(34.4520919977564,-13.2044045823054,-34.2918998972067));
#25314=CARTESIAN_POINT('Ctrl Pts',(34.7488729746945,-13.2044045823054,-34.1940362076806));
#25315=CARTESIAN_POINT('Ctrl Pts',(34.4246143593772,-13.5169045582439,-34.2085713368222));
#25316=CARTESIAN_POINT('Ctrl Pts',(34.4350349767327,-13.1861191316365,-34.2401728533213));
#25317=CARTESIAN_POINT('Ctrl Pts',(34.7491730539449,-13.2044045823054,-34.1381738077117));
#25318=CARTESIAN_POINT('Ctrl Pts',(34.3978522728513,-13.5027466839946,-34.1274127557131));
#25319=CARTESIAN_POINT('Ctrl Pts',(34.420802744593,-13.1578432798921,-34.1970122512738));
#25320=CARTESIAN_POINT('Ctrl Pts',(34.7495154373051,-13.1973256316197,-34.0836803810649));
#25321=CARTESIAN_POINT('Ctrl Pts',(34.3459175121228,-13.4449866817215,-33.9699156380316));
#25322=CARTESIAN_POINT('Ctrl Pts',(34.3984170950457,-13.0892356355763,-34.1291256329142));
#25323=CARTESIAN_POINT('Ctrl Pts',(34.7502673139448,-13.1684456335482,-33.9777792652241));
#25324=CARTESIAN_POINT('Ctrl Pts',(34.3222371758063,-13.4031153721669,-33.8981027585021));
#25325=CARTESIAN_POINT('Ctrl Pts',(34.3914218944348,-13.0503322093645,-34.1079120195585));
#25326=CARTESIAN_POINT('Ctrl Pts',(34.7506550934714,-13.147509967376,-33.9294147505826));
#25327=CARTESIAN_POINT('Ctrl Pts',(34.2800267092033,-13.2902331116006,-33.770095490678));
#25328=CARTESIAN_POINT('Ctrl Pts',(34.3847390713609,-12.9767617731721,-34.087645720892));
#25329=CARTESIAN_POINT('Ctrl Pts',(34.7513994248545,-13.0910688568131,-33.8431120353597));
#25330=CARTESIAN_POINT('Ctrl Pts',(34.2628371595374,-13.2224528271011,-33.717966541037));
#25331=CARTESIAN_POINT('Ctrl Pts',(34.3858673504075,-12.9460615526398,-34.091067334764));
#25332=CARTESIAN_POINT('Ctrl Pts',(34.7517320489624,-13.0571787063097,-33.8079153247474));
#25333=CARTESIAN_POINT('Ctrl Pts',(34.2384230621111,-13.065416935761,-33.6439284609247));
#25334=CARTESIAN_POINT('Ctrl Pts',(34.3902784659414,-12.9052920386063,-34.1044444635434));
#25335=CARTESIAN_POINT('Ctrl Pts',(34.7522178573803,-12.9786607574268,-33.7579024304006));
#25336=CARTESIAN_POINT('Ctrl Pts',(34.2319045968862,-12.9802875861309,-33.6241605931184));
#25337=CARTESIAN_POINT('Ctrl Pts',(34.393033636199,-12.8977806170666,-34.1127997802578));
#25338=CARTESIAN_POINT('Ctrl Pts',(34.7523554491597,-12.9360960854271,-33.7445354129988));
#25339=CARTESIAN_POINT('Ctrl Pts',(34.2319046026008,-12.8919045823054,-33.6241606104485));
#25340=CARTESIAN_POINT('Ctrl Pts',(34.3930336345113,-12.8919045823054,-34.112799775138));
#25341=CARTESIAN_POINT('Ctrl Pts',(34.7523554432478,-12.8919045823054,-33.7445354190578));
#25342=CARTESIAN_POINT('Ctrl Pts',(37.7386905645208,-14.6563598281215,-42.7974778141527));
#25343=CARTESIAN_POINT('Ctrl Pts',(37.8152217296418,-14.7669045823078,-42.8493171995473));
#25344=CARTESIAN_POINT('Ctrl Pts',(37.935395944751,-14.7669045823054,-42.9300026606738));
#25345=CARTESIAN_POINT('Ctrl Pts',(37.7175355100096,-14.6732979129446,-42.8591973289493));
#25346=CARTESIAN_POINT('Ctrl Pts',(37.7874533080794,-14.7669045823044,-42.9232591435907));
#25347=CARTESIAN_POINT('Ctrl Pts',(37.8823038919049,-14.7669045823054,-43.0182648484161));
#25348=CARTESIAN_POINT('Ctrl Pts',(37.6775546541054,-14.6836226395046,-42.9057319112783));
#25349=CARTESIAN_POINT('Ctrl Pts',(37.7271961037498,-14.7669045823054,-42.9839489162578));
#25350=CARTESIAN_POINT('Ctrl Pts',(37.7948585081688,-14.7669045823054,-43.0905896374617));
#25351=CARTESIAN_POINT('Ctrl Pts',(37.5997129170687,-14.6837071744148,-42.9316733022326));
#25352=CARTESIAN_POINT('Ctrl Pts',(37.6161850043513,-14.7669045823054,-43.0208827520291));
#25353=CARTESIAN_POINT('Ctrl Pts',(37.6386288705569,-14.7669045823054,-43.1424614647264));
#25354=CARTESIAN_POINT('Ctrl Pts',(37.5689613038834,-14.6805726740705,-42.9316885218425));
#25355=CARTESIAN_POINT('Ctrl Pts',(37.5728052530044,-14.7669045823053,-43.022898282639));
#25356=CARTESIAN_POINT('Ctrl Pts',(37.5790568393347,-14.7669045823054,-43.1489392469548));
#25357=CARTESIAN_POINT('Ctrl Pts',(37.4757303120884,-14.66352762411,-42.9073579283318));
#25358=CARTESIAN_POINT('Ctrl Pts',(37.445202377388,-14.7669045823055,-42.9986732904205));
#25359=CARTESIAN_POINT('Ctrl Pts',(37.4036140787982,-14.7669045823054,-43.1351870004211));
#25360=CARTESIAN_POINT('Ctrl Pts',(37.4132032793102,-14.6424796666972,-42.8599547573657));
#25361=CARTESIAN_POINT('Ctrl Pts',(37.364845501704,-14.7669045823051,-42.9421725988748));
#25362=CARTESIAN_POINT('Ctrl Pts',(37.2925429683339,-14.7669045823054,-43.0833710447635));
#25363=CARTESIAN_POINT('Ctrl Pts',(37.2264916052012,-14.5607785229746,-42.657224059441));
#25364=CARTESIAN_POINT('Ctrl Pts',(37.1424895246967,-14.7669045823062,-42.6940481533457));
#25365=CARTESIAN_POINT('Ctrl Pts',(36.9739954005229,-14.7669045823054,-42.8448791143223));
#25366=CARTESIAN_POINT('Ctrl Pts',(37.1311194555558,-14.4859905466154,-42.4463288741486));
#25367=CARTESIAN_POINT('Ctrl Pts',(37.0866121993381,-14.7669045823059,-42.4219753342952));
#25368=CARTESIAN_POINT('Ctrl Pts',(36.8345069741914,-14.7669045823054,-42.5760612268253));
#25369=CARTESIAN_POINT('Ctrl Pts',(37.0775149489995,-14.4183787521282,-42.2439952620268));
#25370=CARTESIAN_POINT('Ctrl Pts',(37.1178746289163,-14.766904582305,-42.2357920123654));
#25371=CARTESIAN_POINT('Ctrl Pts',(36.7741979390219,-14.7669045823054,-42.3109485117452));
#25372=CARTESIAN_POINT('Origin',(36.8109793750892,-14.4544045823054,-42.4433312829855));
#25373=CARTESIAN_POINT('Origin',(0.0835265683620477,-14.4544045823054,0.0824317919394229));
#25374=CARTESIAN_POINT('Origin',(47.5194292675621,-14.4544045823054,32.2548881068839));
#25375=CARTESIAN_POINT('Ctrl Pts',(39.8249086674878,-6.28105857414855,27.6158484236678));
#25376=CARTESIAN_POINT('Ctrl Pts',(39.9934560522847,-6.09633085020216,27.6714270160236));
#25377=CARTESIAN_POINT('Ctrl Pts',(40.1051877166575,-6.06008770502775,27.4437781582428));
#25378=CARTESIAN_POINT('Ctrl Pts',(41.997582097766,-8.47898077424469,28.3322886760592));
#25379=CARTESIAN_POINT('Ctrl Pts',(42.1761782548842,-8.30110493968489,28.3911808565934));
#25380=CARTESIAN_POINT('Ctrl Pts',(42.2795010816781,-8.25800948639213,28.1578189230589));
#25381=CARTESIAN_POINT('Ctrl Pts',(44.1644194400702,-10.6833293750622,29.0468044752481));
#25382=CARTESIAN_POINT('Ctrl Pts',(44.3429038866861,-10.5025148293853,29.1056598191394));
#25383=CARTESIAN_POINT('Ctrl Pts',(44.4477081038169,-10.4623581523692,28.8702339699961));
#25384=CARTESIAN_POINT('Ctrl Pts',(46.3272934177549,-12.8919045823054,29.7600133527852));
#25385=CARTESIAN_POINT('Ctrl Pts',(46.5008548189629,-12.7034528674627,29.8172453197959));
#25386=CARTESIAN_POINT('Ctrl Pts',(46.611780876039,-12.6709337131846,29.5815526781396));
#25387=CARTESIAN_POINT('Ctrl Pts',(40.153012388794,-6.10843371318468,27.4594837601833));
#25388=CARTESIAN_POINT('Ctrl Pts',(40.1486301258045,-6.10756827058304,27.4643636112223));
#25389=CARTESIAN_POINT('Ctrl Pts',(40.14431636544,-6.10708538385354,27.4693390586013));
#25390=CARTESIAN_POINT('Ctrl Pts',(40.1401031486147,-6.10700426240365,27.4743794740622));
#25391=CARTESIAN_POINT('Ctrl Pts',(40.1337833233766,-6.10688258022881,27.4819400972536));
#25392=CARTESIAN_POINT('Ctrl Pts',(40.127689581349,-6.10766522922463,27.4896462179766));
#25393=CARTESIAN_POINT('Ctrl Pts',(40.1219384863636,-6.1094056136749,27.4974038197989));
#25394=CARTESIAN_POINT('Ctrl Pts',(40.119062938871,-6.11027580590004,27.5012826207101));
#25395=CARTESIAN_POINT('Ctrl Pts',(40.1162731700049,-6.1113852520171,27.5051744892978));
#25396=CARTESIAN_POINT('Ctrl Pts',(40.1135841376133,-6.11273984167805,27.5090689245252));
#25397=CARTESIAN_POINT('Ctrl Pts',(40.1129118795153,-6.11307848909328,27.510042533332));
#25398=CARTESIAN_POINT('Ctrl Pts',(40.1122459177464,-6.11343245632759,27.511016306785));
#25399=CARTESIAN_POINT('Ctrl Pts',(40.1115864861771,-6.11380183251757,27.5119900892948));
#25400=CARTESIAN_POINT('Ctrl Pts',(40.1105973388232,-6.11435589680255,27.5134507630594));
#25401=CARTESIAN_POINT('Ctrl Pts',(40.1096228845693,-6.11494463135663,27.5149114564014));
#25402=CARTESIAN_POINT('Ctrl Pts',(40.1086639111446,-6.115568333847,27.5163716586017));
#25403=CARTESIAN_POINT('Ctrl Pts',(40.1077049377198,-6.11619203633737,27.517831860802));
#25404=CARTESIAN_POINT('Ctrl Pts',(40.1067614452345,-6.11685070666524,27.519291571862));
#25405=CARTESIAN_POINT('Ctrl Pts',(40.1058342180418,-6.11754464002828,27.5207502983356));
#25406=CARTESIAN_POINT('Ctrl Pts',(40.1008056546947,-6.12130799802938,27.5286613028186));
#25407=CARTESIAN_POINT('Ctrl Pts',(40.0963697525875,-6.12597258662923,27.5363115221513));
#25408=CARTESIAN_POINT('Ctrl Pts',(40.0924653997853,-6.13138771967841,27.5436694209767));
#25409=CARTESIAN_POINT('Ctrl Pts',(40.0912502383763,-6.13307308497174,27.5459594380823));
#25410=CARTESIAN_POINT('Ctrl Pts',(40.090086516912,-6.13483149128332,27.5482213190137));
#25411=CARTESIAN_POINT('Ctrl Pts',(40.0889722671577,-6.13665930617706,27.5504545293107));
#25412=CARTESIAN_POINT('Ctrl Pts',(40.0883854708883,-6.13762188656504,27.5516306026875));
#25413=CARTESIAN_POINT('Ctrl Pts',(40.0878124152614,-6.13860357319269,27.5527985817608));
#25414=CARTESIAN_POINT('Ctrl Pts',(40.0872528103463,-6.13960373328463,27.5539582878036));
#25415=CARTESIAN_POINT('Ctrl Pts',(40.0870002128769,-6.14005519091391,27.5544817621404));
#25416=CARTESIAN_POINT('Ctrl Pts',(40.0867503319911,-6.14051040725672,27.555003558958));
#25417=CARTESIAN_POINT('Ctrl Pts',(40.086503247387,-6.14096936706302,27.5555236415609));
#25418=CARTESIAN_POINT('Ctrl Pts',(40.0862713642513,-6.14140009013227,27.5560117269487));
#25419=CARTESIAN_POINT('Ctrl Pts',(40.0860418533618,-6.1418340234271,27.5564983732832));
#25420=CARTESIAN_POINT('Ctrl Pts',(40.0858147608252,-6.14227112540981,27.5569835610311));
#25421=CARTESIAN_POINT('Ctrl Pts',(40.0825312534216,-6.14859113758575,27.563998840292));
#25422=CARTESIAN_POINT('Ctrl Pts',(40.0797513639648,-6.15557322588934,27.5707108135461));
#25423=CARTESIAN_POINT('Ctrl Pts',(40.0774276984569,-6.1630485902823,27.5771166413194));
#25424=CARTESIAN_POINT('Ctrl Pts',(40.075339709593,-6.16976576947768,27.5828727611265));
#25425=CARTESIAN_POINT('Ctrl Pts',(40.0736091318008,-6.17677030338731,27.5883069387177));
#25426=CARTESIAN_POINT('Ctrl Pts',(40.0721954246486,-6.18399336848783,27.5934675539933));
#25427=CARTESIAN_POINT('Ctrl Pts',(40.0715542408364,-6.18726937399525,27.5958081398567));
#25428=CARTESIAN_POINT('Ctrl Pts',(40.070978696512,-6.19059093207267,27.5980923367893));
#25429=CARTESIAN_POINT('Ctrl Pts',(40.07046715491,-6.19395424178566,27.600324154726));
#25430=CARTESIAN_POINT('Ctrl Pts',(40.0698523767083,-6.19799631673864,27.6030063862633));
#25431=CARTESIAN_POINT('Ctrl Pts',(40.0693281053813,-6.20209746439246,27.6056128186841));
#25432=CARTESIAN_POINT('Ctrl Pts',(40.0688877556671,-6.20624978925051,27.6081491750566));
#25433=CARTESIAN_POINT('Ctrl Pts',(40.0685024496673,-6.20988307350131,27.6103684868826));
#25434=CARTESIAN_POINT('Ctrl Pts',(40.0681813835459,-6.21355555791223,27.6125341305234));
#25435=CARTESIAN_POINT('Ctrl Pts',(40.0679199399159,-6.2172623580558,27.6146493155572));
#25436=CARTESIAN_POINT('Ctrl Pts',(40.0671497781398,-6.22818186595188,27.6208802367785));
#25437=CARTESIAN_POINT('Ctrl Pts',(40.0668900862771,-6.23942896207781,27.6266930616364));
#25438=CARTESIAN_POINT('Ctrl Pts',(40.0670349189619,-6.25083884461348,27.6321118626055));
#25439=CARTESIAN_POINT('Ctrl Pts',(40.0670644700791,-6.25316687420515,27.6332174944092));
#25440=CARTESIAN_POINT('Ctrl Pts',(40.0671108919301,-6.25550185226918,27.6343067222454));
#25441=CARTESIAN_POINT('Ctrl Pts',(40.0671733296103,-6.25784263179034,27.6353797440325));
#25442=CARTESIAN_POINT('Ctrl Pts',(40.0675320452674,-6.27129082943959,27.641544446408));
#25443=CARTESIAN_POINT('Ctrl Pts',(40.0683768978808,-6.28489536287217,27.6472113601885));
#25444=CARTESIAN_POINT('Ctrl Pts',(40.0695536495387,-6.29858154433864,27.6524587325793));
#25445=CARTESIAN_POINT('Ctrl Pts',(40.0704275122879,-6.30874498373682,27.6563554623885));
#25446=CARTESIAN_POINT('Ctrl Pts',(40.0715188210737,-6.31897515340961,27.6600258390141));
#25447=CARTESIAN_POINT('Ctrl Pts',(40.0728000600482,-6.32926010589388,27.6634970067625));
#25448=CARTESIAN_POINT('Ctrl Pts',(40.074950602702,-6.34652326245748,27.6693233158672));
#25449=CARTESIAN_POINT('Ctrl Pts',(40.0776339280651,-6.36392973954521,27.6745857947252));
#25450=CARTESIAN_POINT('Ctrl Pts',(40.0807437314268,-6.38139910656903,27.6793726882152));
#25451=CARTESIAN_POINT('Ctrl Pts',(40.0841784757829,-6.400693834502,27.6846597605749));
#25452=CARTESIAN_POINT('Ctrl Pts',(40.0881335071639,-6.42006561697338,27.6893667923115));
#25453=CARTESIAN_POINT('Ctrl Pts',(40.0925060685141,-6.43945161631725,27.6935864739196));
#25454=CARTESIAN_POINT('Ctrl Pts',(40.0971878544237,-6.46020858032532,27.6981045685358));
#25455=CARTESIAN_POINT('Ctrl Pts',(40.1023486755735,-6.48098271074861,27.7020639266992));
#25456=CARTESIAN_POINT('Ctrl Pts',(40.1079031404676,-6.50173650943862,27.705549038395));
#25457=CARTESIAN_POINT('Ctrl Pts',(40.1141796220518,-6.52518806377629,27.7094871746142));
#25458=CARTESIAN_POINT('Ctrl Pts',(40.1209590306374,-6.54861499437352,27.712820039933));
#25459=CARTESIAN_POINT('Ctrl Pts',(40.1281636304217,-6.57199467991746,27.7156308755257));
#25460=CARTESIAN_POINT('Ctrl Pts',(40.1305643122126,-6.57978514532063,27.7165674885266));
#25461=CARTESIAN_POINT('Ctrl Pts',(40.1330125170019,-6.58757049925619,27.7174458345116));
#25462=CARTESIAN_POINT('Ctrl Pts',(40.1355061827836,-6.5953500914164,27.7182681242769));
#25463=CARTESIAN_POINT('Origin',(46.4251571072811,-12.8919045823054,29.4632323758471));
#25464=CARTESIAN_POINT('Ctrl Pts',(-39.6578555996089,-6.28105864379379,
-27.4509848624907));
#25465=CARTESIAN_POINT('Ctrl Pts',(-39.826402984466,-6.09633091980368,-27.5065634548664));
#25466=CARTESIAN_POINT('Ctrl Pts',(-39.9381346488306,-6.060087774673,-27.2789145969897));
#25467=CARTESIAN_POINT('Ctrl Pts',(-41.8305313962535,-8.47898323805638,
-28.1674258951927));
#25468=CARTESIAN_POINT('Ctrl Pts',(-42.0091275727744,-8.30110741938527,
-28.2263180821171));
#25469=CARTESIAN_POINT('Ctrl Pts',(-42.1124503819745,-8.25801195014743,
-27.9929561395079));
#25470=CARTESIAN_POINT('Ctrl Pts',(-43.9973666758772,-10.6833297554487,
-28.8819410142116));
#25471=CARTESIAN_POINT('Ctrl Pts',(-44.1758511208521,-10.5025152076406,
-28.9407963575876));
#25472=CARTESIAN_POINT('Ctrl Pts',(-44.2806553397966,-10.4623585327411,
-28.7053705086298));
#25473=CARTESIAN_POINT('Ctrl Pts',(-46.1602402810308,-12.8919045823054,
-29.5951497689063));
#25474=CARTESIAN_POINT('Ctrl Pts',(-46.3338016822388,-12.7034528674627,
-29.6523817359171));
#25475=CARTESIAN_POINT('Ctrl Pts',(-46.4447277393149,-12.6709337131846,
-29.4166890942607));
#25476=CARTESIAN_POINT('Ctrl Pts',(-39.9859592520697,-6.10843371318464,
-27.2946201763047));
#25477=CARTESIAN_POINT('Ctrl Pts',(-39.9815769890805,-6.10756827058306,
-27.2995000273434));
#25478=CARTESIAN_POINT('Ctrl Pts',(-39.9772632287159,-6.10708538385355,
-27.3044754747224));
#25479=CARTESIAN_POINT('Ctrl Pts',(-39.9730500118906,-6.10700426240366,
-27.3095158901833));
#25480=CARTESIAN_POINT('Ctrl Pts',(-39.9667301866525,-6.10688258022884,
-27.3170765133747));
#25481=CARTESIAN_POINT('Ctrl Pts',(-39.9606364446249,-6.10766522922467,
-27.3247826340977));
#25482=CARTESIAN_POINT('Ctrl Pts',(-39.9548853496395,-6.10940561367495,
-27.3325402359201));
#25483=CARTESIAN_POINT('Ctrl Pts',(-39.9520098021468,-6.11027580590009,
-27.3364190368312));
#25484=CARTESIAN_POINT('Ctrl Pts',(-39.9492200332808,-6.11138525201715,
-27.340310905419));
#25485=CARTESIAN_POINT('Ctrl Pts',(-39.9465310008892,-6.1127398416781,-27.3442053406463));
#25486=CARTESIAN_POINT('Ctrl Pts',(-39.9458587427912,-6.11307848909333,
-27.3451789494531));
#25487=CARTESIAN_POINT('Ctrl Pts',(-39.9451927810223,-6.11343245632765,
-27.3461527229061));
#25488=CARTESIAN_POINT('Ctrl Pts',(-39.944533349453,-6.11380183251763,-27.3471265054159));
#25489=CARTESIAN_POINT('Ctrl Pts',(-39.9435442020991,-6.11435589680261,
-27.3485871791806));
#25490=CARTESIAN_POINT('Ctrl Pts',(-39.9425697478452,-6.11494463135667,
-27.3500478725225));
#25491=CARTESIAN_POINT('Ctrl Pts',(-39.9416107744204,-6.11556833384704,
-27.3515080747228));
#25492=CARTESIAN_POINT('Ctrl Pts',(-39.9406518009957,-6.11619203633741,
-27.3529682769231));
#25493=CARTESIAN_POINT('Ctrl Pts',(-39.9397083085104,-6.11685070666528,
-27.3544279879831));
#25494=CARTESIAN_POINT('Ctrl Pts',(-39.9387810813177,-6.11754464002833,
-27.3558867144568));
#25495=CARTESIAN_POINT('Ctrl Pts',(-39.933752517971,-6.12130799802912,-27.3637977189391));
#25496=CARTESIAN_POINT('Ctrl Pts',(-39.9293166158641,-6.12597258662852,
-27.3714479382713));
#25497=CARTESIAN_POINT('Ctrl Pts',(-39.9254122630621,-6.13138771967716,
-27.3788058370961));
#25498=CARTESIAN_POINT('Ctrl Pts',(-39.9241971016528,-6.13307308497087,
-27.3810958542024));
#25499=CARTESIAN_POINT('Ctrl Pts',(-39.9230333801882,-6.13483149128286,
-27.3833577351343));
#25500=CARTESIAN_POINT('Ctrl Pts',(-39.9219191304336,-6.13665930617706,
-27.3855909454319));
#25501=CARTESIAN_POINT('Ctrl Pts',(-39.9213323341642,-6.13762188656503,
-27.3867670188086));
#25502=CARTESIAN_POINT('Ctrl Pts',(-39.9207592785374,-6.13860357319269,
-27.3879349978819));
#25503=CARTESIAN_POINT('Ctrl Pts',(-39.9201996736223,-6.13960373328462,
-27.3890947039248));
#25504=CARTESIAN_POINT('Ctrl Pts',(-39.9199470761528,-6.1400551909139,-27.3896181782615));
#25505=CARTESIAN_POINT('Ctrl Pts',(-39.919697195267,-6.14051040725671,-27.3901399750791));
#25506=CARTESIAN_POINT('Ctrl Pts',(-39.9194501106629,-6.14096936706301,
-27.3906600576821));
#25507=CARTESIAN_POINT('Ctrl Pts',(-39.9192182275272,-6.14140009013226,
-27.3911481430698));
#25508=CARTESIAN_POINT('Ctrl Pts',(-39.9189887166377,-6.1418340234271,-27.3916347894044));
#25509=CARTESIAN_POINT('Ctrl Pts',(-39.9187616241011,-6.1422711254098,-27.3921199771522));
#25510=CARTESIAN_POINT('Ctrl Pts',(-39.9154781166975,-6.14859113758575,
-27.3991352564131));
#25511=CARTESIAN_POINT('Ctrl Pts',(-39.9126982272407,-6.15557322588935,
-27.4058472296673));
#25512=CARTESIAN_POINT('Ctrl Pts',(-39.9103745617328,-6.16304859028231,
-27.4122530574405));
#25513=CARTESIAN_POINT('Ctrl Pts',(-39.9082865728688,-6.16976576947789,
-27.4180091772478));
#25514=CARTESIAN_POINT('Ctrl Pts',(-39.9065559950766,-6.17677030338776,
-27.4234433548392));
#25515=CARTESIAN_POINT('Ctrl Pts',(-39.9051422879244,-6.18399336848851,
-27.4286039701149));
#25516=CARTESIAN_POINT('Ctrl Pts',(-39.9045011041123,-6.18726937399572,
-27.4309445559781));
#25517=CARTESIAN_POINT('Ctrl Pts',(-39.9039255597879,-6.19059093207291,
-27.4332287529105));
#25518=CARTESIAN_POINT('Ctrl Pts',(-39.9034140181859,-6.19395424178567,
-27.4354605708472));
#25519=CARTESIAN_POINT('Ctrl Pts',(-39.9027992399842,-6.19799631673865,
-27.4381428023844));
#25520=CARTESIAN_POINT('Ctrl Pts',(-39.9022749686572,-6.20209746439248,
-27.4407492348052));
#25521=CARTESIAN_POINT('Ctrl Pts',(-39.901834618943,-6.20624978925053,-27.4432855911778));
#25522=CARTESIAN_POINT('Ctrl Pts',(-39.9014493129432,-6.20988307350132,
-27.4455049030038));
#25523=CARTESIAN_POINT('Ctrl Pts',(-39.9011282468218,-6.21355555791224,
-27.4476705466445));
#25524=CARTESIAN_POINT('Ctrl Pts',(-39.9008668031918,-6.21726235805581,
-27.4497857316783));
#25525=CARTESIAN_POINT('Ctrl Pts',(-39.9000966414157,-6.22818186595271,
-27.4560166529001));
#25526=CARTESIAN_POINT('Ctrl Pts',(-39.899836949553,-6.2394289620795,-27.4618294777584));
#25527=CARTESIAN_POINT('Ctrl Pts',(-39.8999817822378,-6.25083884461606,
-27.4672482787279));
#25528=CARTESIAN_POINT('Ctrl Pts',(-39.900011333355,-6.25316687420688,-27.4683539105311));
#25529=CARTESIAN_POINT('Ctrl Pts',(-39.900057755206,-6.25550185227005,-27.469443138367));
#25530=CARTESIAN_POINT('Ctrl Pts',(-39.9001201928862,-6.25784263179036,
-27.4705161601537));
#25531=CARTESIAN_POINT('Ctrl Pts',(-39.9004789085434,-6.27129082943962,
-27.4766808625291));
#25532=CARTESIAN_POINT('Ctrl Pts',(-39.9013237611568,-6.28489536287222,
-27.4823477763096));
#25533=CARTESIAN_POINT('Ctrl Pts',(-39.9025005128147,-6.29858154433868,
-27.4875951487004));
#25534=CARTESIAN_POINT('Ctrl Pts',(-39.9033743755616,-6.30874498371071,
-27.4914918784995));
#25535=CARTESIAN_POINT('Ctrl Pts',(-39.904465684344,-6.31897515335698,-27.4951622551162));
#25536=CARTESIAN_POINT('Ctrl Pts',(-39.905746923314,-6.32926010581451,-27.4986334228567));
#25537=CARTESIAN_POINT('Ctrl Pts',(-39.9078974659659,-6.3465232623761,-27.5044597319625));
#25538=CARTESIAN_POINT('Ctrl Pts',(-39.910580791327,-6.36392973946194,-27.5097222108217));
#25539=CARTESIAN_POINT('Ctrl Pts',(-39.9136905946869,-6.38139910648396,
-27.5145091043127));
#25540=CARTESIAN_POINT('Ctrl Pts',(-39.917125339041,-6.40069383441468,-27.5197961766734));
#25541=CARTESIAN_POINT('Ctrl Pts',(-39.9210803704199,-6.42006561688391,
-27.5245032084111));
#25542=CARTESIAN_POINT('Ctrl Pts',(-39.9254529317683,-6.43945161622571,
-27.5287228900203));
#25543=CARTESIAN_POINT('Ctrl Pts',(-39.9301347176756,-6.46020858023109,
-27.5332409846376));
#25544=CARTESIAN_POINT('Ctrl Pts',(-39.9352955388234,-6.48098271065176,
-27.537200342802));
#25545=CARTESIAN_POINT('Ctrl Pts',(-39.9408500037156,-6.50173650933919,
-27.5406854544989));
#25546=CARTESIAN_POINT('Ctrl Pts',(-39.9471264852975,-6.52518806367359,
-27.5446235907193));
#25547=CARTESIAN_POINT('Ctrl Pts',(-39.953905893881,-6.54861499426759,-27.5479564560394));
#25548=CARTESIAN_POINT('Ctrl Pts',(-39.9611104936634,-6.57199467980834,
-27.5507672916335));
#25549=CARTESIAN_POINT('Ctrl Pts',(-39.963511175461,-6.57978514523424,-27.5517039046378));
#25550=CARTESIAN_POINT('Ctrl Pts',(-39.9659593802573,-6.58757049919249,
-27.5525822506258));
#25551=CARTESIAN_POINT('Ctrl Pts',(-39.9684530460464,-6.59535009137536,
-27.5534045403938));
#25552=CARTESIAN_POINT('Origin',(-46.258103970557,-12.8919045823054,-29.2983687919682));
#25553=CARTESIAN_POINT('Origin',(0.0835265683620477,-5.88746284406389,0.0824317919394229));
#25554=CARTESIAN_POINT('Origin',(40.3354637847015,-5.88746284406389,27.5841417448109));
#25555=CARTESIAN_POINT('Origin',(-32.9108164063353,-12.8919045823054,-35.8053910964449));
#25556=CARTESIAN_POINT('Origin',(-32.9108164063353,-12.8919045823054,-35.8053910964449));
#25557=CARTESIAN_POINT('Origin',(-41.2766849510695,-13.5169045823054,-36.9187829158523));
#25558=CARTESIAN_POINT('Origin',(-41.2766849510695,-13.5169045823054,-36.9187829158523));
#25559=CARTESIAN_POINT('Origin',(19.8255764196421,-11.0169045823054,-10.0436051386457));
#25560=CARTESIAN_POINT('Origin',(19.8255764196421,-11.3294045823054,-10.0436051386457));
#25561=CARTESIAN_POINT('Origin',(15.4714058027788,-11.3294045823054,5.15659338881741));
#25562=CARTESIAN_POINT('Origin',(20.4191383735183,-11.3294045823054,-9.84787775959334));
#25563=CARTESIAN_POINT('Origin',(0.0835265683620477,-10.7044045823054,0.0824317919394229));
#25564=CARTESIAN_POINT('Origin',(34.0350086811056,-10.7044045823054,-34.02493526194));
#25565=CARTESIAN_POINT('Origin',(29.4071186530799,-14.4544045823054,-19.9904171446541));
#25566=CARTESIAN_POINT('Origin',(20.56141397709,-14.4544045823054,6.83502636924522));
#25567=CARTESIAN_POINT('Ctrl Pts',(46.5427518284381,-14.426701821061,32.1322496158952));
#25568=CARTESIAN_POINT('Ctrl Pts',(46.5548124230274,-14.7669045823053,32.1041265430089));
#25569=CARTESIAN_POINT('Ctrl Pts',(46.4212196497479,-14.7669045823054,32.418869262555));
#25570=CARTESIAN_POINT('Ctrl Pts',(46.6932699125038,-14.479760966508,32.1906930433489));
#25571=CARTESIAN_POINT('Ctrl Pts',(46.6642075899464,-14.7669045823056,32.2097370359491));
#25572=CARTESIAN_POINT('Ctrl Pts',(46.6172868947414,-14.7669045823054,32.5015126714166));
#25573=CARTESIAN_POINT('Ctrl Pts',(46.8607640732745,-14.5360769750828,32.2283316967679));
#25574=CARTESIAN_POINT('Ctrl Pts',(46.8417224039433,-14.766904582305,32.2976409195446));
#25575=CARTESIAN_POINT('Ctrl Pts',(46.8413031346229,-14.7669045823054,32.5405339499658));
#25576=CARTESIAN_POINT('Ctrl Pts',(47.1709605059096,-14.6333609973517,32.229273177524));
#25577=CARTESIAN_POINT('Ctrl Pts',(47.1941665884612,-14.7669045823058,32.3240183566974));
#25578=CARTESIAN_POINT('Ctrl Pts',(47.2703848519362,-14.7669045823054,32.4794795677955));
#25579=CARTESIAN_POINT('Ctrl Pts',(47.3217202935107,-14.6768299128519,32.1923234499164));
#25580=CARTESIAN_POINT('Ctrl Pts',(47.3886116492137,-14.7669045823039,32.2741675910805));
#25581=CARTESIAN_POINT('Ctrl Pts',(47.4871835016963,-14.7669045823054,32.3766099734313));
#25582=CARTESIAN_POINT('Ctrl Pts',(47.3673683496366,-14.6796363815825,32.0810224279246));
#25583=CARTESIAN_POINT('Ctrl Pts',(47.4538839948076,-14.7669045823063,32.1097343017417));
#25584=CARTESIAN_POINT('Ctrl Pts',(47.5723707391893,-14.7669045823054,32.1528630624247));
#25585=CARTESIAN_POINT('Origin',(46.5214090713319,-14.4544045823054,32.4564357525968));
#25586=CARTESIAN_POINT('Ctrl Pts',(47.3365522275749,-14.6753754514101,32.1308553965272));
#25587=CARTESIAN_POINT('Ctrl Pts',(47.3288511935299,-14.6738626255535,32.1395148208736));
#25588=CARTESIAN_POINT('Ctrl Pts',(47.3204694543763,-14.672133306496,32.1473732471581));
#25589=CARTESIAN_POINT('Ctrl Pts',(47.3115921752356,-14.6701816478973,32.1544833559118));
#25590=CARTESIAN_POINT('Ctrl Pts',(47.3024303523205,-14.6681674327095,32.1618213652585));
#25591=CARTESIAN_POINT('Ctrl Pts',(47.2927409984408,-14.6659157786114,32.1683633490873));
#25592=CARTESIAN_POINT('Ctrl Pts',(47.2826925623907,-14.6634429331545,32.1742040106302));
#25593=CARTESIAN_POINT('Ctrl Pts',(47.2720840164946,-14.6608322488258,32.1803702364718));
#25594=CARTESIAN_POINT('Ctrl Pts',(47.2610753316299,-14.6579745808512,32.1857558736056));
#25595=CARTESIAN_POINT('Ctrl Pts',(47.249822974311,-14.654922626477,32.1904958266184));
#25596=CARTESIAN_POINT('Ctrl Pts',(47.2381991868033,-14.6517699298355,32.1953922412145));
#25597=CARTESIAN_POINT('Ctrl Pts',(47.2263150294869,-14.6484098887065,32.1996007485996));
#25598=CARTESIAN_POINT('Ctrl Pts',(47.2143018980764,-14.6449389709829,32.203276757552));
#25599=CARTESIAN_POINT('Ctrl Pts',(47.2017394876037,-14.6413093517213,32.2071208454741));
#25600=CARTESIAN_POINT('Ctrl Pts',(47.1890355849868,-14.6375586122335,32.2103836120104));
#25601=CARTESIAN_POINT('Ctrl Pts',(47.1763025037334,-14.6338375655308,32.213233443221));
#25602=CARTESIAN_POINT('Ctrl Pts',(47.1737601155823,-14.6330945917872,32.2138024631588));
#25603=CARTESIAN_POINT('Ctrl Pts',(47.1712164612877,-14.6323529212115,32.2143549657298));
#25604=CARTESIAN_POINT('Ctrl Pts',(47.1686722902479,-14.6316139267952,32.2148922001907));
#25605=CARTESIAN_POINT('Ctrl Pts',(47.1511506028079,-14.6265244776268,32.2185921300137));
#25606=CARTESIAN_POINT('Ctrl Pts',(47.1334820998403,-14.6213443098223,32.2214605564035));
#25607=CARTESIAN_POINT('Ctrl Pts',(47.1157563330173,-14.6160583702064,32.2236226908213));
#25608=CARTESIAN_POINT('Ctrl Pts',(47.097382295013,-14.6105791118837,32.2258638993602));
#25609=CARTESIAN_POINT('Ctrl Pts',(47.0789461280096,-14.6049864174423,32.2273473716443));
#25610=CARTESIAN_POINT('Ctrl Pts',(47.0605081098987,-14.5993048356876,32.2282053347277));
#25611=CARTESIAN_POINT('Ctrl Pts',(47.0410799411183,-14.5933181440265,32.2291093717826));
#25612=CARTESIAN_POINT('Ctrl Pts',(47.0216489808795,-14.5872331623026,32.2293199157884));
#25613=CARTESIAN_POINT('Ctrl Pts',(47.0022532252739,-14.5811189364151,32.2289664413872));
#25614=CARTESIAN_POINT('Ctrl Pts',(46.9957233691671,-14.579060495586,32.2288474392187));
#25615=CARTESIAN_POINT('Ctrl Pts',(46.9891972935831,-14.5769990339995,32.2286642430615));
#25616=CARTESIAN_POINT('Ctrl Pts',(46.9826759110969,-14.5749379971501,32.2284209330324));
#25617=CARTESIAN_POINT('Ctrl Pts',(46.9572265784279,-14.5668949154057,32.2274714291682));
#25618=CARTESIAN_POINT('Ctrl Pts',(46.931861218954,-14.5588253828872,32.2255941220409));
#25619=CARTESIAN_POINT('Ctrl Pts',(46.9066155065142,-14.5507005312868,32.2229083201426));
#25620=CARTESIAN_POINT('Ctrl Pts',(46.8790846852559,-14.541840260946,32.2199794136135));
#25621=CARTESIAN_POINT('Ctrl Pts',(46.8516950608053,-14.5329148917791,32.2160902190248));
#25622=CARTESIAN_POINT('Ctrl Pts',(46.824464099245,-14.5239279943211,32.2113568491449));
#25623=CARTESIAN_POINT('Ctrl Pts',(46.7960547265605,-14.5145521917591,32.2064186442022));
#25624=CARTESIAN_POINT('Ctrl Pts',(46.7678165411628,-14.5051108161017,32.2005618978972));
#25625=CARTESIAN_POINT('Ctrl Pts',(46.739760685689,-14.4956334644481,32.1938663766911));
#25626=CARTESIAN_POINT('Ctrl Pts',(46.7105476404483,-14.48576521064,32.1868946925061));
#25627=CARTESIAN_POINT('Ctrl Pts',(46.6815308177066,-14.4758595759461,32.1790130518177));
#25628=CARTESIAN_POINT('Ctrl Pts',(46.6527371605959,-14.4659531415139,32.1702582008432));
#25629=CARTESIAN_POINT('Ctrl Pts',(46.6415474723804,-14.4621033383368,32.1668559219176));
#25630=CARTESIAN_POINT('Ctrl Pts',(46.6303917529274,-14.4582533144083,32.1633212693771));
#25631=CARTESIAN_POINT('Ctrl Pts',(46.6192727816467,-14.4544045595309,32.1596547825137));
#25632=CARTESIAN_POINT('Ctrl Pts',(46.8756079148278,-13.2959337131847,30.3286338949779));
#25633=CARTESIAN_POINT('Ctrl Pts',(46.7987395491116,-13.2044045823055,30.2789465107479));
#25634=CARTESIAN_POINT('Ctrl Pts',(46.6900312637983,-13.2044045823055,30.208677938091));
#25635=CARTESIAN_POINT('Ctrl Pts',(46.92843243666,-13.2959337183951,30.2469122618309));
#25636=CARTESIAN_POINT('Ctrl Pts',(46.8409103036131,-13.2092798238961,30.2226873530845));
#25637=CARTESIAN_POINT('Ctrl Pts',(46.7280932516454,-13.2044045823055,30.1716843588109));
#25638=CARTESIAN_POINT('Ctrl Pts',(46.9609035199605,-13.2734166054794,30.1546855181066));
#25639=CARTESIAN_POINT('Ctrl Pts',(46.8649125651919,-13.1931723515307,30.1556415155577));
#25640=CARTESIAN_POINT('Ctrl Pts',(46.7449795511239,-13.1931460297457,30.1261487195746));
#25641=CARTESIAN_POINT('Ctrl Pts',(46.9737602628944,-13.1901047283843,29.9799549937871));
#25642=CARTESIAN_POINT('Ctrl Pts',(46.8644616166491,-13.126047486873,30.0321632131418));
#25643=CARTESIAN_POINT('Ctrl Pts',(46.7309855396157,-13.1514900886124,30.0323613044136));
#25644=CARTESIAN_POINT('Ctrl Pts',(46.9552502383954,-13.1321577745915,29.901072349635));
#25645=CARTESIAN_POINT('Ctrl Pts',(46.8409166506036,-13.076707210209,29.9774630678603));
#25646=CARTESIAN_POINT('Ctrl Pts',(46.7015662774492,-13.1225166214136,29.9863856596473));
#25647=CARTESIAN_POINT('Ctrl Pts',(46.8583542680918,-12.9456232578405,29.7057221755481));
#25648=CARTESIAN_POINT('Ctrl Pts',(46.7341681938515,-12.9177593310992,29.8496415056206));
#25649=CARTESIAN_POINT('Ctrl Pts',(46.5801991147773,-13.0292493378239,29.8648950373845));
#25650=CARTESIAN_POINT('Ctrl Pts',(46.7403255599353,-12.8021218234308,29.6238045764194));
#25651=CARTESIAN_POINT('Ctrl Pts',(46.6127393034986,-12.7965826300641,29.8149715922655));
#25652=CARTESIAN_POINT('Ctrl Pts',(46.4557286211812,-12.9574790903504,29.802364931387));
#25653=CARTESIAN_POINT('Ctrl Pts',(46.611780876039,-12.6709337131846,29.5815526781396));
#25654=CARTESIAN_POINT('Ctrl Pts',(46.5008548189629,-12.7034528674627,29.8172453197959));
#25655=CARTESIAN_POINT('Ctrl Pts',(46.3272934177549,-12.8919045823054,29.7600133527852));
#25656=CARTESIAN_POINT('Origin',(46.6900312637982,-13.5169045823054,30.2086779380909));
#25657=CARTESIAN_POINT('Ctrl Pts',(46.3272934177549,-12.8919045823054,29.7600133527852));
#25658=CARTESIAN_POINT('Ctrl Pts',(46.3510582803902,-12.9040380872518,29.7678498292419));
#25659=CARTESIAN_POINT('Ctrl Pts',(46.3744908825881,-12.9162817766913,29.7763081787903));
#25660=CARTESIAN_POINT('Ctrl Pts',(46.3975595440145,-12.928642750848,29.7854378206903));
#25661=CARTESIAN_POINT('Ctrl Pts',(46.4180047368047,-12.9395979811943,29.7935291999558));
#25662=CARTESIAN_POINT('Ctrl Pts',(46.4381656146539,-12.9506462200823,29.8021486241306));
#25663=CARTESIAN_POINT('Ctrl Pts',(46.4580019948025,-12.9617976021836,29.8113620702633));
#25664=CARTESIAN_POINT('Ctrl Pts',(46.4763437466883,-12.9721087518064,29.8198813031936));
#25665=CARTESIAN_POINT('Ctrl Pts',(46.494408944746,-12.9825085406161,29.8289087144576));
#25666=CARTESIAN_POINT('Ctrl Pts',(46.512133587223,-12.9930011868727,29.8385186549454));
#25667=CARTESIAN_POINT('Ctrl Pts',(46.5287360724235,-13.0028295376794,29.8475201845917));
#25668=CARTESIAN_POINT('Ctrl Pts',(46.545040388102,-13.0127396637185,29.8570329809913));
#25669=CARTESIAN_POINT('Ctrl Pts',(46.5609542191196,-13.0227264646561,29.8671353539293));
#25670=CARTESIAN_POINT('Ctrl Pts',(46.5756034413391,-13.0319196542807,29.8764349315074));
#25671=CARTESIAN_POINT('Ctrl Pts',(46.5899220587733,-13.0411779829359,29.8862342539382));
#25672=CARTESIAN_POINT('Ctrl Pts',(46.6037973990955,-13.050486888578,29.8966073103123));
#25673=CARTESIAN_POINT('Ctrl Pts',(46.6109666672577,-13.0552967194935,29.9019669786938));
#25674=CARTESIAN_POINT('Ctrl Pts',(46.6180168846007,-13.0601198606027,29.9074800216699));
#25675=CARTESIAN_POINT('Ctrl Pts',(46.6249272899651,-13.064952825595,29.913157992511));
#25676=CARTESIAN_POINT('Ctrl Pts',(46.6354219377737,-13.0722925202713,29.9217809749703));
#25677=CARTESIAN_POINT('Ctrl Pts',(46.6455357175484,-13.0796093213736,29.9307303372787));
#25678=CARTESIAN_POINT('Ctrl Pts',(46.6552437527905,-13.0869314629286,29.9400978119362));
#25679=CARTESIAN_POINT('Ctrl Pts',(46.657225258145,-13.0884259839451,29.94200980553));
#25680=CARTESIAN_POINT('Ctrl Pts',(46.6591897022381,-13.0899206854313,29.9439392731158));
#25681=CARTESIAN_POINT('Ctrl Pts',(46.6611366181773,-13.091415738093,29.9458870799904));
#25682=CARTESIAN_POINT('Ctrl Pts',(46.6690767883509,-13.0975130596636,29.9538308836947));
#25683=CARTESIAN_POINT('Ctrl Pts',(46.6767231203679,-13.1036283475445,29.9621128151418));
#25684=CARTESIAN_POINT('Ctrl Pts',(46.6839712973621,-13.1097352160117,29.9707640545256));
#25685=CARTESIAN_POINT('Ctrl Pts',(46.6908187716549,-13.1155044770096,29.9789370253745));
#25686=CARTESIAN_POINT('Ctrl Pts',(46.6973113229118,-13.1212664690668,29.9874398372937));
#25687=CARTESIAN_POINT('Ctrl Pts',(46.7033197908501,-13.1269828032025,29.9962982353705));
#25688=CARTESIAN_POINT('Ctrl Pts',(46.708869254037,-13.1322624495576,30.0044799140491));
#25689=CARTESIAN_POINT('Ctrl Pts',(46.7140059302817,-13.1375032622583,30.0129650894761));
#25690=CARTESIAN_POINT('Ctrl Pts',(46.7185881839945,-13.1426584957564,30.021770855088));
#25691=CARTESIAN_POINT('Ctrl Pts',(46.7220537204315,-13.1465573740482,30.0284306132541));
#25692=CARTESIAN_POINT('Ctrl Pts',(46.7252014487815,-13.1504070236376,30.0352737091184));
#25693=CARTESIAN_POINT('Ctrl Pts',(46.7279518132448,-13.1541794056116,30.0423052686843));
#25694=CARTESIAN_POINT('Ctrl Pts',(46.732511491481,-13.1604334305654,30.053962505224));
#25695=CARTESIAN_POINT('Ctrl Pts',(46.7360832461396,-13.1665823184279,30.0663511701297));
#25696=CARTESIAN_POINT('Ctrl Pts',(46.7380257804305,-13.1723138052614,30.0792601551115));
#25697=CARTESIAN_POINT('Ctrl Pts',(46.7394171453584,-13.1764190557076,30.0885063800258));
#25698=CARTESIAN_POINT('Ctrl Pts',(46.7399127125584,-13.1802529865566,30.0979299368269));
#25699=CARTESIAN_POINT('Ctrl Pts',(46.7394048359389,-13.1837286680709,30.1074032472023));
#25700=CARTESIAN_POINT('Ctrl Pts',(46.7390261893497,-13.1863199567817,30.1144660583743));
#25701=CARTESIAN_POINT('Ctrl Pts',(46.7380907473884,-13.1887123032026,30.1215561565728));
#25702=CARTESIAN_POINT('Ctrl Pts',(46.736571681541,-13.1908748315003,30.128616804082));
#25703=CARTESIAN_POINT('Ctrl Pts',(46.7347953705731,-13.1934035716073,30.1368731318983));
#25704=CARTESIAN_POINT('Ctrl Pts',(46.7322325088647,-13.1955933528871,30.1450105858529));
#25705=CARTESIAN_POINT('Ctrl Pts',(46.7289332541082,-13.1974205800258,30.152924044601));
#25706=CARTESIAN_POINT('Ctrl Pts',(46.7256175087789,-13.1992569401429,30.1608770569688));
#25707=CARTESIAN_POINT('Ctrl Pts',(46.7215582129827,-13.2007270768473,30.1686033690315));
#25708=CARTESIAN_POINT('Ctrl Pts',(46.7168512222028,-13.2018302796858,30.1760119191985));
#25709=CARTESIAN_POINT('Ctrl Pts',(46.7120681506037,-13.2029513139965,30.1835402164805));
#25710=CARTESIAN_POINT('Ctrl Pts',(46.7066165411459,-13.2036934504427,30.1907399768785));
#25711=CARTESIAN_POINT('Ctrl Pts',(46.7006396922035,-13.2040802847478,30.1975385766591));
#25712=CARTESIAN_POINT('Ctrl Pts',(46.6972603068424,-13.204299005716,30.2013825902514));
#25713=CARTESIAN_POINT('Ctrl Pts',(46.6937137589004,-13.2044045823055,30.2050988114553));
#25714=CARTESIAN_POINT('Ctrl Pts',(46.6900312637983,-13.2044045823055,30.208677938091));
#25715=CARTESIAN_POINT('Ctrl Pts',(40.153012388794,-6.10843371318469,27.4594837601833));
#25716=CARTESIAN_POINT('Ctrl Pts',(40.0774385461352,-6.01690458230548,27.4078487322925));
#25717=CARTESIAN_POINT('Ctrl Pts',(40.0774385461352,-5.88746284406389,27.4078487322925));
#25718=CARTESIAN_POINT('Ctrl Pts',(40.1242331962091,-6.1027501834569,27.4915307194576));
#25719=CARTESIAN_POINT('Ctrl Pts',(40.0445399338239,-6.01222811250157,27.4559996605526));
#25720=CARTESIAN_POINT('Ctrl Pts',(40.03154277396,-5.88746285448661,27.4750225096052));
#25721=CARTESIAN_POINT('Ctrl Pts',(40.1009218644572,-6.11419577460901,27.5251818602439));
#25722=CARTESIAN_POINT('Ctrl Pts',(40.0112197519127,-6.02882146164764,27.5045867865534));
#25723=CARTESIAN_POINT('Ctrl Pts',(39.9853851293292,-5.9106557086834,27.5421815181704));
#25724=CARTESIAN_POINT('Ctrl Pts',(40.0720849274312,-6.1677431863177,27.5858654582369));
#25725=CARTESIAN_POINT('Ctrl Pts',(39.9576202879931,-6.0978035275072,27.5825741675642));
#25726=CARTESIAN_POINT('Ctrl Pts',(39.9069533697846,-5.99623773973419,27.655803900523));
#25727=CARTESIAN_POINT('Ctrl Pts',(40.066209509497,-6.20950986590618,27.6131711938117));
#25728=CARTESIAN_POINT('Ctrl Pts',(39.9366893821544,-6.15046547604274,27.6129453446739));
#25729=CARTESIAN_POINT('Ctrl Pts',(39.8741328667897,-6.05824038173977,27.7030926868508));
#25730=CARTESIAN_POINT('Ctrl Pts',(40.0694547712359,-6.3546301407075,27.6798043375759));
#25731=CARTESIAN_POINT('Ctrl Pts',(39.8956196052046,-6.32861804115437,27.6726104606096));
#25732=CARTESIAN_POINT('Ctrl Pts',(39.8004265980845,-6.26685602924677,27.8090735783451));
#25733=CARTESIAN_POINT('Ctrl Pts',(40.0973050091181,-6.47617237885447,27.7056712663594));
#25734=CARTESIAN_POINT('Ctrl Pts',(39.8976526694977,-6.47276044373899,27.6698898995951));
#25735=CARTESIAN_POINT('Ctrl Pts',(39.7815264643901,-6.43425950785913,27.8359939147546));
#25736=CARTESIAN_POINT('Ctrl Pts',(40.1355062937731,-6.59535043767467,27.7182681608758));
#25737=CARTESIAN_POINT('Ctrl Pts',(39.9147276464474,-6.59535043767467,27.6454662811233));
#25738=CARTESIAN_POINT('Ctrl Pts',(39.7815264758118,-6.59535043767467,27.8359938984173));
#25739=CARTESIAN_POINT('Ctrl Pts',(-46.7085547781037,-13.2959337131847,
-30.163770311099));
#25740=CARTESIAN_POINT('Ctrl Pts',(-46.6316864123875,-13.2044045823055,
-30.114082926869));
#25741=CARTESIAN_POINT('Ctrl Pts',(-46.5229781270742,-13.2044045823055,
-30.0438143542121));
#25742=CARTESIAN_POINT('Ctrl Pts',(-46.761379299936,-13.2959337183952,-30.0820486779521));
#25743=CARTESIAN_POINT('Ctrl Pts',(-46.673857166889,-13.2092798238962,-30.057823769206));
#25744=CARTESIAN_POINT('Ctrl Pts',(-46.5610401149215,-13.2044045823055,
-30.0068207749323));
#25745=CARTESIAN_POINT('Ctrl Pts',(-46.7938503832366,-13.2734166054797,
-29.9898219342279));
#25746=CARTESIAN_POINT('Ctrl Pts',(-46.6978594284684,-13.1931723515309,
-29.9907779316791));
#25747=CARTESIAN_POINT('Ctrl Pts',(-46.5779264144001,-13.1931460297457,
-29.961285135696));
#25748=CARTESIAN_POINT('Ctrl Pts',(-46.8067071261701,-13.1901047283841,
-29.8150914099081));
#25749=CARTESIAN_POINT('Ctrl Pts',(-46.6974084799243,-13.1260474868728,
-29.8672996292628));
#25750=CARTESIAN_POINT('Ctrl Pts',(-46.5639324028913,-13.1514900886123,
-29.8674977205345));
#25751=CARTESIAN_POINT('Ctrl Pts',(-46.7881971016712,-13.1321577745915,
-29.7362087657564));
#25752=CARTESIAN_POINT('Ctrl Pts',(-46.6738635138795,-13.0767072102089,
-29.8125994839813));
#25753=CARTESIAN_POINT('Ctrl Pts',(-46.5345131407245,-13.1225166214137,
-29.8215220757683));
#25754=CARTESIAN_POINT('Ctrl Pts',(-46.691301131368,-12.9456232578405,-29.5408585916687));
#25755=CARTESIAN_POINT('Ctrl Pts',(-46.5671150571274,-12.9177593310994,
-29.684777921742));
#25756=CARTESIAN_POINT('Ctrl Pts',(-46.4131459780545,-13.0292493378237,
-29.7000314535059));
#25757=CARTESIAN_POINT('Ctrl Pts',(-46.5732724232098,-12.8021218234311,
-29.4589409925433));
#25758=CARTESIAN_POINT('Ctrl Pts',(-46.4456861667736,-12.7965826300651,
-29.6501080083888));
#25759=CARTESIAN_POINT('Ctrl Pts',(-46.2886754844563,-12.9574790903503,
-29.6375013475079));
#25760=CARTESIAN_POINT('Ctrl Pts',(-46.4447277393149,-12.6709337131846,
-29.4166890942607));
#25761=CARTESIAN_POINT('Ctrl Pts',(-46.3338016822388,-12.7034528674627,
-29.6523817359171));
#25762=CARTESIAN_POINT('Ctrl Pts',(-46.1602402810308,-12.8919045823054,
-29.5951497689063));
#25763=CARTESIAN_POINT('Origin',(-46.5229781270741,-13.5169045823054,-30.0438143542121));
#25764=CARTESIAN_POINT('Ctrl Pts',(-46.1602402810308,-12.8919045823054,
-29.5951497689063));
#25765=CARTESIAN_POINT('Ctrl Pts',(-46.1840051436653,-12.9040380872515,
-29.6029862453627));
#25766=CARTESIAN_POINT('Ctrl Pts',(-46.2074377458625,-12.9162817766905,
-29.6114445949109));
#25767=CARTESIAN_POINT('Ctrl Pts',(-46.2305064072882,-12.9286427508468,
-29.6205742368105));
#25768=CARTESIAN_POINT('Ctrl Pts',(-46.2509516000786,-12.9395979811933,
-29.6286656160761));
#25769=CARTESIAN_POINT('Ctrl Pts',(-46.271112477928,-12.9506462200813,-29.6372850402509));
#25770=CARTESIAN_POINT('Ctrl Pts',(-46.2909488580768,-12.9617976021827,
-29.6464984863837));
#25771=CARTESIAN_POINT('Ctrl Pts',(-46.3092906099622,-12.9721087518052,
-29.6550177193137));
#25772=CARTESIAN_POINT('Ctrl Pts',(-46.3273558080195,-12.9825085406146,
-29.6640451305775));
#25773=CARTESIAN_POINT('Ctrl Pts',(-46.3450804504962,-12.9930011868708,
-29.673655071065));
#25774=CARTESIAN_POINT('Ctrl Pts',(-46.3616829356962,-13.0028295376772,
-29.6826566007109));
#25775=CARTESIAN_POINT('Ctrl Pts',(-46.3779872513743,-13.012739663716,-29.6921693971101));
#25776=CARTESIAN_POINT('Ctrl Pts',(-46.3939010823914,-13.0227264646533,
-29.7022717700477));
#25777=CARTESIAN_POINT('Ctrl Pts',(-46.4085503046105,-13.0319196542775,
-29.7115713476254));
#25778=CARTESIAN_POINT('Ctrl Pts',(-46.4228689220442,-13.0411779829323,
-29.7213706700557));
#25779=CARTESIAN_POINT('Ctrl Pts',(-46.436744262366,-13.0504868885741,-29.7317437264293));
#25780=CARTESIAN_POINT('Ctrl Pts',(-46.4439135305301,-13.0552967194909,
-29.7371033948121));
#25781=CARTESIAN_POINT('Ctrl Pts',(-46.450963747875,-13.0601198606014,-29.7426164377896));
#25782=CARTESIAN_POINT('Ctrl Pts',(-46.4578741532412,-13.0649528255949,
-29.7482944086321));
#25783=CARTESIAN_POINT('Ctrl Pts',(-46.4683688010496,-13.0722925202711,
-29.7569173910913));
#25784=CARTESIAN_POINT('Ctrl Pts',(-46.4784825808242,-13.0796093213733,
-29.7658667533996));
#25785=CARTESIAN_POINT('Ctrl Pts',(-46.488190616066,-13.0869314629283,-29.7752342280569));
#25786=CARTESIAN_POINT('Ctrl Pts',(-46.4901721214206,-13.0884259839449,
-29.7771462216509));
#25787=CARTESIAN_POINT('Ctrl Pts',(-46.4921365655139,-13.0899206854312,
-29.7790756892368));
#25788=CARTESIAN_POINT('Ctrl Pts',(-46.4940834814532,-13.091415738093,-29.7810234961116));
#25789=CARTESIAN_POINT('Ctrl Pts',(-46.5020236516268,-13.0975130596636,
-29.7889672998159));
#25790=CARTESIAN_POINT('Ctrl Pts',(-46.5096699836439,-13.1036283475445,
-29.797249231263));
#25791=CARTESIAN_POINT('Ctrl Pts',(-46.516918160638,-13.1097352160118,-29.8059004706468));
#25792=CARTESIAN_POINT('Ctrl Pts',(-46.5237656349308,-13.1155044770098,
-29.8140734414958));
#25793=CARTESIAN_POINT('Ctrl Pts',(-46.5302581861878,-13.1212664690669,
-29.822576253415));
#25794=CARTESIAN_POINT('Ctrl Pts',(-46.5362666541262,-13.1269828032027,
-29.8314346514919));
#25795=CARTESIAN_POINT('Ctrl Pts',(-46.5418161173131,-13.1322624495578,
-29.8396163301706));
#25796=CARTESIAN_POINT('Ctrl Pts',(-46.5469527935578,-13.1375032622586,
-29.8481015055977));
#25797=CARTESIAN_POINT('Ctrl Pts',(-46.5515350472707,-13.1426584957567,
-29.8569072712097));
#25798=CARTESIAN_POINT('Ctrl Pts',(-46.5550005837076,-13.1465573740484,
-29.8635670293756));
#25799=CARTESIAN_POINT('Ctrl Pts',(-46.5581483120574,-13.1504070236377,
-29.8704101252397));
#25800=CARTESIAN_POINT('Ctrl Pts',(-46.5608986765207,-13.1541794056116,
-29.8774416848054));
#25801=CARTESIAN_POINT('Ctrl Pts',(-46.5654583547569,-13.1604334305654,
-29.8890989213451));
#25802=CARTESIAN_POINT('Ctrl Pts',(-46.5690301094155,-13.1665823184279,
-29.9014875862509));
#25803=CARTESIAN_POINT('Ctrl Pts',(-46.5709726437064,-13.1723138052614,
-29.9143965712326));
#25804=CARTESIAN_POINT('Ctrl Pts',(-46.5723640086343,-13.1764190557077,
-29.9236427961473));
#25805=CARTESIAN_POINT('Ctrl Pts',(-46.5728595758343,-13.1802529865569,
-29.9330663529488));
#25806=CARTESIAN_POINT('Ctrl Pts',(-46.5723516992147,-13.1837286680714,
-29.9425396633246));
#25807=CARTESIAN_POINT('Ctrl Pts',(-46.5719730526255,-13.186319956782,-29.9496024744962));
#25808=CARTESIAN_POINT('Ctrl Pts',(-46.5710376106642,-13.1887123032027,
-29.9566925726943));
#25809=CARTESIAN_POINT('Ctrl Pts',(-46.5695185448169,-13.1908748315003,
-29.9637532202032));
#25810=CARTESIAN_POINT('Ctrl Pts',(-46.567742233849,-13.1934035716073,-29.9720095480195));
#25811=CARTESIAN_POINT('Ctrl Pts',(-46.5651793721406,-13.1955933528871,
-29.980147001974));
#25812=CARTESIAN_POINT('Ctrl Pts',(-46.5618801173841,-13.1974205800258,
-29.9880604607222));
#25813=CARTESIAN_POINT('Ctrl Pts',(-46.5585643720548,-13.1992569401429,
-29.99601347309));
#25814=CARTESIAN_POINT('Ctrl Pts',(-46.5545050762587,-13.2007270768473,
-30.0037397851527));
#25815=CARTESIAN_POINT('Ctrl Pts',(-46.5497980854788,-13.2018302796858,
-30.0111483353198));
#25816=CARTESIAN_POINT('Ctrl Pts',(-46.5450150138797,-13.2029513139966,
-30.0186766326018));
#25817=CARTESIAN_POINT('Ctrl Pts',(-46.5395634044218,-13.2036934504427,
-30.0258763929997));
#25818=CARTESIAN_POINT('Ctrl Pts',(-46.5335865554794,-13.2040802847478,
-30.0326749927803));
#25819=CARTESIAN_POINT('Ctrl Pts',(-46.5302071701183,-13.204299005716,-30.0365190063726));
#25820=CARTESIAN_POINT('Ctrl Pts',(-46.5266606221764,-13.2044045823055,
-30.0402352275765));
#25821=CARTESIAN_POINT('Ctrl Pts',(-46.5229781270742,-13.2044045823055,
-30.0438143542121));
#25822=CARTESIAN_POINT('Ctrl Pts',(-39.9859592520697,-6.10843371318464,
-27.2946201763047));
#25823=CARTESIAN_POINT('Ctrl Pts',(-39.9103854094108,-6.01690458230545,
-27.242985148414));
#25824=CARTESIAN_POINT('Ctrl Pts',(-39.9103854094107,-5.88746284406389,
-27.2429851484142));
#25825=CARTESIAN_POINT('Ctrl Pts',(-39.9571800594855,-6.1027501834571,-27.3266671355783));
#25826=CARTESIAN_POINT('Ctrl Pts',(-39.8774867971012,-6.01222811250108,
-27.2911360766742));
#25827=CARTESIAN_POINT('Ctrl Pts',(-39.8644896372362,-5.88746285448629,
-27.3101589257258));
#25828=CARTESIAN_POINT('Ctrl Pts',(-39.9338687277324,-6.11419577460858,
-27.3603182763651));
#25829=CARTESIAN_POINT('Ctrl Pts',(-39.844166615188,-6.02882146164754,-27.3397232026743));
#25830=CARTESIAN_POINT('Ctrl Pts',(-39.8183319926051,-5.91065570868315,
-27.3773179342917));
#25831=CARTESIAN_POINT('Ctrl Pts',(-39.9050317907078,-6.16774318631813,
-27.421001874358));
#25832=CARTESIAN_POINT('Ctrl Pts',(-39.7905671512696,-6.09780352750732,
-27.4177105836857));
#25833=CARTESIAN_POINT('Ctrl Pts',(-39.7399002330605,-5.99623773973444,
-27.4909403166441));
#25834=CARTESIAN_POINT('Ctrl Pts',(-39.8991563727726,-6.20950986590617,
-27.4483076099329));
#25835=CARTESIAN_POINT('Ctrl Pts',(-39.7696362454303,-6.15046547604259,
-27.4480817607952));
#25836=CARTESIAN_POINT('Ctrl Pts',(-39.7070797300657,-6.05824038173967,
-27.5382291029718));
#25837=CARTESIAN_POINT('Ctrl Pts',(-39.9024016345124,-6.35463014070754,
-27.514940753697));
#25838=CARTESIAN_POINT('Ctrl Pts',(-39.7285664684805,-6.32861804115478,
-27.5077468767305));
#25839=CARTESIAN_POINT('Ctrl Pts',(-39.6333734613603,-6.26685602924698,
-27.6442099944664));
#25840=CARTESIAN_POINT('Ctrl Pts',(-39.930251872391,-6.47617237885538,-27.5408076824795));
#25841=CARTESIAN_POINT('Ctrl Pts',(-39.7305995327717,-6.47276044373959,
-27.5050263157192));
#25842=CARTESIAN_POINT('Ctrl Pts',(-39.6144733276653,-6.43425950785897,
-27.6711303308768));
#25843=CARTESIAN_POINT('Ctrl Pts',(-39.968453157049,-6.59535043767467,-27.553404576997));
#25844=CARTESIAN_POINT('Ctrl Pts',(-39.7476745097234,-6.59535043767467,
-27.4806026972444));
#25845=CARTESIAN_POINT('Ctrl Pts',(-39.6144733390877,-6.59535043767467,
-27.6711303145384));
#25846=CARTESIAN_POINT('Origin',(-40.1684106479774,-5.8874628440639,-27.419278160932));
#25847=CARTESIAN_POINT('Origin',(-39.8705894675228,-6.59535043767467,-27.8501855539351));
#25848=CARTESIAN_POINT('Origin',(0.0835265683620477,-13.5169045823054,0.0824317919394229));
#25849=CARTESIAN_POINT('Origin',(-45.6231018412815,-13.5169045823054,-31.3923375671359));
#25850=CARTESIAN_POINT('Origin',(4.47264233855679,-12.8919045823054,-13.2279806039107));
#25851=CARTESIAN_POINT('Origin',(-39.8705894675228,-12.8919045823054,-27.8501855539351));
#25852=CARTESIAN_POINT('Origin',(-39.8705894675228,-14.7669045823054,-27.8501855539351));
#25853=CARTESIAN_POINT('Origin',(-39.8705894675228,-12.8919045823054,-27.8501855539351));
#25854=CARTESIAN_POINT('Origin',(0.0835265683620477,-12.8919045823054,0.0824317919394229));
#25855=CARTESIAN_POINT('Ctrl Pts',(-34.1929414312581,-13.2044045823054,
-34.5829146143929));
#25856=CARTESIAN_POINT('Ctrl Pts',(-34.1680403069389,-13.2044045823054,
-34.5830483771525));
#25857=CARTESIAN_POINT('Ctrl Pts',(-34.1434060402122,-13.2030022087212,
-34.5831873558775));
#25858=CARTESIAN_POINT('Ctrl Pts',(-34.1189478462075,-13.2001447338013,
-34.5833336044956));
#25859=CARTESIAN_POINT('Ctrl Pts',(-34.094935431709,-13.1973393397406,-34.5834771875598));
#25860=CARTESIAN_POINT('Ctrl Pts',(-34.071092686807,-13.193131465653,-34.5836278043066));
#25861=CARTESIAN_POINT('Ctrl Pts',(-34.0473441304472,-13.1874220362844,
-34.5837878944019));
#25862=CARTESIAN_POINT('Ctrl Pts',(-34.0414387028137,-13.1860023027455,
-34.5838277031574));
#25863=CARTESIAN_POINT('Ctrl Pts',(-34.0355391523601,-13.184489476873,-34.5838680990468));
#25864=CARTESIAN_POINT('Ctrl Pts',(-34.0296444264616,-13.1828815404475,
-34.5839091214968));
#25865=CARTESIAN_POINT('Ctrl Pts',(-34.0075950038454,-13.1768669995857,
-34.5840625673653));
#25866=CARTESIAN_POINT('Ctrl Pts',(-33.9861383901114,-13.1696750914267,
-34.5842210504987));
#25867=CARTESIAN_POINT('Ctrl Pts',(-33.9652968749802,-13.1611455958503,
-34.5843848815461));
#25868=CARTESIAN_POINT('Ctrl Pts',(-33.9444553598491,-13.1526161002739,
-34.5845487125934));
#25869=CARTESIAN_POINT('Ctrl Pts',(-33.9242285971081,-13.1427495299604,
-34.5847179161621));
#25870=CARTESIAN_POINT('Ctrl Pts',(-33.9046719627877,-13.1313389816383,
-34.5848921573841));
#25871=CARTESIAN_POINT('Ctrl Pts',(-33.8980736200928,-13.1274891009823,
-34.5849509457869));
#25872=CARTESIAN_POINT('Ctrl Pts',(-33.8915791335182,-13.1234784566375,
-34.5850085468875));
#25873=CARTESIAN_POINT('Ctrl Pts',(-33.8851706792542,-13.1192883941035,
-34.5850653658929));
#25874=CARTESIAN_POINT('Ctrl Pts',(-33.8744851575582,-13.1123018412982,
-34.5851601064793));
#25875=CARTESIAN_POINT('Ctrl Pts',(-33.86420405785,-13.104916612557,-34.5852512337119));
#25876=CARTESIAN_POINT('Ctrl Pts',(-33.854304863418,-13.0970443878827,-34.5853399947737));
#25877=CARTESIAN_POINT('Ctrl Pts',(-33.8506201662143,-13.0941141732634,
-34.585373033587));
#25878=CARTESIAN_POINT('Ctrl Pts',(-33.846988814313,-13.0911162306683,-34.5854057405226));
#25879=CARTESIAN_POINT('Ctrl Pts',(-33.843411289417,-13.088045086031,-34.5854381632075));
#25880=CARTESIAN_POINT('Ctrl Pts',(-33.8339347977663,-13.0799099430592,
-34.5855240475303));
#25881=CARTESIAN_POINT('Ctrl Pts',(-33.8248750204272,-13.071295025075,-34.585607570458));
#25882=CARTESIAN_POINT('Ctrl Pts',(-33.8163189539575,-13.0621639241565,
-34.5856851785447));
#25883=CARTESIAN_POINT('Ctrl Pts',(-33.8077628874879,-13.053032823238,-34.5857627866313));
#25884=CARTESIAN_POINT('Ctrl Pts',(-33.7997113740151,-13.0433849467635,
-34.5858333463418));
#25885=CARTESIAN_POINT('Ctrl Pts',(-33.7922539399743,-13.0331862397832,
-34.5859071947319));
#25886=CARTESIAN_POINT('Ctrl Pts',(-33.7886347380691,-13.0282366579925,
-34.5859430344366));
#25887=CARTESIAN_POINT('Ctrl Pts',(-33.7851501101384,-13.0231465710756,
-34.5859776488828));
#25888=CARTESIAN_POINT('Ctrl Pts',(-33.7818190947318,-13.0179182754031,
-34.5860108176103));
#25889=CARTESIAN_POINT('Ctrl Pts',(-33.7743334296083,-13.0061689239908,
-34.5860853564389));
#25890=CARTESIAN_POINT('Ctrl Pts',(-33.7677565298757,-12.993904917636,-34.5861511719067));
#25891=CARTESIAN_POINT('Ctrl Pts',(-33.7622772370354,-12.9812267133663,
-34.5862062450479));
#25892=CARTESIAN_POINT('Ctrl Pts',(-33.7569248855037,-12.9688422309121,
-34.5862600422842));
#25893=CARTESIAN_POINT('Ctrl Pts',(-33.7526202667613,-12.9560629035318,
-34.5863035817044));
#25894=CARTESIAN_POINT('Ctrl Pts',(-33.7494937045786,-12.9430006092192,
-34.5863353326885));
#25895=CARTESIAN_POINT('Ctrl Pts',(-33.7464514954637,-12.9302907290069,
-34.5863662270471));
#25896=CARTESIAN_POINT('Ctrl Pts',(-33.7445248498179,-12.9173133257079,
-34.5863859545434));
#25897=CARTESIAN_POINT('Ctrl Pts',(-33.7437856904794,-12.9041833323892,
-34.5863935387912));
#25898=CARTESIAN_POINT('Ctrl Pts',(-33.7435560357035,-12.9001038795344,
-34.5863958951962));
#25899=CARTESIAN_POINT('Ctrl Pts',(-33.7434406426353,-12.896009762608,-34.5863970829463));
#25900=CARTESIAN_POINT('Ctrl Pts',(-33.7434406426353,-12.8919045823054,
-34.5863970829463));
#25901=CARTESIAN_POINT('Origin',(7.03184852472011,-13.5169045823054,-20.9890175706648));
#25902=CARTESIAN_POINT('Origin',(-34.1929414312581,-13.5169045823054,-34.5829146143929));
#25903=CARTESIAN_POINT('Origin',(19.8255764196421,-11.3294045823054,-10.0436051386457));
#25904=CARTESIAN_POINT('Origin',(19.2694623393243,-11.3294045823054,-9.75836466172779));
#25905=CARTESIAN_POINT('Ctrl Pts',(34.2554728506688,-10.7044045823054,-34.2464116713807));
#25906=CARTESIAN_POINT('Ctrl Pts',(34.2554728506688,-11.0169045823054,-34.2464116713807));
#25907=CARTESIAN_POINT('Ctrl Pts',(34.0350086811056,-11.0169045823054,-34.02493526194));
#25908=CARTESIAN_POINT('Ctrl Pts',(34.3179692702965,-10.7044046073823,-34.1842008865451));
#25909=CARTESIAN_POINT('Ctrl Pts',(34.2942143893231,-11.034944931327,-34.2078471963309));
#25910=CARTESIAN_POINT('Ctrl Pts',(34.0599086143365,-11.0169045823054,-33.9753904270529));
#25911=CARTESIAN_POINT('Ctrl Pts',(34.3787106266475,-10.718650676671,-34.123396588746));
#25912=CARTESIAN_POINT('Ctrl Pts',(34.3266517180123,-11.063071415628,-34.1754830902681));
#25913=CARTESIAN_POINT('Ctrl Pts',(34.084059078646,-11.0240276257398,-33.9269149742339));
#25914=CARTESIAN_POINT('Ctrl Pts',(34.4961549499042,-10.7765752156551,-34.005239772344));
#25915=CARTESIAN_POINT('Ctrl Pts',(34.377889924456,-11.1314870357703,-34.1245297803838));
#25916=CARTESIAN_POINT('Ctrl Pts',(34.1306669722307,-11.0529899027286,-33.8326289586376));
#25917=CARTESIAN_POINT('Ctrl Pts',(34.5495749085591,-10.8185639645427,-33.95119120071));
#25918=CARTESIAN_POINT('Ctrl Pts',(34.3941245222472,-11.1704305366375,-34.1085208978415));
#25919=CARTESIAN_POINT('Ctrl Pts',(34.1518217449246,-11.0739842709863,-33.7894549020566));
#25920=CARTESIAN_POINT('Ctrl Pts',(34.6445000675177,-10.9314866347395,-33.8547910317575));
#25921=CARTESIAN_POINT('Ctrl Pts',(34.4101878971174,-11.2441510617714,-34.0933162668226));
#25922=CARTESIAN_POINT('Ctrl Pts',(34.1893600410275,-11.1304456109602,-33.7123980746659));
#25923=CARTESIAN_POINT('Ctrl Pts',(34.6830766509629,-10.999293715727,-33.8154157688772));
#25924=CARTESIAN_POINT('Ctrl Pts',(34.4081565684008,-11.2750326114058,-34.0959850824422));
#25925=CARTESIAN_POINT('Ctrl Pts',(34.2045857764074,-11.1643491474262,-33.6808947305844));
#25926=CARTESIAN_POINT('Ctrl Pts',(34.7377600096266,-11.1560957480195,-33.7595102293617));
#25927=CARTESIAN_POINT('Ctrl Pts',(34.3990150768359,-11.3160025899706,-34.1063442197293));
#25928=CARTESIAN_POINT('Ctrl Pts',(34.2261553564882,-11.2427501667525,-33.636152825177));
#25929=CARTESIAN_POINT('Ctrl Pts',(34.752355455618,-11.2411599901507,-33.7445354063799));
#25930=CARTESIAN_POINT('Ctrl Pts',(34.3930336310338,-11.3235538600012,-34.1127997789392));
#25931=CARTESIAN_POINT('Ctrl Pts',(34.2319046000613,-11.2852822850309,-33.6241606027471));
#25932=CARTESIAN_POINT('Ctrl Pts',(34.7523554432478,-11.3294045823054,-33.7445354190578));
#25933=CARTESIAN_POINT('Ctrl Pts',(34.3930336345113,-11.3294045823054,-34.112799775138));
#25934=CARTESIAN_POINT('Ctrl Pts',(34.2319046026008,-11.3294045823054,-33.6241606104485));
#25935=CARTESIAN_POINT('Ctrl Pts',(34.2319046026008,-11.3294045823054,-33.6241606104486));
#25936=CARTESIAN_POINT('Ctrl Pts',(34.2319046026008,-11.3159760597526,-33.6241606104486));
#25937=CARTESIAN_POINT('Ctrl Pts',(34.2313701235195,-11.3026664608407,-33.6252754613691));
#25938=CARTESIAN_POINT('Ctrl Pts',(34.2303262007385,-11.2895978753996,-33.6274497561314));
#25939=CARTESIAN_POINT('Ctrl Pts',(34.2292621420608,-11.2762772141441,-33.6296659901783));
#25940=CARTESIAN_POINT('Ctrl Pts',(34.2276689072531,-11.2632073639016,-33.6329826731796));
#25941=CARTESIAN_POINT('Ctrl Pts',(34.2255963210687,-11.2505062466188,-33.6372928524732));
#25942=CARTESIAN_POINT('Ctrl Pts',(34.2234556661661,-11.2373879940772,-33.641744588428));
#25943=CARTESIAN_POINT('Ctrl Pts',(34.2208037862985,-11.2246635682847,-33.6472558461806));
#25944=CARTESIAN_POINT('Ctrl Pts',(34.2177184383504,-11.212443933042,-33.6536619679777));
#25945=CARTESIAN_POINT('Ctrl Pts',(34.2169622262201,-11.2094489267884,-33.6552320946191));
#25946=CARTESIAN_POINT('Ctrl Pts',(34.2161800730707,-11.2064841392024,-33.6568557778232));
#25947=CARTESIAN_POINT('Ctrl Pts',(34.2153733079896,-11.2035509891889,-33.6585302199796));
#25948=CARTESIAN_POINT('Ctrl Pts',(34.2139688035159,-11.1984446423577,-33.6614452711567));
#25949=CARTESIAN_POINT('Ctrl Pts',(34.212499775488,-11.19346758092,-33.6644930487698));
#25950=CARTESIAN_POINT('Ctrl Pts',(34.2109735777768,-11.18862206557,-33.6676578884119));
#25951=CARTESIAN_POINT('Ctrl Pts',(34.2077635090097,-11.1784304387767,-33.6743145311349));
#25952=CARTESIAN_POINT('Ctrl Pts',(34.2042866771259,-11.1687879968701,-33.6814958205249));
#25953=CARTESIAN_POINT('Ctrl Pts',(34.2005926189786,-11.1596600078883,-33.6891304879687));
#25954=CARTESIAN_POINT('Ctrl Pts',(34.1964998574857,-11.149546826037,-33.697589172613));
#25955=CARTESIAN_POINT('Ctrl Pts',(34.1921518053766,-11.1400969285548,-33.706563836516));
#25956=CARTESIAN_POINT('Ctrl Pts',(34.1875784009834,-11.1312146907202,-33.7159897117274));
#25957=CARTESIAN_POINT('Ctrl Pts',(34.1827894597102,-11.1219138479108,-33.7258598126315));
#25958=CARTESIAN_POINT('Ctrl Pts',(34.1777533000673,-11.113235294885,-33.7362249700341));
#25959=CARTESIAN_POINT('Ctrl Pts',(34.1724822309008,-11.1050933657994,-33.7470566898643));
#25960=CARTESIAN_POINT('Ctrl Pts',(34.1718566195823,-11.1041270185878,-33.7483422822765));
#25961=CARTESIAN_POINT('Ctrl Pts',(34.1712276759863,-11.1031682588511,-33.7496344946185));
#25962=CARTESIAN_POINT('Ctrl Pts',(34.1705954024983,-11.1022169660873,-33.7509333164964));
#25963=CARTESIAN_POINT('Ctrl Pts',(34.1678668043632,-11.0981116292185,-33.7565384272931));
#25964=CARTESIAN_POINT('Ctrl Pts',(34.1651007375946,-11.0941782436166,-33.7622161899406));
#25965=CARTESIAN_POINT('Ctrl Pts',(34.162294156686,-11.0904041712721,-33.7679726124447));
#25966=CARTESIAN_POINT('Ctrl Pts',(34.1537568943567,-11.0789239229899,-33.785482917901));
#25967=CARTESIAN_POINT('Ctrl Pts',(34.1448975552561,-11.0689908784591,-33.8035911672373));
#25968=CARTESIAN_POINT('Ctrl Pts',(34.1357398214884,-11.0604019317832,-33.8222409108108));
#25969=CARTESIAN_POINT('Ctrl Pts',(34.1265820877206,-11.0518129851072,-33.8408906543843));
#25970=CARTESIAN_POINT('Ctrl Pts',(34.1171258275511,-11.0445686309467,-33.8600822647688));
#25971=CARTESIAN_POINT('Ctrl Pts',(34.1073798559662,-11.0385127393806,-33.8797906568829));
#25972=CARTESIAN_POINT('Ctrl Pts',(34.0969865438925,-11.0320546073838,-33.9008081068036));
#25973=CARTESIAN_POINT('Ctrl Pts',(34.0865219665413,-11.0271158190903,-33.9218908816861));
#25974=CARTESIAN_POINT('Ctrl Pts',(34.075958462414,-11.0235921824178,-33.943096926213));
#25975=CARTESIAN_POINT('Ctrl Pts',(34.0652130000177,-11.0200078504663,-33.9646682486918));
#25976=CARTESIAN_POINT('Ctrl Pts',(34.0543651598294,-11.0178879088427,-33.986367234626));
#25977=CARTESIAN_POINT('Ctrl Pts',(34.0433794528319,-11.0171750715249,-34.008264765842));
#25978=CARTESIAN_POINT('Ctrl Pts',(34.0405982750767,-11.0169946072825,-34.0138084169449));
#25979=CARTESIAN_POINT('Ctrl Pts',(34.037808230387,-11.0169045823054,-34.0193648371644));
#25980=CARTESIAN_POINT('Ctrl Pts',(34.0350086811056,-11.0169045823054,-34.02493526194));
#25981=CARTESIAN_POINT('Origin',(0.0835265683620477,-14.4544045823054,0.0824317919394229));
#25982=CARTESIAN_POINT('Origin',(9.92432302202933,-14.4544045823054,19.2683675629017));
#25983=CARTESIAN_POINT('Origin',(-4.99063502851588,-14.4544045823054,15.4703110263562));
#25984=CARTESIAN_POINT('Origin',(18.7518431265311,-14.4544045823054,23.2994061884498));
#25985=CARTESIAN_POINT('Ctrl Pts',(47.3447344898066,-14.6836564585996,32.1335442243844));
#25986=CARTESIAN_POINT('Ctrl Pts',(47.2330781733367,-14.7195047625521,32.3620574462612));
#25987=CARTESIAN_POINT('Ctrl Pts',(47.0639886181844,-14.9046273277204,32.306300072934));
#25988=CARTESIAN_POINT('Ctrl Pts',(46.88743888664,-14.2208393515121,31.9832691884364));
#25989=CARTESIAN_POINT('Ctrl Pts',(46.7760368073049,-14.2572370951372,32.2113478057363));
#25990=CARTESIAN_POINT('Ctrl Pts',(46.6069803497971,-14.44181022121,32.1556013463856));
#25991=CARTESIAN_POINT('Ctrl Pts',(46.4299123063411,-13.7582547217156,31.8329303749028));
#25992=CARTESIAN_POINT('Ctrl Pts',(46.3184777038413,-13.7949155819421,32.060467441034));
#25993=CARTESIAN_POINT('Ctrl Pts',(46.1497497223463,-13.9792255914392,32.0048292968144));
#25994=CARTESIAN_POINT('Ctrl Pts',(45.9721485234461,-13.2959337131846,31.6825266249535));
#25995=CARTESIAN_POINT('Ctrl Pts',(45.8603516012668,-13.3325299785125,31.9094001080471));
#25996=CARTESIAN_POINT('Ctrl Pts',(45.6922912884794,-13.5169045823054,31.8539821279529));
#25997=CARTESIAN_POINT('Origin',(45.7901549780056,-13.5169045823054,31.5572011510148));
#25998=CARTESIAN_POINT('Origin',(0.0835265683620477,-13.5169045823054,0.0824317919394229));
#25999=CARTESIAN_POINT('Origin',(45.7901549780056,-13.5169045823054,31.5572011510148));
#26000=CARTESIAN_POINT('Origin',(-4.3055892018327,-12.8919045823054,13.3928441877896));
#26001=CARTESIAN_POINT('Origin',(40.0376426042469,-12.8919045823054,28.0150491378139));
#26002=CARTESIAN_POINT('Origin',(0.0835265683620477,-5.8874628440639,0.0824317919394229));
#26003=CARTESIAN_POINT('Ctrl Pts',(-48.3539734316379,-14.9741386829693,
-30.3741755844114));
#26004=CARTESIAN_POINT('Ctrl Pts',(-48.3539734316379,-14.8357920829905,
-30.4481591048434));
#26005=CARTESIAN_POINT('Ctrl Pts',(-48.2281585089893,-14.7531448966919,
-30.4923562863941));
#26006=CARTESIAN_POINT('Ctrl Pts',(-48.3539734316379,-13.8793029116966,
-28.3268709202925));
#26007=CARTESIAN_POINT('Ctrl Pts',(-48.353973431638,-13.7458678866791,-28.4041169753078));
#26008=CARTESIAN_POINT('Ctrl Pts',(-48.2317488064611,-13.6583075326763,
-28.439377201631));
#26009=CARTESIAN_POINT('Ctrl Pts',(-48.3539734316379,-12.8434482903031,
-26.2438196848709));
#26010=CARTESIAN_POINT('Ctrl Pts',(-48.3539734316379,-12.7103751542451,
-26.3167263455105));
#26011=CARTESIAN_POINT('Ctrl Pts',(-48.2353559924772,-12.6224528665257,
-26.3500637611613));
#26012=CARTESIAN_POINT('Ctrl Pts',(-48.3539734316379,-11.4077451872907,
-23.0475925985065));
#26013=CARTESIAN_POINT('Ctrl Pts',(-48.353973431638,-11.2735898053161,-23.1079173838282));
#26014=CARTESIAN_POINT('Ctrl Pts',(-48.2406193805204,-11.1867499400323,
-23.143370974004));
#26015=CARTESIAN_POINT('Ctrl Pts',(-48.3539734316379,-10.9489604127269,
-21.9701832380143));
#26016=CARTESIAN_POINT('Ctrl Pts',(-48.353973431638,-10.8151504288127,-22.0280335561356));
#26017=CARTESIAN_POINT('Ctrl Pts',(-48.2423483273574,-10.7279650272951,
-22.0622935359395));
#26018=CARTESIAN_POINT('Ctrl Pts',(-48.3539734316379,-10.0773547210536,
-19.7874828213299));
#26019=CARTESIAN_POINT('Ctrl Pts',(-48.353973431638,-9.94441815656983,-19.8402912091848));
#26020=CARTESIAN_POINT('Ctrl Pts',(-48.2457130710704,-9.85635900888278,
-19.871869217566));
#26021=CARTESIAN_POINT('Ctrl Pts',(-48.3539734316379,-9.66512413195427,
-18.6831101240159));
#26022=CARTESIAN_POINT('Ctrl Pts',(-48.353973431638,-9.53246556459247,-18.7331822824075));
#26023=CARTESIAN_POINT('Ctrl Pts',(-48.2473467934865,-9.44412830209105,
-18.7634428488815));
#26024=CARTESIAN_POINT('Ctrl Pts',(-48.3539734316379,-7.7573342368428,-13.1446350442278));
#26025=CARTESIAN_POINT('Ctrl Pts',(-48.353973431638,-7.63508483858545,-13.2059559526897));
#26026=CARTESIAN_POINT('Ctrl Pts',(-48.2550691977422,-7.53633525781305,
-13.2039172467247));
#26027=CARTESIAN_POINT('Ctrl Pts',(-48.3539734316379,-6.70462823796961,
-8.61608142151409));
#26028=CARTESIAN_POINT('Ctrl Pts',(-48.353973431638,-6.57519149764306,-8.64715660898112));
#26029=CARTESIAN_POINT('Ctrl Pts',(-48.259869139976,-6.48363668557058,-8.65580178786413));
#26030=CARTESIAN_POINT('Ctrl Pts',(-48.3539734316379,-6.31501530004509,
-3.95028918791133));
#26031=CARTESIAN_POINT('Ctrl Pts',(-48.353973431638,-6.18536424665269,-3.96111558677735));
#26032=CARTESIAN_POINT('Ctrl Pts',(-48.2616461026061,-6.09401826675112,
-3.9687433536743));
#26033=CARTESIAN_POINT('Ctrl Pts',(-48.2284487824325,-14.6753754514262,
-30.3462212704574));
#26034=CARTESIAN_POINT('Ctrl Pts',(-48.2380517942861,-14.6690745001747,
-30.3191514097119));
#26035=CARTESIAN_POINT('Ctrl Pts',(-48.2467246024825,-14.6627081744215,
-30.2917846168048));
#26036=CARTESIAN_POINT('Ctrl Pts',(-48.2546340278731,-14.656301600065,-30.26422929553));
#26037=CARTESIAN_POINT('Ctrl Pts',(-48.2630249404881,-14.6495050247221,
-30.2349965407501));
#26038=CARTESIAN_POINT('Ctrl Pts',(-48.2705565129546,-14.6426630446869,
-30.2055511526331));
#26039=CARTESIAN_POINT('Ctrl Pts',(-48.2773911339934,-14.6357952456547,
-30.1759776611132));
#26040=CARTESIAN_POINT('Ctrl Pts',(-48.2850046107278,-14.6281448100487,
-30.1430340511656));
#26041=CARTESIAN_POINT('Ctrl Pts',(-48.2917532457326,-14.6204622387226,
-30.1099310736677));
#26042=CARTESIAN_POINT('Ctrl Pts',(-48.2978182296841,-14.6127635931359,
-30.0767379272495));
#26043=CARTESIAN_POINT('Ctrl Pts',(-48.3045464712037,-14.6042230351895,
-30.0399148280156));
#26044=CARTESIAN_POINT('Ctrl Pts',(-48.3104330917546,-14.5956624333502,
-30.0029796599166));
#26045=CARTESIAN_POINT('Ctrl Pts',(-48.3156769463159,-14.5870937621613,
-29.9659834425651));
#26046=CARTESIAN_POINT('Ctrl Pts',(-48.3196586203822,-14.5805875451302,
-29.9378921068009));
#26047=CARTESIAN_POINT('Ctrl Pts',(-48.3232685595429,-14.5740764123797,
-29.9097644296832));
#26048=CARTESIAN_POINT('Ctrl Pts',(-48.3265802528816,-14.567564046071,-29.8816156801631));
#26049=CARTESIAN_POINT('Ctrl Pts',(-48.3269187812443,-14.5668983380848,
-29.8787382548971));
#26050=CARTESIAN_POINT('Ctrl Pts',(-48.3272539901496,-14.5662323997339,
-29.8758596817254));
#26051=CARTESIAN_POINT('Ctrl Pts',(-48.3275859006452,-14.5655662082161,
-29.8729798623161));
#26052=CARTESIAN_POINT('Ctrl Pts',(-48.3385590056696,-14.5435416275269,
-29.7777717828841));
#26053=CARTESIAN_POINT('Ctrl Pts',(-48.3458113929029,-14.521489722448,-29.6822597427751));
#26054=CARTESIAN_POINT('Ctrl Pts',(-48.349892235323,-14.4994225808413,-29.5864906154957));
#26055=CARTESIAN_POINT('Ctrl Pts',(-48.3526660001049,-14.4844234571493,
-29.5213959597605));
#26056=CARTESIAN_POINT('Ctrl Pts',(-48.3539733066297,-14.4694172066211,
-29.4561822481182));
#26057=CARTESIAN_POINT('Ctrl Pts',(-48.353973431629,-14.454406734056,-29.3908610634297));
#26058=CARTESIAN_POINT('Ctrl Pts',(-48.2281934536869,-14.7531486984911,
30.6571717707886));
#26059=CARTESIAN_POINT('Ctrl Pts',(-48.3539734316379,-14.8357969973015,
30.6129740313388));
#26060=CARTESIAN_POINT('Ctrl Pts',(-48.3539734316379,-14.9741195676119,
30.5390034232244));
#26061=CARTESIAN_POINT('Ctrl Pts',(-48.2317820061024,-13.6585793127022,
28.6046931834481));
#26062=CARTESIAN_POINT('Ctrl Pts',(-48.353973431646,-13.7461362596114,28.5694255116643));
#26063=CARTESIAN_POINT('Ctrl Pts',(-48.3539734316379,-13.8795503180259,
28.4921954301588));
#26064=CARTESIAN_POINT('Ctrl Pts',(-48.2353869404035,-12.6231097579324,
26.5161580434808));
#26065=CARTESIAN_POINT('Ctrl Pts',(-48.353973431638,-12.711026527187,26.4828083346013));
#26066=CARTESIAN_POINT('Ctrl Pts',(-48.3539734316379,-12.844080626948,26.4099196549775));
#26067=CARTESIAN_POINT('Ctrl Pts',(-48.2406462654066,-11.1881005852611,
23.3112728899427));
#26068=CARTESIAN_POINT('Ctrl Pts',(-48.353973431638,-11.2749369501005,23.2758135504267));
#26069=CARTESIAN_POINT('Ctrl Pts',(-48.3539734316379,-11.4090714544345,
23.2154943062685));
#26070=CARTESIAN_POINT('Ctrl Pts',(-48.24237374671,-10.7295656511252,22.2309062509719));
#26071=CARTESIAN_POINT('Ctrl Pts',(-48.353973431638,-10.816746996712,22.1966391076998));
#26072=CARTESIAN_POINT('Ctrl Pts',(-48.3539734316379,-10.9505365201866,
22.1387927374662));
#26073=CARTESIAN_POINT('Ctrl Pts',(-48.2457354335294,-9.85847188921457,
20.0421726047875));
#26074=CARTESIAN_POINT('Ctrl Pts',(-48.3539734316379,-9.94652588376064,
20.0105850435767));
#26075=CARTESIAN_POINT('Ctrl Pts',(-48.3539734316379,-10.0794427583948,
19.9577755041285));
#26076=CARTESIAN_POINT('Ctrl Pts',(-48.2473707001107,-9.44570717935305,
18.932638230004));
#26077=CARTESIAN_POINT('Ctrl Pts',(-48.3539734316379,-9.53404162556803,
18.9023748976264));
#26078=CARTESIAN_POINT('Ctrl Pts',(-48.3539734316379,-9.66667804843004,
18.852297914388));
#26079=CARTESIAN_POINT('Ctrl Pts',(-48.2550987080888,-7.53595817693284,
13.3683509755226));
#26080=CARTESIAN_POINT('Ctrl Pts',(-48.353973431638,-7.63471881015775,13.3704269700606));
#26081=CARTESIAN_POINT('Ctrl Pts',(-48.3539734316379,-7.75692904622887,
13.3090686823533));
#26082=CARTESIAN_POINT('Ctrl Pts',(-48.2598967761517,-6.48350292013321,
8.81865536350909));
#26083=CARTESIAN_POINT('Ctrl Pts',(-48.3539734316379,-6.57505277910396,
8.81000220468341));
#26084=CARTESIAN_POINT('Ctrl Pts',(-48.3539734316379,-6.70446830386371,
8.77894670225279));
#26085=CARTESIAN_POINT('Ctrl Pts',(-48.2616725171888,-6.0940504675403,4.13367737178086));
#26086=CARTESIAN_POINT('Ctrl Pts',(-48.3539734316379,-6.18539206100946,
4.12604983539374));
#26087=CARTESIAN_POINT('Ctrl Pts',(-48.3539734316379,-6.3150213366611,4.11522506237069));
#26088=CARTESIAN_POINT('Ctrl Pts',(-48.3539734316292,-14.4544067125518,
29.5557245537287));
#26089=CARTESIAN_POINT('Ctrl Pts',(-48.3539732674099,-14.474282601141,29.6422186055862));
#26090=CARTESIAN_POINT('Ctrl Pts',(-48.3516784774865,-14.4941426280635,
29.7284873150456));
#26091=CARTESIAN_POINT('Ctrl Pts',(-48.3467303041063,-14.5139794995535,
29.8145018353666));
#26092=CARTESIAN_POINT('Ctrl Pts',(-48.3424398274083,-14.5311797123081,
29.8890835581078));
#26093=CARTESIAN_POINT('Ctrl Pts',(-48.3361540294485,-14.5483624868197,
29.9634740170122));
#26094=CARTESIAN_POINT('Ctrl Pts',(-48.3276091486579,-14.5655203189316,
30.0376437438476));
#26095=CARTESIAN_POINT('Ctrl Pts',(-48.3272263411088,-14.5662889835649,
30.0409665206127));
#26096=CARTESIAN_POINT('Ctrl Pts',(-48.3268391006314,-14.5670573738945,
30.044287911485));
#26097=CARTESIAN_POINT('Ctrl Pts',(-48.3264473967985,-14.5678255143183,
30.0476080213421));
#26098=CARTESIAN_POINT('Ctrl Pts',(-48.3217619067946,-14.5770138703539,
30.0873225715689));
#26099=CARTESIAN_POINT('Ctrl Pts',(-48.316495168063,-14.5862107044412,30.1270431157074));
#26100=CARTESIAN_POINT('Ctrl Pts',(-48.3104154469146,-14.5953989044386,
30.1666965637756));
#26101=CARTESIAN_POINT('Ctrl Pts',(-48.3049006360659,-14.6037333631727,
30.2026655268679));
#26102=CARTESIAN_POINT('Ctrl Pts',(-48.2987173294784,-14.6120609299868,
30.2385801726924));
#26103=CARTESIAN_POINT('Ctrl Pts',(-48.291662149791,-14.6203642532736,30.2743658179158));
#26104=CARTESIAN_POINT('Ctrl Pts',(-48.2850866379861,-14.6281030498333,
30.3077184670388));
#26105=CARTESIAN_POINT('Ctrl Pts',(-48.2777540899714,-14.6358209223575,
30.3409596295151));
#26106=CARTESIAN_POINT('Ctrl Pts',(-48.2694670548976,-14.6434973280408,
30.3740007357241));
#26107=CARTESIAN_POINT('Ctrl Pts',(-48.2618294825168,-14.6505721266279,
30.4044523795226));
#26108=CARTESIAN_POINT('Ctrl Pts',(-48.2533812725397,-14.6576117669145,
30.4347343630163));
#26109=CARTESIAN_POINT('Ctrl Pts',(-48.2439363682233,-14.6645931621416,
30.4647471875625));
#26110=CARTESIAN_POINT('Ctrl Pts',(-48.2390509274011,-14.6682043361774,
30.480271524635));
#26111=CARTESIAN_POINT('Ctrl Pts',(-48.2338982763733,-14.6717998028497,
30.4957233152332));
#26112=CARTESIAN_POINT('Ctrl Pts',(-48.2284487824329,-14.6753754514261,
30.5110848543365));
#26113=CARTESIAN_POINT('Ctrl Pts',(-48.2616069689928,-6.10843371319294,
4.30318191980438));
#26114=CARTESIAN_POINT('Ctrl Pts',(-48.2619184079005,-6.10843410331518,
4.29961926247631));
#26115=CARTESIAN_POINT('Ctrl Pts',(-48.2763274441054,-6.12223873054911,
4.29756562167191));
#26116=CARTESIAN_POINT('Ctrl Pts',(-48.3054382973494,-6.16064820739694,
4.29414588360541));
#26117=CARTESIAN_POINT('Ctrl Pts',(-48.319962915512,-6.1854892637356,4.29278763374148));
#26118=CARTESIAN_POINT('Ctrl Pts',(-48.3299590819564,-6.2094696845087,4.291470939112));
#26119=CARTESIAN_POINT('Origin',(-48.6664734316379,-14.4544045823054,-44.2925682080606));
#26120=CARTESIAN_POINT('Origin',(-48.6664734316379,-14.4544045823054,29.555715283519));
#26121=CARTESIAN_POINT('Origin',(-48.6664734316379,-14.4544045823054,-29.3908516996402));
#26122=CARTESIAN_POINT('Ctrl Pts',(-48.666473431638,-14.7669045823054,-29.3908516996402));
#26123=CARTESIAN_POINT('Ctrl Pts',(-48.353973431638,-14.7669045823054,-29.3908516996402));
#26124=CARTESIAN_POINT('Ctrl Pts',(-48.353973431638,-14.4544045823054,-29.3908516996402));
#26125=CARTESIAN_POINT('Ctrl Pts',(-48.6664734300675,-14.7669045823054,
-29.5764473463203));
#26126=CARTESIAN_POINT('Ctrl Pts',(-48.3898840300057,-14.7669045823054,
-29.5471242124449));
#26127=CARTESIAN_POINT('Ctrl Pts',(-48.353973431638,-14.4924835039823,-29.5565600468581));
#26128=CARTESIAN_POINT('Ctrl Pts',(-48.6496385395544,-14.7669045823054,
-29.760152449079));
#26129=CARTESIAN_POINT('Ctrl Pts',(-48.4083048654681,-14.7669045823054,
-29.7192585224243));
#26130=CARTESIAN_POINT('Ctrl Pts',(-48.345555980154,-14.5302479546778,-29.7203266919373));
#26131=CARTESIAN_POINT('Ctrl Pts',(-48.5737303814916,-14.7669045823054,
-30.1225239035316));
#26132=CARTESIAN_POINT('Ctrl Pts',(-48.3969357334759,-14.7669045823054,
-30.0607578147132));
#26133=CARTESIAN_POINT('Ctrl Pts',(-48.307601912007,-14.6048732634489,-30.0429041209019));
#26134=CARTESIAN_POINT('Ctrl Pts',(-48.5155778976522,-14.7669045823054,
-30.3049694134568));
#26135=CARTESIAN_POINT('Ctrl Pts',(-48.3721493817961,-14.7669045823059,
-30.2369968366664));
#26136=CARTESIAN_POINT('Ctrl Pts',(-48.2786791401611,-14.6424170542665,
-30.2046271131434));
#26137=CARTESIAN_POINT('Ctrl Pts',(-48.415424133227,-14.7669045823054,-30.4639852003989));
#26138=CARTESIAN_POINT('Ctrl Pts',(-48.305896508561,-14.7669045823054,-30.3950006873975));
#26139=CARTESIAN_POINT('Ctrl Pts',(-48.2284487824325,-14.6753754514262,
-30.3462212704574));
#26140=CARTESIAN_POINT('Origin',(-48.415424133227,-14.4544045823054,-30.4639852003989));
#26141=CARTESIAN_POINT('Origin',(-45.6231018412815,-13.5169045823054,-31.3923375671359));
#26142=CARTESIAN_POINT('Origin',(-45.6231018412815,-13.5169045823054,-31.3923375671359));
#26143=CARTESIAN_POINT('Origin',(-45.6231018412815,-13.5169045823054,-31.3923375671359));
#26144=CARTESIAN_POINT('Origin',(-39.8705894675228,-12.8919045823054,-27.8501855539351));
#26145=CARTESIAN_POINT('Origin',(-39.8705894675228,-12.8919045823054,-27.8501855539351));
#26146=CARTESIAN_POINT('Ctrl Pts',(-34.2908051207842,-13.5169045823054,
-34.2861336374548));
#26147=CARTESIAN_POINT('Ctrl Pts',(-34.2908051207842,-13.2044045823054,
-34.2861336374548));
#26148=CARTESIAN_POINT('Ctrl Pts',(-34.1929414312581,-13.2044045823054,
-34.5829146143929));
#26149=CARTESIAN_POINT('Ctrl Pts',(-34.2074765603999,-13.5169045582439,
-34.2586559990757));
#26150=CARTESIAN_POINT('Ctrl Pts',(-34.2390780768993,-13.186119131637,-34.2690766164313));
#26151=CARTESIAN_POINT('Ctrl Pts',(-34.1370790312896,-13.2044045823054,
-34.583214693643));
#26152=CARTESIAN_POINT('Ctrl Pts',(-34.1263179792903,-13.5027466839947,
-34.2318939125496));
#26153=CARTESIAN_POINT('Ctrl Pts',(-34.1959174748504,-13.1578432798924,
-34.2548443842914));
#26154=CARTESIAN_POINT('Ctrl Pts',(-34.0825856046419,-13.1973256316195,
-34.5835570770033));
#26155=CARTESIAN_POINT('Ctrl Pts',(-33.9688208616094,-13.4449866817214,
-34.1799591518213));
#26156=CARTESIAN_POINT('Ctrl Pts',(-34.1280308564926,-13.0892356355759,
-34.2324587347441));
#26157=CARTESIAN_POINT('Ctrl Pts',(-33.9766844888021,-13.1684456335484,
-34.5843089536435));
#26158=CARTESIAN_POINT('Ctrl Pts',(-33.8970079820796,-13.4031153721668,
-34.1562788155047));
#26159=CARTESIAN_POINT('Ctrl Pts',(-34.106817243136,-13.0503322093645,-34.2254635341332));
#26160=CARTESIAN_POINT('Ctrl Pts',(-33.92831997416,-13.147509967376,-34.5846967331698));
#26161=CARTESIAN_POINT('Ctrl Pts',(-33.7690007142555,-13.2902331116007,
-34.1140683489017));
#26162=CARTESIAN_POINT('Ctrl Pts',(-34.0865509444696,-12.9767617731722,
-34.2187807110593));
#26163=CARTESIAN_POINT('Ctrl Pts',(-33.8420172589373,-13.0910688568131,
-34.585441064553));
#26164=CARTESIAN_POINT('Ctrl Pts',(-33.7168717646145,-13.2224528271011,
-34.0968787992358));
#26165=CARTESIAN_POINT('Ctrl Pts',(-34.0899725583413,-12.9460615526393,
-34.2199089901059));
#26166=CARTESIAN_POINT('Ctrl Pts',(-33.8068205483247,-13.0571787063092,
-34.5857736886607));
#26167=CARTESIAN_POINT('Ctrl Pts',(-33.6428336845022,-13.0654169357611,
-34.0724647018095));
#26168=CARTESIAN_POINT('Ctrl Pts',(-34.1033496871212,-12.9052920386068,
-34.2243201056398));
#26169=CARTESIAN_POINT('Ctrl Pts',(-33.7568076539782,-12.9786607574272,
-34.5862594970788));
#26170=CARTESIAN_POINT('Ctrl Pts',(-33.6230658166974,-12.9802875861308,
-34.0659462365851));
#26171=CARTESIAN_POINT('Ctrl Pts',(-34.1117050038364,-12.8977806170664,
-34.2270752758985));
#26172=CARTESIAN_POINT('Ctrl Pts',(-33.7434406365763,-12.9360960854268,
-34.5863970888581));
#26173=CARTESIAN_POINT('Ctrl Pts',(-33.6230658340261,-12.8919045823054,
-34.0659462422992));
#26174=CARTESIAN_POINT('Ctrl Pts',(-34.1117049987155,-12.8919045823054,
-34.2270752742097));
#26175=CARTESIAN_POINT('Ctrl Pts',(-33.7434406426353,-12.8919045823054,
-34.5863970829463));
#26176=CARTESIAN_POINT('Origin',(-33.5252021444999,-12.8919045823054,-34.3627272192373));
#26177=CARTESIAN_POINT('Origin',(0.0835265683620477,-11.3294045823054,0.0824317919394229));
#26178=CARTESIAN_POINT('Origin',(6.83612114566777,-11.3294045823054,-20.3954556167886));
#26179=CARTESIAN_POINT('Origin',(20.56141397709,-11.3294045823054,6.83502636924522));
#26180=CARTESIAN_POINT('Origin',(20.56141397709,-11.3294045823054,6.83502636924522));
#26181=CARTESIAN_POINT('Origin',(10.2095634989472,-14.4544045823054,19.8244816432194));
#26182=CARTESIAN_POINT('Origin',(10.2095634989472,-14.4544045823054,19.8244816432194));
#26183=CARTESIAN_POINT('Origin',(45.7901549780056,-13.5169045823054,31.5572011510148));
#26184=CARTESIAN_POINT('Origin',(45.7901549780056,-13.5169045823054,31.5572011510148));
#26185=CARTESIAN_POINT('Origin',(40.0376426042469,-12.8919045823054,28.0150491378139));
#26186=CARTESIAN_POINT('Origin',(40.0376426042469,-12.8919045823054,28.0150491378139));
#26187=CARTESIAN_POINT('Ctrl Pts',(-48.353987706665,-6.00666333723547,0.0824317919588709));
#26188=CARTESIAN_POINT('Ctrl Pts',(-48.3539878230387,-6.01200137934915,
0.433477096833169));
#26189=CARTESIAN_POINT('Ctrl Pts',(-48.3525306312191,-6.02125184123593,
0.784346425692766));
#26190=CARTESIAN_POINT('Ctrl Pts',(-48.3492030226928,-6.04818290219923,
1.48575918442931));
#26191=CARTESIAN_POINT('Ctrl Pts',(-48.3473326059861,-6.06586350127576,
1.83630261430625));
#26192=CARTESIAN_POINT('Ctrl Pts',(-48.3448536057857,-6.13245845075532,
2.88748313503321));
#26193=CARTESIAN_POINT('Ctrl Pts',(-48.3401597427993,-6.17306838545285,
3.5897554902018));
#26194=CARTESIAN_POINT('Ctrl Pts',(-48.3299590819564,-6.20946968450872,
4.29147093911199));
#26195=CARTESIAN_POINT('Ctrl Pts',(-48.3539875902919,-6.00132529512177,
0.433477096832907));
#26196=CARTESIAN_POINT('Ctrl Pts',(-48.3530459746152,-6.00879525432317,
0.706493516793873));
#26197=CARTESIAN_POINT('Ctrl Pts',(-48.3513305951691,-6.01828947675677,
0.997236185068297));
#26198=CARTESIAN_POINT('Ctrl Pts',(-48.3474462842671,-6.04432658407327,
1.61112122473693));
#26199=CARTESIAN_POINT('Ctrl Pts',(-48.3452802018324,-6.06089216512325,
1.9342619765643));
#26200=CARTESIAN_POINT('Ctrl Pts',(-48.341640774377,-6.12571278894257,2.9477088419804));
#26201=CARTESIAN_POINT('Ctrl Pts',(-48.3361613302943,-6.16367997403222,
3.62572661437067));
#26202=CARTESIAN_POINT('Ctrl Pts',(-48.3249609987342,-6.19747947412216,
4.29212928642674));
#26203=CARTESIAN_POINT('Ctrl Pts',(-48.3525301621497,-5.99973567328063,
0.784574339470114));
#26204=CARTESIAN_POINT('Ctrl Pts',(-48.3509583174057,-6.00835114797897,
0.9975813791029));
#26205=CARTESIAN_POINT('Ctrl Pts',(-48.34894252132,-6.01789996842715,1.24226674486999));
#26206=CARTESIAN_POINT('Ctrl Pts',(-48.344356416097,-6.04289085428958,1.78530549517593));
#26207=CARTESIAN_POINT('Ctrl Pts',(-48.3417903804913,-6.05836696395447,
2.08365645036453));
#26208=CARTESIAN_POINT('Ctrl Pts',(-48.3366078653997,-6.11975101512505,
3.0446847621152));
#26209=CARTESIAN_POINT('Ctrl Pts',(-48.3302694595669,-6.15479195325803,
3.68769530697585));
#26210=CARTESIAN_POINT('Ctrl Pts',(-48.3188308025825,-6.18527410484421,
4.29279802255009));
#26211=CARTESIAN_POINT('Ctrl Pts',(-48.3427993418055,-5.9982057973697,1.48689990262106));
#26212=CARTESIAN_POINT('Ctrl Pts',(-48.3410826227124,-6.0082917350609,1.61268346924727));
#26213=CARTESIAN_POINT('Ctrl Pts',(-48.3390430002227,-6.01814206512131,
1.78661204317002));
#26214=CARTESIAN_POINT('Ctrl Pts',(-48.3339923325764,-6.04173521008623,
2.20924933968616));
#26215=CARTESIAN_POINT('Ctrl Pts',(-48.3309866293343,-6.05552058030403,
2.45795502559173));
#26216=CARTESIAN_POINT('Ctrl Pts',(-48.3235830578663,-6.10935599904105,
3.28398546777139));
#26217=CARTESIAN_POINT('Ctrl Pts',(-48.316046725529,-6.13882811018934,3.83329116275982));
#26218=CARTESIAN_POINT('Ctrl Pts',(-48.3054305681491,-6.16205725113851,
4.29423379157955));
#26219=CARTESIAN_POINT('Ctrl Pts',(-48.3345259496034,-5.9982655432999,1.8381282231348));
#26220=CARTESIAN_POINT('Ctrl Pts',(-48.3332754509115,-6.00864450579851,
1.93670273202018));
#26221=CARTESIAN_POINT('Ctrl Pts',(-48.3315028514988,-6.01872578611233,
2.08593433407471));
#26222=CARTESIAN_POINT('Ctrl Pts',(-48.3266822403813,-6.04195544062561,
2.45901835426532));
#26223=CARTESIAN_POINT('Ctrl Pts',(-48.3236392144634,-6.05514353311748,
2.68286793815945));
#26224=CARTESIAN_POINT('Ctrl Pts',(-48.3155720249932,-6.10489083408607,
3.42631528823035));
#26225=CARTESIAN_POINT('Ctrl Pts',(-48.3077158622186,-6.13175228789483,
3.9169183259386));
#26226=CARTESIAN_POINT('Ctrl Pts',(-48.2981605298675,-6.15104576671075,
4.29500082448565));
#26227=CARTESIAN_POINT('Ctrl Pts',(-48.293629816125,-5.99214762358688,2.89205060501609));
#26228=CARTESIAN_POINT('Ctrl Pts',(-48.2931970947763,-6.0038166575676,2.9533318756659));
#26229=CARTESIAN_POINT('Ctrl Pts',(-48.2925867091264,-6.01569196513301,
3.05034122028972));
#26230=CARTESIAN_POINT('Ctrl Pts',(-48.2905861997381,-6.040339618854,3.28859696686724));
#26231=CARTESIAN_POINT('Ctrl Pts',(-48.2891989250207,-6.05313466117666,
3.4298417492541));
#26232=CARTESIAN_POINT('Ctrl Pts',(-48.2851290640768,-6.09364276617915,
3.87910729199725));
#26233=CARTESIAN_POINT('Ctrl Pts',(-48.2810866692063,-6.11446024451104,
4.15478252188684));
#26234=CARTESIAN_POINT('Ctrl Pts',(-48.2763272274218,-6.12223844465217,
4.29756564712637));
#26235=CARTESIAN_POINT('Ctrl Pts',(-48.2504292399881,-5.99475664078892,
3.59330337787141));
#26236=CARTESIAN_POINT('Ctrl Pts',(-48.2516773068009,-6.00697011627484,
3.63027912062932));
#26237=CARTESIAN_POINT('Ctrl Pts',(-48.253021728415,-6.02014444454773,3.69245653521261));
#26238=CARTESIAN_POINT('Ctrl Pts',(-48.2556497470798,-6.04594588203951,
3.83761867006235));
#26239=CARTESIAN_POINT('Ctrl Pts',(-48.2569333441305,-6.05857299125839,
3.92060339032879));
#26240=CARTESIAN_POINT('Ctrl Pts',(-48.260312597188,-6.09193010339209,4.15637445270144));
#26241=CARTESIAN_POINT('Ctrl Pts',(-48.2619367151003,-6.10813589078396,
4.29597769638096));
#26242=CARTESIAN_POINT('Ctrl Pts',(-48.2619179788887,-6.1084336923001,4.29961932362109));
#26243=CARTESIAN_POINT('Ctrl Pts',(-48.1943732865555,-6.00705144710499,
4.29441317095732));
#26244=CARTESIAN_POINT('Ctrl Pts',(-48.1993391601324,-6.01900581052063,
4.29446585817732));
#26245=CARTESIAN_POINT('Ctrl Pts',(-48.2060243727241,-6.03128117156189,
4.29459893941721));
#26246=CARTESIAN_POINT('Ctrl Pts',(-48.2204933169654,-6.05467770199134,
4.29515956957315));
#26247=CARTESIAN_POINT('Ctrl Pts',(-48.2282770486149,-6.06579887137953,
4.2955871184892));
#26248=CARTESIAN_POINT('Ctrl Pts',(-48.2497657836928,-6.09473681170807,
4.29751198620615));
#26249=CARTESIAN_POINT('Ctrl Pts',(-48.2616083272502,-6.10812801481236,
4.29965152597587));
#26250=CARTESIAN_POINT('Ctrl Pts',(-48.2616069550931,-6.10843371318469,
4.30318207891618));
#26251=CARTESIAN_POINT('Ctrl Pts',(-48.2616069551289,-6.10843370450312,
4.30318197869235));
#26252=CARTESIAN_POINT('Ctrl Pts',(-48.2616070232649,-6.10841554618156,
4.30297243702759));
#26253=CARTESIAN_POINT('Ctrl Pts',(-48.261568504835,-6.10835892241089,4.30281626830296));
#26254=CARTESIAN_POINT('Ctrl Pts',(-48.2615317413218,-6.10830758140196,
4.30270005783412));
#26255=CARTESIAN_POINT('Ctrl Pts',(-48.2614948949699,-6.108256124707,4.30258358550975));
#26256=CARTESIAN_POINT('Ctrl Pts',(-48.2614587515144,-6.10820886405691,
4.30250736538357));
#26257=CARTESIAN_POINT('Ctrl Pts',(-48.2614364198362,-6.10817971723294,
4.3024610753784));
#26258=CARTESIAN_POINT('Ctrl Pts',(-48.261391803134,-6.10812148447717,4.30236859207495));
#26259=CARTESIAN_POINT('Ctrl Pts',(-48.2613611308546,-6.10808254421549,
4.30231835467004));
#26260=CARTESIAN_POINT('Ctrl Pts',(-48.2613314964975,-6.10804496697612,
4.30227052055935));
#26261=CARTESIAN_POINT('Ctrl Pts',(-48.2612722277834,-6.10796981249738,
4.30217485233798));
#26262=CARTESIAN_POINT('Ctrl Pts',(-48.2612207139529,-6.10790555145939,
4.30210514206976));
#26263=CARTESIAN_POINT('Ctrl Pts',(-48.2611666188386,-6.10783843371047,
4.30203697537195));
#26264=CARTESIAN_POINT('Ctrl Pts',(-48.2609812244811,-6.10760840828066,
4.30180335499264));
#26265=CARTESIAN_POINT('Ctrl Pts',(-48.2607712975097,-6.10735331838435,
4.30161270338785));
#26266=CARTESIAN_POINT('Ctrl Pts',(-48.2605614051161,-6.10709948505642,
4.30144691969731));
#26267=CARTESIAN_POINT('Ctrl Pts',(-48.2602786597362,-6.10675754698275,
4.30122359301185));
#26268=CARTESIAN_POINT('Ctrl Pts',(-48.2599937148647,-6.10641533300863,
4.30104387204264));
#26269=CARTESIAN_POINT('Ctrl Pts',(-48.2596984045309,-6.10606098282255,
4.30087738558224));
#26270=CARTESIAN_POINT('Ctrl Pts',(-48.2592951604377,-6.1055771202446,4.30065004954269));
#26271=CARTESIAN_POINT('Ctrl Pts',(-48.2588878641398,-6.10508918081615,
4.30045936658896));
#26272=CARTESIAN_POINT('Ctrl Pts',(-48.2584803602671,-6.10460034109874,
4.30028708750468));
#26273=CARTESIAN_POINT('Ctrl Pts',(-48.2577834928373,-6.10376438222755,
4.29999247513237));
#26274=CARTESIAN_POINT('Ctrl Pts',(-48.2570827132334,-6.10292193531566,
4.2997513336239));
#26275=CARTESIAN_POINT('Ctrl Pts',(-48.2563837106908,-6.10207801393888,
4.29953565913165));
#26276=CARTESIAN_POINT('Ctrl Pts',(-48.2552039588319,-6.10065367317838,
4.29917165132385));
#26277=CARTESIAN_POINT('Ctrl Pts',(-48.254026426545,-6.09922194596883,4.29888122427205));
#26278=CARTESIAN_POINT('Ctrl Pts',(-48.2528540013546,-6.09778441771827,
4.29862403126663));
#26279=CARTESIAN_POINT('Ctrl Pts',(-48.2510293554768,-6.09554719182277,
4.29822376167079));
#26280=CARTESIAN_POINT('Ctrl Pts',(-48.2492165852536,-6.09329562622209,
4.29790736627066));
#26281=CARTESIAN_POINT('Ctrl Pts',(-48.2474182713127,-6.09103086693172,
4.2976305747359));
#26282=CARTESIAN_POINT('Ctrl Pts',(-48.2447139428525,-6.08762509174139,
4.29721433193871));
#26283=CARTESIAN_POINT('Ctrl Pts',(-48.2420414322396,-6.08418870246316,
4.29689093118225));
#26284=CARTESIAN_POINT('Ctrl Pts',(-48.239407025734,-6.08072383167611,4.29661384152446));
#26285=CARTESIAN_POINT('Ctrl Pts',(-48.2380751607036,-6.07897211255965,
4.2964737545543));
#26286=CARTESIAN_POINT('Ctrl Pts',(-48.2367524918963,-6.07721238041329,
4.29634631195034));
#26287=CARTESIAN_POINT('Ctrl Pts',(-48.2354399603075,-6.07544485148905,
4.29622874106152));
#26288=CARTESIAN_POINT('Ctrl Pts',(-48.2312254371352,-6.06976933733557,
4.29585122234916));
#26289=CARTESIAN_POINT('Ctrl Pts',(-48.22711583857,-6.06401604656339,4.29557214159525));
#26290=CARTESIAN_POINT('Ctrl Pts',(-48.2231376376079,-6.05817108586382,
4.29534669590986));
#26291=CARTESIAN_POINT('Ctrl Pts',(-48.2197392166315,-6.05317796529557,
4.29515410650737));
#26292=CARTESIAN_POINT('Ctrl Pts',(-48.2164370013549,-6.04811857023788,
4.29500239895895));
#26293=CARTESIAN_POINT('Ctrl Pts',(-48.2132588448447,-6.04297943677661,
4.29487925449518));
#26294=CARTESIAN_POINT('Ctrl Pts',(-48.2098408541154,-6.03745248727896,
4.29474681714221));
#26295=CARTESIAN_POINT('Ctrl Pts',(-48.206564810075,-6.03183339812509,4.29464768913944));
#26296=CARTESIAN_POINT('Ctrl Pts',(-48.2034906784034,-6.02609676302333,
4.29457335819765));
#26297=CARTESIAN_POINT('Ctrl Pts',(-48.2008503025217,-6.02116955931759,
4.29450951525046));
#26298=CARTESIAN_POINT('Ctrl Pts',(-48.1983577537265,-6.01615482893866,
4.29446412495472));
#26299=CARTESIAN_POINT('Ctrl Pts',(-48.1960855539946,-6.01103540679842,
4.29443373440248));
#26300=CARTESIAN_POINT('Ctrl Pts',(-48.195712281463,-6.01019439813361,4.29442874190195));
#26301=CARTESIAN_POINT('Ctrl Pts',(-48.1953450670276,-6.00935058232647,
4.29442415648971));
#26302=CARTESIAN_POINT('Ctrl Pts',(-48.1949843830272,-6.00850392013414,
4.2944199650574));
#26303=CARTESIAN_POINT('Ctrl Pts',(-48.1947785238618,-6.00802069056991,
4.29441757281168));
#26304=CARTESIAN_POINT('Ctrl Pts',(-48.1945747929681,-6.00753653413945,
4.29441530891201));
#26305=CARTESIAN_POINT('Ctrl Pts',(-48.1943732865555,-6.007051447105,4.29441317095728));
#26306=CARTESIAN_POINT('Ctrl Pts',(-48.352959262434,-14.4313124010519,29.4551542809743));
#26307=CARTESIAN_POINT('Ctrl Pts',(-48.3280930508149,-14.7671408703067,
29.45593300004));
#26308=CARTESIAN_POINT('Ctrl Pts',(-48.6646643620667,-14.7669045053135,
29.4431122185066));
#26309=CARTESIAN_POINT('Ctrl Pts',(-48.3569869626293,-14.4776157931201,
29.656936726707));
#26310=CARTESIAN_POINT('Ctrl Pts',(-48.3813383783207,-14.7670932226576,
29.6397654298998));
#26311=CARTESIAN_POINT('Ctrl Pts',(-48.6727054456496,-14.766904515933,29.668999675558));
#26312=CARTESIAN_POINT('Ctrl Pts',(-48.3491923518221,-14.5232222287049,
29.8548235931214));
#26313=CARTESIAN_POINT('Ctrl Pts',(-48.4096589429883,-14.7670538266339,
29.8485725191841));
#26314=CARTESIAN_POINT('Ctrl Pts',(-48.6570966106634,-14.7669045263941,
29.8909334903031));
#26315=CARTESIAN_POINT('Ctrl Pts',(-48.3036995582031,-14.6124212350927,
30.2403918438327));
#26316=CARTESIAN_POINT('Ctrl Pts',(-48.395816449558,-14.7669897766186,30.2571389072456));
#26317=CARTESIAN_POINT('Ctrl Pts',(-48.5660672929221,-14.7669045468573,
30.3240933952862));
#26318=CARTESIAN_POINT('Ctrl Pts',(-48.2672919864971,-14.6570503433833,
30.4325068115059));
#26319=CARTESIAN_POINT('Ctrl Pts',(-48.3627479488335,-14.7669625172413,
30.4679205353142));
#26320=CARTESIAN_POINT('Ctrl Pts',(-48.492687194552,-14.766904557097,30.5411709062376));
#26321=CARTESIAN_POINT('Ctrl Pts',(-48.1953287895212,-14.694785451968,30.5944226583824));
#26322=CARTESIAN_POINT('Ctrl Pts',(-48.2623775405895,-14.7669413153286,
30.6502218321353));
#26323=CARTESIAN_POINT('Ctrl Pts',(-48.3495845206488,-14.7669045657556,
30.7223070272069));
#26324=CARTESIAN_POINT('Origin',(-48.415424133227,-14.4544045823054,30.6288487842778));
#26325=CARTESIAN_POINT('Origin',(0.0835265683620477,-14.4544045823054,0.0824317919394229));
#26326=CARTESIAN_POINT('Origin',(-47.352376130838,-14.4544045823054,-32.090024523005));
#26327=CARTESIAN_POINT('Ctrl Pts',(-47.1776813530825,-14.6836564585996,
-31.9686806405055));
#26328=CARTESIAN_POINT('Ctrl Pts',(-47.0660250366126,-14.7195047625521,
-32.1971938623823));
#26329=CARTESIAN_POINT('Ctrl Pts',(-46.8969354814603,-14.9046273277204,
-32.1414364890551));
#26330=CARTESIAN_POINT('Ctrl Pts',(-46.7203857499136,-14.2208393515128,
-31.8184056045622));
#26331=CARTESIAN_POINT('Ctrl Pts',(-46.6089836705754,-14.2572370951416,
-32.0464842218602));
#26332=CARTESIAN_POINT('Ctrl Pts',(-46.43992721307,-14.4418102212131,-31.9907377625058));
#26333=CARTESIAN_POINT('Ctrl Pts',(-46.2628591696178,-13.7582547217153,
-31.6680667910224));
#26334=CARTESIAN_POINT('Ctrl Pts',(-46.1514245671171,-13.7949155819443,
-31.895603857149));
#26335=CARTESIAN_POINT('Ctrl Pts',(-45.9826965856166,-13.9792255914456,
-31.8399657129337));
#26336=CARTESIAN_POINT('Ctrl Pts',(-45.805095386722,-13.2959337131846,-31.5176630410747));
#26337=CARTESIAN_POINT('Ctrl Pts',(-45.6932984645427,-13.3325299785125,
-31.7445365241682));
#26338=CARTESIAN_POINT('Ctrl Pts',(-45.5252381517553,-13.5169045823054,
-31.689118544074));
#26339=CARTESIAN_POINT('Ctrl Pts',(-46.45221964492,-14.4544045595336,-31.994791198634));
#26340=CARTESIAN_POINT('Ctrl Pts',(-46.4816446151428,-14.4645898091214,
-32.0044940986644));
#26341=CARTESIAN_POINT('Ctrl Pts',(-46.5113244534831,-14.4747854410082,
-32.0132766896869));
#26342=CARTESIAN_POINT('Ctrl Pts',(-46.5412186258095,-14.4849571274434,
-32.0211162927955));
#26343=CARTESIAN_POINT('Ctrl Pts',(-46.5691103832093,-14.4944474791848,
-32.0284307722073));
#26344=CARTESIAN_POINT('Ctrl Pts',(-46.5971900557739,-14.5039154723653,
-32.0349249639908));
#26345=CARTESIAN_POINT('Ctrl Pts',(-46.6254440592878,-14.513327931455,-32.040538038467));
#26346=CARTESIAN_POINT('Ctrl Pts',(-46.6523812355758,-14.5223017064346,
-32.0458895057948));
#26347=CARTESIAN_POINT('Ctrl Pts',(-46.6794781232448,-14.5312237762472,
-32.0504400452471));
#26348=CARTESIAN_POINT('Ctrl Pts',(-46.7067229940643,-14.5400795913945,
-32.054093202545));
#26349=CARTESIAN_POINT('Ctrl Pts',(-46.7320468275605,-14.548310982534,-32.0574887755232));
#26350=CARTESIAN_POINT('Ctrl Pts',(-46.7574994914588,-14.5564843935861,
-32.0601083525393));
#26351=CARTESIAN_POINT('Ctrl Pts',(-46.7830561411086,-14.5646141114386,
-32.0618415033403));
#26352=CARTESIAN_POINT('Ctrl Pts',(-46.7938944251968,-14.5680618322021,
-32.0625765128586));
#26353=CARTESIAN_POINT('Ctrl Pts',(-46.8047511303372,-14.5715020908807,
-32.0631517327013));
#26354=CARTESIAN_POINT('Ctrl Pts',(-46.8156227743728,-14.5749379971502,
-32.0635573491533));
#26355=CARTESIAN_POINT('Ctrl Pts',(-46.8348797214202,-14.5810240191793,
-32.0642758177227));
#26356=CARTESIAN_POINT('Ctrl Pts',(-46.8541789969005,-14.587111545562,-32.0644726060865));
#26357=CARTESIAN_POINT('Ctrl Pts',(-46.8734909509673,-14.5931215908451,
-32.0640314432956));
#26358=CARTESIAN_POINT('Ctrl Pts',(-46.8920891917075,-14.5989095224366,
-32.0636065845909));
#26359=CARTESIAN_POINT('Ctrl Pts',(-46.9106999302976,-14.6046251025895,
-32.0625893261362));
#26360=CARTESIAN_POINT('Ctrl Pts',(-46.9292727569436,-14.6102297042048,
-32.0608503486169));
#26361=CARTESIAN_POINT('Ctrl Pts',(-46.946858713788,-14.6155365045112,-32.0592037719169));
#26362=CARTESIAN_POINT('Ctrl Pts',(-46.9644111583127,-14.6207436431621,
-32.0569091901701));
#26363=CARTESIAN_POINT('Ctrl Pts',(-46.9818569474271,-14.6258519573889,
-32.0538455697298));
#26364=CARTESIAN_POINT('Ctrl Pts',(-46.9884617944842,-14.62778592747,-32.0526857056321));
#26365=CARTESIAN_POINT('Ctrl Pts',(-46.9950509954036,-14.6297061021637,
-32.051415567437));
#26366=CARTESIAN_POINT('Ctrl Pts',(-47.0016191535238,-14.6316139267952,
-32.0500286163118));
#26367=CARTESIAN_POINT('Ctrl Pts',(-47.0143605766674,-14.6353148731592,
-32.0473381008213));
#26368=CARTESIAN_POINT('Ctrl Pts',(-47.027091438687,-14.6390800656574,-32.0442661993923));
#26369=CARTESIAN_POINT('Ctrl Pts',(-47.0397058401586,-14.6427512671777,
-32.0406480116584));
#26370=CARTESIAN_POINT('Ctrl Pts',(-47.0517158141394,-14.6462465606196,
-32.0372031918119));
#26371=CARTESIAN_POINT('Ctrl Pts',(-47.0636206116162,-14.6496565428155,
-32.0332623412524));
#26372=CARTESIAN_POINT('Ctrl Pts',(-47.075298133029,-14.6528783603918,-32.0286727207447));
#26373=CARTESIAN_POINT('Ctrl Pts',(-47.0864623275873,-14.6559585515542,
-32.0242848532781));
#26374=CARTESIAN_POINT('Ctrl Pts',(-47.0974190452162,-14.6588667966838,
-32.0193031007959));
#26375=CARTESIAN_POINT('Ctrl Pts',(-47.10802817365,-14.6615453756124,-32.0135965587108));
#26376=CARTESIAN_POINT('Ctrl Pts',(-47.118301340523,-14.6641391314037,-32.0080707269261));
#26377=CARTESIAN_POINT('Ctrl Pts',(-47.1282486966118,-14.6665177507384,
-32.0018642831368));
#26378=CARTESIAN_POINT('Ctrl Pts',(-47.1377081632209,-14.6686579758303,
-31.9948745418285));
#26379=CARTESIAN_POINT('Ctrl Pts',(-47.1467984820774,-14.6707146804327,
-31.9881575693139));
#26380=CARTESIAN_POINT('Ctrl Pts',(-47.155438026338,-14.6725517512547,-31.9807163227433));
#26381=CARTESIAN_POINT('Ctrl Pts',(-47.1634510955046,-14.6741705573044,
-31.9724887075062));
#26382=CARTESIAN_POINT('Ctrl Pts',(-47.1655096976883,-14.6745864376119,
-31.9703749872398));
#26383=CARTESIAN_POINT('Ctrl Pts',(-47.1675267947758,-14.6749880046777,
-31.9682095601077));
#26384=CARTESIAN_POINT('Ctrl Pts',(-47.1694990908454,-14.6753754514118,
-31.9659918126594));
#26385=CARTESIAN_POINT('Origin',(4.96196078618764,-13.5169045823054,-14.7118854886012));
#26386=CARTESIAN_POINT('Origin',(-38.9085015017574,-13.5169045823054,-29.1781944313494));
#26387=CARTESIAN_POINT('Origin',(0.0835265683620477,-12.8919045823054,0.0824317919394229));
#26388=CARTESIAN_POINT('Ctrl Pts',(-38.5307586915594,-12.8919045823054,
-29.1601464137424));
#26389=CARTESIAN_POINT('Ctrl Pts',(-38.5307586915594,-12.9139187960387,
-29.1601464137424));
#26390=CARTESIAN_POINT('Ctrl Pts',(-38.5337445953841,-12.9356278245207,
-29.1602796388799));
#26391=CARTESIAN_POINT('Ctrl Pts',(-38.5392655962948,-12.9566097073211,
-29.1605287235832));
#26392=CARTESIAN_POINT('Ctrl Pts',(-38.5446601059366,-12.9771108756598,
-29.160772101524));
#26393=CARTESIAN_POINT('Ctrl Pts',(-38.5524746087403,-12.9969176625741,
-29.1611260778435));
#26394=CARTESIAN_POINT('Ctrl Pts',(-38.5623024668082,-13.0156824718616,
-29.1615748389679));
#26395=CARTESIAN_POINT('Ctrl Pts',(-38.5724342229867,-13.0350275286508,
-29.1620374767332));
#26396=CARTESIAN_POINT('Ctrl Pts',(-38.5847053607061,-13.0532645768204,
-29.1626008360293));
#26397=CARTESIAN_POINT('Ctrl Pts',(-38.5986906617097,-13.0700686738439,
-29.1632482299304));
#26398=CARTESIAN_POINT('Ctrl Pts',(-38.6117491326753,-13.0857591343516,
-29.1638527199202));
#26399=CARTESIAN_POINT('Ctrl Pts',(-38.6263021044288,-13.1002006435705,
-29.1645304749228));
#26400=CARTESIAN_POINT('Ctrl Pts',(-38.6420231546125,-13.1131767225593,
-29.1652685557058));
#26401=CARTESIAN_POINT('Ctrl Pts',(-38.6431389622425,-13.1140977047949,
-29.1653209412755));
#26402=CARTESIAN_POINT('Ctrl Pts',(-38.6442606627878,-13.1150113249631,
-29.1653736310233));
#26403=CARTESIAN_POINT('Ctrl Pts',(-38.6453881435972,-13.1159175149051,
-29.1654266204564));
#26404=CARTESIAN_POINT('Ctrl Pts',(-38.6482835083063,-13.1182446058459,
-29.1655626970383));
#26405=CARTESIAN_POINT('Ctrl Pts',(-38.6512164926939,-13.1205242789863,
-29.1657007960921));
#26406=CARTESIAN_POINT('Ctrl Pts',(-38.6541844981536,-13.1227565895721,
-29.1658408010566));
#26407=CARTESIAN_POINT('Ctrl Pts',(-38.6686039641446,-13.1336018279015,
-29.1665209874148));
#26408=CARTESIAN_POINT('Ctrl Pts',(-38.6838415011964,-13.143325954299,-29.167242672684));
#26409=CARTESIAN_POINT('Ctrl Pts',(-38.6996821390438,-13.1519718238994,
-29.1679966343372));
#26410=CARTESIAN_POINT('Ctrl Pts',(-38.7169622638872,-13.161403369997,-29.1688191107818));
#26411=CARTESIAN_POINT('Ctrl Pts',(-38.7349606742429,-13.1695524259116,
-29.1696800142245));
#26412=CARTESIAN_POINT('Ctrl Pts',(-38.7534545213138,-13.1764446443681,
-29.1705703361828));
#26413=CARTESIAN_POINT('Ctrl Pts',(-38.7727096512048,-13.1836205748875,
-29.1714973074553));
#26414=CARTESIAN_POINT('Ctrl Pts',(-38.7925031927513,-13.1894346380336,
-29.1724562261581));
#26415=CARTESIAN_POINT('Ctrl Pts',(-38.812625947123,-13.1938753423331,-29.1734393751561));
#26416=CARTESIAN_POINT('Ctrl Pts',(-38.8328614137049,-13.1983409200464,
-29.1744280309994));
#26417=CARTESIAN_POINT('Ctrl Pts',(-38.8534314395746,-13.2014181302604,
-29.1754412664497));
#26418=CARTESIAN_POINT('Ctrl Pts',(-38.8741419834054,-13.2030479859155,
-29.1764726165817));
#26419=CARTESIAN_POINT('Ctrl Pts',(-38.8855632109547,-13.2039468011499,
-29.1770413744393));
#26420=CARTESIAN_POINT('Ctrl Pts',(-38.897027358863,-13.2044045823054,-29.177615659075));
#26421=CARTESIAN_POINT('Ctrl Pts',(-38.9085015017574,-13.2044045823054,
-29.1781944313494));
#26422=CARTESIAN_POINT('Origin',(-33.5252021444999,-14.7669045823054,-34.3627272192373));
#26423=CARTESIAN_POINT('Origin',(-33.5252021444999,-11.3294045823054,-34.3627272192373));
#26424=CARTESIAN_POINT('Origin',(6.83612114566777,-11.3294045823054,-20.3954556167886));
#26425=CARTESIAN_POINT('Ctrl Pts',(-34.0238404855175,-11.0169045823054,
-33.869050320804));
#26426=CARTESIAN_POINT('Ctrl Pts',(-34.001815058166,-11.0169045823054,-33.8801197224743));
#26427=CARTESIAN_POINT('Ctrl Pts',(-33.9800079311155,-11.0183080822726,
-33.8910410032133));
#26428=CARTESIAN_POINT('Ctrl Pts',(-33.9583457631457,-11.0211596046316,
-33.9018512749977));
#26429=CARTESIAN_POINT('Ctrl Pts',(-33.9370471546751,-11.023963269452,-33.912480116327));
#26430=CARTESIAN_POINT('Ctrl Pts',(-33.9158885755623,-11.0281667153259,
-33.9230016547809));
#26431=CARTESIAN_POINT('Ctrl Pts',(-33.8948092427032,-11.0338614984686,
-33.9334452009051));
#26432=CARTESIAN_POINT('Ctrl Pts',(-33.8894330516898,-11.0353139278296,
-33.9361087813512));
#26433=CARTESIAN_POINT('Ctrl Pts',(-33.884062065986,-11.0368636220457,-33.9387672573208));
#26434=CARTESIAN_POINT('Ctrl Pts',(-33.878695385463,-11.0385126341271,-33.9414210499132));
#26435=CARTESIAN_POINT('Ctrl Pts',(-33.8589867794304,-11.0445684687008,
-33.9511668420231));
#26436=CARTESIAN_POINT('Ctrl Pts',(-33.8397948590732,-11.0518127318511,
-33.9606228528326));
#26437=CARTESIAN_POINT('Ctrl Pts',(-33.8211446482646,-11.0604015318982,
-33.9697802594569));
#26438=CARTESIAN_POINT('Ctrl Pts',(-33.802494437456,-11.0689903319452,-33.9789376660811));
#26439=CARTESIAN_POINT('Ctrl Pts',(-33.7843855638675,-11.0789231726624,
-33.9877965998101));
#26440=CARTESIAN_POINT('Ctrl Pts',(-33.7668743980404,-11.0904031558603,
-33.9963333935331));
#26441=CARTESIAN_POINT('Ctrl Pts',(-33.7611096994568,-11.0941823812718,
-33.9991437171386));
#26442=CARTESIAN_POINT('Ctrl Pts',(-33.755434798592,-11.0981143207712,-34.0019084815749));
#26443=CARTESIAN_POINT('Ctrl Pts',(-33.7498350694776,-11.1022159367836,
-34.0046347500796));
#26444=CARTESIAN_POINT('Ctrl Pts',(-33.7402458756978,-11.1092397034604,
-34.0093033182287));
#26445=CARTESIAN_POINT('Ctrl Pts',(-33.7310218705821,-11.116663053783,-34.0137885684103));
#26446=CARTESIAN_POINT('Ctrl Pts',(-33.722142970915,-11.1245727500517,-34.0181002904555));
#26447=CARTESIAN_POINT('Ctrl Pts',(-33.7187799860189,-11.1275686380651,
-34.0197334045414));
#26448=CARTESIAN_POINT('Ctrl Pts',(-33.7154669091464,-11.1306345602644,
-34.0213414284975));
#26449=CARTESIAN_POINT('Ctrl Pts',(-33.712204213352,-11.133776202165,-34.0229241322475));
#26450=CARTESIAN_POINT('Ctrl Pts',(-33.7037506457484,-11.1419161219939,
-34.0270248802151));
#26451=CARTESIAN_POINT('Ctrl Pts',(-33.6956687991695,-11.1505315993466,
-34.0309393829992));
#26452=CARTESIAN_POINT('Ctrl Pts',(-33.6880349165851,-11.1596598005335,
-34.0346338552862));
#26453=CARTESIAN_POINT('Ctrl Pts',(-33.6804010340008,-11.1687880017203,
-34.0383283275731));
#26454=CARTESIAN_POINT('Ctrl Pts',(-33.6732197547124,-11.1784304387767,
-34.0418051487081));
#26455=CARTESIAN_POINT('Ctrl Pts',(-33.6665631119894,-11.18862206557,-34.0450152174752));
#26456=CARTESIAN_POINT('Ctrl Pts',(-33.6633982723472,-11.19346758092,-34.0465414151864));
#26457=CARTESIAN_POINT('Ctrl Pts',(-33.6603504947342,-11.1984446423577,
-34.0480104432143));
#26458=CARTESIAN_POINT('Ctrl Pts',(-33.6574354435571,-11.2035509891889,
-34.049414947688));
#26459=CARTESIAN_POINT('Ctrl Pts',(-33.6506402480387,-11.2154542536581,
-34.0526889493864));
#26460=CARTESIAN_POINT('Ctrl Pts',(-33.6446840759846,-11.2278803704208,
-34.0555560984262));
#26461=CARTESIAN_POINT('Ctrl Pts',(-33.6397392256017,-11.240725680505,-34.0579348223755));
#26462=CARTESIAN_POINT('Ctrl Pts',(-33.634908566084,-11.2532743553102,-34.0602586147242));
#26463=CARTESIAN_POINT('Ctrl Pts',(-33.6310434307528,-11.2662226779423,
-34.0621161155791));
#26464=CARTESIAN_POINT('Ctrl Pts',(-33.6282635085628,-11.2794553416036,
-34.0634513323074));
#26465=CARTESIAN_POINT('Ctrl Pts',(-33.6255593642006,-11.2923272964251,
-34.0647501523971));
#26466=CARTESIAN_POINT('Ctrl Pts',(-33.6238822840565,-11.3054678991102,
-34.0655546880424));
#26467=CARTESIAN_POINT('Ctrl Pts',(-33.6232990879972,-11.3187590936903,
-34.0658343883027));
#26468=CARTESIAN_POINT('Ctrl Pts',(-33.6231438180531,-11.3222977373521,
-34.0659088556161));
#26469=CARTESIAN_POINT('Ctrl Pts',(-33.6230658340261,-11.3258470068808,
-34.0659462422992));
#26470=CARTESIAN_POINT('Ctrl Pts',(-33.6230658340261,-11.3294045823054,
-34.0659462422992));
#26471=CARTESIAN_POINT('Origin',(0.0835265683620477,-11.3294045823054,0.0824317919394229));
#26472=CARTESIAN_POINT('Origin',(9.92432302202933,-11.3294045823054,19.2683675629017));
#26473=CARTESIAN_POINT('Origin',(10.2095634989472,-11.0169045823054,19.8244816432194));
#26474=CARTESIAN_POINT('Origin',(10.2095634989472,-11.3294045823054,19.8244816432194));
#26475=CARTESIAN_POINT('Origin',(-4.79490764946355,-13.5169045823054,14.87674907248));
#26476=CARTESIAN_POINT('Origin',(39.0755546384815,-13.5169045823054,29.3430580152282));
#26477=CARTESIAN_POINT('Origin',(0.0835265683620477,-12.8919045823054,0.0824317919394229));
#26478=CARTESIAN_POINT('Ctrl Pts',(38.6978118282835,-12.8919045823054,29.3250099976212));
#26479=CARTESIAN_POINT('Ctrl Pts',(38.6978118282835,-12.9139187960388,29.3250099976212));
#26480=CARTESIAN_POINT('Ctrl Pts',(38.7007977321083,-12.9356278245209,29.3251432227588));
#26481=CARTESIAN_POINT('Ctrl Pts',(38.7063187330191,-12.9566097073213,29.325392307462));
#26482=CARTESIAN_POINT('Ctrl Pts',(38.711713242661,-12.9771108756606,29.3256356854028));
#26483=CARTESIAN_POINT('Ctrl Pts',(38.7195277454651,-12.9969176625753,29.3259896617223));
#26484=CARTESIAN_POINT('Ctrl Pts',(38.7293556035333,-13.0156824718633,29.3264384228467));
#26485=CARTESIAN_POINT('Ctrl Pts',(38.7394873597118,-13.0350275286521,29.326901060612));
#26486=CARTESIAN_POINT('Ctrl Pts',(38.7517584974311,-13.0532645768214,29.3274644199081));
#26487=CARTESIAN_POINT('Ctrl Pts',(38.7657437984346,-13.0700686738447,29.3281118138092));
#26488=CARTESIAN_POINT('Ctrl Pts',(38.7788022694006,-13.0857591343528,29.328716303799));
#26489=CARTESIAN_POINT('Ctrl Pts',(38.7933552411545,-13.100200643572,29.3293940588016));
#26490=CARTESIAN_POINT('Ctrl Pts',(38.8090762913388,-13.1131767225611,29.3301321395847));
#26491=CARTESIAN_POINT('Ctrl Pts',(38.8101920989681,-13.114097704796,29.3301845251543));
#26492=CARTESIAN_POINT('Ctrl Pts',(38.8113137995126,-13.1150113249637,29.3302372149021));
#26493=CARTESIAN_POINT('Ctrl Pts',(38.8124412803214,-13.115917514905,29.3302902043352));
#26494=CARTESIAN_POINT('Ctrl Pts',(38.8153366450305,-13.1182446058459,29.3304262809171));
#26495=CARTESIAN_POINT('Ctrl Pts',(38.818269629418,-13.1205242789863,29.3305643799709));
#26496=CARTESIAN_POINT('Ctrl Pts',(38.8212376348777,-13.1227565895721,29.3307043849354));
#26497=CARTESIAN_POINT('Ctrl Pts',(38.8356571008678,-13.1336018279008,29.3313845712936));
#26498=CARTESIAN_POINT('Ctrl Pts',(38.8508946379186,-13.1433259542978,29.3321062565627));
#26499=CARTESIAN_POINT('Ctrl Pts',(38.8667352757648,-13.1519718238976,29.3328602182159));
#26500=CARTESIAN_POINT('Ctrl Pts',(38.8840154006071,-13.1614033699948,29.3336826946604));
#26501=CARTESIAN_POINT('Ctrl Pts',(38.9020138109617,-13.1695524259092,29.3345435981031));
#26502=CARTESIAN_POINT('Ctrl Pts',(38.9205076580314,-13.1764446443656,29.3354339200614));
#26503=CARTESIAN_POINT('Ctrl Pts',(38.9397627879212,-13.1836205748849,29.3363608913338));
#26504=CARTESIAN_POINT('Ctrl Pts',(38.9595563294665,-13.1894346380311,29.3373198100366));
#26505=CARTESIAN_POINT('Ctrl Pts',(38.9796790838369,-13.1938753423308,29.3383029590345));
#26506=CARTESIAN_POINT('Ctrl Pts',(38.9999145504174,-13.1983409200443,29.3392916148777));
#26507=CARTESIAN_POINT('Ctrl Pts',(39.0204845762857,-13.2014181302587,29.3403048503279));
#26508=CARTESIAN_POINT('Ctrl Pts',(39.0411951201151,-13.2030479859143,29.3413362004598));
#26509=CARTESIAN_POINT('Ctrl Pts',(39.0526163476692,-13.2039468011495,29.3419049583177));
#26510=CARTESIAN_POINT('Ctrl Pts',(39.0640804955822,-13.2044045823054,29.3424792429536));
#26511=CARTESIAN_POINT('Ctrl Pts',(39.0755546384815,-13.2044045823054,29.3430580152282));
#26512=CARTESIAN_POINT('Origin',(0.0835265683620477,-5.88746284406389,0.0824317919394229));
#26513=CARTESIAN_POINT('Origin',(-36.4579813137992,-5.88746284406388,32.3513131127716));
#26514=CARTESIAN_POINT('Ctrl Pts',(-38.3808256972991,-13.5144022830795,
39.8924656416407));
#26515=CARTESIAN_POINT('Ctrl Pts',(-38.4711302762978,-13.1933434688295,
40.1663228945616));
#26516=CARTESIAN_POINT('Ctrl Pts',(-38.8323465692944,-13.2935409679816,
39.9525013588595));
#26517=CARTESIAN_POINT('Ctrl Pts',(-37.4650940302067,-10.8876753972538,
37.115421979291));
#26518=CARTESIAN_POINT('Ctrl Pts',(-37.5465445455966,-10.5315615515785,
37.3624284395829));
#26519=CARTESIAN_POINT('Ctrl Pts',(-37.9202835812346,-10.666849201302,37.1719078497633));
#26520=CARTESIAN_POINT('Ctrl Pts',(-36.5421507433461,-8.28316552043086,
34.3165083918393));
#26521=CARTESIAN_POINT('Ctrl Pts',(-36.6205153658898,-7.90880842130267,
34.5541565874725));
#26522=CARTESIAN_POINT('Ctrl Pts',(-37.0014278556075,-8.0623563845108,34.3687899544871));
#26523=CARTESIAN_POINT('Ctrl Pts',(-35.6087810892669,-5.72100919352294,
31.485975850882));
#26524=CARTESIAN_POINT('Ctrl Pts',(-35.7020590377777,-5.37442444069083,
31.7688501306084));
#26525=CARTESIAN_POINT('Ctrl Pts',(-36.0726730777933,-5.50017071946578,
31.5328901029015));
#26526=CARTESIAN_POINT('Origin',(-38.4603055734906,-12.8919045823054,39.1356156285706));
#26527=CARTESIAN_POINT('Ctrl Pts',(-36.101076272966,-7.07886051013274,32.9789079716315));
#26528=CARTESIAN_POINT('Ctrl Pts',(-36.0899132796569,-6.97591157388736,
32.9450525778012));
#26529=CARTESIAN_POINT('Ctrl Pts',(-36.0884195965777,-6.87711064623164,
32.898798434336));
#26530=CARTESIAN_POINT('Ctrl Pts',(-36.0959936162844,-6.68740381001555,
32.7941789389639));
#26531=CARTESIAN_POINT('Ctrl Pts',(-36.1053616074735,-6.59673597566757,
32.7354819475306));
#26532=CARTESIAN_POINT('Ctrl Pts',(-36.1345672829262,-6.42451466437637,
32.6062788880432));
#26533=CARTESIAN_POINT('Ctrl Pts',(-36.1540093300512,-6.34396835910597,
32.5368889705491));
#26534=CARTESIAN_POINT('Ctrl Pts',(-36.1942336893731,-6.23614184370368,
32.4215531154926));
#26535=CARTESIAN_POINT('Ctrl Pts',(-36.2094997401739,-6.2025085626214,32.3812785420796));
#26536=CARTESIAN_POINT('Ctrl Pts',(-36.245538447344,-6.14483638321708,32.2965923390849));
#26537=CARTESIAN_POINT('Ctrl Pts',(-36.2661556687914,-6.11985717446073,
32.2519654539084));
#26538=CARTESIAN_POINT('Ctrl Pts',(-36.2923483136821,-6.10843371318468,
32.2050467999301));
#26539=CARTESIAN_POINT('Origin',(0.0835265683620477,-14.4544045823054,0.0824317919394229));
#26540=CARTESIAN_POINT('Origin',(-37.6790715732587,-14.4544045823054,43.2010819542467));
#26541=CARTESIAN_POINT('Origin',(-11.548656164376,-14.4544045823054,-33.4956062992654));
#26542=CARTESIAN_POINT('Origin',(-20.394360840366,-14.4544045823054,-6.6701627853663));
#26543=CARTESIAN_POINT('Origin',(-36.6439262383654,-14.4544045823054,42.6081948668641));
#26544=CARTESIAN_POINT('Ctrl Pts',(-46.3756986917116,-14.426701821065,-31.967386032015));
#26545=CARTESIAN_POINT('Ctrl Pts',(-46.3877592862997,-14.7669045823054,
-31.9392629591333));
#26546=CARTESIAN_POINT('Ctrl Pts',(-46.2541665130207,-14.7669045823054,
-32.2540056786749));
#26547=CARTESIAN_POINT('Ctrl Pts',(-46.5262167757777,-14.4797609665103,
-32.0258294594699));
#26548=CARTESIAN_POINT('Ctrl Pts',(-46.4971544532193,-14.7669045823055,
-32.0448734520714));
#26549=CARTESIAN_POINT('Ctrl Pts',(-46.4502337580146,-14.7669045823054,
-32.3366490875369));
#26550=CARTESIAN_POINT('Ctrl Pts',(-46.6937109365492,-14.5360769750864,
-32.0634681128903));
#26551=CARTESIAN_POINT('Ctrl Pts',(-46.6746692672182,-14.7669045823052,
-32.1327773356701));
#26552=CARTESIAN_POINT('Ctrl Pts',(-46.6742499978977,-14.7669045823054,
-32.3756703660879));
#26553=CARTESIAN_POINT('Ctrl Pts',(-47.0039073691806,-14.6333609973518,
-32.0644095936465));
#26554=CARTESIAN_POINT('Ctrl Pts',(-47.0271134517325,-14.7669045823056,
-32.1591547728184));
#26555=CARTESIAN_POINT('Ctrl Pts',(-47.1033317152047,-14.7669045823054,
-32.3146159839169));
#26556=CARTESIAN_POINT('Ctrl Pts',(-47.1546671567785,-14.6768299128525,
-32.0274598660431));
#26557=CARTESIAN_POINT('Ctrl Pts',(-47.2215585124842,-14.7669045823053,
-32.109304007213));
#26558=CARTESIAN_POINT('Ctrl Pts',(-47.3201303649606,-14.7669045823054,
-32.2117463895627));
#26559=CARTESIAN_POINT('Ctrl Pts',(-47.2003152129085,-14.6796363815825,
-31.9161588440568));
#26560=CARTESIAN_POINT('Ctrl Pts',(-47.2868308580741,-14.7669045823054,
-31.9448707178761));
#26561=CARTESIAN_POINT('Ctrl Pts',(-47.4053176024544,-14.7669045823054,
-31.9879994785672));
#26562=CARTESIAN_POINT('Origin',(-46.3543559346078,-14.4544045823054,-32.2915721687179));
#26563=CARTESIAN_POINT('Ctrl Pts',(-38.1837705810014,-12.8919045823054,
-29.2682655958051));
#26564=CARTESIAN_POINT('Ctrl Pts',(-38.3959057211593,-12.8919045823054,
-29.3382172743398));
#26565=CARTESIAN_POINT('Ctrl Pts',(-38.5307586915594,-12.8919045823054,
-29.1601464137424));
#26566=CARTESIAN_POINT('Ctrl Pts',(-38.183770659511,-13.0608832998915,-29.2682656216937));
#26567=CARTESIAN_POINT('Ctrl Pts',(-38.3959057800757,-12.9975414109163,
-29.3382172937695));
#26568=CARTESIAN_POINT('Ctrl Pts',(-38.5307587078212,-12.9763939382003,
-29.1601463922689));
#26569=CARTESIAN_POINT('Ctrl Pts',(-38.2565492552502,-13.2263898891533,
-29.2922644034588));
#26570=CARTESIAN_POINT('Ctrl Pts',(-38.4533226892664,-13.1003236725306,
-29.3571505509882));
#26571=CARTESIAN_POINT('Ctrl Pts',(-38.574755077224,-13.0591472399314,-29.1621091252889));
#26572=CARTESIAN_POINT('Ctrl Pts',(-38.4907620671097,-13.453458690012,-29.3694962063167));
#26573=CARTESIAN_POINT('Ctrl Pts',(-38.6179212721247,-13.2166231342359,
-29.4114270237444));
#26574=CARTESIAN_POINT('Ctrl Pts',(-38.7160379547609,-13.1726816319567,
-29.1687114403196));
#26575=CARTESIAN_POINT('Ctrl Pts',(-38.6517584445698,-13.5169045492971,
-29.4225848498718));
#26576=CARTESIAN_POINT('Ctrl Pts',(-38.7263955296224,-13.2287751252084,
-29.4471964695062));
#26577=CARTESIAN_POINT('Ctrl Pts',(-38.8130299365641,-13.2044045823054,
-29.1733787082547));
#26578=CARTESIAN_POINT('Ctrl Pts',(-38.8106378122312,-13.5169045823054,
-29.4749754082874));
#26579=CARTESIAN_POINT('Ctrl Pts',(-38.8106378122312,-13.2044045823054,
-29.4749754082874));
#26580=CARTESIAN_POINT('Ctrl Pts',(-38.9085015017574,-13.2044045823054,
-29.1781944313494));
#26581=CARTESIAN_POINT('Ctrl Pts',(-34.2453168949582,-10.7044045823054,
-34.0895144903673));
#26582=CARTESIAN_POINT('Ctrl Pts',(-34.2453168949582,-11.0169045823054,
-34.0895144903673));
#26583=CARTESIAN_POINT('Ctrl Pts',(-34.0238404855175,-11.0169045823054,
-33.869050320804));
#26584=CARTESIAN_POINT('Ctrl Pts',(-34.1831061101228,-10.7044046073823,
-34.1520109099947));
#26585=CARTESIAN_POINT('Ctrl Pts',(-34.2067524199087,-11.0349449313269,
-34.1282560290212));
#26586=CARTESIAN_POINT('Ctrl Pts',(-33.9742956506306,-11.0169045823054,
-33.8939502540348));
#26587=CARTESIAN_POINT('Ctrl Pts',(-34.1223018123232,-10.7186506766711,
-34.2127522663462));
#26588=CARTESIAN_POINT('Ctrl Pts',(-34.174388313845,-11.0630714156278,-34.160693357711));
#26589=CARTESIAN_POINT('Ctrl Pts',(-33.9258201978111,-11.0240276257398,
-33.9181007183444));
#26590=CARTESIAN_POINT('Ctrl Pts',(-34.0041449959219,-10.7765752156549,
-34.3301965896023));
#26591=CARTESIAN_POINT('Ctrl Pts',(-34.1234350039619,-11.1314870357705,
-34.2119315641541));
#26592=CARTESIAN_POINT('Ctrl Pts',(-33.8315341822154,-11.0529899027286,
-33.9647086119291));
#26593=CARTESIAN_POINT('Ctrl Pts',(-33.9500964242875,-10.8185639645428,
-34.3836165482575));
#26594=CARTESIAN_POINT('Ctrl Pts',(-34.107426121419,-11.1704305366376,-34.2281661619454));
#26595=CARTESIAN_POINT('Ctrl Pts',(-33.7883601256341,-11.0739842709864,
-33.985863384623));
#26596=CARTESIAN_POINT('Ctrl Pts',(-33.853696255335,-10.9314866347395,-34.4785417072161));
#26597=CARTESIAN_POINT('Ctrl Pts',(-34.0922214904,-11.2441510617713,-34.2442295368161));
#26598=CARTESIAN_POINT('Ctrl Pts',(-33.7113032982434,-11.1304456109602,
-34.0234016807259));
#26599=CARTESIAN_POINT('Ctrl Pts',(-33.8143209924547,-10.9992937157271,
-34.5171182906613));
#26600=CARTESIAN_POINT('Ctrl Pts',(-34.0948903060196,-11.275032611406,-34.2421982080992));
#26601=CARTESIAN_POINT('Ctrl Pts',(-33.6797999541619,-11.1643491474262,
-34.0386274161058));
#26602=CARTESIAN_POINT('Ctrl Pts',(-33.7584154529392,-11.1560957480195,
-34.571801649325));
#26603=CARTESIAN_POINT('Ctrl Pts',(-34.1052494433068,-11.3160025899705,
-34.2330567165343));
#26604=CARTESIAN_POINT('Ctrl Pts',(-33.6350580487545,-11.2427501667525,
-34.0601969961866));
#26605=CARTESIAN_POINT('Ctrl Pts',(-33.7434406299571,-11.2411599901508,
-34.5863970953167));
#26606=CARTESIAN_POINT('Ctrl Pts',(-34.111705002517,-11.3235538600013,-34.2270752707322));
#26607=CARTESIAN_POINT('Ctrl Pts',(-33.6230658263241,-11.2852822850309,
-34.0659462397595));
#26608=CARTESIAN_POINT('Ctrl Pts',(-33.7434406426353,-11.3294045823054,
-34.5863970829463));
#26609=CARTESIAN_POINT('Ctrl Pts',(-34.1117049987155,-11.3294045823054,
-34.2270752742097));
#26610=CARTESIAN_POINT('Ctrl Pts',(-33.6230658340261,-11.3294045823054,
-34.0659462422992));
#26611=CARTESIAN_POINT('Origin',(-34.0238404855175,-10.7044045823054,-33.869050320804));
#26612=CARTESIAN_POINT('Origin',(10.2095634989472,-11.3294045823054,19.8244816432194));
#26613=CARTESIAN_POINT('Ctrl Pts',(38.3508237177255,-12.8919045823054,29.4331291796839));
#26614=CARTESIAN_POINT('Ctrl Pts',(38.5629588578834,-12.8919045823054,29.5030808582187));
#26615=CARTESIAN_POINT('Ctrl Pts',(38.6978118282835,-12.8919045823054,29.3250099976212));
#26616=CARTESIAN_POINT('Ctrl Pts',(38.350823796233,-13.0608832998915,29.4331292055718));
#26617=CARTESIAN_POINT('Ctrl Pts',(38.5629589167962,-12.9975414109165,29.5030808776454));
#26618=CARTESIAN_POINT('Ctrl Pts',(38.6978118445448,-12.9763939382002,29.3250099761484));
#26619=CARTESIAN_POINT('Ctrl Pts',(38.4236023919749,-13.2263898891533,29.4571279873378));
#26620=CARTESIAN_POINT('Ctrl Pts',(38.620375825991,-13.1003236725305,29.5220141348676));
#26621=CARTESIAN_POINT('Ctrl Pts',(38.7418082139485,-13.0591472399316,29.3269727091676));
#26622=CARTESIAN_POINT('Ctrl Pts',(38.6578152038332,-13.453458690012,29.5343597901954));
#26623=CARTESIAN_POINT('Ctrl Pts',(38.7849744088482,-13.2166231342361,29.5762906076227));
#26624=CARTESIAN_POINT('Ctrl Pts',(38.8830910914846,-13.1726816319565,29.3335750241986));
#26625=CARTESIAN_POINT('Ctrl Pts',(38.8188115812943,-13.5169045492971,29.5874484337508));
#26626=CARTESIAN_POINT('Ctrl Pts',(38.8934486663472,-13.2287751252085,29.6120600533846));
#26627=CARTESIAN_POINT('Ctrl Pts',(38.9800830732885,-13.2044045823054,29.3382422921337));
#26628=CARTESIAN_POINT('Ctrl Pts',(38.9776909489554,-13.5169045823054,29.6398389921663));
#26629=CARTESIAN_POINT('Ctrl Pts',(38.9776909489554,-13.2044045823054,29.6398389921663));
#26630=CARTESIAN_POINT('Ctrl Pts',(39.0755546384815,-13.2044045823054,29.3430580152282));
#26631=CARTESIAN_POINT('Origin',(38.4486874072517,-12.8919045823054,29.1363482027458));
#26632=CARTESIAN_POINT('Ctrl Pts',(-36.1113722880935,-7.15534954836531,
33.0016931755516));
#26633=CARTESIAN_POINT('Ctrl Pts',(-35.9763481816599,-7.11664814652194,
32.4278063923816));
#26634=CARTESIAN_POINT('Ctrl Pts',(-35.5783817078538,-7.18677502450287,
32.8607815258895));
#26635=CARTESIAN_POINT('Ctrl Pts',(-36.0918388255004,-7.0323813740435,32.9705852224084));
#26636=CARTESIAN_POINT('Ctrl Pts',(-35.9090565323606,-7.08021162564815,
32.5013078276263));
#26637=CARTESIAN_POINT('Ctrl Pts',(-35.564706282625,-7.01162141061937,32.8756284637236));
#26638=CARTESIAN_POINT('Ctrl Pts',(-36.0873692866412,-6.90078625143554,
32.9127559686128));
#26639=CARTESIAN_POINT('Ctrl Pts',(-35.8673102683238,-6.94927177587728,
32.5462760319206));
#26640=CARTESIAN_POINT('Ctrl Pts',(-35.585966365718,-6.83269992246867,32.8525765797321));
#26641=CARTESIAN_POINT('Ctrl Pts',(-36.0969671734838,-6.67697195553551,
32.7883008612393));
#26642=CARTESIAN_POINT('Ctrl Pts',(-35.8606408249945,-6.69622936404145,
32.5523589912722));
#26643=CARTESIAN_POINT('Ctrl Pts',(-35.6598372587195,-6.53795985193932,
32.7719667293062));
#26644=CARTESIAN_POINT('Ctrl Pts',(-36.1074306592358,-6.58104909157621,
32.7253234355767));
#26645=CARTESIAN_POINT('Ctrl Pts',(-35.8746421662079,-6.57996991861085,
32.5365087108499));
#26646=CARTESIAN_POINT('Ctrl Pts',(-35.7054143329339,-6.41511471179787,
32.7221349900562));
#26647=CARTESIAN_POINT('Ctrl Pts',(-36.1398197461798,-6.40173475569592,
32.587610085579));
#26648=CARTESIAN_POINT('Ctrl Pts',(-35.9337948307645,-6.36383534698761,
32.4703146792546));
#26649=CARTESIAN_POINT('Ctrl Pts',(-35.8188321691327,-6.19278444406303,
32.597338416161));
#26650=CARTESIAN_POINT('Ctrl Pts',(-36.161056277475,-6.32050524456483,32.5150029822516));
#26651=CARTESIAN_POINT('Ctrl Pts',(-35.9753922140543,-6.26307762141936,
32.4239108003766));
#26652=CARTESIAN_POINT('Ctrl Pts',(-35.8846472105432,-6.0958003221978,32.5246216325155));
#26653=CARTESIAN_POINT('Ctrl Pts',(-36.2247954239019,-6.1637311406174,32.3388151446257));
#26654=CARTESIAN_POINT('Ctrl Pts',(-36.0984890197755,-6.07811517886866,
32.2859259488243));
#26655=CARTESIAN_POINT('Ctrl Pts',(-36.0617904772832,-5.92198390396995,
32.3272652323252));
#26656=CARTESIAN_POINT('Ctrl Pts',(-36.2697309116477,-6.09886182624416,
32.2364305893108));
#26657=CARTESIAN_POINT('Ctrl Pts',(-36.1863184857959,-6.00005797774074,
32.1870934995707));
#26658=CARTESIAN_POINT('Ctrl Pts',(-36.1766072923992,-5.86097989286269,
32.1982982661301));
#26659=CARTESIAN_POINT('Ctrl Pts',(-36.3252333085416,-6.10268725738925,
32.1504346278648));
#26660=CARTESIAN_POINT('Ctrl Pts',(-36.2789940619947,-6.01584203958864,
32.0817863832517));
#26661=CARTESIAN_POINT('Ctrl Pts',(-36.2968040480299,-5.898811532747,32.0615249766501));
#26662=CARTESIAN_POINT('Ctrl Pts',(-38.5771295391607,-12.5761796977906,
39.1976374646442));
#26663=CARTESIAN_POINT('Ctrl Pts',(-38.1814665062544,-12.4966730216623,
39.4769498488669));
#26664=CARTESIAN_POINT('Ctrl Pts',(-38.1281921118528,-12.8445798972105,
39.1371073079634));
#26665=CARTESIAN_POINT('Ctrl Pts',(-38.6656700537214,-12.7679658886679,
39.3797570567454));
#26666=CARTESIAN_POINT('Ctrl Pts',(-38.3164513392329,-12.6138199372472,
39.5074230596676));
#26667=CARTESIAN_POINT('Ctrl Pts',(-38.2040132293918,-12.9405865508062,
39.3235687157183));
#26668=CARTESIAN_POINT('Ctrl Pts',(-38.6835395010857,-12.9477999797135,
39.6148827885762));
#26669=CARTESIAN_POINT('Ctrl Pts',(-38.4171318344341,-12.8036087634358,
39.6739467335942));
#26670=CARTESIAN_POINT('Ctrl Pts',(-38.2488933633745,-13.0304169137555,
39.5493551304408));
#26671=CARTESIAN_POINT('Ctrl Pts',(-38.6136496865685,-13.1418528526573,
39.9537410970356));
#26672=CARTESIAN_POINT('Ctrl Pts',(-38.4275839700741,-13.0167291165574,
39.9599051875636));
#26673=CARTESIAN_POINT('Ctrl Pts',(-38.2612346165967,-13.1274080636024,
39.8605733849698));
#26674=CARTESIAN_POINT('Ctrl Pts',(-38.5809055860187,-13.1924895597096,
40.0560225836614));
#26675=CARTESIAN_POINT('Ctrl Pts',(-38.4187069710969,-13.0721360087909,
40.0454055866277));
#26676=CARTESIAN_POINT('Ctrl Pts',(-38.2585765398713,-13.1527155106484,
39.9527626777571));
#26677=CARTESIAN_POINT('Ctrl Pts',(-38.4632970463556,-13.2848578326183,
40.2976226616114));
#26678=CARTESIAN_POINT('Ctrl Pts',(-38.3591702059311,-13.1766908654361,
40.2474509195671));
#26679=CARTESIAN_POINT('Ctrl Pts',(-38.2302344992928,-13.1988763557094,
40.1644744741364));
#26680=CARTESIAN_POINT('Ctrl Pts',(-38.3630673365025,-13.3151873395653,
40.4354786226433));
#26681=CARTESIAN_POINT('Ctrl Pts',(-38.2948355383256,-13.2202535090903,
40.3691988363216));
#26682=CARTESIAN_POINT('Ctrl Pts',(-38.1960676382616,-13.2140287022007,
40.2800075145154));
#26683=CARTESIAN_POINT('Ctrl Pts',(-38.2173764537126,-13.2823030560807,
40.5281034214334));
#26684=CARTESIAN_POINT('Ctrl Pts',(-38.187738902338,-13.2034487358311,40.4475707889938));
#26685=CARTESIAN_POINT('Ctrl Pts',(-38.1297266991476,-13.1975864244367,
40.346688751385));
#26686=CARTESIAN_POINT('Ctrl Pts',(-38.1790905589799,-13.2044045823054,
40.2785649063406));
#26687=CARTESIAN_POINT('Ctrl Pts',(-38.1856818137954,-13.2044045823054,
40.2663278736349));
#26688=CARTESIAN_POINT('Ctrl Pts',(-38.1915975569677,-13.2039200465849,
40.2538279098479));
#26689=CARTESIAN_POINT('Ctrl Pts',(-38.1969375577795,-13.2030865921358,
40.2411359927187));
#26690=CARTESIAN_POINT('Ctrl Pts',(-38.2024977186271,-13.2022187756393,
40.2279208073302));
#26691=CARTESIAN_POINT('Ctrl Pts',(-38.2074344665983,-13.2009724747263,
40.2144972565484));
#26692=CARTESIAN_POINT('Ctrl Pts',(-38.2118784236692,-13.199446062585,40.2009395294364));
#26693=CARTESIAN_POINT('Ctrl Pts',(-38.2165642026475,-13.1978365893588,
40.1866440464508));
#26694=CARTESIAN_POINT('Ctrl Pts',(-38.2207027909829,-13.1959155151288,
40.1721991593937));
#26695=CARTESIAN_POINT('Ctrl Pts',(-38.2244552324016,-13.1937414656796,
40.157689229008));
#26696=CARTESIAN_POINT('Ctrl Pts',(-38.2252951287549,-13.1932548554969,
40.1544415200478));
#26697=CARTESIAN_POINT('Ctrl Pts',(-38.226115686824,-13.1927553638524,40.1511905502003));
#26698=CARTESIAN_POINT('Ctrl Pts',(-38.2269187125116,-13.1922433006301,
40.1479372654108));
#26699=CARTESIAN_POINT('Ctrl Pts',(-38.2314857089357,-13.1893310763501,
40.1294350677485));
#26700=CARTESIAN_POINT('Ctrl Pts',(-38.2354089008154,-13.1860397456251,
40.1108869668906));
#26701=CARTESIAN_POINT('Ctrl Pts',(-38.2387936588154,-13.1824628010599,
40.09230074261));
#26702=CARTESIAN_POINT('Ctrl Pts',(-38.2423548715809,-13.1786993826273,
40.0727455782024));
#26703=CARTESIAN_POINT('Ctrl Pts',(-38.2453207997392,-13.1746195596086,
40.0531479638576));
#26704=CARTESIAN_POINT('Ctrl Pts',(-38.247815409911,-13.1702746943006,40.0335165509597));
#26705=CARTESIAN_POINT('Ctrl Pts',(-38.2486922977607,-13.1687474177584,
40.0266158545555));
#26706=CARTESIAN_POINT('Ctrl Pts',(-38.2495109068342,-13.1671869117775,
40.019710995831));
#26707=CARTESIAN_POINT('Ctrl Pts',(-38.2502764087794,-13.1655939279676,
40.0128024206661));
#26708=CARTESIAN_POINT('Ctrl Pts',(-38.2531564049936,-13.1596007526788,
39.9868107554002));
#26709=CARTESIAN_POINT('Ctrl Pts',(-38.2552721004159,-13.1531817886309,
39.9609037786925));
#26710=CARTESIAN_POINT('Ctrl Pts',(-38.2567195588292,-13.1464435609449,
39.9350831105545));
#26711=CARTESIAN_POINT('Ctrl Pts',(-38.2582169555115,-13.1394728599642,
39.9083716123535));
#26712=CARTESIAN_POINT('Ctrl Pts',(-38.2590000580469,-13.1321600180536,
39.8817522013977));
#26713=CARTESIAN_POINT('Ctrl Pts',(-38.2591711854353,-13.1245659628583,
39.8552280016203));
#26714=CARTESIAN_POINT('Ctrl Pts',(-38.2593494923536,-13.1166533043877,
39.8275909975895));
#26715=CARTESIAN_POINT('Ctrl Pts',(-38.2588642050127,-13.1084348255795,
39.8000570949086));
#26716=CARTESIAN_POINT('Ctrl Pts',(-38.2578137673921,-13.0999262547331,
39.7726355324511));
#26717=CARTESIAN_POINT('Ctrl Pts',(-38.2574542693167,-13.0970143113833,
39.763250873396));
#26718=CARTESIAN_POINT('Ctrl Pts',(-38.2570283786661,-13.094067983939,39.753879437865));
#26719=CARTESIAN_POINT('Ctrl Pts',(-38.2565393565581,-13.0910867263844,
39.744521822069));
#26720=CARTESIAN_POINT('Ctrl Pts',(-38.254737729453,-13.0801033488869,39.7100470325268));
#26721=CARTESIAN_POINT('Ctrl Pts',(-38.2520429901721,-13.0686901791307,
39.6757525940363));
#26722=CARTESIAN_POINT('Ctrl Pts',(-38.2485217298626,-13.0568974025755,
39.6416630585085));
#26723=CARTESIAN_POINT('Ctrl Pts',(-38.244892138822,-13.0447418240704,39.6065247665745));
#26724=CARTESIAN_POINT('Ctrl Pts',(-38.2403853064657,-13.0321818870426,
39.5716038765946));
#26725=CARTESIAN_POINT('Ctrl Pts',(-38.2350383815156,-13.0192318837648,
39.5369390751942));
#26726=CARTESIAN_POINT('Ctrl Pts',(-38.229762434248,-13.0064537851295,39.5027344312285));
#26727=CARTESIAN_POINT('Ctrl Pts',(-38.2236689920591,-12.9932945861615,
39.4687789762929));
#26728=CARTESIAN_POINT('Ctrl Pts',(-38.2167496847683,-12.9797471343051,
39.4351244052383));
#26729=CARTESIAN_POINT('Ctrl Pts',(-38.2096907485999,-12.9659263002422,
39.4007906982848));
#26730=CARTESIAN_POINT('Ctrl Pts',(-38.2017728575461,-12.9516999140197,
39.3667699506476));
#26731=CARTESIAN_POINT('Ctrl Pts',(-38.1929328601229,-12.9370593466235,
39.333134943979));
#26732=CARTESIAN_POINT('Ctrl Pts',(-38.1848265223924,-12.923633846796,39.3022914142165));
#26733=CARTESIAN_POINT('Ctrl Pts',(-38.1759442687234,-12.9098590019422,
39.2717724245339));
#26734=CARTESIAN_POINT('Ctrl Pts',(-38.1661935582769,-12.8957449858576,
39.241648555329));
#26735=CARTESIAN_POINT('Ctrl Pts',(-38.1653110755248,-12.894467604499,39.2389222109108));
#26736=CARTESIAN_POINT('Ctrl Pts',(-38.1644214502429,-12.8931874634454,
39.2361991124934));
#26737=CARTESIAN_POINT('Ctrl Pts',(-38.1635245965525,-12.8919045823054,
39.2334793180968));
#26738=CARTESIAN_POINT('Origin',(-38.1790905589799,-13.5169045823054,40.2785649063406));
#26739=CARTESIAN_POINT('Ctrl Pts',(-37.571637427794,-14.6563598281178,42.9623413980297));
#26740=CARTESIAN_POINT('Ctrl Pts',(-37.6481685929094,-14.766904582306,43.0141807834233));
#26741=CARTESIAN_POINT('Ctrl Pts',(-37.7683428080284,-14.7669045823054,
43.0948662445537));
#26742=CARTESIAN_POINT('Ctrl Pts',(-37.5504823732842,-14.6732979129414,
43.0240609128249));
#26743=CARTESIAN_POINT('Ctrl Pts',(-37.620400171357,-14.7669045823051,43.088122727466));
#26744=CARTESIAN_POINT('Ctrl Pts',(-37.7152507551813,-14.7669045823054,
43.1831284322925));
#26745=CARTESIAN_POINT('Ctrl Pts',(-37.5105015173806,-14.6836226395025,
43.0705954951548));
#26746=CARTESIAN_POINT('Ctrl Pts',(-37.5601429670254,-14.7669045823055,
43.1488125001359));
#26747=CARTESIAN_POINT('Ctrl Pts',(-37.6278053714458,-14.7669045823054,
43.2554532213409));
#26748=CARTESIAN_POINT('Ctrl Pts',(-37.4326597803442,-14.683707174412,43.0965368861083));
#26749=CARTESIAN_POINT('Ctrl Pts',(-37.4491318676269,-14.7669045823053,
43.1857463359048));
#26750=CARTESIAN_POINT('Ctrl Pts',(-37.4715757338329,-14.7669045823054,
43.3073250486046));
#26751=CARTESIAN_POINT('Ctrl Pts',(-37.4019081671593,-14.6805726740677,
43.0965521057182));
#26752=CARTESIAN_POINT('Ctrl Pts',(-37.4057521162803,-14.7669045823054,
43.1877618665153));
#26753=CARTESIAN_POINT('Ctrl Pts',(-37.4120037026109,-14.7669045823054,
43.313802830833));
#26754=CARTESIAN_POINT('Ctrl Pts',(-37.308677175366,-14.6635276241073,43.0722215122081));
#26755=CARTESIAN_POINT('Ctrl Pts',(-37.2781492406654,-14.7669045823054,
43.1635368742967));
#26756=CARTESIAN_POINT('Ctrl Pts',(-37.2365609420744,-14.7669045823054,
43.3000505843005));
#26757=CARTESIAN_POINT('Ctrl Pts',(-37.2461501425878,-14.6424796666936,
43.0248183412419));
#26758=CARTESIAN_POINT('Ctrl Pts',(-37.1977923649815,-14.7669045823054,
43.1070361827516));
#26759=CARTESIAN_POINT('Ctrl Pts',(-37.1254898316105,-14.7669045823054,
43.2482346286421));
#26760=CARTESIAN_POINT('Ctrl Pts',(-37.0594384684801,-14.5607785229691,
42.822087643319));
#26761=CARTESIAN_POINT('Ctrl Pts',(-36.9754363879768,-14.7669045823054,
42.8589117372199));
#26762=CARTESIAN_POINT('Ctrl Pts',(-36.8069422637988,-14.7669045823054,
43.0097426982014));
#26763=CARTESIAN_POINT('Ctrl Pts',(-36.9640663188338,-14.4859905466075,
42.6111924580297));
#26764=CARTESIAN_POINT('Ctrl Pts',(-36.9195590626158,-14.7669045823054,
42.5868389181748));
#26765=CARTESIAN_POINT('Ctrl Pts',(-36.667453837466,-14.7669045823054,42.7409248107066));
#26766=CARTESIAN_POINT('Ctrl Pts',(-36.9104618122751,-14.4183787521222,
42.408858845907));
#26767=CARTESIAN_POINT('Ctrl Pts',(-36.9508214922036,-14.7669045823054,
42.4006555962426));
#26768=CARTESIAN_POINT('Ctrl Pts',(-36.6071448023002,-14.7669045823054,
42.4758120956255));
#26769=CARTESIAN_POINT('Ctrl Pts',(-36.9407072321466,-14.4544045238109,
42.5103312284163));
#26770=CARTESIAN_POINT('Ctrl Pts',(-36.9503813816065,-14.4643868520269,
42.5396690097907));
#26771=CARTESIAN_POINT('Ctrl Pts',(-36.9608880608343,-14.474401186739,42.568722463887));
#26772=CARTESIAN_POINT('Ctrl Pts',(-36.9722124826523,-14.48440991971,42.5974253617278));
#26773=CARTESIAN_POINT('Ctrl Pts',(-36.9833401708954,-14.4942447759172,
42.6256296183318));
#26774=CARTESIAN_POINT('Ctrl Pts',(-36.9952567764507,-14.5040728389243,
42.6534969499852));
#26775=CARTESIAN_POINT('Ctrl Pts',(-37.0079962202933,-14.5138432176011,
42.6809634158137));
#26776=CARTESIAN_POINT('Ctrl Pts',(-37.0196774642178,-14.5228020212953,
42.7061483839371));
#26777=CARTESIAN_POINT('Ctrl Pts',(-37.0320511295469,-14.5317110776814,
42.7309973259379));
#26778=CARTESIAN_POINT('Ctrl Pts',(-37.0451828697107,-14.5405368969067,
42.7554423470322));
#26779=CARTESIAN_POINT('Ctrl Pts',(-37.0576149177858,-14.5488924543227,
42.7785848760231));
#26780=CARTESIAN_POINT('Ctrl Pts',(-37.0707272229527,-14.5571724059614,
42.8013660847167));
#26781=CARTESIAN_POINT('Ctrl Pts',(-37.0846026821019,-14.5653692837006,
42.8236990877515));
#26782=CARTESIAN_POINT('Ctrl Pts',(-37.0974382804467,-14.5729518673982,
42.8443584009825));
#26783=CARTESIAN_POINT('Ctrl Pts',(-37.1109279894093,-14.5804628051681,
42.864634363072));
#26784=CARTESIAN_POINT('Ctrl Pts',(-37.1251480886583,-14.5879251019716,
42.8844266395982));
#26785=CARTESIAN_POINT('Ctrl Pts',(-37.1324432310159,-14.5917533816863,
42.8945803995904));
#26786=CARTESIAN_POINT('Ctrl Pts',(-37.1399306955635,-14.5955693937985,
42.9046063116132));
#26787=CARTESIAN_POINT('Ctrl Pts',(-37.1476204401308,-14.5993802185554,
42.9144870863799));
#26788=CARTESIAN_POINT('Ctrl Pts',(-37.157835260641,-14.6044424011217,42.9276124041145));
#26789=CARTESIAN_POINT('Ctrl Pts',(-37.1683738566588,-14.6095732512801,
42.940512250732));
#26790=CARTESIAN_POINT('Ctrl Pts',(-37.1793254324901,-14.6146451518329,
42.9530852762723));
#26791=CARTESIAN_POINT('Ctrl Pts',(-37.189587205736,-14.619397590587,42.9648663696143));
#26792=CARTESIAN_POINT('Ctrl Pts',(-37.2002124359805,-14.624097891655,42.976360600664));
#26793=CARTESIAN_POINT('Ctrl Pts',(-37.2112872605342,-14.6286695523061,
42.9874527708991));
#26794=CARTESIAN_POINT('Ctrl Pts',(-37.2219162798294,-14.6330571856303,
42.9980984376436));
#26795=CARTESIAN_POINT('Ctrl Pts',(-37.2329603033943,-14.6373259480376,
43.0083738395466));
#26796=CARTESIAN_POINT('Ctrl Pts',(-37.2444954462343,-14.6414408657884,
43.0181454813071));
#26797=CARTESIAN_POINT('Ctrl Pts',(-37.2557075809083,-14.6454405572214,
43.0276434966264));
#26798=CARTESIAN_POINT('Ctrl Pts',(-37.2673847753206,-14.6492945993133,
43.0366655113334));
#26799=CARTESIAN_POINT('Ctrl Pts',(-37.2795829118597,-14.6530074411929,
43.045058089822));
#26800=CARTESIAN_POINT('Ctrl Pts',(-37.2910154425439,-14.6564872496521,
43.0529239151293));
#26801=CARTESIAN_POINT('Ctrl Pts',(-37.3029064669486,-14.6598432010014,
43.0602363732956));
#26802=CARTESIAN_POINT('Ctrl Pts',(-37.3152758152603,-14.6631120254243,
43.0668456988466));
#26803=CARTESIAN_POINT('Ctrl Pts',(-37.316104157274,-14.6633309298109,43.0672883076161));
#26804=CARTESIAN_POINT('Ctrl Pts',(-37.3169346310621,-14.6635494557759,
43.067727755555));
#26805=CARTESIAN_POINT('Ctrl Pts',(-37.3177672364761,-14.6637676196426,
43.0681639945637));
#26806=CARTESIAN_POINT('Ctrl Pts',(-37.3288904156748,-14.6666821764584,
43.0739919228776));
#26807=CARTESIAN_POINT('Ctrl Pts',(-37.3404597867255,-14.6694736866496,
43.0792128120357));
#26808=CARTESIAN_POINT('Ctrl Pts',(-37.3523931238171,-14.6719975663698,
43.0834732187685));
#26809=CARTESIAN_POINT('Ctrl Pts',(-37.363947582839,-14.6744413140473,43.0875983595094));
#26810=CARTESIAN_POINT('Ctrl Pts',(-37.3758439124062,-14.6766346712664,
43.0908223244708));
#26811=CARTESIAN_POINT('Ctrl Pts',(-37.3879640412811,-14.6784666962726,
43.0928188912063));
#26812=CARTESIAN_POINT('Ctrl Pts',(-37.3996182825084,-14.6802282997653,
43.0947387115814));
#26813=CARTESIAN_POINT('Ctrl Pts',(-37.411479676887,-14.6816565741044,43.0955228683507));
#26814=CARTESIAN_POINT('Ctrl Pts',(-37.4233961687224,-14.6826626743679,
43.0948873632353));
#26815=CARTESIAN_POINT('Ctrl Pts',(-37.4263170846554,-14.6829092850592,
43.0947315911304));
#26816=CARTESIAN_POINT('Ctrl Pts',(-37.4292410753172,-14.6831305465446,
43.0944905860586));
#26817=CARTESIAN_POINT('Ctrl Pts',(-37.4321654362444,-14.6833251552392,
43.094160314464));
#26818=CARTESIAN_POINT('Ctrl Pts',(-37.4416164879093,-14.6839540984074,
43.0930929312029));
#26819=CARTESIAN_POINT('Ctrl Pts',(-37.4508975843209,-14.6841943737355,
43.090998399424));
#26820=CARTESIAN_POINT('Ctrl Pts',(-37.4598652509752,-14.6841331258666,
43.0879880811904));
#26821=CARTESIAN_POINT('Ctrl Pts',(-37.4689847795451,-14.6840708408026,
43.0849267850702));
#26822=CARTESIAN_POINT('Ctrl Pts',(-37.4777791878974,-14.6836965195602,
43.0809189561397));
#26823=CARTESIAN_POINT('Ctrl Pts',(-37.4861222057687,-14.6830632794737,
43.0761109723373));
#26824=CARTESIAN_POINT('Ctrl Pts',(-37.4946188905762,-14.682418375974,43.0712144320734));
#26825=CARTESIAN_POINT('Ctrl Pts',(-37.5026467486571,-14.6815043446902,
43.0654887721282));
#26826=CARTESIAN_POINT('Ctrl Pts',(-37.5101105739052,-14.680343837413,43.0591084748772));
#26827=CARTESIAN_POINT('Ctrl Pts',(-37.5178759953978,-14.6791364366697,
43.0524703642896));
#26828=CARTESIAN_POINT('Ctrl Pts',(-37.5250305556585,-14.6776614503336,
43.0451245148125));
#26829=CARTESIAN_POINT('Ctrl Pts',(-37.5315160929354,-14.6759191474477,
43.0372757278879));
#26830=CARTESIAN_POINT('Ctrl Pts',(-37.5321802112215,-14.6757407358286,
43.0364720129916));
#26831=CARTESIAN_POINT('Ctrl Pts',(-37.5328373566078,-14.6755595065434,
43.0356630246841));
#26832=CARTESIAN_POINT('Ctrl Pts',(-37.5334874951132,-14.6753754510087,
43.0348489820804));
#26833=CARTESIAN_POINT('Origin',(0.0835265683620477,-14.4544045823054,0.0824317919394229));
#26834=CARTESIAN_POINT('Origin',(-9.75726988530523,-14.4544045823054,-19.1035039790228));
#26835=CARTESIAN_POINT('Origin',(5.15768816523998,-14.4544045823054,-15.3054474424773));
#26836=CARTESIAN_POINT('Origin',(-9.84678298317079,-14.4544045823054,-20.2531800132168));
#26837=CARTESIAN_POINT('Origin',(0.0835265683620477,-10.7044045823054,0.0824317919394229));
#26838=CARTESIAN_POINT('Origin',(-37.87826784707,-10.7044045823054,-29.4965774842428));
#26839=CARTESIAN_POINT('Origin',(-4.99063502851588,-11.3294045823054,15.4703110263562));
#26840=CARTESIAN_POINT('Origin',(18.7518431265311,-11.3294045823054,23.2994061884498));
#26841=CARTESIAN_POINT('Ctrl Pts',(38.3508237177256,-11.3294045823054,29.4331291796839));
#26842=CARTESIAN_POINT('Ctrl Pts',(38.3508237177256,-11.3124780874426,29.4331291796839));
#26843=CARTESIAN_POINT('Ctrl Pts',(38.3494530102577,-11.2956902155653,29.4341292951345));
#26844=CARTESIAN_POINT('Ctrl Pts',(38.3468401936668,-11.2792729854166,29.4360772676558));
#26845=CARTESIAN_POINT('Ctrl Pts',(38.3442080910596,-11.2627345745579,29.4380396187715));
#26846=CARTESIAN_POINT('Ctrl Pts',(38.3403156398042,-11.2465729047032,29.4409633712592));
#26847=CARTESIAN_POINT('Ctrl Pts',(38.3353075372331,-11.230993405314,29.444754978997));
#26848=CARTESIAN_POINT('Ctrl Pts',(38.3302312794146,-11.2152018845814,29.448598186709));
#26849=CARTESIAN_POINT('Ctrl Pts',(38.3240089967403,-11.2000089946043,29.4533324285803));
#26850=CARTESIAN_POINT('Ctrl Pts',(38.3168021619072,-11.1855875760929,29.4588275743199));
#26851=CARTESIAN_POINT('Ctrl Pts',(38.309537501841,-11.1710504449412,29.4643668112716));
#26852=CARTESIAN_POINT('Ctrl Pts',(38.3012726649942,-11.1572975033337,29.4706784891979));
#26853=CARTESIAN_POINT('Ctrl Pts',(38.2921805812085,-11.1444582968067,29.4776064573043));
#26854=CARTESIAN_POINT('Ctrl Pts',(38.2829617933224,-11.1314401675872,29.4846309711517));
#26855=CARTESIAN_POINT('Ctrl Pts',(38.2728927915826,-11.1193615571096,29.4922883129586));
#26856=CARTESIAN_POINT('Ctrl Pts',(38.2621578342495,-11.1083055247257,29.5004035894501));
#26857=CARTESIAN_POINT('Ctrl Pts',(38.2586229712668,-11.1046649364685,29.5030758302028));
#26858=CARTESIAN_POINT('Ctrl Pts',(38.2550159150995,-11.1011348042002,29.5057976770622));
#26859=CARTESIAN_POINT('Ctrl Pts',(38.251343266964,-11.0977168667273,29.5085628175253));
#26860=CARTESIAN_POINT('Ctrl Pts',(38.237970490606,-11.0852715379768,29.5186311942514));
#26861=CARTESIAN_POINT('Ctrl Pts',(38.2237563987941,-11.0742682117852,29.5293337237824));
#26862=CARTESIAN_POINT('Ctrl Pts',(38.2089071620523,-11.0647125800551,29.5404697723536));
#26863=CARTESIAN_POINT('Ctrl Pts',(38.1922829478517,-11.054014732653,29.5529369489509));
#26864=CARTESIAN_POINT('Ctrl Pts',(38.1748627193941,-11.0451301475312,29.5659473342625));
#26865=CARTESIAN_POINT('Ctrl Pts',(38.1569165881815,-11.0380420023619,29.5792775735416));
#26866=CARTESIAN_POINT('Ctrl Pts',(38.136953098194,-11.0301570653,29.5941062903957));
#26867=CARTESIAN_POINT('Ctrl Pts',(38.116338530399,-11.0244934293336,29.6093317055714));
#26868=CARTESIAN_POINT('Ctrl Pts',(38.0954239674044,-11.0210242012062,29.6247092634801));
#26869=CARTESIAN_POINT('Ctrl Pts',(38.0788552940599,-11.0182758527174,29.6368914799525));
#26870=CARTESIAN_POINT('Ctrl Pts',(38.0620977574343,-11.0169045823054,29.6491709647271));
#26871=CARTESIAN_POINT('Ctrl Pts',(38.0453209837941,-11.0169045823054,29.6614410681217));
#26872=CARTESIAN_POINT('Origin',(38.4486874072517,-14.7669045823054,29.1363482027458));
#26873=CARTESIAN_POINT('Origin',(38.4486874072517,-11.3294045823054,29.1363482027458));
#26874=CARTESIAN_POINT('Origin',(-22.4718276789325,-12.8919045823054,-7.35520861204973));
#26875=CARTESIAN_POINT('Origin',(-35.8042963200226,-12.8919045823054,33.0767747666364));
#26876=CARTESIAN_POINT('Origin',(0.0835265683620477,-13.5169045823054,0.0824317919394229));
#26877=CARTESIAN_POINT('Origin',(-36.9176881394302,-13.5169045823054,41.4426433113705));
#26878=CARTESIAN_POINT('Ctrl Pts',(-37.1002562688466,-14.9232028613467,
42.9941789068619));
#26879=CARTESIAN_POINT('Ctrl Pts',(-37.1882368306857,-14.6181128259927,
43.2609883560109));
#26880=CARTESIAN_POINT('Ctrl Pts',(-37.5425880812871,-14.7022319922259,
43.0625772974519));
#26881=CARTESIAN_POINT('Ctrl Pts',(-36.9406416502711,-14.45386212998,42.510132345121));
#26882=CARTESIAN_POINT('Ctrl Pts',(-37.0285175912917,-14.147074607213,42.7766245216622));
#26883=CARTESIAN_POINT('Ctrl Pts',(-37.3835541595816,-14.232891259592,42.5780223744643));
#26884=CARTESIAN_POINT('Ctrl Pts',(-36.7808584715544,-13.9850662226631,
42.0255746086673));
#26885=CARTESIAN_POINT('Ctrl Pts',(-36.8688690141397,-13.6772499732338,
42.2924749773334));
#26886=CARTESIAN_POINT('Ctrl Pts',(-37.2243639950202,-13.7640953522129,
42.0929401326293));
#26887=CARTESIAN_POINT('Ctrl Pts',(-36.6209071624921,-13.5169045823054,
41.5405070008967));
#26888=CARTESIAN_POINT('Ctrl Pts',(-36.7093350047365,-13.2088427643879,
41.8086728705558));
#26889=CARTESIAN_POINT('Ctrl Pts',(-37.0650186795419,-13.2959337131846,
41.6073303993598));
#26890=CARTESIAN_POINT('Origin',(-36.9176881394302,-13.5169045823054,41.4426433113705));
#26891=CARTESIAN_POINT('Origin',(-10.0425103622231,-14.4544045823054,-19.6596180593406));
#26892=CARTESIAN_POINT('Origin',(-10.0425103622231,-14.4544045823054,-19.6596180593406));
#26893=CARTESIAN_POINT('Ctrl Pts',(-38.5307586915594,-11.3294045823054,
-29.1601464137424));
#26894=CARTESIAN_POINT('Ctrl Pts',(-38.3959057211593,-11.3294045823054,
-29.3382172743398));
#26895=CARTESIAN_POINT('Ctrl Pts',(-38.1837705810015,-11.3294045823054,
-29.2682655958051));
#26896=CARTESIAN_POINT('Ctrl Pts',(-38.530758641258,-11.1601003758277,-29.1601464801644));
#26897=CARTESIAN_POINT('Ctrl Pts',(-38.3959056833756,-11.2236230318997,
-29.3382173235993));
#26898=CARTESIAN_POINT('Ctrl Pts',(-38.1837705555596,-11.2447524820092,
-29.2682655874156));
#26899=CARTESIAN_POINT('Ctrl Pts',(-38.4840830247557,-10.9943058431436,
-29.2219436452516));
#26900=CARTESIAN_POINT('Ctrl Pts',(-38.3590718330862,-11.120480985332,-29.3862883502537));
#26901=CARTESIAN_POINT('Ctrl Pts',(-38.148800374239,-11.1618552084332,-29.2950794305781));
#26902=CARTESIAN_POINT('Ctrl Pts',(-38.3328185949133,-10.7673610427476,
-29.4199639376802));
#26903=CARTESIAN_POINT('Ctrl Pts',(-38.2519922408775,-11.0035905561212,
-29.5250467467008));
#26904=CARTESIAN_POINT('Ctrl Pts',(-38.0351381216391,-11.0483828168177,
-29.3807494825232));
#26905=CARTESIAN_POINT('Ctrl Pts',(-38.2284284200153,-10.7044046130696,
-29.5556172851081));
#26906=CARTESIAN_POINT('Ctrl Pts',(-38.180551033523,-10.9913613137611,-29.6170632772379));
#26907=CARTESIAN_POINT('Ctrl Pts',(-37.9565673174692,-11.0169045823054,
-29.4393112525611));
#26908=CARTESIAN_POINT('Ctrl Pts',(-38.1247730056117,-10.7044045823054,
-29.6886489730492));
#26909=CARTESIAN_POINT('Ctrl Pts',(-38.1247730056117,-11.0169045823054,
-29.6886489730492));
#26910=CARTESIAN_POINT('Ctrl Pts',(-37.87826784707,-11.0169045823054,-29.4965774842428));
#26911=CARTESIAN_POINT('Ctrl Pts',(-37.87826784707,-11.0169045823054,-29.4965774842428));
#26912=CARTESIAN_POINT('Ctrl Pts',(-37.8972057124971,-11.0169045823054,
-29.4827268135568));
#26913=CARTESIAN_POINT('Ctrl Pts',(-37.9161246770386,-11.0187415076311,
-29.468841193656));
#26914=CARTESIAN_POINT('Ctrl Pts',(-37.9347738006665,-11.0223262068999,
-29.4551060632967));
#26915=CARTESIAN_POINT('Ctrl Pts',(-37.9525585139756,-11.0257447508523,
-29.4420075734922));
#26916=CARTESIAN_POINT('Ctrl Pts',(-37.9700990191786,-11.0307535195289,
-29.4290449639884));
#26917=CARTESIAN_POINT('Ctrl Pts',(-37.9871678607578,-11.0373176231361,
-29.4163864282423));
#26918=CARTESIAN_POINT('Ctrl Pts',(-38.0016526834004,-11.0428879997851,
-29.4056442437568));
#26919=CARTESIAN_POINT('Ctrl Pts',(-38.0158017303236,-11.0495814926574,
-29.3951108985677));
#26920=CARTESIAN_POINT('Ctrl Pts',(-38.0294827462888,-11.0574216164515,
-29.3848835313139));
#26921=CARTESIAN_POINT('Ctrl Pts',(-38.0323151592383,-11.0590447757414,
-29.3827661353894));
#26922=CARTESIAN_POINT('Ctrl Pts',(-38.035127405604,-11.0607171987449,-29.380661935915));
#26923=CARTESIAN_POINT('Ctrl Pts',(-38.0379181304706,-11.0624392724587,
-29.3785719346032));
#26924=CARTESIAN_POINT('Ctrl Pts',(-38.0505386215989,-11.0702270039859,
-29.369120324618));
#26925=CARTESIAN_POINT('Ctrl Pts',(-38.0627212545858,-11.0790298901558,
-29.3599545277751));
#26926=CARTESIAN_POINT('Ctrl Pts',(-38.0743506094951,-11.0888942095793,
-29.3511988246088));
#26927=CARTESIAN_POINT('Ctrl Pts',(-38.0777138589611,-11.0917470047078,
-29.3486666451176));
#26928=CARTESIAN_POINT('Ctrl Pts',(-38.0810305830642,-11.0946887229259,
-29.3461689091715));
#26929=CARTESIAN_POINT('Ctrl Pts',(-38.0842973331891,-11.0977208509785,
-29.3437090106853));
#26930=CARTESIAN_POINT('Ctrl Pts',(-38.0868926890118,-11.1001298051059,
-29.3417546794339));
#26931=CARTESIAN_POINT('Ctrl Pts',(-38.0894544429346,-11.1025951245287,
-29.3398243956254));
#26932=CARTESIAN_POINT('Ctrl Pts',(-38.0919798954887,-11.1051169477604,
-29.3379202081949));
#26933=CARTESIAN_POINT('Ctrl Pts',(-38.1045664389756,-11.117685403153,-29.3284299733211));
#26934=CARTESIAN_POINT('Ctrl Pts',(-38.1162463847602,-11.1317057213303,
-29.3196014738052));
#26935=CARTESIAN_POINT('Ctrl Pts',(-38.1267717929096,-11.1469740767481,
-29.3116302992635));
#26936=CARTESIAN_POINT('Ctrl Pts',(-38.1376151029358,-11.1627035866192,
-29.3034183690845));
#26937=CARTESIAN_POINT('Ctrl Pts',(-38.1472329395675,-11.1797576681432,
-29.296116441489));
#26938=CARTESIAN_POINT('Ctrl Pts',(-38.155340711547,-11.1978608317538,-29.2899503483155));
#26939=CARTESIAN_POINT('Ctrl Pts',(-38.1636385340936,-11.2163883433257,
-29.2836397185779));
#26940=CARTESIAN_POINT('Ctrl Pts',(-38.1703544452564,-11.2360145397413,
-29.2785189731724));
#26941=CARTESIAN_POINT('Ctrl Pts',(-38.1751722595047,-11.2563909917677,
-29.2748403601573));
#26942=CARTESIAN_POINT('Ctrl Pts',(-38.1801949750669,-11.2776340529195,
-29.2710052959796));
#26943=CARTESIAN_POINT('Ctrl Pts',(-38.1831544089492,-11.2996924044415,
-29.268737876305));
#26944=CARTESIAN_POINT('Ctrl Pts',(-38.1836843650225,-11.3221161967233,
-29.2683316856799));
#26945=CARTESIAN_POINT('Ctrl Pts',(-38.1837416869597,-11.3245416339992,
-29.2682877506545));
#26946=CARTESIAN_POINT('Ctrl Pts',(-38.1837705810015,-11.3269712973028,
-29.2682655958051));
#26947=CARTESIAN_POINT('Ctrl Pts',(-38.1837705810015,-11.3294045823054,
-29.2682655958051));
#26948=CARTESIAN_POINT('Ctrl Pts',(38.6963701433757,-11.3806731536973,29.3269198996342));
#26949=CARTESIAN_POINT('Ctrl Pts',(38.5618177595307,-11.3615458683564,29.5045706843909));
#26950=CARTESIAN_POINT('Ctrl Pts',(38.3497262416573,-11.3550383295792,29.4339522003598));
#26951=CARTESIAN_POINT('Ctrl Pts',(38.706929772342,-11.1940655928605,29.3129266693747));
#26952=CARTESIAN_POINT('Ctrl Pts',(38.5701244778425,-11.2445867749092,29.4937245996208));
#26953=CARTESIAN_POINT('Ctrl Pts',(38.3576357632337,-11.2617365126274,29.4278794464172));
#26954=CARTESIAN_POINT('Ctrl Pts',(38.6587619695313,-11.0057469829272,29.3768242824327));
#26955=CARTESIAN_POINT('Ctrl Pts',(38.5312471098703,-11.1260887992138,29.5445145967177));
#26956=CARTESIAN_POINT('Ctrl Pts',(38.3215665264224,-11.1675791668517,29.4556168052334));
#26957=CARTESIAN_POINT('Ctrl Pts',(38.4922459235859,-10.755919902964,29.5948104682567));
#26958=CARTESIAN_POINT('Ctrl Pts',(38.4133590232755,-10.9974050091189,29.6972789722255));
#26959=CARTESIAN_POINT('Ctrl Pts',(38.1964443230947,-11.0426657521647,29.5499206069573));
#26960=CARTESIAN_POINT('Ctrl Pts',(38.374138394728,-10.6922226875528,29.7482085696384));
#26961=CARTESIAN_POINT('Ctrl Pts',(38.3324029890132,-10.989329898887,29.8015013235227));
#26962=CARTESIAN_POINT('Ctrl Pts',(38.1075385459645,-11.0108152118554,29.6161302248789));
#26963=CARTESIAN_POINT('Ctrl Pts',(38.2605248298428,-10.7063374044318,29.8936321146768));
#26964=CARTESIAN_POINT('Ctrl Pts',(38.2746985341136,-11.0262754940985,29.8754832605275));
#26965=CARTESIAN_POINT('Ctrl Pts',(38.0216496713564,-11.0178704045121,29.6786922008474));
#26966=CARTESIAN_POINT('Origin',(38.0453209837941,-10.7044045823054,29.6614410681217));
#26967=CARTESIAN_POINT('Origin',(-35.8042963200226,-12.8919045823054,33.0767747666364));
#26968=CARTESIAN_POINT('Origin',(-35.8042963200226,-12.8919045823054,33.0767747666364));
#26969=CARTESIAN_POINT('Origin',(-36.9176881394302,-13.5169045823054,41.4426433113705));
#26970=CARTESIAN_POINT('Origin',(-36.9176881394301,-13.5169045823054,41.4426433113705));
#26971=CARTESIAN_POINT('Origin',(-10.0425103622231,-11.0169045823054,-19.6596180593406));
#26972=CARTESIAN_POINT('Origin',(-10.0425103622231,-11.3294045823054,-19.6596180593406));
#26973=CARTESIAN_POINT('Origin',(5.15768816523998,-11.3294045823054,-15.3054474424773));
#26974=CARTESIAN_POINT('Origin',(-9.84678298317079,-11.3294045823054,-20.2531800132168));
#26975=CARTESIAN_POINT('Origin',(0.0835265683620477,-10.7044045823054,0.0824317919394229));
#26976=CARTESIAN_POINT('Origin',(34.1908936222416,-10.7044045823054,34.0339139046828));
#26977=CARTESIAN_POINT('Origin',(33.692255281224,-14.7669045823054,34.5275908031162));
#26978=CARTESIAN_POINT('Origin',(33.692255281224,-11.3294045823054,34.5275908031162));
#26979=CARTESIAN_POINT('Origin',(33.692255281224,-12.8919045823054,34.5275908031162));
#26980=CARTESIAN_POINT('Origin',(-6.86479538799601,-13.5169045823054,21.1538811545436));
#26981=CARTESIAN_POINT('Origin',(34.3599945679822,-13.5169045823054,34.7477781982718));
#26982=CARTESIAN_POINT('Origin',(41.4437380877936,-13.5169045823054,37.0836464997312));
#26983=CARTESIAN_POINT('Ctrl Pts',(34.4578582575083,-13.5169045823054,34.4509972213337));
#26984=CARTESIAN_POINT('Ctrl Pts',(34.4578582575083,-13.2044045823054,34.4509972213337));
#26985=CARTESIAN_POINT('Ctrl Pts',(34.3599945679822,-13.2044045823054,34.7477781982718));
#26986=CARTESIAN_POINT('Ctrl Pts',(34.3745296971238,-13.5169045582439,34.4235195829545));
#26987=CARTESIAN_POINT('Ctrl Pts',(34.4061312136231,-13.1861191316369,34.43394020031));
#26988=CARTESIAN_POINT('Ctrl Pts',(34.3041321680135,-13.2044045823054,34.7480782775218));
#26989=CARTESIAN_POINT('Ctrl Pts',(34.2933711160147,-13.5027466839947,34.3967574964286));
#26990=CARTESIAN_POINT('Ctrl Pts',(34.3629706115748,-13.1578432798925,34.4197079681703));
#26991=CARTESIAN_POINT('Ctrl Pts',(34.2496387413663,-13.1973256316196,34.7484206608821));
#26992=CARTESIAN_POINT('Ctrl Pts',(34.1358739983332,-13.4449866817213,34.3448227357001));
#26993=CARTESIAN_POINT('Ctrl Pts',(34.2950839932164,-13.0892356355758,34.397322318623));
#26994=CARTESIAN_POINT('Ctrl Pts',(34.1437376255259,-13.1684456335483,34.7491725375223));
#26995=CARTESIAN_POINT('Ctrl Pts',(34.064061118804,-13.4031153721667,34.3211423993836));
#26996=CARTESIAN_POINT('Ctrl Pts',(34.2738703798607,-13.0503322093643,34.390327118012));
#26997=CARTESIAN_POINT('Ctrl Pts',(34.0953731108843,-13.1475099673761,34.7495603170485));
#26998=CARTESIAN_POINT('Ctrl Pts',(33.9360538509793,-13.2902331116008,34.2789319327805));
#26999=CARTESIAN_POINT('Ctrl Pts',(34.253604081193,-12.9767617731724,34.3836442949382));
#27000=CARTESIAN_POINT('Ctrl Pts',(34.0090703956612,-13.0910688568131,34.750304648432));
#27001=CARTESIAN_POINT('Ctrl Pts',(33.8839249013386,-13.222452827101,34.2617423831146));
#27002=CARTESIAN_POINT('Ctrl Pts',(34.2570256950654,-12.9460615526393,34.3847725739844));
#27003=CARTESIAN_POINT('Ctrl Pts',(33.9738736850488,-13.0571787063092,34.7506372725395));
#27004=CARTESIAN_POINT('Ctrl Pts',(33.8098868212263,-13.0654169357612,34.2373282856884));
#27005=CARTESIAN_POINT('Ctrl Pts',(34.2704028238453,-12.9052920386068,34.389183689519));
#27006=CARTESIAN_POINT('Ctrl Pts',(33.9238607907023,-12.9786607574272,34.7511230809577));
#27007=CARTESIAN_POINT('Ctrl Pts',(33.7901189534223,-12.9802875861308,34.2308098204642));
#27008=CARTESIAN_POINT('Ctrl Pts',(34.2787581405614,-12.8977806170664,34.3919388597773));
#27009=CARTESIAN_POINT('Ctrl Pts',(33.9104937733009,-12.9360960854268,34.7512606727365));
#27010=CARTESIAN_POINT('Ctrl Pts',(33.7901189707501,-12.8919045823054,34.2308098261781));
#27011=CARTESIAN_POINT('Ctrl Pts',(34.2787581354395,-12.8919045823054,34.3919388580886));
#27012=CARTESIAN_POINT('Ctrl Pts',(33.9104937793594,-12.8919045823054,34.7512606668251));
#27013=CARTESIAN_POINT('Ctrl Pts',(33.9104937793594,-12.8919045823054,34.7512606668251));
#27014=CARTESIAN_POINT('Ctrl Pts',(33.9104937793594,-12.9051774018388,34.7512606668251));
#27015=CARTESIAN_POINT('Ctrl Pts',(33.9117040823358,-12.9183340038153,34.7512482101544));
#27016=CARTESIAN_POINT('Ctrl Pts',(33.9140678651876,-12.9312552225994,34.7512241292996));
#27017=CARTESIAN_POINT('Ctrl Pts',(33.9164761535976,-12.9444197234828,34.7511995950479));
#27018=CARTESIAN_POINT('Ctrl Pts',(33.9200814988752,-12.9573395068935,34.7511630014824));
#27019=CARTESIAN_POINT('Ctrl Pts',(33.9247701430341,-12.9698996728684,34.7511157321652));
#27020=CARTESIAN_POINT('Ctrl Pts',(33.9296145840165,-12.9828771948836,34.7510668921574));
#27021=CARTESIAN_POINT('Ctrl Pts',(33.9356152049093,-12.9954703520459,34.7510066623665));
#27022=CARTESIAN_POINT('Ctrl Pts',(33.9425940244808,-13.0075707507672,34.7509369943112));
#27023=CARTESIAN_POINT('Ctrl Pts',(33.9446073176688,-13.0110615488982,34.7509168960382));
#27024=CARTESIAN_POINT('Ctrl Pts',(33.9467017142206,-13.0145114746282,34.7508960145068));
#27025=CARTESIAN_POINT('Ctrl Pts',(33.9488722314559,-13.0179182754031,34.7508744014892));
#27026=CARTESIAN_POINT('Ctrl Pts',(33.9522032468625,-13.0231465710756,34.7508412327616));
#27027=CARTESIAN_POINT('Ctrl Pts',(33.9556878747932,-13.0282366579925,34.7508066183155));
#27028=CARTESIAN_POINT('Ctrl Pts',(33.9593070766984,-13.0331862397833,34.7507707786108));
#27029=CARTESIAN_POINT('Ctrl Pts',(33.9667645107392,-13.0433849467635,34.7506969302207));
#27030=CARTESIAN_POINT('Ctrl Pts',(33.9748160481855,-13.0530328316013,34.7506263796451));
#27031=CARTESIAN_POINT('Ctrl Pts',(33.9833730071236,-13.0621635675362,34.7505475422118));
#27032=CARTESIAN_POINT('Ctrl Pts',(33.9928680087852,-13.0722952455658,34.7504600623531));
#27033=CARTESIAN_POINT('Ctrl Pts',(34.0029431003418,-13.0817557997662,34.7503681518668));
#27034=CARTESIAN_POINT('Ctrl Pts',(34.0135255597351,-13.0906427434663,34.7502724193904));
#27035=CARTESIAN_POINT('Ctrl Pts',(34.0246022815835,-13.099944759169,34.75017221565));
#27036=CARTESIAN_POINT('Ctrl Pts',(34.0362351994585,-13.1086184489897,34.7500678136454));
#27037=CARTESIAN_POINT('Ctrl Pts',(34.0483916685675,-13.1167513951577,34.7499593789485));
#27038=CARTESIAN_POINT('Ctrl Pts',(34.0496640078893,-13.1176026182488,34.7499480297872));
#27039=CARTESIAN_POINT('Ctrl Pts',(34.0509421236522,-13.1184478958543,34.7499366360809));
#27040=CARTESIAN_POINT('Ctrl Pts',(34.0522260065119,-13.119287313057,34.7499251977801));
#27041=CARTESIAN_POINT('Ctrl Pts',(34.0586407621694,-13.1234813531983,34.7498680477804));
#27042=CARTESIAN_POINT('Ctrl Pts',(34.0651387821861,-13.1274936111504,34.7498103139349));
#27043=CARTESIAN_POINT('Ctrl Pts',(34.0717272061634,-13.1313379140666,34.7497518934144));
#27044=CARTESIAN_POINT('Ctrl Pts',(34.0912832509352,-13.1427487401161,34.7495784871006));
#27045=CARTESIAN_POINT('Ctrl Pts',(34.1115096164517,-13.1526155242428,34.7494099515472));
#27046=CARTESIAN_POINT('Ctrl Pts',(34.1323508455064,-13.1611451738774,34.7492466433572));
#27047=CARTESIAN_POINT('Ctrl Pts',(34.1531920745612,-13.1696748235119,34.7490833351672));
#27048=CARTESIAN_POINT('Ctrl Pts',(34.1746485137788,-13.1768668275904,34.7489252300396));
#27049=CARTESIAN_POINT('Ctrl Pts',(34.1966978194881,-13.1828814286543,34.7487720524465));
#27050=CARTESIAN_POINT('Ctrl Pts',(34.2203748666754,-13.1893400444075,34.7486075668547));
#27051=CARTESIAN_POINT('Ctrl Pts',(34.2441289381238,-13.19426816731,34.7484530498353));
#27052=CARTESIAN_POINT('Ctrl Pts',(34.268032456907,-13.1977771930991,34.7483060606209));
#27053=CARTESIAN_POINT('Ctrl Pts',(34.2923821257301,-13.201351713513,34.7481563279091));
#27054=CARTESIAN_POINT('Ctrl Pts',(34.3168869206479,-13.2034535833856,34.7480143798219));
#27055=CARTESIAN_POINT('Ctrl Pts',(34.3416346865736,-13.2041479208638,34.7478780637107));
#27056=CARTESIAN_POINT('Ctrl Pts',(34.3477393394683,-13.2043191964977,34.7478444379465));
#27057=CARTESIAN_POINT('Ctrl Pts',(34.3538588277594,-13.2044045823054,34.74781115797));
#27058=CARTESIAN_POINT('Ctrl Pts',(34.3599945679822,-13.2044045823054,34.7477781982718));
#27059=CARTESIAN_POINT('Origin',(0.0835265683620477,-12.8919045823054,0.0824317919394229));
#27060=CARTESIAN_POINT('Ctrl Pts',(-34.5818198379706,-13.2044045823054,
34.3588997915592));
#27061=CARTESIAN_POINT('Ctrl Pts',(-34.5819536007302,-13.2044045823054,
34.3339986672398));
#27062=CARTESIAN_POINT('Ctrl Pts',(-34.5820925794552,-13.2030022087212,
34.3093644005129));
#27063=CARTESIAN_POINT('Ctrl Pts',(-34.5822388280734,-13.2001447338013,
34.2849062065081));
#27064=CARTESIAN_POINT('Ctrl Pts',(-34.5823824111376,-13.1973393397405,
34.2608937920094));
#27065=CARTESIAN_POINT('Ctrl Pts',(-34.5825330278843,-13.1931314656529,
34.2370510471072));
#27066=CARTESIAN_POINT('Ctrl Pts',(-34.5826931179797,-13.1874220362842,
34.2133024907471));
#27067=CARTESIAN_POINT('Ctrl Pts',(-34.5827329267351,-13.1860023027453,
34.207397063114));
#27068=CARTESIAN_POINT('Ctrl Pts',(-34.5827733226246,-13.1844894768729,
34.2014975126608));
#27069=CARTESIAN_POINT('Ctrl Pts',(-34.5828143450745,-13.1828815404475,
34.1956027867627));
#27070=CARTESIAN_POINT('Ctrl Pts',(-34.582967790943,-13.1768669995857,34.1735533641464));
#27071=CARTESIAN_POINT('Ctrl Pts',(-34.5831262740765,-13.1696750914266,
34.1520967504123));
#27072=CARTESIAN_POINT('Ctrl Pts',(-34.5832901051238,-13.1611455958502,
34.1312552352812));
#27073=CARTESIAN_POINT('Ctrl Pts',(-34.5834539361711,-13.1526161002738,
34.11041372015));
#27074=CARTESIAN_POINT('Ctrl Pts',(-34.5836231397398,-13.1427495299604,
34.0901869574092));
#27075=CARTESIAN_POINT('Ctrl Pts',(-34.5837973809619,-13.1313389816383,
34.0706303230888));
#27076=CARTESIAN_POINT('Ctrl Pts',(-34.5838561693646,-13.1274891009823,
34.0640319803939));
#27077=CARTESIAN_POINT('Ctrl Pts',(-34.5839137704652,-13.1234784566375,
34.0575374938193));
#27078=CARTESIAN_POINT('Ctrl Pts',(-34.5839705894707,-13.1192883941035,
34.0511290395554));
#27079=CARTESIAN_POINT('Ctrl Pts',(-34.5840653300571,-13.1123018412983,
34.0404435178594));
#27080=CARTESIAN_POINT('Ctrl Pts',(-34.5841564572897,-13.1049166125572,
34.0301624181513));
#27081=CARTESIAN_POINT('Ctrl Pts',(-34.5842452183515,-13.097044387883,34.0202632237194));
#27082=CARTESIAN_POINT('Ctrl Pts',(-34.5842782571648,-13.0941141732637,
34.0165785265156));
#27083=CARTESIAN_POINT('Ctrl Pts',(-34.5843109641004,-13.0911162306685,
34.0129471746141));
#27084=CARTESIAN_POINT('Ctrl Pts',(-34.5843433867853,-13.088045086031,34.009369649718));
#27085=CARTESIAN_POINT('Ctrl Pts',(-34.5844292711082,-13.0799099430592,
33.9998931580673));
#27086=CARTESIAN_POINT('Ctrl Pts',(-34.5845127940359,-13.0712950250751,
33.9908333807281));
#27087=CARTESIAN_POINT('Ctrl Pts',(-34.5845904021225,-13.0621639241565,
33.9822773142586));
#27088=CARTESIAN_POINT('Ctrl Pts',(-34.5846680102091,-13.053032823238,33.973721247789));
#27089=CARTESIAN_POINT('Ctrl Pts',(-34.5847385699196,-13.0433849467635,
33.9656697343162));
#27090=CARTESIAN_POINT('Ctrl Pts',(-34.5848124183096,-13.0331862397832,
33.9582123002755));
#27091=CARTESIAN_POINT('Ctrl Pts',(-34.5848482580143,-13.0282366579925,
33.9545930983703));
#27092=CARTESIAN_POINT('Ctrl Pts',(-34.5848828724605,-13.0231465710756,
33.9511084704396));
#27093=CARTESIAN_POINT('Ctrl Pts',(-34.5849160411879,-13.0179182754031,
33.9477774550331));
#27094=CARTESIAN_POINT('Ctrl Pts',(-34.5849905800164,-13.0061689239906,
33.9402917899096));
#27095=CARTESIAN_POINT('Ctrl Pts',(-34.5850563954841,-12.9939049176357,
33.933714890177));
#27096=CARTESIAN_POINT('Ctrl Pts',(-34.5851114686253,-12.981226713366,33.9282355973367));
#27097=CARTESIAN_POINT('Ctrl Pts',(-34.5851652658616,-12.9688422309119,
33.922883245805));
#27098=CARTESIAN_POINT('Ctrl Pts',(-34.5852088052819,-12.9560629035317,
33.9185786270626));
#27099=CARTESIAN_POINT('Ctrl Pts',(-34.5852405562661,-12.9430006092193,
33.9154520648799));
#27100=CARTESIAN_POINT('Ctrl Pts',(-34.5852714506247,-12.9302907290071,
33.912409855765));
#27101=CARTESIAN_POINT('Ctrl Pts',(-34.585291178121,-12.9173133257082,33.9104832101191));
#27102=CARTESIAN_POINT('Ctrl Pts',(-34.585298762369,-12.9041833323897,33.9097440507805));
#27103=CARTESIAN_POINT('Ctrl Pts',(-34.585301118774,-12.9001038795348,33.9095143960046));
#27104=CARTESIAN_POINT('Ctrl Pts',(-34.585302306524,-12.8960097626081,33.9093990029364));
#27105=CARTESIAN_POINT('Ctrl Pts',(-34.585302306524,-12.8919045823054,33.9093990029364));
#27106=CARTESIAN_POINT('Origin',(-20.9879227942421,-13.5169045823054,-6.86589016441886));
#27107=CARTESIAN_POINT('Origin',(-34.5818198379706,-13.5169045823054,34.3588997915592));
#27108=CARTESIAN_POINT('Origin',(-10.0425103622231,-11.3294045823054,-19.6596180593406));
#27109=CARTESIAN_POINT('Origin',(-9.75726988530523,-11.3294045823054,-19.1035039790228));
#27110=CARTESIAN_POINT('Ctrl Pts',(34.4123700316823,-10.7044045823054,34.2543780742461));
#27111=CARTESIAN_POINT('Ctrl Pts',(34.4123700316823,-11.0169045823054,34.2543780742461));
#27112=CARTESIAN_POINT('Ctrl Pts',(34.1908936222416,-11.0169045823054,34.0339139046828));
#27113=CARTESIAN_POINT('Ctrl Pts',(34.3501592468467,-10.7044046073823,34.3168744938738));
#27114=CARTESIAN_POINT('Ctrl Pts',(34.3738055566337,-11.034944931328,34.2931196129008));
#27115=CARTESIAN_POINT('Ctrl Pts',(34.1413487873541,-11.0169045823054,34.058813837913));
#27116=CARTESIAN_POINT('Ctrl Pts',(34.2893549490476,-10.718650676671,34.3776158502248));
#27117=CARTESIAN_POINT('Ctrl Pts',(34.3414414505694,-11.0630714156275,34.3255569415899));
#27118=CARTESIAN_POINT('Ctrl Pts',(34.0928733345355,-11.0240276257398,34.0829643022232));
#27119=CARTESIAN_POINT('Ctrl Pts',(34.1711981326456,-10.7765752156551,34.4950601734815));
#27120=CARTESIAN_POINT('Ctrl Pts',(34.2904881406856,-11.1314870357709,34.376795148033));
#27121=CARTESIAN_POINT('Ctrl Pts',(33.9985873189392,-11.0529899027286,34.1295721958079));
#27122=CARTESIAN_POINT('Ctrl Pts',(34.1171495610117,-10.8185639645426,34.5484801321362));
#27123=CARTESIAN_POINT('Ctrl Pts',(34.2744792581431,-11.1704305366374,34.3930297458242));
#27124=CARTESIAN_POINT('Ctrl Pts',(33.9554132623581,-11.0739842709862,34.1507269685016));
#27125=CARTESIAN_POINT('Ctrl Pts',(34.0207493920589,-10.9314866347397,34.6434052910951));
#27126=CARTESIAN_POINT('Ctrl Pts',(34.2592746271241,-11.2441510617714,34.4090931206949));
#27127=CARTESIAN_POINT('Ctrl Pts',(33.8783564349675,-11.1304456109604,34.188265264605));
#27128=CARTESIAN_POINT('Ctrl Pts',(33.981374129179,-10.9992937157271,34.68198187454));
#27129=CARTESIAN_POINT('Ctrl Pts',(34.2619434427441,-11.2750326114056,34.4070617919781));
#27130=CARTESIAN_POINT('Ctrl Pts',(33.8468530908865,-11.1643491474262,34.2034909999848));
#27131=CARTESIAN_POINT('Ctrl Pts',(33.9254685896631,-11.1560957480194,34.736665233204));
#27132=CARTESIAN_POINT('Ctrl Pts',(34.2723025800306,-11.3160025899709,34.3979203004132));
#27133=CARTESIAN_POINT('Ctrl Pts',(33.802111185478,-11.2427501667525,34.2250605800652));
#27134=CARTESIAN_POINT('Ctrl Pts',(33.9104937666812,-11.2411599901508,34.7512606791955));
#27135=CARTESIAN_POINT('Ctrl Pts',(34.2787581392411,-11.3235538600011,34.3919388546111));
#27136=CARTESIAN_POINT('Ctrl Pts',(33.7901189630482,-11.2852822850309,34.2308098236384));
#27137=CARTESIAN_POINT('Ctrl Pts',(33.9104937793594,-11.3294045823054,34.7512606668251));
#27138=CARTESIAN_POINT('Ctrl Pts',(34.2787581354396,-11.3294045823054,34.3919388580886));
#27139=CARTESIAN_POINT('Ctrl Pts',(33.7901189707501,-11.3294045823054,34.2308098261781));
#27140=CARTESIAN_POINT('Ctrl Pts',(33.7901189707501,-11.3294045823054,34.2308098261781));
#27141=CARTESIAN_POINT('Ctrl Pts',(33.7901189707501,-11.3159760597524,34.2308098261781));
#27142=CARTESIAN_POINT('Ctrl Pts',(33.7912338216707,-11.3026664608401,34.2302753470968));
#27143=CARTESIAN_POINT('Ctrl Pts',(33.7934081164331,-11.2895978753989,34.2292314243157));
#27144=CARTESIAN_POINT('Ctrl Pts',(33.79562435048,-11.2762772141433,34.228167365638));
#27145=CARTESIAN_POINT('Ctrl Pts',(33.7989410334812,-11.2632073639008,34.2265741308302));
#27146=CARTESIAN_POINT('Ctrl Pts',(33.8032512127749,-11.250506246618,34.2245015446458));
#27147=CARTESIAN_POINT('Ctrl Pts',(33.8077029487296,-11.2373879940767,34.2223608897432));
#27148=CARTESIAN_POINT('Ctrl Pts',(33.8132142064821,-11.2246635682845,34.2197090098756));
#27149=CARTESIAN_POINT('Ctrl Pts',(33.8196203282791,-11.212443933042,34.2166236619276));
#27150=CARTESIAN_POINT('Ctrl Pts',(33.8211904549206,-11.2094489267884,34.2158674497973));
#27151=CARTESIAN_POINT('Ctrl Pts',(33.8228141381246,-11.2064841392023,34.2150852966479));
#27152=CARTESIAN_POINT('Ctrl Pts',(33.8244885802811,-11.2035509891888,34.2142785315667));
#27153=CARTESIAN_POINT('Ctrl Pts',(33.8274036314582,-11.1984446423577,34.2128740270931));
#27154=CARTESIAN_POINT('Ctrl Pts',(33.8304514090713,-11.1934675809199,34.2114049990652));
#27155=CARTESIAN_POINT('Ctrl Pts',(33.8336162487135,-11.18862206557,34.209878801354));
#27156=CARTESIAN_POINT('Ctrl Pts',(33.8402728914365,-11.1784304387767,34.206668732587));
#27157=CARTESIAN_POINT('Ctrl Pts',(33.8474541808265,-11.1687879968701,34.2031919007031));
#27158=CARTESIAN_POINT('Ctrl Pts',(33.8550888482703,-11.1596600078883,34.1994978425559));
#27159=CARTESIAN_POINT('Ctrl Pts',(33.8635475329149,-11.1495468260368,34.1954050810629));
#27160=CARTESIAN_POINT('Ctrl Pts',(33.8725221968181,-11.1400969285544,34.1910570289537));
#27161=CARTESIAN_POINT('Ctrl Pts',(33.8819480720297,-11.1312146907196,34.1864836245605));
#27162=CARTESIAN_POINT('Ctrl Pts',(33.8918181729339,-11.1219138479102,34.1816946832872));
#27163=CARTESIAN_POINT('Ctrl Pts',(33.9021833303367,-11.1132352948843,34.1766585236442));
#27164=CARTESIAN_POINT('Ctrl Pts',(33.913015050167,-11.1050933657985,34.1713874544776));
#27165=CARTESIAN_POINT('Ctrl Pts',(33.9143006425789,-11.1041270185873,34.1707618431592));
#27166=CARTESIAN_POINT('Ctrl Pts',(33.9155928549205,-11.1031682588508,34.1701328995634));
#27167=CARTESIAN_POINT('Ctrl Pts',(33.916891676798,-11.1022169660873,34.1695006260756));
#27168=CARTESIAN_POINT('Ctrl Pts',(33.9224967875947,-11.0981116292185,34.1667720279404));
#27169=CARTESIAN_POINT('Ctrl Pts',(33.9281745502422,-11.0941782436166,34.1640059611718));
#27170=CARTESIAN_POINT('Ctrl Pts',(33.9339309727463,-11.0904041712721,34.1611993802633));
#27171=CARTESIAN_POINT('Ctrl Pts',(33.9514412782026,-11.0789239229899,34.152662117934));
#27172=CARTESIAN_POINT('Ctrl Pts',(33.969549527539,-11.0689908784592,34.1438027788335));
#27173=CARTESIAN_POINT('Ctrl Pts',(33.9881992711126,-11.0604019317832,34.1346450450658));
#27174=CARTESIAN_POINT('Ctrl Pts',(34.0068490146862,-11.0518129851073,34.1254873112982));
#27175=CARTESIAN_POINT('Ctrl Pts',(34.0260406250709,-11.0445686309469,34.1160310511287));
#27176=CARTESIAN_POINT('Ctrl Pts',(34.045749017185,-11.0385127393807,34.1062850795439));
#27177=CARTESIAN_POINT('Ctrl Pts',(34.0667664671036,-11.0320546073846,34.0958917674714));
#27178=CARTESIAN_POINT('Ctrl Pts',(34.0878492419839,-11.0271158190915,34.0854271901211));
#27179=CARTESIAN_POINT('Ctrl Pts',(34.1090552865085,-11.0235921824189,34.0748636859948));
#27180=CARTESIAN_POINT('Ctrl Pts',(34.1306266089857,-11.0200078504674,34.0641182235992));
#27181=CARTESIAN_POINT('Ctrl Pts',(34.1523255949182,-11.0178879088435,34.0532703834115));
#27182=CARTESIAN_POINT('Ctrl Pts',(34.1742231261325,-11.0171750715253,34.0422846764148));
#27183=CARTESIAN_POINT('Ctrl Pts',(34.1797667772391,-11.0169946072826,34.0395034986577));
#27184=CARTESIAN_POINT('Ctrl Pts',(34.1853231974622,-11.0169045823054,34.0367134539662));
#27185=CARTESIAN_POINT('Ctrl Pts',(34.1908936222416,-11.0169045823054,34.0339139046828));
#27186=CARTESIAN_POINT('Origin',(41.4437380877936,-13.5169045823054,37.0836464997312));
#27187=CARTESIAN_POINT('Origin',(41.4437380877936,-13.5169045823054,37.0836464997312));
#27188=CARTESIAN_POINT('Origin',(41.4437380877936,-13.5169045823054,37.0836464997312));
#27189=CARTESIAN_POINT('Origin',(0.0835265683620477,-13.5169045823054,0.0824317919394229));
#27190=CARTESIAN_POINT('Origin',(40.2796596827637,-13.5169045823054,38.3450489192809));
#27191=CARTESIAN_POINT('Origin',(-7.35411383562686,-12.8919045823054,22.6377860392341));
#27192=CARTESIAN_POINT('Origin',(33.0778695430594,-12.8919045823054,35.9702546803237));
#27193=CARTESIAN_POINT('Ctrl Pts',(39.2345740945198,-12.8919045823054,38.3294829568536));
#27194=CARTESIAN_POINT('Ctrl Pts',(39.264809323272,-12.9061660297064,38.3394530400775));
#27195=CARTESIAN_POINT('Ctrl Pts',(39.2954516743711,-12.920086395132,38.3485334458199));
#27196=CARTESIAN_POINT('Ctrl Pts',(39.3264280099796,-12.9336529684133,38.3568222284112));
#27197=CARTESIAN_POINT('Ctrl Pts',(39.3601265408272,-12.9484117699059,38.3658394278429));
#27198=CARTESIAN_POINT('Ctrl Pts',(39.3942201310872,-12.9627531581661,38.3739203780609));
#27199=CARTESIAN_POINT('Ctrl Pts',(39.4286337339504,-12.9766849821654,38.3811333480185));
#27200=CARTESIAN_POINT('Ctrl Pts',(39.4624584084797,-12.9903783874809,38.3882228806715));
#27201=CARTESIAN_POINT('Ctrl Pts',(39.4965924126089,-13.0036776000038,38.3944733524844));
#27202=CARTESIAN_POINT('Ctrl Pts',(39.5309818914864,-13.0165906742131,38.399896805926));
#27203=CARTESIAN_POINT('Ctrl Pts',(39.5662695137509,-13.0298409966909,38.4054619026551));
#27204=CARTESIAN_POINT('Ctrl Pts',(39.6018262535649,-13.0426862586666,38.4101558421804));
#27205=CARTESIAN_POINT('Ctrl Pts',(39.6376103185495,-13.0551132414191,38.4139419214656));
#27206=CARTESIAN_POINT('Ctrl Pts',(39.6715407016172,-13.0668964830757,38.4175318747179));
#27207=CARTESIAN_POINT('Ctrl Pts',(39.7056757961189,-13.0783045133849,38.4203045946093));
#27208=CARTESIAN_POINT('Ctrl Pts',(39.7399908862156,-13.0892900686274,38.4221956986995));
#27209=CARTESIAN_POINT('Ctrl Pts',(39.7418655854155,-13.0898902305843,38.4222990133437));
#27210=CARTESIAN_POINT('Ctrl Pts',(39.7437408239533,-13.0904891204199,38.4223996902635));
#27211=CARTESIAN_POINT('Ctrl Pts',(39.745616598492,-13.0910867263844,38.4224977168591));
#27212=CARTESIAN_POINT('Ctrl Pts',(39.7728375717412,-13.0997590991245,38.4239202648684));
#27213=CARTESIAN_POINT('Ctrl Pts',(39.8001748601324,-13.1081389493477,38.4248104957089));
#27214=CARTESIAN_POINT('Ctrl Pts',(39.8276166222947,-13.1162261892174,38.4250795370517));
#27215=CARTESIAN_POINT('Ctrl Pts',(39.8542746788235,-13.1240824666798,38.4253408948786));
#27216=CARTESIAN_POINT('Ctrl Pts',(39.8810315488655,-13.1316631802151,38.4250153647531));
#27217=CARTESIAN_POINT('Ctrl Pts',(39.9078825960307,-13.1389242143529,38.4240026130721));
#27218=CARTESIAN_POINT('Ctrl Pts',(39.9334074955964,-13.1458266329428,38.4230398802303));
#27219=CARTESIAN_POINT('Ctrl Pts',(39.9590177371494,-13.1524404698811,38.421455410863));
#27220=CARTESIAN_POINT('Ctrl Pts',(39.9847117520737,-13.1586815279054,38.4191556941318));
#27221=CARTESIAN_POINT('Ctrl Pts',(39.9944282810576,-13.1610416659127,38.4182860260656));
#27222=CARTESIAN_POINT('Ctrl Pts',(40.0041567975574,-13.1633479802309,38.4173140502073));
#27223=CARTESIAN_POINT('Ctrl Pts',(40.0138971970891,-13.1655939279677,38.4162347690805));
#27224=CARTESIAN_POINT('Ctrl Pts',(40.0336369972984,-13.1701455440958,38.414047508307));
#27225=CARTESIAN_POINT('Ctrl Pts',(40.0533462534983,-13.174435676212,38.4114272898243));
#27226=CARTESIAN_POINT('Ctrl Pts',(40.0730154951905,-13.1784305895997,38.4082506512823));
#27227=CARTESIAN_POINT('Ctrl Pts',(40.0916995992408,-13.1822254170047,38.4052331152746));
#27228=CARTESIAN_POINT('Ctrl Pts',(40.1103478051953,-13.1857540666263,38.4017128678585));
#27229=CARTESIAN_POINT('Ctrl Pts',(40.1289527638623,-13.1889407631081,38.397581753751));
#27230=CARTESIAN_POINT('Ctrl Pts',(40.1356516054506,-13.1900881547956,38.3960943180902));
#27231=CARTESIAN_POINT('Ctrl Pts',(40.1423448327474,-13.1911907417383,38.3945277124038));
#27232=CARTESIAN_POINT('Ctrl Pts',(40.1490320418338,-13.1922433006301,38.3928770728127));
#27233=CARTESIAN_POINT('Ctrl Pts',(40.1634532674053,-13.1945131846744,38.3893174045603));
#27234=CARTESIAN_POINT('Ctrl Pts',(40.1778289941368,-13.1965398886054,38.3854132586859));
#27235=CARTESIAN_POINT('Ctrl Pts',(40.1920769307064,-13.1982777342415,38.3810070154518));
#27236=CARTESIAN_POINT('Ctrl Pts',(40.2057841542068,-13.1999496281629,38.3767679903472));
#27237=CARTESIAN_POINT('Ctrl Pts',(40.2193732995346,-13.201354438406,38.3720636577237));
#27238=CARTESIAN_POINT('Ctrl Pts',(40.232769573981,-13.2024042504876,38.3667582778887));
#27239=CARTESIAN_POINT('Ctrl Pts',(40.2453986452936,-13.2033939399492,38.3617567365613));
#27240=CARTESIAN_POINT('Ctrl Pts',(40.2578565021756,-13.2040681761667,38.3562204211069));
#27241=CARTESIAN_POINT('Ctrl Pts',(40.270076341403,-13.204308494197,38.3500481542611));
#27242=CARTESIAN_POINT('Ctrl Pts',(40.2732876902366,-13.2043716492854,38.3484260951188));
#27243=CARTESIAN_POINT('Ctrl Pts',(40.276482568374,-13.2044045823054,38.3467602140877));
#27244=CARTESIAN_POINT('Ctrl Pts',(40.2796596827637,-13.2044045823054,38.3450489192809));
#27245=CARTESIAN_POINT('Origin',(0.0835265683620477,-12.8919045823054,0.0824317919394229));
#27246=CARTESIAN_POINT('Origin',(33.0778695430594,-12.8919045823054,35.9702546803237));
#27247=CARTESIAN_POINT('Ctrl Pts',(-34.2850388610326,-13.5169045823054,
34.4567634810853));
#27248=CARTESIAN_POINT('Ctrl Pts',(-34.2850388610326,-13.2044045823054,
34.4567634810853));
#27249=CARTESIAN_POINT('Ctrl Pts',(-34.5818198379706,-13.2044045823054,
34.3588997915592));
#27250=CARTESIAN_POINT('Ctrl Pts',(-34.2575612226533,-13.5169045582439,
34.3734349207008));
#27251=CARTESIAN_POINT('Ctrl Pts',(-34.2679818400087,-13.1861191316367,
34.4050364372002));
#27252=CARTESIAN_POINT('Ctrl Pts',(-34.5821199172207,-13.2044045823054,
34.3030373915905));
#27253=CARTESIAN_POINT('Ctrl Pts',(-34.2307991361275,-13.5027466839949,
34.2922763395917));
#27254=CARTESIAN_POINT('Ctrl Pts',(-34.2537496078692,-13.1578432798927,
34.3618758351519));
#27255=CARTESIAN_POINT('Ctrl Pts',(-34.582462300581,-13.1973256316196,34.2485439649434));
#27256=CARTESIAN_POINT('Ctrl Pts',(-34.178864375399,-13.4449866817212,34.1347792219102));
#27257=CARTESIAN_POINT('Ctrl Pts',(-34.2313639583219,-13.0892356355756,
34.2939892167934));
#27258=CARTESIAN_POINT('Ctrl Pts',(-34.5832141772212,-13.1684456335483,
34.1426428491029));
#27259=CARTESIAN_POINT('Ctrl Pts',(-34.1551840390824,-13.4031153721666,
34.0629663423807));
#27260=CARTESIAN_POINT('Ctrl Pts',(-34.2243687577112,-13.0503322093644,
34.2727756034371));
#27261=CARTESIAN_POINT('Ctrl Pts',(-34.5836019567474,-13.1475099673759,
34.0942783344611));
#27262=CARTESIAN_POINT('Ctrl Pts',(-34.1129735724795,-13.2902331116009,
33.9349590745566));
#27263=CARTESIAN_POINT('Ctrl Pts',(-34.2176859346367,-12.9767617731723,
34.2525093047707));
#27264=CARTESIAN_POINT('Ctrl Pts',(-34.5843462881308,-13.0910688568132,
34.0079756192384));
#27265=CARTESIAN_POINT('Ctrl Pts',(-34.0957840228135,-13.2224528271012,
33.8828301249157));
#27266=CARTESIAN_POINT('Ctrl Pts',(-34.2188142136836,-12.9460615526393,
34.255930918643));
#27267=CARTESIAN_POINT('Ctrl Pts',(-34.5846789122388,-13.0571787063095,
33.9727789086256));
#27268=CARTESIAN_POINT('Ctrl Pts',(-34.0713699253873,-13.0654169357609,
33.8087920448033));
#27269=CARTESIAN_POINT('Ctrl Pts',(-34.2232253292175,-12.9052920386068,
34.2693080474217));
#27270=CARTESIAN_POINT('Ctrl Pts',(-34.5851647206562,-12.9786607574269,
33.9227660142796));
#27271=CARTESIAN_POINT('Ctrl Pts',(-34.0648514601626,-12.9802875861309,
33.7890241769979));
#27272=CARTESIAN_POINT('Ctrl Pts',(-34.2259804994776,-12.8977806170664,
34.2776633641381));
#27273=CARTESIAN_POINT('Ctrl Pts',(-34.5853023124368,-12.936096085427,33.9093989968765));
#27274=CARTESIAN_POINT('Ctrl Pts',(-34.064851465877,-12.8919045823054,33.7890241943272));
#27275=CARTESIAN_POINT('Ctrl Pts',(-34.2259804977875,-12.8919045823054,
34.2776633590166));
#27276=CARTESIAN_POINT('Ctrl Pts',(-34.585302306524,-12.8919045823054,33.9093990029364));
#27277=CARTESIAN_POINT('Origin',(-34.361632442815,-12.8919045823054,33.691160504801));
#27278=CARTESIAN_POINT('Origin',(0.0835265683620477,-11.3294045823054,0.0824317919394229));
#27279=CARTESIAN_POINT('Origin',(-20.394360840366,-11.3294045823054,-6.6701627853663));
#27280=CARTESIAN_POINT('Origin',(-6.66906800894368,-11.3294045823054,20.5603192006674));
#27281=CARTESIAN_POINT('Origin',(-6.66906800894368,-11.3294045823054,20.5603192006674));
#27282=CARTESIAN_POINT('Ctrl Pts',(42.9952736832849,-14.9232028613467,37.2662146291476));
#27283=CARTESIAN_POINT('Ctrl Pts',(43.262083132434,-14.6181128259928,37.3541951909867));
#27284=CARTESIAN_POINT('Ctrl Pts',(43.0636720738749,-14.7022319922259,37.7085464415881));
#27285=CARTESIAN_POINT('Ctrl Pts',(42.5112271215405,-14.4538621299839,37.106600010571));
#27286=CARTESIAN_POINT('Ctrl Pts',(42.7777192980699,-14.147074607234,37.1944759515764));
#27287=CARTESIAN_POINT('Ctrl Pts',(42.5791171508971,-14.2328912595879,37.5495125198651));
#27288=CARTESIAN_POINT('Ctrl Pts',(42.0266693850915,-13.9850662226618,36.9468168318559));
#27289=CARTESIAN_POINT('Ctrl Pts',(42.2935697537446,-13.6772499732431,37.0348273744504));
#27290=CARTESIAN_POINT('Ctrl Pts',(42.0940349090533,-13.7640953522125,37.3903223553195));
#27291=CARTESIAN_POINT('Ctrl Pts',(41.5416017773197,-13.5169045823054,36.7868655227931));
#27292=CARTESIAN_POINT('Ctrl Pts',(41.8097676469788,-13.2088427643879,36.8752933650375));
#27293=CARTESIAN_POINT('Ctrl Pts',(41.6084251757828,-13.2959337131846,37.2309770398429));
#27294=CARTESIAN_POINT('Ctrl Pts',(43.0359437585039,-14.6753754510085,37.6994458554132));
#27295=CARTESIAN_POINT('Ctrl Pts',(43.0437650201411,-14.6771438430878,37.6931993723333));
#27296=CARTESIAN_POINT('Ctrl Pts',(43.0511197893374,-14.6786525232815,37.6863023375307));
#27297=CARTESIAN_POINT('Ctrl Pts',(43.0578129301505,-14.6799030932779,37.678804973348));
#27298=CARTESIAN_POINT('Ctrl Pts',(43.0643231830576,-14.681119491854,37.6715124722146));
#27299=CARTESIAN_POINT('Ctrl Pts',(43.0702066967261,-14.6820924420366,37.6636521449987));
#27300=CARTESIAN_POINT('Ctrl Pts',(43.075289676931,-14.6828029998434,37.6553127292641));
#27301=CARTESIAN_POINT('Ctrl Pts',(43.0802767004004,-14.6835001437071,37.6471307454057));
#27302=CARTESIAN_POINT('Ctrl Pts',(43.0844923876095,-14.6839452832804,37.6384881509309));
#27303=CARTESIAN_POINT('Ctrl Pts',(43.0877895089784,-14.6840907481788,37.6295050829525));
#27304=CARTESIAN_POINT('Ctrl Pts',(43.0910495157316,-14.6842345756264,37.6206231344291));
#27305=CARTESIAN_POINT('Ctrl Pts',(43.0934109488286,-14.6840857258448,37.6114092174673));
#27306=CARTESIAN_POINT('Ctrl Pts',(43.0947580631468,-14.6835622048232,37.6020045512144));
#27307=CARTESIAN_POINT('Ctrl Pts',(43.0949428628685,-14.683490387207,37.6007144010897));
#27308=CARTESIAN_POINT('Ctrl Pts',(43.0951086225669,-14.6834114599927,37.5994206874669));
#27309=CARTESIAN_POINT('Ctrl Pts',(43.095255090887,-14.6833251552391,37.5981237965455));
#27310=CARTESIAN_POINT('Ctrl Pts',(43.0966138582008,-14.6825245174079,37.5860927102892));
#27311=CARTESIAN_POINT('Ctrl Pts',(43.0964603511804,-14.6812727698323,37.5740720224458));
#27312=CARTESIAN_POINT('Ctrl Pts',(43.0950823298483,-14.679660389819,37.5622300656422));
#27313=CARTESIAN_POINT('Ctrl Pts',(43.093667437698,-14.6780048684051,37.5500712613228));
#27314=CARTESIAN_POINT('Ctrl Pts',(43.090962564536,-14.6759682812647,37.5381006221555));
#27315=CARTESIAN_POINT('Ctrl Pts',(43.0872892963239,-14.6736566051529,37.526446083814));
#27316=CARTESIAN_POINT('Ctrl Pts',(43.0834525783029,-14.6712420661416,37.5142729522322));
#27317=CARTESIAN_POINT('Ctrl Pts',(43.0785602210309,-14.6685267231679,37.5024441163509));
#27318=CARTESIAN_POINT('Ctrl Pts',(43.0729753261427,-14.6656525103353,37.4910532094055));
#27319=CARTESIAN_POINT('Ctrl Pts',(43.0717676935356,-14.6650310137439,37.4885901315988));
#27320=CARTESIAN_POINT('Ctrl Pts',(43.0705276424938,-14.6644021844316,37.486147363895));
#27321=CARTESIAN_POINT('Ctrl Pts',(43.0692587709865,-14.6637676196428,37.4837255967772));
#27322=CARTESIAN_POINT('Ctrl Pts',(43.0626898910944,-14.6604825116884,37.4711882380042));
#27323=CARTESIAN_POINT('Ctrl Pts',(43.0553951151393,-14.6571124630582,37.4591373845352));
#27324=CARTESIAN_POINT('Ctrl Pts',(43.0475293371387,-14.6536176840779,37.4475549388437));
#27325=CARTESIAN_POINT('Ctrl Pts',(43.0393170978584,-14.6499689717425,37.4354623250598));
#27326=CARTESIAN_POINT('Ctrl Pts',(43.0304828845192,-14.6461842219896,37.4238791913252));
#27327=CARTESIAN_POINT('Ctrl Pts',(43.0211759207055,-14.6422568272867,37.4127532083216));
#27328=CARTESIAN_POINT('Ctrl Pts',(43.0112246040603,-14.6380575256604,37.400856935587));
#27329=CARTESIAN_POINT('Ctrl Pts',(43.000733118812,-14.633695204416,37.3894821905549));
#27330=CARTESIAN_POINT('Ctrl Pts',(42.9898473507829,-14.6292054571919,37.3785473267842));
#27331=CARTESIAN_POINT('Ctrl Pts',(42.9781990027406,-14.624401189992,37.3668464436992));
#27332=CARTESIAN_POINT('Ctrl Pts',(42.9660992717873,-14.6194513461048,37.355648033558));
#27333=CARTESIAN_POINT('Ctrl Pts',(42.9536832408992,-14.6144447802759,37.3448514158025));
#27334=CARTESIAN_POINT('Ctrl Pts',(42.941267210011,-14.6094382144471,37.334054798047));
#27335=CARTESIAN_POINT('Ctrl Pts',(42.9285343617696,-14.6043757482479,37.3236591241839));
#27336=CARTESIAN_POINT('Ctrl Pts',(42.9155818628024,-14.5993802185557,37.3135788004322));
#27337=CARTESIAN_POINT('Ctrl Pts',(42.8962894060687,-14.591939489111,37.2985643842694));
#27338=CARTESIAN_POINT('Ctrl Pts',(42.8764459695827,-14.5844764296233,37.2843215640082));
#27339=CARTESIAN_POINT('Ctrl Pts',(42.856170967152,-14.5769485180958,37.2707744162756));
#27340=CARTESIAN_POINT('Ctrl Pts',(42.834697130939,-14.5689754912259,37.2564262438126));
#27341=CARTESIAN_POINT('Ctrl Pts',(42.8127390058597,-14.5609303686276,37.2428570639408));
#27342=CARTESIAN_POINT('Ctrl Pts',(42.7903962775658,-14.5528049305382,37.229980197936));
#27343=CARTESIAN_POINT('Ctrl Pts',(42.7658972710589,-14.5438953131449,37.2158605962522));
#27344=CARTESIAN_POINT('Ctrl Pts',(42.7409353913648,-14.5348900830952,37.2025719529671));
#27345=CARTESIAN_POINT('Ctrl Pts',(42.7155973478082,-14.5258150805526,37.1900277465265));
#27346=CARTESIAN_POINT('Ctrl Pts',(42.6891346188931,-14.5163372638596,37.1769267376128));
#27347=CARTESIAN_POINT('Ctrl Pts',(42.6622603264008,-14.5067848826421,37.1646370305515));
#27348=CARTESIAN_POINT('Ctrl Pts',(42.6350409751707,-14.4972049637156,37.153106204072));
#27349=CARTESIAN_POINT('Ctrl Pts',(42.6066694342357,-14.487219528733,37.1410872800091));
#27350=CARTESIAN_POINT('Ctrl Pts',(42.5779214158317,-14.4772057790315,37.1298929502604));
#27351=CARTESIAN_POINT('Ctrl Pts',(42.5488605293239,-14.4672106594487,37.1195178237689));
#27352=CARTESIAN_POINT('Ctrl Pts',(42.5364377106081,-14.462937990114,37.1150827107684));
#27353=CARTESIAN_POINT('Ctrl Pts',(42.5239577230844,-14.4586685042083,37.1107979333954));
#27354=CARTESIAN_POINT('Ctrl Pts',(42.5114260048381,-14.4544045238124,37.1066655924472));
#27355=CARTESIAN_POINT('Ctrl Pts',(39.1987322410677,-12.5761796977903,38.7430878994609));
#27356=CARTESIAN_POINT('Ctrl Pts',(39.4780446252898,-12.4966730216635,38.3474248665547));
#27357=CARTESIAN_POINT('Ctrl Pts',(39.1382020843858,-12.8445798972105,38.2941504721537));
#27358=CARTESIAN_POINT('Ctrl Pts',(39.3808518331676,-12.7679658886685,38.831628414024));
#27359=CARTESIAN_POINT('Ctrl Pts',(39.5085178360912,-12.6138199372454,38.4824096995347));
#27360=CARTESIAN_POINT('Ctrl Pts',(39.3246634921425,-12.9405865508064,38.3699715896931));
#27361=CARTESIAN_POINT('Ctrl Pts',(39.6159775649996,-12.9477999797133,38.8494978613861));
#27362=CARTESIAN_POINT('Ctrl Pts',(39.6750415100163,-12.8036087634362,38.5830901947362));
#27363=CARTESIAN_POINT('Ctrl Pts',(39.5504499068629,-13.0304169137554,38.4148517236754));
#27364=CARTESIAN_POINT('Ctrl Pts',(39.9548358734585,-13.1418528526574,38.7796080468698));
#27365=CARTESIAN_POINT('Ctrl Pts',(39.960999963987,-13.0167291165573,38.5935423303748));
#27366=CARTESIAN_POINT('Ctrl Pts',(39.8616681613932,-13.1274080636025,38.4271929768978));
#27367=CARTESIAN_POINT('Ctrl Pts',(40.0571173600845,-13.1924895597094,38.7468639463194));
#27368=CARTESIAN_POINT('Ctrl Pts',(40.0465003630512,-13.072136008791,38.5846653313979));
#27369=CARTESIAN_POINT('Ctrl Pts',(39.9538574541801,-13.1527155106484,38.4245349001724));
#27370=CARTESIAN_POINT('Ctrl Pts',(40.2987174380344,-13.2848578326186,38.6292554066571));
#27371=CARTESIAN_POINT('Ctrl Pts',(40.2485456959896,-13.176690865436,38.5251285662321));
#27372=CARTESIAN_POINT('Ctrl Pts',(40.1655692505595,-13.1988763557094,38.3961928595937));
#27373=CARTESIAN_POINT('Ctrl Pts',(40.4365733990678,-13.3151873395665,38.5290256968038));
#27374=CARTESIAN_POINT('Ctrl Pts',(40.3702936127468,-13.2202535090894,38.460793898628));
#27375=CARTESIAN_POINT('Ctrl Pts',(40.2811022909383,-13.2140287022007,38.3620259985628));
#27376=CARTESIAN_POINT('Ctrl Pts',(40.5291981978548,-13.2823030560792,38.3833348140131));
#27377=CARTESIAN_POINT('Ctrl Pts',(40.4486655654144,-13.2034487358322,38.3536972626374));
#27378=CARTESIAN_POINT('Ctrl Pts',(40.3477835278082,-13.1975864244367,38.2956850594486));
#27379=CARTESIAN_POINT('Origin',(39.1367104049936,-12.8919045823054,38.6262639337916));
#27380=CARTESIAN_POINT('Origin',(33.0778695430594,-12.8919045823054,35.9702546803237));
#27381=CARTESIAN_POINT('Origin',(33.0778695430594,-12.8919045823054,35.9702546803237));
#27382=CARTESIAN_POINT('Origin',(-34.361632442815,-14.7669045823054,33.691160504801));
#27383=CARTESIAN_POINT('Origin',(-34.361632442815,-11.3294045823054,33.691160504801));
#27384=CARTESIAN_POINT('Origin',(-20.3943608403659,-11.3294045823054,-6.67016278536651));
#27385=CARTESIAN_POINT('Ctrl Pts',(-33.8679555443817,-11.0169045823054,
34.1897988458186));
#27386=CARTESIAN_POINT('Ctrl Pts',(-33.8790249460546,-11.0169045823054,
34.1677734184622));
#27387=CARTESIAN_POINT('Ctrl Pts',(-33.8899462267957,-11.0183080822731,
34.1459662914066));
#27388=CARTESIAN_POINT('Ctrl Pts',(-33.9007564985824,-11.0211596046334,
34.1243041234319));
#27389=CARTESIAN_POINT('Ctrl Pts',(-33.9113853399145,-11.0239632694552,
34.1030055149551));
#27390=CARTESIAN_POINT('Ctrl Pts',(-33.9219068783712,-11.0281667153314,
34.0818469358361));
#27391=CARTESIAN_POINT('Ctrl Pts',(-33.9323504244984,-11.0338614984773,
34.0607676029711));
#27392=CARTESIAN_POINT('Ctrl Pts',(-33.9350140049392,-11.0353139278358,
34.0553914119685));
#27393=CARTESIAN_POINT('Ctrl Pts',(-33.9376724809033,-11.0368636220489,
34.0500204262757));
#27394=CARTESIAN_POINT('Ctrl Pts',(-33.9403262734905,-11.038512634127,34.0446537457636));
#27395=CARTESIAN_POINT('Ctrl Pts',(-33.9500720656005,-11.0445684687007,
34.0249451397312));
#27396=CARTESIAN_POINT('Ctrl Pts',(-33.9595280764102,-11.0518127318511,
34.0057532193741));
#27397=CARTESIAN_POINT('Ctrl Pts',(-33.9686854830345,-11.0604015318982,
33.9871030085655));
#27398=CARTESIAN_POINT('Ctrl Pts',(-33.9778428896589,-11.0689903319452,
33.968452797757));
#27399=CARTESIAN_POINT('Ctrl Pts',(-33.9867018233878,-11.0789231726624,
33.9503439241685));
#27400=CARTESIAN_POINT('Ctrl Pts',(-33.9952386171108,-11.0904031558603,
33.9328327583415));
#27401=CARTESIAN_POINT('Ctrl Pts',(-33.9980489407163,-11.0941823812718,
33.9270680597579));
#27402=CARTESIAN_POINT('Ctrl Pts',(-34.0008137051527,-11.0981143207712,
33.9213931588931));
#27403=CARTESIAN_POINT('Ctrl Pts',(-34.0035399736574,-11.1022159367836,
33.9157934297787));
#27404=CARTESIAN_POINT('Ctrl Pts',(-34.0082085418066,-11.1092397034607,
33.9062042359987));
#27405=CARTESIAN_POINT('Ctrl Pts',(-34.0126937919884,-11.1166630537835,
33.8969802308828));
#27406=CARTESIAN_POINT('Ctrl Pts',(-34.0170055140338,-11.1245727500526,
33.8881013312154));
#27407=CARTESIAN_POINT('Ctrl Pts',(-34.0186386281196,-11.1275686380657,
33.8847383463196));
#27408=CARTESIAN_POINT('Ctrl Pts',(-34.0202466520755,-11.1306345602647,
33.8814252694475));
#27409=CARTESIAN_POINT('Ctrl Pts',(-34.0218293558254,-11.1337762021651,
33.8781625736533));
#27410=CARTESIAN_POINT('Ctrl Pts',(-34.0259301037929,-11.141916121994,33.8697090060497));
#27411=CARTESIAN_POINT('Ctrl Pts',(-34.029844606577,-11.1505315993467,33.8616271594708));
#27412=CARTESIAN_POINT('Ctrl Pts',(-34.033539078864,-11.1596598005335,33.8539932768864));
#27413=CARTESIAN_POINT('Ctrl Pts',(-34.0372335511508,-11.1687880017203,
33.8463593943019));
#27414=CARTESIAN_POINT('Ctrl Pts',(-34.0407103722858,-11.1784304387767,
33.8391781150135));
#27415=CARTESIAN_POINT('Ctrl Pts',(-34.0439204410529,-11.18862206557,33.8325214722905));
#27416=CARTESIAN_POINT('Ctrl Pts',(-34.0454466387641,-11.1934675809199,
33.8293566326483));
#27417=CARTESIAN_POINT('Ctrl Pts',(-34.046915666792,-11.1984446423577,33.8263088550353));
#27418=CARTESIAN_POINT('Ctrl Pts',(-34.0483201712657,-11.2035509891889,
33.8233938038582));
#27419=CARTESIAN_POINT('Ctrl Pts',(-34.051594172964,-11.2154542536579,33.8165986083399));
#27420=CARTESIAN_POINT('Ctrl Pts',(-34.0544613220038,-11.2278803704204,
33.8106424362858));
#27421=CARTESIAN_POINT('Ctrl Pts',(-34.056840045953,-11.2407256805043,33.805697585903));
#27422=CARTESIAN_POINT('Ctrl Pts',(-34.0591638383017,-11.2532743553093,
33.8008669263854));
#27423=CARTESIAN_POINT('Ctrl Pts',(-34.0610213391567,-11.2662226779411,
33.7970017910542));
#27424=CARTESIAN_POINT('Ctrl Pts',(-34.062356555885,-11.2794553416021,33.7942218688642));
#27425=CARTESIAN_POINT('Ctrl Pts',(-34.0636553759747,-11.2923272964232,
33.791517724502));
#27426=CARTESIAN_POINT('Ctrl Pts',(-34.06445991162,-11.3054678991079,33.7898406443579));
#27427=CARTESIAN_POINT('Ctrl Pts',(-34.0647396118803,-11.3187590936875,
33.7892574482984));
#27428=CARTESIAN_POINT('Ctrl Pts',(-34.0648140791939,-11.3222977373503,
33.7891021783543));
#27429=CARTESIAN_POINT('Ctrl Pts',(-34.064851465877,-11.3258470068799,33.7890241943272));
#27430=CARTESIAN_POINT('Ctrl Pts',(-34.064851465877,-11.3294045823054,33.7890241943272));
#27431=CARTESIAN_POINT('Origin',(0.0835265683620477,-11.3294045823054,0.0824317919394229));
#27432=CARTESIAN_POINT('Ctrl Pts',(42.9634361744535,-14.6563598281187,37.7375957880963));
#27433=CARTESIAN_POINT('Ctrl Pts',(43.0152755598457,-14.7669045823054,37.8141269532137));
#27434=CARTESIAN_POINT('Ctrl Pts',(43.0959610209804,-14.7669045823054,37.9343011683297));
#27435=CARTESIAN_POINT('Ctrl Pts',(43.0251556892479,-14.6732979129397,37.7164407335828));
#27436=CARTESIAN_POINT('Ctrl Pts',(43.0892175038907,-14.7669045823054,37.7863585316547));
#27437=CARTESIAN_POINT('Ctrl Pts',(43.1842232087159,-14.7669045823054,37.881209115481));
#27438=CARTESIAN_POINT('Ctrl Pts',(43.0716902715764,-14.6836226395009,37.6764598776803));
#27439=CARTESIAN_POINT('Ctrl Pts',(43.1499072765567,-14.7669045823054,37.7261013273251));
#27440=CARTESIAN_POINT('Ctrl Pts',(43.2565479977638,-14.7669045823054,37.7937637317459));
#27441=CARTESIAN_POINT('Ctrl Pts',(43.0976316625303,-14.6837071744111,37.5986181406452));
#27442=CARTESIAN_POINT('Ctrl Pts',(43.1868411123276,-14.7669045823054,37.6150902279279));
#27443=CARTESIAN_POINT('Ctrl Pts',(43.3084198250278,-14.7669045823054,37.6375340941341));
#27444=CARTESIAN_POINT('Ctrl Pts',(43.0976468821399,-14.6805726740665,37.5678665274605));
#27445=CARTESIAN_POINT('Ctrl Pts',(43.1888566429373,-14.7669045823055,37.5717104765813));
#27446=CARTESIAN_POINT('Ctrl Pts',(43.3148976072562,-14.7669045823054,37.5779620629119));
#27447=CARTESIAN_POINT('Ctrl Pts',(43.0733162886299,-14.6635276241059,37.474635535667));
#27448=CARTESIAN_POINT('Ctrl Pts',(43.1646316507186,-14.7669045823052,37.4441076009668));
#27449=CARTESIAN_POINT('Ctrl Pts',(43.3011453607231,-14.7669045823054,37.4025193023754));
#27450=CARTESIAN_POINT('Ctrl Pts',(43.0259131176636,-14.642479666692,37.4121085028892));
#27451=CARTESIAN_POINT('Ctrl Pts',(43.1081309591734,-14.7669045823054,37.3637507252828));
#27452=CARTESIAN_POINT('Ctrl Pts',(43.2493294050651,-14.7669045823054,37.2914481919115));
#27453=CARTESIAN_POINT('Ctrl Pts',(42.8231824197416,-14.5607785229662,37.2253968287826));
#27454=CARTESIAN_POINT('Ctrl Pts',(42.860006513641,-14.7669045823054,37.14139474828));
#27455=CARTESIAN_POINT('Ctrl Pts',(43.0108374746241,-14.7669045823054,36.9729006240994));
#27456=CARTESIAN_POINT('Ctrl Pts',(42.612287234451,-14.4859905466056,37.1300246791343));
#27457=CARTESIAN_POINT('Ctrl Pts',(42.5879336945949,-14.7669045823054,37.085517422922));
#27458=CARTESIAN_POINT('Ctrl Pts',(42.7420195871275,-14.7669045823054,36.8334121977696));
#27459=CARTESIAN_POINT('Ctrl Pts',(42.4099536223294,-14.4183787521173,37.0764201725757));
#27460=CARTESIAN_POINT('Ctrl Pts',(42.4017503726634,-14.7669045823054,37.1167798525067));
#27461=CARTESIAN_POINT('Ctrl Pts',(42.4769068720474,-14.7669045823054,36.7731031625989));
#27462=CARTESIAN_POINT('Origin',(42.6092896432871,-14.4544045823054,36.8098845986664));
#27463=CARTESIAN_POINT('Origin',(43.2021767306697,-14.4544045823054,37.8450299335598));
#27464=CARTESIAN_POINT('Origin',(0.0835265683620477,-14.4544045823054,0.0824317919394229));
#27465=CARTESIAN_POINT('Origin',(30.6299435607004,-14.4544045823054,48.5813824935285));
#27466=CARTESIAN_POINT('Ctrl Pts',(39.89356043033,-13.5144022946802,38.546784061645));
#27467=CARTESIAN_POINT('Ctrl Pts',(40.16741768324,-13.1933434804542,38.6370886406434));
#27468=CARTESIAN_POINT('Ctrl Pts',(39.9535961475603,-13.2935409795845,38.9983049336294));
#27469=CARTESIAN_POINT('Ctrl Pts',(37.1165167598647,-10.8876754010549,37.6310523918765));
#27470=CARTESIAN_POINT('Ctrl Pts',(37.3635232200226,-10.5315615552175,37.7125029072161));
#27471=CARTESIAN_POINT('Ctrl Pts',(37.1730026303393,-10.6668492051076,38.0862419429111));
#27472=CARTESIAN_POINT('Ctrl Pts',(34.317603164163,-8.28316551656738,36.7081091022954));
#27473=CARTESIAN_POINT('Ctrl Pts',(34.5552513595784,-7.90880841716609,36.7864737246854));
#27474=CARTESIAN_POINT('Ctrl Pts',(34.3698847268169,-8.06235638062368,37.1673862145963));
#27475=CARTESIAN_POINT('Ctrl Pts',(31.4870706148097,-5.72100918219894,35.7747394454477));
#27476=CARTESIAN_POINT('Ctrl Pts',(31.7699448945489,-5.37442442931235,35.8680173939828));
#27477=CARTESIAN_POINT('Ctrl Pts',(31.5339848667978,-5.50017070815072,36.2386314339953));
#27478=CARTESIAN_POINT('Ctrl Pts',(32.9800027480559,-7.07886051013688,36.2670346332676));
#27479=CARTESIAN_POINT('Ctrl Pts',(32.9461473542254,-6.97591157389001,36.2558716399581));
#27480=CARTESIAN_POINT('Ctrl Pts',(32.8998932107597,-6.87711064623292,36.2543779568787));
#27481=CARTESIAN_POINT('Ctrl Pts',(32.7952737153869,-6.68740381001556,36.2619519765855));
#27482=CARTESIAN_POINT('Ctrl Pts',(32.7365767239536,-6.59673597566759,36.2713199677746));
#27483=CARTESIAN_POINT('Ctrl Pts',(32.6073736644662,-6.42451466437639,36.3005256432273));
#27484=CARTESIAN_POINT('Ctrl Pts',(32.5379837469721,-6.34396835910597,36.3199676903523));
#27485=CARTESIAN_POINT('Ctrl Pts',(32.4226478919156,-6.23614184370368,36.3601920496742));
#27486=CARTESIAN_POINT('Ctrl Pts',(32.3823733185026,-6.20250856262141,36.375458100475));
#27487=CARTESIAN_POINT('Ctrl Pts',(32.2976871155079,-6.14483638321709,36.4114968076452));
#27488=CARTESIAN_POINT('Ctrl Pts',(32.2530602303314,-6.11985717446073,36.4321140290926));
#27489=CARTESIAN_POINT('Ctrl Pts',(32.2061415763531,-6.10843371318469,36.4583066739833));
#27490=CARTESIAN_POINT('Origin',(33.0778695430594,-14.7669045823054,35.9702546803237));
#27491=CARTESIAN_POINT('Origin',(33.0778695430594,-7.07886995352309,35.9702546803237));
#27492=CARTESIAN_POINT('Ctrl Pts',(-34.088419713945,-10.7044045823054,34.4112752552593));
#27493=CARTESIAN_POINT('Ctrl Pts',(-34.088419713945,-11.0169045823054,34.4112752552593));
#27494=CARTESIAN_POINT('Ctrl Pts',(-33.8679555443817,-11.0169045823054,
34.1897988458186));
#27495=CARTESIAN_POINT('Ctrl Pts',(-34.1509161335726,-10.7044046073822,
34.3490644704238));
#27496=CARTESIAN_POINT('Ctrl Pts',(-34.1271612526014,-11.0349449313272,
34.3727107802124));
#27497=CARTESIAN_POINT('Ctrl Pts',(-33.8928554776138,-11.0169045823054,
34.1402540109324));
#27498=CARTESIAN_POINT('Ctrl Pts',(-34.2116574899238,-10.718650676671,34.2882601726245));
#27499=CARTESIAN_POINT('Ctrl Pts',(-34.1595985812887,-11.0630714156278,
34.3403466741461));
#27500=CARTESIAN_POINT('Ctrl Pts',(-33.9170059419221,-11.0240276257398,
34.0917785581122));
#27501=CARTESIAN_POINT('Ctrl Pts',(-34.3291018131802,-10.7765752156551,
34.1701033562228));
#27502=CARTESIAN_POINT('Ctrl Pts',(-34.2108367877319,-11.1314870357705,
34.289393364263));
#27503=CARTESIAN_POINT('Ctrl Pts',(-33.9636138355068,-11.0529899027286,
33.9974925425165));
#27504=CARTESIAN_POINT('Ctrl Pts',(-34.3825217718355,-10.8185639645428,
34.1160547845883));
#27505=CARTESIAN_POINT('Ctrl Pts',(-34.2270713855228,-11.1704305366382,
34.2733844817198));
#27506=CARTESIAN_POINT('Ctrl Pts',(-33.9847686082005,-11.0739842709863,
33.9543184859346));
#27507=CARTESIAN_POINT('Ctrl Pts',(-34.4774469307935,-10.9314866347395,
34.0196546156364));
#27508=CARTESIAN_POINT('Ctrl Pts',(-34.2431347603941,-11.2441510617705,
34.2581798507015));
#27509=CARTESIAN_POINT('Ctrl Pts',(-34.0223069043039,-11.1304456109602,
33.8772616585451));
#27510=CARTESIAN_POINT('Ctrl Pts',(-34.516023514239,-10.999293715727,33.9802793527558));
#27511=CARTESIAN_POINT('Ctrl Pts',(-34.2411034316767,-11.2750326114057,
34.2608486663205));
#27512=CARTESIAN_POINT('Ctrl Pts',(-34.0375326396835,-11.1643491474262,
33.845758314463));
#27513=CARTESIAN_POINT('Ctrl Pts',(-34.5707068729028,-11.1560957480195,
33.9243738132403));
#27514=CARTESIAN_POINT('Ctrl Pts',(-34.2319619401124,-11.3160025899707,
34.2712078036082));
#27515=CARTESIAN_POINT('Ctrl Pts',(-34.0591022197643,-11.2427501667525,
33.8010164090556));
#27516=CARTESIAN_POINT('Ctrl Pts',(-34.5853023188946,-11.2411599901507,
33.909398990258));
#27517=CARTESIAN_POINT('Ctrl Pts',(-34.2259804943108,-11.3235538600013,
34.2776633628159));
#27518=CARTESIAN_POINT('Ctrl Pts',(-34.0648514633374,-11.2852822850309,
33.7890241866258));
#27519=CARTESIAN_POINT('Ctrl Pts',(-34.585302306524,-11.3294045823054,33.9093990029365));
#27520=CARTESIAN_POINT('Ctrl Pts',(-34.2259804977875,-11.3294045823054,
34.2776633590166));
#27521=CARTESIAN_POINT('Ctrl Pts',(-34.064851465877,-11.3294045823054,33.7890241943272));
#27522=CARTESIAN_POINT('Origin',(-33.8679555443817,-10.7044045823054,34.1897988458186));
#27523=CARTESIAN_POINT('Origin',(-59.8897726849335,-14.4544045823054,3.01076271456695));
#27524=CARTESIAN_POINT('Origin',(-6.66906800894368,-14.4544045823054,20.5603192006674));
#27525=CARTESIAN_POINT('Ctrl Pts',(29.4562490573973,-14.4313124010515,48.5189176227355));
#27526=CARTESIAN_POINT('Ctrl Pts',(29.457027776463,-14.7671408702893,48.4940514111173));
#27527=CARTESIAN_POINT('Ctrl Pts',(29.4442069949301,-14.7669045053135,48.830622722352));
#27528=CARTESIAN_POINT('Ctrl Pts',(29.6580315031289,-14.4776157931207,48.5229453229308));
#27529=CARTESIAN_POINT('Ctrl Pts',(29.6408602063225,-14.7670932226436,48.5472967386214));
#27530=CARTESIAN_POINT('Ctrl Pts',(29.6700944519785,-14.766904515933,48.8386638059359));
#27531=CARTESIAN_POINT('Ctrl Pts',(29.8559183695444,-14.5232222287052,48.5151507121236));
#27532=CARTESIAN_POINT('Ctrl Pts',(29.8496672956075,-14.7670538266229,48.575617303287));
#27533=CARTESIAN_POINT('Ctrl Pts',(29.8920282667238,-14.7669045263941,48.8230549709512));
#27534=CARTESIAN_POINT('Ctrl Pts',(30.2414866202549,-14.6124212350924,48.4696579185046));
#27535=CARTESIAN_POINT('Ctrl Pts',(30.2582336836672,-14.7669897766123,48.5617748098557));
#27536=CARTESIAN_POINT('Ctrl Pts',(30.3251881717043,-14.7669045468573,48.7320256532131));
#27537=CARTESIAN_POINT('Ctrl Pts',(30.4336015879291,-14.6570503433836,48.4332503467984));
#27538=CARTESIAN_POINT('Ctrl Pts',(30.469015311734,-14.7669625172365,48.5287063091267));
#27539=CARTESIAN_POINT('Ctrl Pts',(30.5422656826559,-14.766904557097,48.6586455548447));
#27540=CARTESIAN_POINT('Ctrl Pts',(30.5955174348047,-14.6947854519679,48.3612871498227));
#27541=CARTESIAN_POINT('Ctrl Pts',(30.6513166085568,-14.7669413153261,48.4283359008911));
#27542=CARTESIAN_POINT('Ctrl Pts',(30.7234018036246,-14.7669045657556,48.5155428809447));
#27543=CARTESIAN_POINT('Origin',(29.5568100599416,-14.4544045823054,48.8324317919394));
#27544=CARTESIAN_POINT('Ctrl Pts',(30.5121796307591,-14.6753754514261,48.3944071427343));
#27545=CARTESIAN_POINT('Ctrl Pts',(30.4827135809989,-14.6685167481303,48.4048602007603));
#27546=CARTESIAN_POINT('Ctrl Pts',(30.4529177837429,-14.6615856670199,48.4142233306906));
#27547=CARTESIAN_POINT('Ctrl Pts',(30.4229080014734,-14.654609080261,48.4226966921314));
#27548=CARTESIAN_POINT('Ctrl Pts',(30.3899725761781,-14.6469523485344,48.4319961185727));
#27549=CARTESIAN_POINT('Ctrl Pts',(30.3567792072589,-14.6392407575338,48.4402238158605));
#27550=CARTESIAN_POINT('Ctrl Pts',(30.3234353759554,-14.6314992383768,48.4475985057719));
#27551=CARTESIAN_POINT('Ctrl Pts',(30.2877811427954,-14.62322130755,48.4554841896691));
#27552=CARTESIAN_POINT('Ctrl Pts',(30.2519542200175,-14.6149090026934,48.462394188985));
#27553=CARTESIAN_POINT('Ctrl Pts',(30.2160434238487,-14.6065829337796,48.4685491967709));
#27554=CARTESIAN_POINT('Ctrl Pts',(30.1745971023505,-14.5969734300696,48.4756529777708));
#27555=CARTESIAN_POINT('Ctrl Pts',(30.1330381930019,-14.5873453832253,48.4817509213698));
#27556=CARTESIAN_POINT('Ctrl Pts',(30.0914599002124,-14.5777205278759,48.4871254258683));
#27557=CARTESIAN_POINT('Ctrl Pts',(30.0772090127902,-14.5744216254719,48.4889675279226));
#27558=CARTESIAN_POINT('Ctrl Pts',(30.0629555875867,-14.5711230389444,48.4907242246678));
#27559=CARTESIAN_POINT('Ctrl Pts',(30.0487027977647,-14.5678255143184,48.4924057571001));
#27560=CARTESIAN_POINT('Ctrl Pts',(30.0453826879077,-14.5670573738946,48.492797460933));
#27561=CARTESIAN_POINT('Ctrl Pts',(30.0420612970355,-14.566288983565,48.4931847014103));
#27562=CARTESIAN_POINT('Ctrl Pts',(30.0387385202705,-14.5655203189317,48.4935675089594));
#27563=CARTESIAN_POINT('Ctrl Pts',(29.9531991516571,-14.5457323247158,48.5034222534608));
#27564=CARTESIAN_POINT('Ctrl Pts',(29.8673665740185,-14.5259112556569,48.5102733066289));
#27565=CARTESIAN_POINT('Ctrl Pts',(29.7812847600966,-14.5060682995347,48.5145218129766));
#27566=CARTESIAN_POINT('Ctrl Pts',(29.7066446881537,-14.4888628108834,48.5182056203338));
#27567=CARTESIAN_POINT('Ctrl Pts',(29.6318168465408,-14.471640756376,48.5199316495389));
#27568=CARTESIAN_POINT('Ctrl Pts',(29.5568193301503,-14.4544067125516,48.5199317919306));
#27569=CARTESIAN_POINT('Ctrl Pts',(33.0027879519579,-7.15534954830154,36.2773306483844));
#27570=CARTESIAN_POINT('Ctrl Pts',(32.4289011688471,-7.11664814650066,36.1423065419147));
#27571=CARTESIAN_POINT('Ctrl Pts',(32.8618763023223,-7.18677502441217,35.7443400681459));
#27572=CARTESIAN_POINT('Ctrl Pts',(32.9716799988102,-7.03238137399795,36.2577971857996));
#27573=CARTESIAN_POINT('Ctrl Pts',(32.5024026040697,-7.0802116255979,36.0750148926511));
#27574=CARTESIAN_POINT('Ctrl Pts',(32.8767232401359,-7.01162141055725,35.7306646429359));
#27575=CARTESIAN_POINT('Ctrl Pts',(32.9138507450232,-6.90078625141428,36.2533276469428));
#27576=CARTESIAN_POINT('Ctrl Pts',(32.5473708083471,-6.94927177584817,36.0332686286228));
#27577=CARTESIAN_POINT('Ctrl Pts',(32.8536713561474,-6.83269992244044,35.7519247260262));
#27578=CARTESIAN_POINT('Ctrl Pts',(32.7893956376618,-6.6769719555354,36.2629255337844));
#27579=CARTESIAN_POINT('Ctrl Pts',(32.5534537676943,-6.69622936404116,36.0265991852956));
#27580=CARTESIAN_POINT('Ctrl Pts',(32.7730615057291,-6.5379598519392,35.8257956190207));
#27581=CARTESIAN_POINT('Ctrl Pts',(32.7264182119996,-6.58104909157649,36.2733890195365));
#27582=CARTESIAN_POINT('Ctrl Pts',(32.5376034872748,-6.57996991860998,36.0406005265092));
#27583=CARTESIAN_POINT('Ctrl Pts',(32.7232297664787,-6.41511471179781,35.8713726932354));
#27584=CARTESIAN_POINT('Ctrl Pts',(32.5887048620014,-6.40173475569555,36.3057781064803));
#27585=CARTESIAN_POINT('Ctrl Pts',(32.4714094556764,-6.36383534698751,36.099753191065));
#27586=CARTESIAN_POINT('Ctrl Pts',(32.5984331925844,-6.1927844440631,35.9847905294333));
#27587=CARTESIAN_POINT('Ctrl Pts',(32.5160977586742,-6.32050524456458,36.3270146377757));
#27588=CARTESIAN_POINT('Ctrl Pts',(32.4250055767998,-6.26307762141852,36.1413505743537));
#27589=CARTESIAN_POINT('Ctrl Pts',(32.5257164089387,-6.09580032219768,36.0506055708441));
#27590=CARTESIAN_POINT('Ctrl Pts',(32.3399099210657,-6.1637311406324,36.3907537841966));
#27591=CARTESIAN_POINT('Ctrl Pts',(32.2870207252597,-6.07811517888562,36.2644473800673));
#27592=CARTESIAN_POINT('Ctrl Pts',(32.328360008767,-5.92198390398685,36.2277488375675));
#27593=CARTESIAN_POINT('Ctrl Pts',(32.2375253657692,-6.09886182626739,36.4356892719343));
#27594=CARTESIAN_POINT('Ctrl Pts',(32.1881882760276,-6.00005797775949,36.3522768460648));
#27595=CARTESIAN_POINT('Ctrl Pts',(32.1993930425981,-5.86097989287912,36.3425656526602));
#27596=CARTESIAN_POINT('Ctrl Pts',(32.151529404332,-6.10268725738615,36.4911916688128));
#27597=CARTESIAN_POINT('Ctrl Pts',(32.0828811597279,-6.01584203958569,36.4449524222502));
#27598=CARTESIAN_POINT('Ctrl Pts',(32.0626197531438,-5.89881153273095,36.4627624082688));
#27599=CARTESIAN_POINT('Origin',(32.3524078891946,-5.88746284406389,36.6239396741003));
#27600=CARTESIAN_POINT('Origin',(0.0835265683620477,-10.7044045823054,0.0824317919394229));
#27601=CARTESIAN_POINT('Origin',(-29.4954827078206,-10.7044045823054,38.0442262073711));
#27602=CARTESIAN_POINT('Origin',(-15.3043526660546,-11.3294045823054,-4.99172980493867));
#27603=CARTESIAN_POINT('Ctrl Pts',(-29.2671708193829,-11.3294045823054,
38.3497289413026));
#27604=CARTESIAN_POINT('Ctrl Pts',(-29.2671708193829,-11.3124780874426,
38.3497289413026));
#27605=CARTESIAN_POINT('Ctrl Pts',(-29.2681709348334,-11.2956902155653,
38.3483582338347));
#27606=CARTESIAN_POINT('Ctrl Pts',(-29.2701189073547,-11.2792729854166,
38.3457454172439));
#27607=CARTESIAN_POINT('Ctrl Pts',(-29.2720812584704,-11.2627345745579,
38.3431133146366));
#27608=CARTESIAN_POINT('Ctrl Pts',(-29.2750050109582,-11.2465729047032,
38.3392208633812));
#27609=CARTESIAN_POINT('Ctrl Pts',(-29.2787966186959,-11.2309934053141,
38.3342127608102));
#27610=CARTESIAN_POINT('Ctrl Pts',(-29.2826398264079,-11.2152018845814,
38.3291365029917));
#27611=CARTESIAN_POINT('Ctrl Pts',(-29.2873740682792,-11.2000089946043,
38.3229142203174));
#27612=CARTESIAN_POINT('Ctrl Pts',(-29.2928692140188,-11.1855875760929,
38.3157073854842));
#27613=CARTESIAN_POINT('Ctrl Pts',(-29.2984084509705,-11.1710504449412,
38.3084427254181));
#27614=CARTESIAN_POINT('Ctrl Pts',(-29.3047201288968,-11.1572975033337,
38.3001778885712));
#27615=CARTESIAN_POINT('Ctrl Pts',(-29.3116480970033,-11.1444582968067,
38.2910858047855));
#27616=CARTESIAN_POINT('Ctrl Pts',(-29.3186726108507,-11.1314401675872,
38.2818670168995));
#27617=CARTESIAN_POINT('Ctrl Pts',(-29.3263299526575,-11.1193615571096,
38.2717980151597));
#27618=CARTESIAN_POINT('Ctrl Pts',(-29.3344452291491,-11.1083055247257,
38.2610630578265));
#27619=CARTESIAN_POINT('Ctrl Pts',(-29.3371174699017,-11.1046649364684,
38.2575281948438));
#27620=CARTESIAN_POINT('Ctrl Pts',(-29.3398393167612,-11.1011348042002,
38.2539211386765));
#27621=CARTESIAN_POINT('Ctrl Pts',(-29.3426044572242,-11.0977168667273,
38.2502484905411));
#27622=CARTESIAN_POINT('Ctrl Pts',(-29.3526728339503,-11.0852715379768,
38.236875714183));
#27623=CARTESIAN_POINT('Ctrl Pts',(-29.3633753634814,-11.0742682117852,
38.2226616223712));
#27624=CARTESIAN_POINT('Ctrl Pts',(-29.3745114120525,-11.0647125800551,
38.2078123856294));
#27625=CARTESIAN_POINT('Ctrl Pts',(-29.3869785886498,-11.054014732653,38.1911881714288));
#27626=CARTESIAN_POINT('Ctrl Pts',(-29.3999889739614,-11.0451301475312,
38.1737679429712));
#27627=CARTESIAN_POINT('Ctrl Pts',(-29.4133192132405,-11.038042002362,38.1558218117586));
#27628=CARTESIAN_POINT('Ctrl Pts',(-29.4281479300946,-11.0301570653,38.1358583217711));
#27629=CARTESIAN_POINT('Ctrl Pts',(-29.4433733452703,-11.0244934293336,
38.1152437539762));
#27630=CARTESIAN_POINT('Ctrl Pts',(-29.4587509031789,-11.0210242012062,
38.0943291909816));
#27631=CARTESIAN_POINT('Ctrl Pts',(-29.4709331196514,-11.0182758527174,
38.077760517637));
#27632=CARTESIAN_POINT('Ctrl Pts',(-29.483212604426,-11.0169045823054,38.0610029810114));
#27633=CARTESIAN_POINT('Ctrl Pts',(-29.4954827078206,-11.0169045823054,
38.0442262073711));
#27634=CARTESIAN_POINT('Origin',(0.0835265683620477,-14.4544045823054,0.0824317919394229));
#27635=CARTESIAN_POINT('Origin',(-19.1024092026003,-14.4544045823054,9.9232282456065));
#27636=CARTESIAN_POINT('Origin',(-44.291473431638,-14.4544045823054,48.8324317919394));
#27637=CARTESIAN_POINT('Origin',(-29.3897569232175,-14.4544045823054,48.8324317919394));
#27638=CARTESIAN_POINT('Ctrl Pts',(-30.3730808079888,-14.9741386829693,
48.5199317919394));
#27639=CARTESIAN_POINT('Ctrl Pts',(-30.4470643284216,-14.8357920829891,
48.5199317919394));
#27640=CARTESIAN_POINT('Ctrl Pts',(-30.4912615099722,-14.7531448966905,
48.3941168692887));
#27641=CARTESIAN_POINT('Ctrl Pts',(-28.3257761438679,-13.879302911696,48.5199317919394));
#27642=CARTESIAN_POINT('Ctrl Pts',(-28.4030221988792,-13.7458678866789,
48.5199317919394));
#27643=CARTESIAN_POINT('Ctrl Pts',(-28.4382824252071,-13.658307532674,48.3977071667607));
#27644=CARTESIAN_POINT('Ctrl Pts',(-26.2427249084523,-12.8434482903011,
48.5199317919394));
#27645=CARTESIAN_POINT('Ctrl Pts',(-26.3156315690958,-12.7103751542413,
48.5199317919394));
#27646=CARTESIAN_POINT('Ctrl Pts',(-26.3489689847425,-12.6224528665242,
48.401314352775));
#27647=CARTESIAN_POINT('Ctrl Pts',(-23.0464978220819,-11.4077451872917,
48.5199317919394));
#27648=CARTESIAN_POINT('Ctrl Pts',(-23.1068226074019,-11.2735898053156,
48.5199317919394));
#27649=CARTESIAN_POINT('Ctrl Pts',(-23.1422761975804,-11.1867499400309,
48.4065777408208));
#27650=CARTESIAN_POINT('Ctrl Pts',(-21.9690884615937,-10.9489604127228,
48.5199317919394));
#27651=CARTESIAN_POINT('Ctrl Pts',(-22.0269387797156,-10.8151504288072,
48.5199317919394));
#27652=CARTESIAN_POINT('Ctrl Pts',(-22.0611987595185,-10.727965027292,48.4083066876547));
#27653=CARTESIAN_POINT('Ctrl Pts',(-19.7863880449052,-10.0773547210577,
48.5199317919394));
#27654=CARTESIAN_POINT('Ctrl Pts',(-19.8391964327606,-9.94441815657253,
48.5199317919394));
#27655=CARTESIAN_POINT('Ctrl Pts',(-19.8707744411429,-9.85635900888291,
48.4116714313723));
#27656=CARTESIAN_POINT('Ctrl Pts',(-18.6820153475912,-9.66512413195019,
48.5199317919394));
#27657=CARTESIAN_POINT('Ctrl Pts',(-18.7320875059833,-9.53246556458702,
48.5199317919394));
#27658=CARTESIAN_POINT('Ctrl Pts',(-18.7623480724567,-9.44412830208715,
48.4133051537846));
#27659=CARTESIAN_POINT('Ctrl Pts',(-13.1435402678133,-7.75733423685904,
48.5199317919394));
#27660=CARTESIAN_POINT('Ctrl Pts',(-13.2048611762757,-7.63508483860035,
48.5199317919394));
#27661=CARTESIAN_POINT('Ctrl Pts',(-13.2028224703124,-7.53633525782087,
48.4210275580482));
#27662=CARTESIAN_POINT('Ctrl Pts',(-8.61498664508566,-6.70462823795387,
48.5199317919394));
#27663=CARTESIAN_POINT('Ctrl Pts',(-8.64606183255299,-6.57519149762604,
48.5199317919394));
#27664=CARTESIAN_POINT('Ctrl Pts',(-8.6547070114339,-6.48363668556085,48.4258275002683));
#27665=CARTESIAN_POINT('Ctrl Pts',(-3.94919441148868,-6.31501530004509,
48.5199317919394));
#27666=CARTESIAN_POINT('Ctrl Pts',(-3.9600208103548,-6.18536424665137,48.5199317919394));
#27667=CARTESIAN_POINT('Ctrl Pts',(-3.96764857725177,-6.09401826674954,
48.427604462906));
#27668=CARTESIAN_POINT('Ctrl Pts',(-30.3451264940348,-14.6753754514262,
48.3944071427339));
#27669=CARTESIAN_POINT('Ctrl Pts',(-30.3179204768622,-14.6690428075473,
48.4040584559733));
#27670=CARTESIAN_POINT('Ctrl Pts',(-30.2904148515138,-14.662644201776,48.4127711185442));
#27671=CARTESIAN_POINT('Ctrl Pts',(-30.2627186133094,-14.656204897716,48.4207135901973));
#27672=CARTESIAN_POINT('Ctrl Pts',(-30.233332298686,-14.6493726552408,48.4291407263725));
#27673=CARTESIAN_POINT('Ctrl Pts',(-30.2037309448942,-14.6424944891886,
48.4367006178514));
#27674=CARTESIAN_POINT('Ctrl Pts',(-30.1740000760399,-14.6355902170491,
48.4435574472146));
#27675=CARTESIAN_POINT('Ctrl Pts',(-30.1408726297333,-14.6278971722979,
48.4511976291304));
#27676=CARTESIAN_POINT('Ctrl Pts',(-30.1075839758143,-14.6201716175816,
48.4579649341589));
#27677=CARTESIAN_POINT('Ctrl Pts',(-30.0742050848433,-14.6124300278826,
48.4640429319486));
#27678=CARTESIAN_POINT('Ctrl Pts',(-30.0371113350464,-14.6038268483589,
48.4707973723365));
#27679=CARTESIAN_POINT('Ctrl Pts',(-29.9999050324531,-14.5952036013938,
48.476700265973));
#27680=CARTESIAN_POINT('Ctrl Pts',(-29.9626404188634,-14.586573014867,48.4819545588626));
#27681=CARTESIAN_POINT('Ctrl Pts',(-29.9352609645243,-14.5802318582854,
48.4858150489737));
#27682=CARTESIAN_POINT('Ctrl Pts',(-29.9078489587586,-14.5738864928743,
48.489324267419));
#27683=CARTESIAN_POINT('Ctrl Pts',(-29.880419746453,-14.5675406076309,48.4925504988627));
#27684=CARTESIAN_POINT('Ctrl Pts',(-29.8775679819405,-14.5668808376697,
48.4928859241836));
#27685=CARTESIAN_POINT('Ctrl Pts',(-29.874715080232,-14.5662208392319,48.4932180901505));
#27686=CARTESIAN_POINT('Ctrl Pts',(-29.8718609472941,-14.5655605905129,
48.4935470170228));
#27687=CARTESIAN_POINT('Ctrl Pts',(-29.7770689367495,-14.543632283427,48.5044713993929));
#27688=CARTESIAN_POINT('Ctrl Pts',(-29.6819707966549,-14.5216757688499,
48.5117080083146));
#27689=CARTESIAN_POINT('Ctrl Pts',(-29.5866135500324,-14.4997031659203,
48.5157983084356));
#27690=CARTESIAN_POINT('Ctrl Pts',(-29.5211163517266,-14.4846110362463,
48.5186077771193));
#27691=CARTESIAN_POINT('Ctrl Pts',(-29.4554966227567,-14.4695112274358,
48.5199316661313));
#27692=CARTESIAN_POINT('Ctrl Pts',(-29.3897662870071,-14.454406734056,48.5199317919305));
#27693=CARTESIAN_POINT('Ctrl Pts',(30.6582665472115,-14.7531486984913,48.3941518139883));
#27694=CARTESIAN_POINT('Ctrl Pts',(30.6140688077616,-14.8357969973016,48.5199317919394));
#27695=CARTESIAN_POINT('Ctrl Pts',(30.5400981996473,-14.974119567612,48.5199317919394));
#27696=CARTESIAN_POINT('Ctrl Pts',(28.6057879598596,-13.6585793127033,48.3977403664122));
#27697=CARTESIAN_POINT('Ctrl Pts',(28.5705202880773,-13.7461362596172,48.5199317919394));
#27698=CARTESIAN_POINT('Ctrl Pts',(28.4932902065677,-13.8795503180319,48.5199317919394));
#27699=CARTESIAN_POINT('Ctrl Pts',(26.5172528199154,-12.6231097579372,48.4013453007044));
#27700=CARTESIAN_POINT('Ctrl Pts',(26.4839031110322,-12.7110265271892,48.5199317919394));
#27701=CARTESIAN_POINT('Ctrl Pts',(26.4110144314125,-12.8440806269522,48.5199317919394));
#27702=CARTESIAN_POINT('Ctrl Pts',(23.3123676663596,-11.1881005852588,48.4066046257084));
#27703=CARTESIAN_POINT('Ctrl Pts',(23.2769083268454,-11.2749369500996,48.5199317919394));
#27704=CARTESIAN_POINT('Ctrl Pts',(23.2165890826852,-11.4090714544326,48.5199317919394));
#27705=CARTESIAN_POINT('Ctrl Pts',(22.2320010273984,-10.7295656511261,48.4083321070107));
#27706=CARTESIAN_POINT('Ctrl Pts',(22.1977338841284,-10.816746996713,48.5199317919394));
#27707=CARTESIAN_POINT('Ctrl Pts',(22.1398875138931,-10.9505365201866,48.5199317919394));
#27708=CARTESIAN_POINT('Ctrl Pts',(20.0432673812065,-9.85847188921382,48.4116937938316));
#27709=CARTESIAN_POINT('Ctrl Pts',(20.0116798199932,-9.9465258837596,48.5199317919394));
#27710=CARTESIAN_POINT('Ctrl Pts',(19.9588702805472,-10.0794427583948,48.5199317919394));
#27711=CARTESIAN_POINT('Ctrl Pts',(18.9337330064251,-9.44570717935327,48.4133290604129));
#27712=CARTESIAN_POINT('Ctrl Pts',(18.9034696740469,-9.534041625569,48.5199317919394));
#27713=CARTESIAN_POINT('Ctrl Pts',(18.8533926908108,-9.66667804843112,48.5199317919394));
#27714=CARTESIAN_POINT('Ctrl Pts',(13.3694457519523,-7.53595817693225,48.421057068387));
#27715=CARTESIAN_POINT('Ctrl Pts',(13.3715217464864,-7.63471881015203,48.5199317919394));
#27716=CARTESIAN_POINT('Ctrl Pts',(13.3101634587761,-7.75692904622486,48.5199317919394));
#27717=CARTESIAN_POINT('Ctrl Pts',(8.81975013992703,-6.48350292012916,48.4258551364495));
#27718=CARTESIAN_POINT('Ctrl Pts',(8.81109698109706,-6.57505277909527,48.5199317919394));
#27719=CARTESIAN_POINT('Ctrl Pts',(8.78004147867651,-6.70446830385567,48.5199317919394));
#27720=CARTESIAN_POINT('Ctrl Pts',(4.1347721482036,-6.09405046754032,48.4276308774903));
#27721=CARTESIAN_POINT('Ctrl Pts',(4.12714461181649,-6.18539206100947,48.5199317919394));
#27722=CARTESIAN_POINT('Ctrl Pts',(4.11631983879343,-6.31502133666111,48.5199317919394));
#27723=CARTESIAN_POINT('Origin',(0.0835265683620477,-5.88746284406389,0.0824317919394229));
#27724=CARTESIAN_POINT('Ctrl Pts',(-29.160961539262,-11.3806731527506,38.6952753670064));
#27725=CARTESIAN_POINT('Ctrl Pts',(-29.338612324035,-11.3615458677611,38.5607229831505));
#27726=CARTESIAN_POINT('Ctrl Pts',(-29.267993840028,-11.355038329106,38.3486314652747));
#27727=CARTESIAN_POINT('Ctrl Pts',(-29.1469683092902,-11.1940655922236,
38.7058349957559));
#27728=CARTESIAN_POINT('Ctrl Pts',(-29.3277662394871,-11.2445867745137,
38.5690297012891));
#27729=CARTESIAN_POINT('Ctrl Pts',(-29.2619210862101,-11.2617365123088,
38.3565409866893));
#27730=CARTESIAN_POINT('Ctrl Pts',(-29.2108659223156,-11.005746982716,38.6576671929678));
#27731=CARTESIAN_POINT('Ctrl Pts',(-29.3785562365388,-11.1260887991107,
38.5301523333543));
#27732=CARTESIAN_POINT('Ctrl Pts',(-29.2896584450123,-11.1675791667462,
38.3204717498946));
#27733=CARTESIAN_POINT('Ctrl Pts',(-29.4288521077717,-10.7559199031752,
38.4911511473035));
#27734=CARTESIAN_POINT('Ctrl Pts',(-29.531320611788,-10.9974050092333,38.4122642469566));
#27735=CARTESIAN_POINT('Ctrl Pts',(-29.3839622465767,-11.0426657522701,
38.1953495467773));
#27736=CARTESIAN_POINT('Ctrl Pts',(-29.5822502088183,-10.6922226877682,
38.3730436187048));
#27737=CARTESIAN_POINT('Ctrl Pts',(-29.6355429628529,-10.989329898915,38.3313082128754));
#27738=CARTESIAN_POINT('Ctrl Pts',(-29.4501718643539,-11.0108152119631,
38.1064437698431));
#27739=CARTESIAN_POINT('Ctrl Pts',(-29.7276737536381,-10.7063374043602,
38.2594300539962));
#27740=CARTESIAN_POINT('Ctrl Pts',(-29.7095248998334,-11.0262754939016,
38.2736037579977));
#27741=CARTESIAN_POINT('Ctrl Pts',(-29.5127338402293,-11.0178704044763,
38.0205548953693));
#27742=CARTESIAN_POINT('Origin',(-28.9703898424448,-11.3294045823054,38.4475926308288));
#27743=CARTESIAN_POINT('Origin',(-19.6585232829181,-14.4544045823054,10.2084687225244));
#27744=CARTESIAN_POINT('Origin',(-20.2520852367942,-14.4544045823054,10.012741343472));
#27745=CARTESIAN_POINT('Ctrl Pts',(-29.3897569232175,-14.7669045823054,
48.8324317919395));
#27746=CARTESIAN_POINT('Ctrl Pts',(-29.3897569232175,-14.7669045823054,
48.5199317919395));
#27747=CARTESIAN_POINT('Ctrl Pts',(-29.3897569232175,-14.4544045823054,
48.5199317919395));
#27748=CARTESIAN_POINT('Ctrl Pts',(-29.5753563162698,-14.7669045823054,
48.8324317903168));
#27749=CARTESIAN_POINT('Ctrl Pts',(-29.546032736532,-14.7669045823054,48.5558431486859));
#27750=CARTESIAN_POINT('Ctrl Pts',(-29.5554686170235,-14.4924842730195,
48.5199317919395));
#27751=CARTESIAN_POINT('Ctrl Pts',(-29.7590263505073,-14.7669045823054,
48.8155939483766));
#27752=CARTESIAN_POINT('Ctrl Pts',(-29.7181422659514,-14.7669045823057,
48.5742539860857));
#27753=CARTESIAN_POINT('Ctrl Pts',(-29.7192039348074,-14.5302415322824,
48.5115128647378));
#27754=CARTESIAN_POINT('Ctrl Pts',(-30.1212331836543,-14.7669045823054,
48.7397392940007));
#27755=CARTESIAN_POINT('Ctrl Pts',(-30.0594836612501,-14.7669045823051,
48.5629091789621));
#27756=CARTESIAN_POINT('Ctrl Pts',(-30.0416350168231,-14.6048328837018,
48.4735855483903));
#27757=CARTESIAN_POINT('Ctrl Pts',(-30.3036979301853,-14.7669045823054,
48.6816475550023));
#27758=CARTESIAN_POINT('Ctrl Pts',(-30.2357168106316,-14.7669045823056,
48.5381854201266));
#27759=CARTESIAN_POINT('Ctrl Pts',(-30.2033686385937,-14.6423789509996,
48.4446955724101));
#27760=CARTESIAN_POINT('Ctrl Pts',(-30.4628904239763,-14.7669045823054,
48.5813824935285));
#27761=CARTESIAN_POINT('Ctrl Pts',(-30.3939059109749,-14.7669045823054,
48.4718548688625));
#27762=CARTESIAN_POINT('Ctrl Pts',(-30.3451264940348,-14.6753754514262,
48.3944071427339));
#27763=CARTESIAN_POINT('Origin',(-30.4628904239763,-14.4544045823054,48.5813824935285));
#27764=CARTESIAN_POINT('Ctrl Pts',(0.0835265683815503,-6.00666333723547,
48.5199460669664));
#27765=CARTESIAN_POINT('Ctrl Pts',(0.0835265683810243,-5.9853111687807,
48.5199456014727));
#27766=CARTESIAN_POINT('Ctrl Pts',(0.0835265683704475,-5.96223275463529,
48.5195872927805));
#27767=CARTESIAN_POINT('Ctrl Pts',(0.0835265683683665,-5.92795641804995,
48.5154826407816));
#27768=CARTESIAN_POINT('Ctrl Pts',(0.0835265683679874,-5.90583775506839,
48.5199317919394));
#27769=CARTESIAN_POINT('Ctrl Pts',(0.0835265683620106,-5.88746284406389,
48.5199317919394));
#27770=CARTESIAN_POINT('Ctrl Pts',(-0.267518736492766,-6.00132529512186,
48.519945950593));
#27771=CARTESIAN_POINT('Ctrl Pts',(-0.189662915894568,-5.98270666392106,
48.5198859104319));
#27772=CARTESIAN_POINT('Ctrl Pts',(-0.172476876202251,-5.9624068608038,
48.5196215918924));
#27773=CARTESIAN_POINT('Ctrl Pts',(-0.194279273758627,-5.92787973562319,
48.5154600083357));
#27774=CARTESIAN_POINT('Ctrl Pts',(-0.233267711014883,-5.90583775506839,
48.5199317919395));
#27775=CARTESIAN_POINT('Ctrl Pts',(-0.267760844335869,-5.88746284406389,
48.5199317919394));
#27776=CARTESIAN_POINT('Ctrl Pts',(-0.61861597912618,-5.99973567328081,
48.5184885224508));
#27777=CARTESIAN_POINT('Ctrl Pts',(-0.485248141372782,-5.98152768121125,
48.5186918880749));
#27778=CARTESIAN_POINT('Ctrl Pts',(-0.459481328260318,-5.96239709811729,
48.51825758671));
#27779=CARTESIAN_POINT('Ctrl Pts',(-0.500506504809839,-5.92723732580309,
48.5133469044267));
#27780=CARTESIAN_POINT('Ctrl Pts',(-0.567298494478176,-5.90562906540035,
48.5168141308037));
#27781=CARTESIAN_POINT('Ctrl Pts',(-0.619048262304899,-5.88746284406389,
48.5161104362146));
#27782=CARTESIAN_POINT('Ctrl Pts',(-1.32094154226152,-5.99820579736984,
48.5087577021076));
#27783=CARTESIAN_POINT('Ctrl Pts',(-1.12790203317576,-5.97907559060225,
48.5103258779008));
#27784=CARTESIAN_POINT('Ctrl Pts',(-1.09571051581296,-5.96099214798813,
48.509167391218));
#27785=CARTESIAN_POINT('Ctrl Pts',(-1.16018842027523,-5.92511301754142,
48.502095049591));
#27786=CARTESIAN_POINT('Ctrl Pts',(-1.25685784210449,-5.9049506781467,48.5026532295389));
#27787=CARTESIAN_POINT('Ctrl Pts',(-1.32154021141508,-5.88746284406389,
48.50082319184));
#27788=CARTESIAN_POINT('Ctrl Pts',(-1.67216986276346,-5.99826554329992,
48.5004843099067));
#27789=CARTESIAN_POINT('Ctrl Pts',(-1.47497921394887,-5.97774718230281,
48.503027618363));
#27790=CARTESIAN_POINT('Ctrl Pts',(-1.44494172976745,-5.95954166014524,
48.501314877539));
#27791=CARTESIAN_POINT('Ctrl Pts',(-1.51364329257245,-5.92360346889973,
48.4928930594133));
#27792=CARTESIAN_POINT('Ctrl Pts',(-1.61238233956212,-5.90448098056108,
48.4916098859259));
#27793=CARTESIAN_POINT('Ctrl Pts',(-1.67274475309919,-5.88746284406389,
48.489357302818));
#27794=CARTESIAN_POINT('Ctrl Pts',(-2.37478478398615,-5.99418693015723,
48.4732202209247));
#27795=CARTESIAN_POINT('Ctrl Pts',(-2.22731576266703,-5.97194742955367,
48.4746917382575));
#27796=CARTESIAN_POINT('Ctrl Pts',(-2.20580868408144,-5.95413393118541,
48.4721918658702));
#27797=CARTESIAN_POINT('Ctrl Pts',(-2.25808685942607,-5.91998502842415,
48.4637155122428));
#27798=CARTESIAN_POINT('Ctrl Pts',(-2.33187211335798,-5.90343694889074,
48.4610292841225));
#27799=CARTESIAN_POINT('Ctrl Pts',(-2.37498775707879,-5.88746284406389,
48.4587755322629));
#27800=CARTESIAN_POINT('Ctrl Pts',(-2.72575170752853,-5.99381953117216,
48.4556040546437));
#27801=CARTESIAN_POINT('Ctrl Pts',(-2.60287727359779,-5.97081802552583,
48.4559496853464));
#27802=CARTESIAN_POINT('Ctrl Pts',(-2.5878494531497,-5.95257589046842,48.4528734062221));
#27803=CARTESIAN_POINT('Ctrl Pts',(-2.63432748026306,-5.91860436677926,
48.4445443128869));
#27804=CARTESIAN_POINT('Ctrl Pts',(-2.69583332782557,-5.90286261480602,
48.4414922321791));
#27805=CARTESIAN_POINT('Ctrl Pts',(-2.72602622991915,-5.88746284406389,
48.439659649984));
#27806=CARTESIAN_POINT('Ctrl Pts',(-3.42730927258553,-5.99717808806687,
48.4131737559685));
#27807=CARTESIAN_POINT('Ctrl Pts',(-3.35965513432601,-5.97321241327165,
48.40967665781));
#27808=CARTESIAN_POINT('Ctrl Pts',(-3.35545842699348,-5.9531419369947,48.4051808771911));
#27809=CARTESIAN_POINT('Ctrl Pts',(-3.38522478840966,-5.9173715840225,48.3973032871653));
#27810=CARTESIAN_POINT('Ctrl Pts',(-3.4191878571586,-5.90176568155595,48.3944770847015));
#27811=CARTESIAN_POINT('Ctrl Pts',(-3.42785327106268,-5.8874628440639,48.3937688119853));
#27812=CARTESIAN_POINT('Ctrl Pts',(-3.77789991410016,-6.00090404394665,
48.3883596235742));
#27813=CARTESIAN_POINT('Ctrl Pts',(-3.74087148412348,-5.97673620504531,
48.3821456831845));
#27814=CARTESIAN_POINT('Ctrl Pts',(-3.74102460738878,-5.95526602423798,
48.3768070663123));
#27815=CARTESIAN_POINT('Ctrl Pts',(-3.75987742959583,-5.91751946291062,
48.3692339775274));
#27816=CARTESIAN_POINT('Ctrl Pts',(-3.77857712853757,-5.9012430823906,48.3669995056146));
#27817=CARTESIAN_POINT('Ctrl Pts',(-3.77864184991379,-5.8874628440639,48.3669938551438));
#27818=CARTESIAN_POINT('Ctrl Pts',(-4.128454810656,-6.007051447105,48.3603316468569));
#27819=CARTESIAN_POINT('Ctrl Pts',(-4.12834943621599,-5.98314272027372,
48.3503998997031));
#27820=CARTESIAN_POINT('Ctrl Pts',(-4.12855150591046,-5.95992641567859,
48.3444127441005));
#27821=CARTESIAN_POINT('Ctrl Pts',(-4.12900833251941,-5.91876732373882,
48.3374043064722));
#27822=CARTESIAN_POINT('Ctrl Pts',(-4.12926308943388,-5.90082453639418,
48.3363830244465));
#27823=CARTESIAN_POINT('Ctrl Pts',(-4.12926308943388,-5.88746284406389,
48.3363830244465));
#27824=CARTESIAN_POINT('Origin',(-4.15507771262755,-5.88723161925861,48.6489825986039));
#27825=CARTESIAN_POINT('Origin',(-28.9703898424448,-14.7669045823054,38.4475926308288));
#27826=CARTESIAN_POINT('Origin',(-28.9703898424448,-12.8919045823054,38.4475926308288));
#27827=CARTESIAN_POINT('Origin',(-15.3043526660546,-14.4544045823054,-4.99172980493867));
#27828=CARTESIAN_POINT('Origin',(-32.2904773922958,-14.4544045823054,46.520314294909));
#27829=CARTESIAN_POINT('Origin',(0.0835265683620477,-14.4544045823054,0.0824317919394229));
#27830=CARTESIAN_POINT('Origin',(-32.0889297465829,-14.4544045823054,47.5183344911391));
#27831=CARTESIAN_POINT('Origin',(0.0835265683620477,-5.88746284406389,0.0824317919394229));
#27832=CARTESIAN_POINT('Origin',(-27.4181833845098,-5.88746284406389,40.3343690082786));
#27833=CARTESIAN_POINT('Origin',(-27.8490907775129,-14.7669045823054,40.036547827824));
#27834=CARTESIAN_POINT('Origin',(-27.8490907775129,-12.8919045823054,40.036547827824));
#27835=CARTESIAN_POINT('Origin',(-27.8490907775129,-6.59535043767466,40.036547827824));
#27836=CARTESIAN_POINT('Origin',(0.0835265683620477,-12.8919045823054,0.0824317919394229));
#27837=CARTESIAN_POINT('Ctrl Pts',(-29.1590516373201,-12.8919045823054,
38.6967170518605));
#27838=CARTESIAN_POINT('Ctrl Pts',(-29.1590516373201,-12.9139187960392,
38.6967170518605));
#27839=CARTESIAN_POINT('Ctrl Pts',(-29.1591848624577,-12.9356278245217,
38.6997029556855));
#27840=CARTESIAN_POINT('Ctrl Pts',(-29.159433947161,-12.9566097073225,38.7052239565964));
#27841=CARTESIAN_POINT('Ctrl Pts',(-29.1596773251019,-12.9771108756619,
38.7106184662385));
#27842=CARTESIAN_POINT('Ctrl Pts',(-29.1600313014214,-12.9969176625769,
38.7184329690427));
#27843=CARTESIAN_POINT('Ctrl Pts',(-29.1604800625459,-13.0156824718651,
38.7282608271112));
#27844=CARTESIAN_POINT('Ctrl Pts',(-29.1609427003112,-13.0350275286535,
38.7383925832896));
#27845=CARTESIAN_POINT('Ctrl Pts',(-29.1615060596073,-13.0532645768225,
38.7506637210088));
#27846=CARTESIAN_POINT('Ctrl Pts',(-29.1621534535084,-13.0700686738455,
38.7646490220121));
#27847=CARTESIAN_POINT('Ctrl Pts',(-29.1627579434982,-13.0857591343535,
38.7777074929781));
#27848=CARTESIAN_POINT('Ctrl Pts',(-29.1634356985008,-13.1002006435726,
38.7922604647321));
#27849=CARTESIAN_POINT('Ctrl Pts',(-29.1641737792839,-13.1131767225616,
38.8079815149163));
#27850=CARTESIAN_POINT('Ctrl Pts',(-29.1642261648535,-13.1140977047964,
38.8090973225455));
#27851=CARTESIAN_POINT('Ctrl Pts',(-29.1642788546012,-13.1150113249639,
38.8102190230898));
#27852=CARTESIAN_POINT('Ctrl Pts',(-29.1643318440343,-13.1159175149051,
38.8113465038983));
#27853=CARTESIAN_POINT('Ctrl Pts',(-29.1644679206162,-13.1182446058459,
38.8142418686074));
#27854=CARTESIAN_POINT('Ctrl Pts',(-29.16460601967,-13.1205242789863,38.817174852995));
#27855=CARTESIAN_POINT('Ctrl Pts',(-29.1647460246345,-13.1227565895721,
38.8201428584547));
#27856=CARTESIAN_POINT('Ctrl Pts',(-29.1654262109927,-13.1336018279011,
38.8345623244452));
#27857=CARTESIAN_POINT('Ctrl Pts',(-29.1661478962618,-13.1433259542984,
38.8497998614965));
#27858=CARTESIAN_POINT('Ctrl Pts',(-29.1669018579151,-13.1519718238984,
38.8656404993433));
#27859=CARTESIAN_POINT('Ctrl Pts',(-29.1677243343596,-13.1614033699958,
38.8829206241859));
#27860=CARTESIAN_POINT('Ctrl Pts',(-29.1685852378023,-13.1695524259102,
38.9009190345409));
#27861=CARTESIAN_POINT('Ctrl Pts',(-29.1694755597606,-13.1764446443666,
38.9194128816111));
#27862=CARTESIAN_POINT('Ctrl Pts',(-29.1704025310331,-13.1836205748858,
38.9386680115012));
#27863=CARTESIAN_POINT('Ctrl Pts',(-29.1713614497358,-13.189434638032,38.9584615530468));
#27864=CARTESIAN_POINT('Ctrl Pts',(-29.1723445987337,-13.1938753423316,
38.9785843074176));
#27865=CARTESIAN_POINT('Ctrl Pts',(-29.173333254577,-13.198340920045,38.9988197739984));
#27866=CARTESIAN_POINT('Ctrl Pts',(-29.1743464900272,-13.2014181302593,
39.019389799867));
#27867=CARTESIAN_POINT('Ctrl Pts',(-29.1753778401591,-13.2030479859147,
39.0401003436967));
#27868=CARTESIAN_POINT('Ctrl Pts',(-29.1759465980169,-13.2039468011497,
39.0515215712493));
#27869=CARTESIAN_POINT('Ctrl Pts',(-29.1765208826526,-13.2044045823054,
39.0629857191608));
#27870=CARTESIAN_POINT('Ctrl Pts',(-29.1770996549272,-13.2044045823054,
39.0744598620586));
#27871=CARTESIAN_POINT('Origin',(-27.8490907775129,-12.8919045823054,40.036547827824));
#27872=CARTESIAN_POINT('Ctrl Pts',(-29.2671708193829,-12.8919045823054,
38.3497289413026));
#27873=CARTESIAN_POINT('Ctrl Pts',(-29.3371224979176,-12.8919045823054,
38.5618640814605));
#27874=CARTESIAN_POINT('Ctrl Pts',(-29.1590516373201,-12.8919045823054,
38.6967170518605));
#27875=CARTESIAN_POINT('Ctrl Pts',(-29.2671708452715,-13.0608832998913,
38.3497290198124));
#27876=CARTESIAN_POINT('Ctrl Pts',(-29.3371225173464,-12.9975414109162,
38.5618641403768));
#27877=CARTESIAN_POINT('Ctrl Pts',(-29.1590516158475,-12.9763939382002,
38.6967170681218));
#27878=CARTESIAN_POINT('Ctrl Pts',(-29.2911696270366,-13.2263898891536,
38.4225076155515));
#27879=CARTESIAN_POINT('Ctrl Pts',(-29.3560557745662,-13.1003236725309,
38.6192810495675));
#27880=CARTESIAN_POINT('Ctrl Pts',(-29.161014348867,-13.0591472399316,38.7407134375252));
#27881=CARTESIAN_POINT('Ctrl Pts',(-29.3684014298945,-13.4534586900117,
38.6567204274108));
#27882=CARTESIAN_POINT('Ctrl Pts',(-29.4103322473219,-13.2166231342357,
38.7838796324259));
#27883=CARTESIAN_POINT('Ctrl Pts',(-29.1676166638971,-13.1726816319565,
38.881996315062));
#27884=CARTESIAN_POINT('Ctrl Pts',(-29.4214900734496,-13.5169045492971,
38.817716804871));
#27885=CARTESIAN_POINT('Ctrl Pts',(-29.4461016930836,-13.2287751252092,
38.8923538899239));
#27886=CARTESIAN_POINT('Ctrl Pts',(-29.1722839318329,-13.2044045823054,
38.9789882968653));
#27887=CARTESIAN_POINT('Ctrl Pts',(-29.4738806318652,-13.5169045823054,
38.9765961725324));
#27888=CARTESIAN_POINT('Ctrl Pts',(-29.4738806318652,-13.2044045823054,
38.9765961725324));
#27889=CARTESIAN_POINT('Ctrl Pts',(-29.1770996549272,-13.2044045823054,
39.0744598620586));
#27890=CARTESIAN_POINT('Origin',(-29.1770996549271,-13.5169045823054,39.0744598620586));
#27891=CARTESIAN_POINT('Ctrl Pts',(-31.9662912555927,-14.4267018210596,
46.5416570520116));
#27892=CARTESIAN_POINT('Ctrl Pts',(-31.938168182706,-14.766904582306,46.5537176466009));
#27893=CARTESIAN_POINT('Ctrl Pts',(-32.2529109022529,-14.7669045823054,
46.4201248733199));
#27894=CARTESIAN_POINT('Ctrl Pts',(-32.024734683047,-14.4797609665061,46.692175136077));
#27895=CARTESIAN_POINT('Ctrl Pts',(-32.043778675644,-14.7669045823045,46.6631128135208));
#27896=CARTESIAN_POINT('Ctrl Pts',(-32.3355543111131,-14.7669045823054,
46.6161921183141));
#27897=CARTESIAN_POINT('Ctrl Pts',(-32.0623733364669,-14.5360769750825,
46.8596692968509));
#27898=CARTESIAN_POINT('Ctrl Pts',(-32.1316825592432,-14.7669045823054,
46.8406276275195));
#27899=CARTESIAN_POINT('Ctrl Pts',(-32.3745755896651,-14.7669045823054,
46.8402083581988));
#27900=CARTESIAN_POINT('Ctrl Pts',(-32.0633148172228,-14.6333609973512,
47.1698657294858));
#27901=CARTESIAN_POINT('Ctrl Pts',(-32.1580599963963,-14.7669045823054,
47.1930718120375));
#27902=CARTESIAN_POINT('Ctrl Pts',(-32.3135212074945,-14.7669045823054,
47.2692900755125));
#27903=CARTESIAN_POINT('Ctrl Pts',(-32.0263650896152,-14.6768299128524,
47.3206255170885));
#27904=CARTESIAN_POINT('Ctrl Pts',(-32.1082092307808,-14.7669045823054,
47.3875168727934));
#27905=CARTESIAN_POINT('Ctrl Pts',(-32.2106516131303,-14.7669045823054,
47.4860887252743));
#27906=CARTESIAN_POINT('Ctrl Pts',(-31.9150640676236,-14.6796363815821,
47.3662735732131));
#27907=CARTESIAN_POINT('Ctrl Pts',(-31.9437759414398,-14.7669045823054,
47.452789218383));
#27908=CARTESIAN_POINT('Ctrl Pts',(-31.9869047021237,-14.7669045823054,
47.5712759627658));
#27909=CARTESIAN_POINT('Ctrl Pts',(-31.9648970362263,-14.6753754514101,
47.3354574511519));
#27910=CARTESIAN_POINT('Ctrl Pts',(-31.9735564605727,-14.6738626255535,
47.3277564171069));
#27911=CARTESIAN_POINT('Ctrl Pts',(-31.9814148868573,-14.672133306496,47.3193746779532));
#27912=CARTESIAN_POINT('Ctrl Pts',(-31.9885249956109,-14.6701816478973,
47.3104973988125));
#27913=CARTESIAN_POINT('Ctrl Pts',(-31.9958630049577,-14.6681674327095,
47.3013355758973));
#27914=CARTESIAN_POINT('Ctrl Pts',(-32.0024049887865,-14.6659157786115,
47.2916462220175));
#27915=CARTESIAN_POINT('Ctrl Pts',(-32.0082456503293,-14.6634429331545,
47.2815977859672));
#27916=CARTESIAN_POINT('Ctrl Pts',(-32.0144118761709,-14.6608322488258,
47.2709892400711));
#27917=CARTESIAN_POINT('Ctrl Pts',(-32.0197975133047,-14.6579745808513,
47.2599805552063));
#27918=CARTESIAN_POINT('Ctrl Pts',(-32.0245374663174,-14.6549226264771,
47.2487281978874));
#27919=CARTESIAN_POINT('Ctrl Pts',(-32.0294338809134,-14.6517699298356,
47.2371044103797));
#27920=CARTESIAN_POINT('Ctrl Pts',(-32.0336423882984,-14.6484098887067,
47.2252202530633));
#27921=CARTESIAN_POINT('Ctrl Pts',(-32.0373183972508,-14.6449389709832,
47.2132071216528));
#27922=CARTESIAN_POINT('Ctrl Pts',(-32.0411624851728,-14.6413093517216,
47.2006447111801));
#27923=CARTESIAN_POINT('Ctrl Pts',(-32.044425251709,-14.6375586122338,47.1879408085633));
#27924=CARTESIAN_POINT('Ctrl Pts',(-32.0472750829195,-14.6338375655311,
47.1752077273099));
#27925=CARTESIAN_POINT('Ctrl Pts',(-32.0478441028572,-14.6330945917876,
47.1726653391589));
#27926=CARTESIAN_POINT('Ctrl Pts',(-32.0483966054282,-14.6323529212119,
47.1701216848644));
#27927=CARTESIAN_POINT('Ctrl Pts',(-32.048933839889,-14.6316139267957,47.1675775138247));
#27928=CARTESIAN_POINT('Ctrl Pts',(-32.0526337697119,-14.6265244776274,
47.150055826385));
#27929=CARTESIAN_POINT('Ctrl Pts',(-32.0555021961016,-14.621344309823,47.1323873234176));
#27930=CARTESIAN_POINT('Ctrl Pts',(-32.0576643305193,-14.6160583702073,
47.114661556595));
#27931=CARTESIAN_POINT('Ctrl Pts',(-32.0599055390581,-14.6105791118847,
47.096287518591));
#27932=CARTESIAN_POINT('Ctrl Pts',(-32.0613890113421,-14.6049864174434,
47.0778513515879));
#27933=CARTESIAN_POINT('Ctrl Pts',(-32.0622469744254,-14.5993048356888,
47.0594133334773));
#27934=CARTESIAN_POINT('Ctrl Pts',(-32.0631510114803,-14.5933181440278,
47.0399851646972));
#27935=CARTESIAN_POINT('Ctrl Pts',(-32.0633615554861,-14.587233162304,47.0205542044588));
#27936=CARTESIAN_POINT('Ctrl Pts',(-32.0630080810849,-14.5811189364166,
47.0011584488534));
#27937=CARTESIAN_POINT('Ctrl Pts',(-32.0628890789164,-14.5790604955872,
46.9946285927458));
#27938=CARTESIAN_POINT('Ctrl Pts',(-32.0627058827591,-14.5769990340003,
46.9881025171608));
#27939=CARTESIAN_POINT('Ctrl Pts',(-32.06246257273,-14.5749379971507,46.9815811346738));
#27940=CARTESIAN_POINT('Ctrl Pts',(-32.0615130688658,-14.5668949154069,
46.9561318020068));
#27941=CARTESIAN_POINT('Ctrl Pts',(-32.0596357617387,-14.5588253828889,
46.9307664425349));
#27942=CARTESIAN_POINT('Ctrl Pts',(-32.0569499598408,-14.5507005312891,
46.905520730097));
#27943=CARTESIAN_POINT('Ctrl Pts',(-32.0540210533122,-14.5418402609492,
46.8779899088413));
#27944=CARTESIAN_POINT('Ctrl Pts',(-32.0501318587241,-14.5329148917832,
46.8506002843932));
#27945=CARTESIAN_POINT('Ctrl Pts',(-32.045398488845,-14.5239279943262,46.8233693228353));
#27946=CARTESIAN_POINT('Ctrl Pts',(-32.0404602839034,-14.5145521917657,
46.7949599501544));
#27947=CARTESIAN_POINT('Ctrl Pts',(-32.0346035375997,-14.5051108161098,
46.7667217647601));
#27948=CARTESIAN_POINT('Ctrl Pts',(-32.0279080163951,-14.4956334644579,
46.7386659092895));
#27949=CARTESIAN_POINT('Ctrl Pts',(-32.0209363322123,-14.4857652106525,
46.7094528640549));
#27950=CARTESIAN_POINT('Ctrl Pts',(-32.0130546915264,-14.4758595759615,
46.6804360413191));
#27951=CARTESIAN_POINT('Ctrl Pts',(-32.0042998405545,-14.4659531415325,
46.651642384214));
#27952=CARTESIAN_POINT('Ctrl Pts',(-32.0008975616248,-14.4621033383507,
46.6404526959834));
#27953=CARTESIAN_POINT('Ctrl Pts',(-31.9973629090797,-14.4582533144174,
46.6292969765153));
#27954=CARTESIAN_POINT('Ctrl Pts',(-31.9936964222114,-14.4544045595354,
46.6181780052196));
#27955=CARTESIAN_POINT('Ctrl Pts',(-27.2935253998823,-6.10843371318469,
40.1519176123711));
#27956=CARTESIAN_POINT('Ctrl Pts',(-27.2418903719914,-6.01690458230549,
40.0763437697123));
#27957=CARTESIAN_POINT('Ctrl Pts',(-27.2418903719914,-5.88746284406389,
40.0763437697123));
#27958=CARTESIAN_POINT('Ctrl Pts',(-27.325572359156,-6.10275018345656,40.1231384197862));
#27959=CARTESIAN_POINT('Ctrl Pts',(-27.2900413002514,-6.01222811250085,
40.0434451574011));
#27960=CARTESIAN_POINT('Ctrl Pts',(-27.3090641493039,-5.88746285448576,
40.0304479975372));
#27961=CARTESIAN_POINT('Ctrl Pts',(-27.3592234999427,-6.1141957746084,40.0998270880335));
#27962=CARTESIAN_POINT('Ctrl Pts',(-27.3386284262519,-6.02882146164725,
40.0101249754889));
#27963=CARTESIAN_POINT('Ctrl Pts',(-27.3762231578696,-5.91065570868276,
39.9842903529062));
#27964=CARTESIAN_POINT('Ctrl Pts',(-27.4199070979359,-6.16774318631831,
40.0709901510091));
#27965=CARTESIAN_POINT('Ctrl Pts',(-27.4166158072636,-6.09780352750759,
39.9565255115711));
#27966=CARTESIAN_POINT('Ctrl Pts',(-27.4898455402218,-5.99623773973482,
39.9058585933618));
#27967=CARTESIAN_POINT('Ctrl Pts',(-27.4472128335106,-6.20950986590621,
40.065114733074));
#27968=CARTESIAN_POINT('Ctrl Pts',(-27.446986984373,-6.15046547604274,39.9355946057315));
#27969=CARTESIAN_POINT('Ctrl Pts',(-27.5371343265496,-6.05824038173979,
39.8730380903669));
#27970=CARTESIAN_POINT('Ctrl Pts',(-27.5138459772748,-6.35463014070743,
40.068359994813));
#27971=CARTESIAN_POINT('Ctrl Pts',(-27.5066521003082,-6.32861804115436,
39.8945248287816));
#27972=CARTESIAN_POINT('Ctrl Pts',(-27.6431152180442,-6.26685602924669,
39.7993318216615));
#27973=CARTESIAN_POINT('Ctrl Pts',(-27.5397129060577,-6.47617237885517,
40.0962102326933));
#27974=CARTESIAN_POINT('Ctrl Pts',(-27.5039315392958,-6.4727604437398,39.8965578930712));
#27975=CARTESIAN_POINT('Ctrl Pts',(-27.6700355544528,-6.43425950785917,
39.7804316879677));
#27976=CARTESIAN_POINT('Ctrl Pts',(-27.5523098005748,-6.59535043767466,
40.1344115173502));
#27977=CARTESIAN_POINT('Ctrl Pts',(-27.4795079208223,-6.59535043767466,
39.9136328700245));
#27978=CARTESIAN_POINT('Ctrl Pts',(-27.6700355381162,-6.59535043767466,
39.7804316993888));
#27979=CARTESIAN_POINT('Ctrl Pts',(-27.5523097639759,-6.59535009141677,
40.1344114063608));
#27980=CARTESIAN_POINT('Ctrl Pts',(-27.549694674541,-6.57060902178217,40.1264809184535));
#27981=CARTESIAN_POINT('Ctrl Pts',(-27.5464955216116,-6.5457384076949,40.1189472692866));
#27982=CARTESIAN_POINT('Ctrl Pts',(-27.5426476143085,-6.52084484397761,
40.1119507718129));
#27983=CARTESIAN_POINT('Ctrl Pts',(-27.5397616703681,-6.50217458409161,
40.1067033742282));
#27984=CARTESIAN_POINT('Ctrl Pts',(-27.5365106509872,-6.48349034080867,
40.1017592884795));
#27985=CARTESIAN_POINT('Ctrl Pts',(-27.532847416671,-6.46482870577695,40.0971928287498));
#27986=CARTESIAN_POINT('Ctrl Pts',(-27.5314737038024,-6.45783059264005,
40.0954804063511));
#27987=CARTESIAN_POINT('Ctrl Pts',(-27.5300417965966,-6.45083562442592,
40.0938211965667));
#27988=CARTESIAN_POINT('Ctrl Pts',(-27.5285483060168,-6.44384570105556,
40.0922194417591));
#27989=CARTESIAN_POINT('Ctrl Pts',(-27.5259346975023,-6.43161333515741,
40.0894163708458));
#27990=CARTESIAN_POINT('Ctrl Pts',(-27.5231328183895,-6.41939631908899,
40.0867892506081));
#27991=CARTESIAN_POINT('Ctrl Pts',(-27.5201202176626,-6.40720563047245,
40.0843613974034));
#27992=CARTESIAN_POINT('Ctrl Pts',(-27.5156013165723,-6.38891959754764,
40.0807196175964));
#27993=CARTESIAN_POINT('Ctrl Pts',(-27.5106097081556,-6.37069173964469,
40.077526777822));
#27994=CARTESIAN_POINT('Ctrl Pts',(-27.5050448441814,-6.35256977567836,
40.0748589437388));
#27995=CARTESIAN_POINT('Ctrl Pts',(-27.5022624121943,-6.34350879369519,
40.0735250266972));
#27996=CARTESIAN_POINT('Ctrl Pts',(-27.4993360567762,-6.3344747311239,40.0723220518095));
#27997=CARTESIAN_POINT('Ctrl Pts',(-27.4962499309249,-6.32547111501694,
40.0712411903706));
#27998=CARTESIAN_POINT('Ctrl Pts',(-27.4947068679993,-6.32096930696347,
40.0707007596512));
#27999=CARTESIAN_POINT('Ctrl Pts',(-27.4931242188518,-6.31647639530748,
40.0701968069396));
#28000=CARTESIAN_POINT('Ctrl Pts',(-27.4914999811189,-6.31199416056962,
40.0697321796178));
#28001=CARTESIAN_POINT('Ctrl Pts',(-27.4898757433861,-6.30751192583176,
40.0692675522959));
#28002=CARTESIAN_POINT('Ctrl Pts',(-27.4882099136517,-6.3030403651958,40.0688422470209));
#28003=CARTESIAN_POINT('Ctrl Pts',(-27.4865003722782,-6.29858154433863,
40.0684588731157));
#28004=CARTESIAN_POINT('Ctrl Pts',(-27.4812555102352,-6.2849019103541,40.0672826844169));
#28005=CARTESIAN_POINT('Ctrl Pts',(-27.4755856598104,-6.27129040223665,
40.0664392906386));
#28006=CARTESIAN_POINT('Ctrl Pts',(-27.4694214423627,-6.25784359490804,
40.066081345996));
#28007=CARTESIAN_POINT('Ctrl Pts',(-27.4646998272645,-6.24754372326264,
40.0658071705887));
#28008=CARTESIAN_POINT('Ctrl Pts',(-27.4596665735312,-6.23735861368961,
40.0658422436823));
#28009=CARTESIAN_POINT('Ctrl Pts',(-27.4543102127987,-6.22740455152369,
40.0662584421382));
#28010=CARTESIAN_POINT('Ctrl Pts',(-27.4527665554702,-6.22453587598482,
40.0663783869717));
#28011=CARTESIAN_POINT('Ctrl Pts',(-27.4511949994592,-6.22168470670841,
40.0665304608586));
#28012=CARTESIAN_POINT('Ctrl Pts',(-27.4495943793826,-6.21885307551209,
40.0667167522398));
#28013=CARTESIAN_POINT('Ctrl Pts',(-27.4481938368156,-6.21637539821531,
40.0668797571984));
#28014=CARTESIAN_POINT('Ctrl Pts',(-27.4467710395402,-6.21391268023894,
40.0670689603025));
#28015=CARTESIAN_POINT('Ctrl Pts',(-27.4453250889059,-6.21146633976482,
40.067285741892));
#28016=CARTESIAN_POINT('Ctrl Pts',(-27.4402642616859,-6.20290414810542,
40.0680444774551));
#28017=CARTESIAN_POINT('Ctrl Pts',(-27.4349211443523,-6.19454160457023,
40.0691416007559));
#28018=CARTESIAN_POINT('Ctrl Pts',(-27.4292461252709,-6.18644670649284,
40.0706326389343));
#28019=CARTESIAN_POINT('Ctrl Pts',(-27.4242153245159,-6.17927072720969,
40.071954417044));
#28020=CARTESIAN_POINT('Ctrl Pts',(-27.4189234410945,-6.17230552110677,
40.0735870072275));
#28021=CARTESIAN_POINT('Ctrl Pts',(-27.4133244598885,-6.16560802962263,
40.0755585967453));
#28022=CARTESIAN_POINT('Ctrl Pts',(-27.4126074833121,-6.16475038350129,
40.0758110683023));
#28023=CARTESIAN_POINT('Ctrl Pts',(-27.4118854594803,-6.16389718068686,
40.0760691435545));
#28024=CARTESIAN_POINT('Ctrl Pts',(-27.4111582810183,-6.16304859028229,
40.076332922034));
#28025=CARTESIAN_POINT('Ctrl Pts',(-27.4069748832889,-6.15816671965832,
40.0778504178759));
#28026=CARTESIAN_POINT('Ctrl Pts',(-27.4026608751707,-6.15349535409897,
40.0795623732513));
#28027=CARTESIAN_POINT('Ctrl Pts',(-27.3982171490606,-6.14908120561047,
40.0814822596477));
#28028=CARTESIAN_POINT('Ctrl Pts',(-27.3965507517694,-6.14742589992728,
40.0822022170464));
#28029=CARTESIAN_POINT('Ctrl Pts',(-27.3948661088259,-6.14580677580884,
40.0829514055659));
#28030=CARTESIAN_POINT('Ctrl Pts',(-27.3931632535548,-6.14422633871427,
40.0837304977834));
#28031=CARTESIAN_POINT('Ctrl Pts',(-27.3924182543737,-6.14353489748539,
40.0840713506286));
#28032=CARTESIAN_POINT('Ctrl Pts',(-27.3916697692507,-6.14285086162515,
40.0844179267829));
#28033=CARTESIAN_POINT('Ctrl Pts',(-27.3909177948451,-6.14217440627914,
40.0847702338091));
#28034=CARTESIAN_POINT('Ctrl Pts',(-27.3904681928918,-6.1417699568157,40.0849808765197));
#28035=CARTESIAN_POINT('Ctrl Pts',(-27.3900173479083,-6.14136823954849,
40.0851935954983));
#28036=CARTESIAN_POINT('Ctrl Pts',(-27.3895652685859,-6.14096928576893,
40.0854083644669));
#28037=CARTESIAN_POINT('Ctrl Pts',(-27.3885996268668,-6.14011712024289,
40.08586711112));
#28038=CARTESIAN_POINT('Ctrl Pts',(-27.3876280770951,-6.13927790427025,
40.0863355648906));
#28039=CARTESIAN_POINT('Ctrl Pts',(-27.3866507863317,-6.13845171955947,
40.0868133190215));
#28040=CARTESIAN_POINT('Ctrl Pts',(-27.3794850171849,-6.13239390224247,
40.0903163458986));
#28041=CARTESIAN_POINT('Ctrl Pts',(-27.3720142576261,-6.12704603863401,
40.09433138839));
#28042=CARTESIAN_POINT('Ctrl Pts',(-27.3642632539306,-6.12254522320978,
40.0989235304305));
#28043=CARTESIAN_POINT('Ctrl Pts',(-27.3611502082718,-6.12073755487833,
40.1007678783891));
#28044=CARTESIAN_POINT('Ctrl Pts',(-27.3579921867464,-6.1190670360301,40.1027052304882));
#28045=CARTESIAN_POINT('Ctrl Pts',(-27.3547919380345,-6.11754464002831,
40.1047394416188));
#28046=CARTESIAN_POINT('Ctrl Pts',(-27.3534952922802,-6.11692781037227,
40.105563643568));
#28047=CARTESIAN_POINT('Ctrl Pts',(-27.3521978688196,-6.11633884284223,
40.1064006970497));
#28048=CARTESIAN_POINT('Ctrl Pts',(-27.3509000135422,-6.11577753018269,
40.1072500513475));
#28049=CARTESIAN_POINT('Ctrl Pts',(-27.3496832742196,-6.11525129956437,
40.1080463210017));
#28050=CARTESIAN_POINT('Ctrl Pts',(-27.3484661554654,-6.1147493750158,40.1088534018512));
#28051=CARTESIAN_POINT('Ctrl Pts',(-27.3472489508901,-6.11427158462743,
40.109670838332));
#28052=CARTESIAN_POINT('Ctrl Pts',(-27.3388812462172,-6.11098700211233,
40.1152903267884));
#28053=CARTESIAN_POINT('Ctrl Pts',(-27.3305072396875,-6.10884307366972,
40.1213990974306));
#28054=CARTESIAN_POINT('Ctrl Pts',(-27.322235046933,-6.10778191357492,40.1278491871424));
#28055=CARTESIAN_POINT('Ctrl Pts',(-27.3214824073746,-6.10768536468047,
40.1284360439549));
#28056=CARTESIAN_POINT('Ctrl Pts',(-27.3207305910292,-6.10759774950087,
40.12902573023));
#28057=CARTESIAN_POINT('Ctrl Pts',(-27.319979666939,-6.10751900703753,40.1296181367441));
#28058=CARTESIAN_POINT('Ctrl Pts',(-27.3122365353699,-6.10670705645327,
40.1357267190111));
#28059=CARTESIAN_POINT('Ctrl Pts',(-27.3045906547513,-6.1068415622247,40.1421229193531));
#28060=CARTESIAN_POINT('Ctrl Pts',(-27.2971463985059,-6.10786410630554,
40.1486937142711));
#28061=CARTESIAN_POINT('Ctrl Pts',(-27.2959339458739,-6.10803064896894,
40.1497639054803));
#28062=CARTESIAN_POINT('Ctrl Pts',(-27.2947268094371,-6.10822064294905,
40.1508387079977));
#28063=CARTESIAN_POINT('Ctrl Pts',(-27.2935253998823,-6.10843371318469,
40.1519176123711));
#28064=CARTESIAN_POINT('Origin',(-27.8490907775129,-12.8919045823054,40.036547827824));
#28065=CARTESIAN_POINT('Origin',(-27.8490907775129,-12.8919045823054,40.036547827824));
#28066=CARTESIAN_POINT('Origin',(-14.7107907121785,-13.5169045823054,-4.79600242588633));
#28067=CARTESIAN_POINT('Origin',(-31.3912427907138,-13.5169045823054,45.7890602015826));
#28068=CARTESIAN_POINT('Ctrl Pts',(-31.9675858640834,-14.6836564585996,
47.3436397133837));
#28069=CARTESIAN_POINT('Ctrl Pts',(-32.1960990859602,-14.7195047625521,
47.2319833969137));
#28070=CARTESIAN_POINT('Ctrl Pts',(-32.140341712633,-14.9046273277204,47.0628938417614));
#28071=CARTESIAN_POINT('Ctrl Pts',(-31.8173108281339,-14.2208393515118,
46.8863441102177));
#28072=CARTESIAN_POINT('Ctrl Pts',(-32.0453894454383,-14.2572370951476,
46.7749420308703));
#28073=CARTESIAN_POINT('Ctrl Pts',(-31.9896429860821,-14.4418102212184,
46.6058855733665));
#28074=CARTESIAN_POINT('Ctrl Pts',(-31.6669720145896,-13.7582547217136,
46.4288175299242));
#28075=CARTESIAN_POINT('Ctrl Pts',(-31.8945090807232,-13.7949155819404,
46.3173829274235));
#28076=CARTESIAN_POINT('Ctrl Pts',(-31.8388709365124,-13.9792255914427,
46.1486549459201));
#28077=CARTESIAN_POINT('Ctrl Pts',(-31.5165682646526,-13.2959337131846,
45.9710537470232));
#28078=CARTESIAN_POINT('Ctrl Pts',(-31.7434417477461,-13.3325299785125,
45.8592568248438));
#28079=CARTESIAN_POINT('Ctrl Pts',(-31.6880237676519,-13.5169045823054,
45.6911965120564));
#28080=CARTESIAN_POINT('Origin',(-31.3912427907138,-13.5169045823054,45.7890602015826));
#28081=CARTESIAN_POINT('Ctrl Pts',(-27.4498900633667,-6.28105857414855,
39.8238138910649));
#28082=CARTESIAN_POINT('Ctrl Pts',(-27.5054686557226,-6.09633085020216,
39.9923612758618));
#28083=CARTESIAN_POINT('Ctrl Pts',(-27.2778197979418,-6.06008770502775,
40.1040929402346));
#28084=CARTESIAN_POINT('Ctrl Pts',(-28.1663303157565,-8.47898077425032,
41.9964873213379));
#28085=CARTESIAN_POINT('Ctrl Pts',(-28.2252224962987,-8.30110493968633,
42.1750834784584));
#28086=CARTESIAN_POINT('Ctrl Pts',(-27.9918605627639,-8.25800948639314,
42.2784063052523));
#28087=CARTESIAN_POINT('Ctrl Pts',(-28.8808461149493,-10.6833293750548,
44.1633246636541));
#28088=CARTESIAN_POINT('Ctrl Pts',(-28.9397014588684,-10.5025148294221,
44.3418091102154));
#28089=CARTESIAN_POINT('Ctrl Pts',(-28.7042756097382,-10.4623581523752,
44.4466133273737));
#28090=CARTESIAN_POINT('Ctrl Pts',(-29.5940549924842,-12.8919045823054,
46.326198641332));
#28091=CARTESIAN_POINT('Ctrl Pts',(-29.651286959495,-12.7034528674627,46.49976004254));
#28092=CARTESIAN_POINT('Ctrl Pts',(-29.4155943178386,-12.6709337131846,
46.6106860996161));
#28093=CARTESIAN_POINT('Origin',(-29.2972740155461,-12.8919045823054,46.4240623308582));
#28094=CARTESIAN_POINT('Origin',(-13.2268858274881,-12.8919045823054,-4.30668397825546));
#28095=CARTESIAN_POINT('Ctrl Pts',(-30.04271957779,-13.2044045823055,46.6889364873753));
#28096=CARTESIAN_POINT('Ctrl Pts',(-30.0368201694537,-13.2044045823055,
46.695006276046));
#28097=CARTESIAN_POINT('Ctrl Pts',(-30.0305178990863,-13.20411637619,46.7007234861797));
#28098=CARTESIAN_POINT('Ctrl Pts',(-30.0238719237597,-13.2035045918484,
46.705933998298));
#28099=CARTESIAN_POINT('Ctrl Pts',(-30.0222118579831,-13.2033517772203,
46.707235506718));
#28100=CARTESIAN_POINT('Ctrl Pts',(-30.0205305478229,-13.2031788924169,
46.7085055118816));
#28101=CARTESIAN_POINT('Ctrl Pts',(-30.0188292749668,-13.2029856357525,
46.7097419077627));
#28102=CARTESIAN_POINT('Ctrl Pts',(-30.0145102056262,-13.2024950096128,
46.7128807808267));
#28103=CARTESIAN_POINT('Ctrl Pts',(-30.0100623794942,-13.2018727723585,
46.7158023935072));
#28104=CARTESIAN_POINT('Ctrl Pts',(-30.0055133346289,-13.2011172816476,
46.7184855719865));
#28105=CARTESIAN_POINT('Ctrl Pts',(-29.998689767331,-13.1999840455812,46.7225103397054));
#28106=CARTESIAN_POINT('Ctrl Pts',(-29.9916496764111,-13.1985506728398,
46.726024129218));
#28107=CARTESIAN_POINT('Ctrl Pts',(-29.9844563032259,-13.1968266777137,
46.7289158118595));
#28108=CARTESIAN_POINT('Ctrl Pts',(-29.9808596166333,-13.1959646801506,
46.7303616531803));
#28109=CARTESIAN_POINT('Ctrl Pts',(-29.9772246319322,-13.195030319004,46.731651963405));
#28110=CARTESIAN_POINT('Ctrl Pts',(-29.9735596330734,-13.1940263590679,
46.7327754786219));
#28111=CARTESIAN_POINT('Ctrl Pts',(-29.971727133644,-13.1935243790998,46.7333372362304));
#28112=CARTESIAN_POINT('Ctrl Pts',(-29.9698871192629,-13.1930050138329,
46.7338572987164));
#28113=CARTESIAN_POINT('Ctrl Pts',(-29.9680405503598,-13.1924686892783,
46.7343342824294));
#28114=CARTESIAN_POINT('Ctrl Pts',(-29.9675789081341,-13.1923346081396,
46.7344535283577));
#28115=CARTESIAN_POINT('Ctrl Pts',(-29.9671168559859,-13.1921994672886,
46.7345700819503));
#28116=CARTESIAN_POINT('Ctrl Pts',(-29.9666544083826,-13.1920632738588,
46.7346839217674));
#28117=CARTESIAN_POINT('Ctrl Pts',(-29.9652670655729,-13.1916546935696,
46.7350254412186));
#28118=CARTESIAN_POINT('Ctrl Pts',(-29.9638761650542,-13.1912366390105,
46.7353425362126));
#28119=CARTESIAN_POINT('Ctrl Pts',(-29.9624820851714,-13.1908093125307,
46.7356346320705));
#28120=CARTESIAN_POINT('Ctrl Pts',(-29.954042205835,-13.188222241323,46.7374030054799));
#28121=CARTESIAN_POINT('Ctrl Pts',(-29.9455363271605,-13.1853020171008,
46.738319884669));
#28122=CARTESIAN_POINT('Ctrl Pts',(-29.9370870977222,-13.1821047274604,
46.7384633004647));
#28123=CARTESIAN_POINT('Ctrl Pts',(-29.9307220034064,-13.1796960995182,
46.7385713405022));
#28124=CARTESIAN_POINT('Ctrl Pts',(-29.924388757318,-13.1771305701858,46.7382414915082));
#28125=CARTESIAN_POINT('Ctrl Pts',(-29.9181337478532,-13.1744346626403,
46.7375255006745));
#28126=CARTESIAN_POINT('Ctrl Pts',(-29.917223866056,-13.1740425038088,46.737421349429));
#28127=CARTESIAN_POINT('Ctrl Pts',(-29.9163156537632,-13.1736476854837,
46.7373084624657));
#28128=CARTESIAN_POINT('Ctrl Pts',(-29.9154092836977,-13.1732503241607,
46.7371869720081));
#28129=CARTESIAN_POINT('Ctrl Pts',(-29.9147043463233,-13.17294127286,46.7370924817249));
#28130=CARTESIAN_POINT('Ctrl Pts',(-29.9140001157073,-13.1726304994968,
46.7369927667443));
#28131=CARTESIAN_POINT('Ctrl Pts',(-29.9132966638191,-13.1723180491455,
46.7368878708566));
#28132=CARTESIAN_POINT('Ctrl Pts',(-29.9033263548421,-13.1678895635671,
46.7354011388876));
#28133=CARTESIAN_POINT('Ctrl Pts',(-29.8936167820225,-13.1631872663844,
46.7329350902098));
#28134=CARTESIAN_POINT('Ctrl Pts',(-29.8843259095194,-13.1583829057193,
46.7297748595837));
#28135=CARTESIAN_POINT('Ctrl Pts',(-29.8816299246712,-13.1569887973022,
46.7288578376483));
#28136=CARTESIAN_POINT('Ctrl Pts',(-29.8789690772141,-13.1555861806432,
46.7278826869499));
#28137=CARTESIAN_POINT('Ctrl Pts',(-29.8763469083833,-13.1541794056116,
46.7268570368218));
#28138=CARTESIAN_POINT('Ctrl Pts',(-29.867948476878,-13.1496737065098,46.723572026243));
#28139=CARTESIAN_POINT('Ctrl Pts',(-29.8598547091022,-13.1450668045687,
46.7197885306234));
#28140=CARTESIAN_POINT('Ctrl Pts',(-29.8520287057686,-13.1404003938699,
46.7155889038217));
#28141=CARTESIAN_POINT('Ctrl Pts',(-29.8476327076698,-13.137779192257,46.7132299025986));
#28142=CARTESIAN_POINT('Ctrl Pts',(-29.843321315133,-13.1351390520035,46.7107385600487));
#28143=CARTESIAN_POINT('Ctrl Pts',(-29.8390887268153,-13.1324866446614,
46.7081225206955));
#28144=CARTESIAN_POINT('Ctrl Pts',(-29.8346758466811,-13.1297212550724,
46.7053950482306));
#28145=CARTESIAN_POINT('Ctrl Pts',(-29.8303485053492,-13.1269417023507,
46.7025350007665));
#28146=CARTESIAN_POINT('Ctrl Pts',(-29.8261007325175,-13.1241525253868,
46.6995556323488));
#28147=CARTESIAN_POINT('Ctrl Pts',(-29.8242423319037,-13.122932260465,46.6982521586661));
#28148=CARTESIAN_POINT('Ctrl Pts',(-29.8223991720806,-13.1217101337094,
46.6969258426594));
#28149=CARTESIAN_POINT('Ctrl Pts',(-29.82057080665,-13.1204864412399,46.6955777768191));
#28150=CARTESIAN_POINT('Ctrl Pts',(-29.8188567140589,-13.1193392295498,
46.6943139650937));
#28151=CARTESIAN_POINT('Ctrl Pts',(-29.8171556245902,-13.1181906410734,
46.6930310372273));
#28152=CARTESIAN_POINT('Ctrl Pts',(-29.8154671982959,-13.117040885084,46.6917298843572));
#28153=CARTESIAN_POINT('Ctrl Pts',(-29.8051941573223,-13.1100453233422,
46.6838131652248));
#28154=CARTESIAN_POINT('Ctrl Pts',(-29.7953494354289,-13.1029809016301,
46.675192533093));
#28155=CARTESIAN_POINT('Ctrl Pts',(-29.7859484771511,-13.0959259298128,
46.6661148193062));
#28156=CARTESIAN_POINT('Ctrl Pts',(-29.7839183747256,-13.0944024345504,
46.6641545203418));
#28157=CARTESIAN_POINT('Ctrl Pts',(-29.7819089162172,-13.0928792536023,
46.6621727676645));
#28158=CARTESIAN_POINT('Ctrl Pts',(-29.7799201851399,-13.0913569710302,
46.6601718236165));
#28159=CARTESIAN_POINT('Ctrl Pts',(-29.7690104052807,-13.0830060341259,
46.6491950458494));
#28160=CARTESIAN_POINT('Ctrl Pts',(-29.7586608103041,-13.0746647314083,
46.6376540788201));
#28161=CARTESIAN_POINT('Ctrl Pts',(-29.7488108236965,-13.0663267356308,
46.6257713981828));
#28162=CARTESIAN_POINT('Ctrl Pts',(-29.748272514602,-13.0658710579598,46.6251220008477));
#28163=CARTESIAN_POINT('Ctrl Pts',(-29.7477357007175,-13.0654153808115,
46.6244715746663));
#28164=CARTESIAN_POINT('Ctrl Pts',(-29.7472003732994,-13.0649596999837,
46.6238201531363));
#28165=CARTESIAN_POINT('Ctrl Pts',(-29.7404781089958,-13.0592375814082,
46.6156400608235));
#28166=CARTESIAN_POINT('Ctrl Pts',(-29.7339925628948,-13.053534176996,46.6072713024434));
#28167=CARTESIAN_POINT('Ctrl Pts',(-29.7277161004611,-13.0478477661443,
46.598737203163));
#28168=CARTESIAN_POINT('Ctrl Pts',(-29.7170149824623,-13.0381526625477,
46.5841869044274));
#28169=CARTESIAN_POINT('Ctrl Pts',(-29.7069273852876,-13.0285130912561,
46.5691662228752));
#28170=CARTESIAN_POINT('Ctrl Pts',(-29.6973719426179,-13.0189444021978,
46.553797195801));
#28171=CARTESIAN_POINT('Ctrl Pts',(-29.6871702002742,-13.0087285175221,
46.5373886567408));
#28172=CARTESIAN_POINT('Ctrl Pts',(-29.6775748886097,-12.9985931561289,
46.5205824904044));
#28173=CARTESIAN_POINT('Ctrl Pts',(-29.6685050610264,-12.9885428112971,
46.503472020218));
#28174=CARTESIAN_POINT('Ctrl Pts',(-29.6583357622502,-12.9772741340857,
46.4842873684781));
#28175=CARTESIAN_POINT('Ctrl Pts',(-29.6488266209448,-12.9661119592019,
46.464719631505));
#28176=CARTESIAN_POINT('Ctrl Pts',(-29.6398905793283,-12.9550504724707,
46.4448415317008));
#28177=CARTESIAN_POINT('Ctrl Pts',(-29.6298393434875,-12.9426085416186,
46.4224826979162));
#28178=CARTESIAN_POINT('Ctrl Pts',(-29.6205123618971,-12.9302931192882,
46.3997297163687));
#28179=CARTESIAN_POINT('Ctrl Pts',(-29.6118286232292,-12.9180916100454,
46.376631896441));
#28180=CARTESIAN_POINT('Ctrl Pts',(-29.6055746337663,-12.9093041380643,
46.3599969505993));
#28181=CARTESIAN_POINT('Ctrl Pts',(-29.5996552034974,-12.9005755951523,
46.3431818156186));
#28182=CARTESIAN_POINT('Ctrl Pts',(-29.5940549924842,-12.8919045823054,
46.326198641332));
#28183=CARTESIAN_POINT('Origin',(-31.3912427907138,-13.5169045823054,45.7890602015826));
#28184=CARTESIAN_POINT('Origin',(-31.3912427907138,-13.5169045823054,45.7890602015826));
#28185=CARTESIAN_POINT('Ctrl Pts',(-30.1626755346769,-13.2959337131847,
46.8745131384049));
#28186=CARTESIAN_POINT('Ctrl Pts',(-30.1129881504469,-13.2044045823055,
46.7976447726886));
#28187=CARTESIAN_POINT('Ctrl Pts',(-30.04271957779,-13.2044045823055,46.6889364873753));
#28188=CARTESIAN_POINT('Ctrl Pts',(-30.08095390153,-13.2959337183951,46.927337660237));
#28189=CARTESIAN_POINT('Ctrl Pts',(-30.0567289927829,-13.209279823895,46.8398155271884));
#28190=CARTESIAN_POINT('Ctrl Pts',(-30.0057259985099,-13.2044045823055,
46.7269984752225));
#28191=CARTESIAN_POINT('Ctrl Pts',(-29.9887271578055,-13.2734166054794,
46.9598087435376));
#28192=CARTESIAN_POINT('Ctrl Pts',(-29.9896831552566,-13.193172351531,46.8638177887699));
#28193=CARTESIAN_POINT('Ctrl Pts',(-29.9601903592735,-13.1931460297457,
46.7438847747009));
#28194=CARTESIAN_POINT('Ctrl Pts',(-29.8139966334862,-13.1901047283844,
46.9726654864714));
#28195=CARTESIAN_POINT('Ctrl Pts',(-29.866204852841,-13.1260474868727,46.8633668402251));
#28196=CARTESIAN_POINT('Ctrl Pts',(-29.8664029441127,-13.1514900886124,
46.7298907631929));
#28197=CARTESIAN_POINT('Ctrl Pts',(-29.7351139893344,-13.1321577745916,
46.9541554619723));
#28198=CARTESIAN_POINT('Ctrl Pts',(-29.8115047075592,-13.0767072102091,
46.83982187418));
#28199=CARTESIAN_POINT('Ctrl Pts',(-29.8204272993462,-13.1225166214137,
46.700471501026));
#28200=CARTESIAN_POINT('Ctrl Pts',(-29.5397638152463,-12.9456232578403,
46.8572594916692));
#28201=CARTESIAN_POINT('Ctrl Pts',(-29.6836831453199,-12.917759331099,46.7330734174298));
#28202=CARTESIAN_POINT('Ctrl Pts',(-29.6989366770835,-13.0292493378237,
46.5791043383549));
#28203=CARTESIAN_POINT('Ctrl Pts',(-29.4578462161212,-12.8021218234312,
46.739230783511));
#28204=CARTESIAN_POINT('Ctrl Pts',(-29.649013231966,-12.7965826300655,46.6116445270736));
#28205=CARTESIAN_POINT('Ctrl Pts',(-29.6364065710858,-12.9574790903514,
46.4546338447575));
#28206=CARTESIAN_POINT('Ctrl Pts',(-29.4155943178386,-12.6709337131846,
46.6106860996161));
#28207=CARTESIAN_POINT('Ctrl Pts',(-29.6512869594949,-12.7034528674627,
46.49976004254));
#28208=CARTESIAN_POINT('Ctrl Pts',(-29.5940549924842,-12.8919045823054,
46.326198641332));
#28209=CARTESIAN_POINT('Origin',(-30.0427195777899,-13.5169045823054,46.6889364873753));
#28210=CARTESIAN_POINT('Origin',(0.0835265683620477,-13.5169045823054,0.0824317919394229));
#28211=CARTESIAN_POINT('Origin',(34.8549570309562,12.3739193162059,-36.4567656030545));
#28212=CARTESIAN_POINT('Origin',(34.5439318808757,11.9341984494201,-36.1457404735404));
#28213=CARTESIAN_POINT('Origin',(35.1659821576994,12.8136401876617,-36.7677907503641));
#28214=CARTESIAN_POINT('Origin',(34.5439318808757,11.9341984494201,-36.1457404735404));
#28215=CARTESIAN_POINT('Origin',(34.5439318808757,11.9341984494201,-36.1457404735404));
#28216=CARTESIAN_POINT('Origin',(35.1659821576994,12.8136401876617,-36.7677907503641));
#28217=CARTESIAN_POINT('Origin',(35.1659821576994,12.8136401876617,-36.7677907503641));
#28218=CARTESIAN_POINT('Origin',(35.1659821576994,12.8136401876617,-36.7677907503641));
#28219=CARTESIAN_POINT('Origin',(0.0835265683620477,11.9341984494201,0.0824317919394229));
#28220=CARTESIAN_POINT('Origin',(-34.3768787441515,11.9341984494201,-36.1457404735405));
#28221=CARTESIAN_POINT('Origin',(0.0835265683620477,12.8136401876617,0.0824317919394229));
#28222=CARTESIAN_POINT('Ctrl Pts',(11.0320394968432,13.1261401876617,-49.6050682080606));
#28223=CARTESIAN_POINT('Ctrl Pts',(10.6578693364404,13.1261401876617,-49.6453148766512));
#28224=CARTESIAN_POINT('Ctrl Pts',(10.2836734751494,13.1182694471953,-49.6836022760034));
#28225=CARTESIAN_POINT('Ctrl Pts',(9.90942930877251,13.1033923474057,-49.7199013138211));
#28226=CARTESIAN_POINT('Ctrl Pts',(9.90937195321906,13.1033900673854,-49.7199068769042));
#28227=CARTESIAN_POINT('Ctrl Pts',(9.90931459767862,13.1033877872104,-49.7199124399391));
#28228=CARTESIAN_POINT('Ctrl Pts',(9.90925724215118,13.1033855068806,-49.7199180029256));
#28229=CARTESIAN_POINT('Ctrl Pts',(9.69153210444253,13.0947292335987,-49.7410354449037));
#28230=CARTESIAN_POINT('Ctrl Pts',(9.47385022844805,13.0838402503218,-49.7614722083415));
#28231=CARTESIAN_POINT('Ctrl Pts',(9.25629353024675,13.069869045462,-49.7812208487346));
#28232=CARTESIAN_POINT('Ctrl Pts',(9.09983844834887,13.0598217059932,-49.7954230092547));
#28233=CARTESIAN_POINT('Ctrl Pts',(8.94344804305751,13.0481798478176,-49.8092691162915));
#28234=CARTESIAN_POINT('Ctrl Pts',(8.78715657141638,13.0346110567867,-49.8227532649998));
#28235=CARTESIAN_POINT('Origin',(24.5746430918789,12.8136401876617,-26.1764516845437));
#28236=CARTESIAN_POINT('Origin',(38.9743995336223,12.8136401876617,-40.5762081262869));
#28237=CARTESIAN_POINT('Origin',(34.5439318808757,-3.61941807409668,-36.1457404735404));
#28238=CARTESIAN_POINT('Origin',(34.5439318808757,-3.61941807409668,-36.1457404735404));
#28239=CARTESIAN_POINT('Origin',(34.5439318808757,-3.61941807409669,-36.1457404735404));
#28240=CARTESIAN_POINT('Origin',(-34.3768787441515,11.9341984494201,-36.1457404735405));
#28241=CARTESIAN_POINT('Origin',(-34.3768787441515,11.9341984494202,-36.1457404735405));
#28242=CARTESIAN_POINT('Ctrl Pts',(11.0320394968433,13.1261401876617,-49.6050682080606));
#28243=CARTESIAN_POINT('Ctrl Pts',(11.0320394968433,13.1261401876617,-49.9175682080606));
#28244=CARTESIAN_POINT('Ctrl Pts',(11.0320394968433,13.4386401876617,-49.9175682080606));
#28245=CARTESIAN_POINT('Ctrl Pts',(10.6584907317851,13.1261401876617,-49.6452480378299));
#28246=CARTESIAN_POINT('Ctrl Pts',(10.6809373469102,13.1639055963026,-49.9175682080606));
#28247=CARTESIAN_POINT('Ctrl Pts',(10.6496370560559,13.4386401851022,-49.9175682080606));
#28248=CARTESIAN_POINT('Ctrl Pts',(10.2842597524009,13.1182927286047,-49.6835453366231));
#28249=CARTESIAN_POINT('Ctrl Pts',(10.2980626523239,13.1821712224823,-49.9175682080606));
#28250=CARTESIAN_POINT('Ctrl Pts',(10.2678955540983,13.4229452699559,-49.9175682080606));
#28251=CARTESIAN_POINT('Ctrl Pts',(9.5345988672954,13.0884919386943,-49.7562572211741));
#28252=CARTESIAN_POINT('Ctrl Pts',(9.54083079601551,13.1804128114024,-49.9175682080606));
#28253=CARTESIAN_POINT('Ctrl Pts',(9.50565038581019,13.3633436893187,-49.9175682080606));
#28254=CARTESIAN_POINT('Ctrl Pts',(9.15977276126021,13.0669605544565,-49.7906055560521));
#28255=CARTESIAN_POINT('Ctrl Pts',(9.1588613746445,13.1642472289417,-49.9175682080606));
#28256=CARTESIAN_POINT('Ctrl Pts',(9.12568496896286,13.3202672259815,-49.9175682080606));
#28257=CARTESIAN_POINT('Ctrl Pts',(8.78715657141589,13.0346110567867,-49.8227532649998));
#28258=CARTESIAN_POINT('Ctrl Pts',(8.77156878298277,13.125337974864,-49.9175682080606));
#28259=CARTESIAN_POINT('Ctrl Pts',(8.74919157457976,13.2555819259088,-49.9175682080606));
#28260=CARTESIAN_POINT('Origin',(11.0320394968432,13.4386401876617,-49.6050682080606));
#28261=CARTESIAN_POINT('Origin',(8.7491915745805,13.2555819259033,-49.6050682080606));
#28262=CARTESIAN_POINT('Origin',(39.8582830101055,12.8136401876617,-39.6923246498037));
#28263=CARTESIAN_POINT('Origin',(40.7421664865887,12.8136401876617,-38.8084411733206));
#28264=CARTESIAN_POINT('Ctrl Pts',(38.0393490816115,-8.24885981233825,-39.1992159360345));
#28265=CARTESIAN_POINT('Ctrl Pts',(37.8856271521298,-8.46631238203733,-39.0454940065529));
#28266=CARTESIAN_POINT('Ctrl Pts',(37.6657443451358,-8.46983068145904,-39.2604024894786));
#28267=CARTESIAN_POINT('Ctrl Pts',(36.9478802019249,-6.70569384849427,-38.1077470563479));
#28268=CARTESIAN_POINT('Ctrl Pts',(36.7944751038544,-6.92339564386804,-37.954341958285));
#28269=CARTESIAN_POINT('Ctrl Pts',(36.5743787698635,-6.92666471828378,-38.1688349292337));
#28270=CARTESIAN_POINT('Ctrl Pts',(35.8563993091448,-5.16254485803399,-37.0162661635679));
#28271=CARTESIAN_POINT('Ctrl Pts',(35.7031187964695,-5.38020745679319,-36.8629856508092));
#28272=CARTESIAN_POINT('Ctrl Pts',(35.483009954652,-5.38351572788346,-37.0772471608648));
#28273=CARTESIAN_POINT('Ctrl Pts',(34.7649027499965,-3.61941807409668,-35.9247696044196));
#28274=CARTESIAN_POINT('Ctrl Pts',(34.6114148933597,-3.83655054711529,-35.7712817477828));
#28275=CARTESIAN_POINT('Ctrl Pts',(34.3916369666325,-3.84038894321747,-35.9856330592972));
#28276=CARTESIAN_POINT('Origin',(37.8183782124907,-8.24885981233827,-39.4201868051553));
#28277=CARTESIAN_POINT('Origin',(0.0835265683620477,-3.61941807409668,0.0824317919394229));
#28278=CARTESIAN_POINT('Origin',(-34.3768787441515,-3.61941807409668,-36.1457404735405));
#28279=CARTESIAN_POINT('Origin',(-34.6879044362409,12.3739187291536,-36.4567658910079));
#28280=CARTESIAN_POINT('Origin',(-34.9989290209752,12.8136401876617,-36.7677907503642));
#28281=CARTESIAN_POINT('Origin',(0.0835265683620477,12.8136401876617,0.0824317919394229));
#28282=CARTESIAN_POINT('Ctrl Pts',(-8.62010343469281,13.0346110567825,-49.8227532650011));
#28283=CARTESIAN_POINT('Ctrl Pts',(-8.88131178011465,13.0572884390954,-49.8002173445413));
#28284=CARTESIAN_POINT('Ctrl Pts',(-9.14274668539152,13.0745923805386,-49.7766769038922));
#28285=CARTESIAN_POINT('Ctrl Pts',(-9.40431840153695,13.0880420718507,-49.7521473008839));
#28286=CARTESIAN_POINT('Ctrl Pts',(-9.51689874960235,13.0938308128951,-49.7415897708677));
#28287=CARTESIAN_POINT('Ctrl Pts',(-9.62950455408787,13.0989048482899,-49.7308488985899));
#28288=CARTESIAN_POINT('Ctrl Pts',(-9.74212903364439,13.1033825850677,-49.7199254399034));
#28289=CARTESIAN_POINT('Ctrl Pts',(-9.74242935783179,13.1033945253906,-49.7198963114327));
#28290=CARTESIAN_POINT('Ctrl Pts',(-9.7427296825782,13.1034064614895,-49.7198671816217));
#28291=CARTESIAN_POINT('Ctrl Pts',(-9.74303000788388,13.1034183933665,-49.7198380504703));
#28292=CARTESIAN_POINT('Ctrl Pts',(-9.98721127321016,13.1131196764878,-49.6961527956236));
#28293=CARTESIAN_POINT('Ctrl Pts',(-10.2314035286019,13.1198333629236,-49.6716164060401));
#28294=CARTESIAN_POINT('Ctrl Pts',(-10.4755740809779,13.1233309724858,-49.6462439593173));
#28295=CARTESIAN_POINT('Ctrl Pts',(-10.6053869203596,13.1251904703815,-49.6327547431972));
#28296=CARTESIAN_POINT('Ctrl Pts',(-10.7351934140452,13.1261401876617,-49.6190290586065));
#28297=CARTESIAN_POINT('Ctrl Pts',(-10.8649863601192,13.1261401876617,-49.6050682080606));
#28298=CARTESIAN_POINT('Origin',(-34.9989290209752,12.8136401876617,-36.7677907503642));
#28299=CARTESIAN_POINT('Ctrl Pts',(8.78715657141686,13.0346110567825,-49.8227532650012));
#28300=CARTESIAN_POINT('Ctrl Pts',(8.77156878298359,13.1253379748597,-49.9175682080606));
#28301=CARTESIAN_POINT('Ctrl Pts',(8.7491915745805,13.2555819259033,-49.9175682080606));
#28302=CARTESIAN_POINT('Ctrl Pts',(5.9167136340953,12.5435283274364,-49.8248727468205));
#28303=CARTESIAN_POINT('Ctrl Pts',(5.91175753908113,12.6357570952065,-49.9175682080606));
#28304=CARTESIAN_POINT('Ctrl Pts',(5.89089499049724,12.7644980954123,-49.9175682080606));
#28305=CARTESIAN_POINT('Ctrl Pts',(3.02011116462985,12.2852858973025,-49.8260360759873));
#28306=CARTESIAN_POINT('Ctrl Pts',(3.01473384245429,12.3768143018313,-49.9175682080606));
#28307=CARTESIAN_POINT('Ctrl Pts',(3.00710937180082,12.5062567663872,-49.9175682080606));
#28308=CARTESIAN_POINT('Ctrl Pts',(-1.36745139963336,12.2842756298963,-49.8260405689135));
#28309=CARTESIAN_POINT('Ctrl Pts',(-1.36478834461974,12.3758051232163,-49.9175682080606));
#28310=CARTESIAN_POINT('Ctrl Pts',(-1.36102716280008,12.5052464990352,-49.9175682080606));
#28311=CARTESIAN_POINT('Ctrl Pts',(-2.84134992071046,12.3489547591764,-49.8257518757999));
#28312=CARTESIAN_POINT('Ctrl Pts',(-2.83674726276666,12.4404805872018,-49.9175682080606));
#28313=CARTESIAN_POINT('Ctrl Pts',(-2.82840051213665,12.5699256283378,-49.9175682080606));
#28314=CARTESIAN_POINT('Ctrl Pts',(-5.75032001544249,12.6021248598315,-49.8246345776219));
#28315=CARTESIAN_POINT('Ctrl Pts',(-5.74047966090505,12.6933787936176,-49.9175682080606));
#28316=CARTESIAN_POINT('Ctrl Pts',(-5.72463777045536,12.8230957289117,-49.9175682080606));
#28317=CARTESIAN_POINT('Ctrl Pts',(-7.19139408987476,12.7901838029064,-49.8238081974504));
#28318=CARTESIAN_POINT('Ctrl Pts',(-7.17966289645425,12.8814125534473,-49.9175682080606));
#28319=CARTESIAN_POINT('Ctrl Pts',(-7.15947736247938,13.0111545790442,-49.9175682080606));
#28320=CARTESIAN_POINT('Ctrl Pts',(-8.62010343469281,13.0346110567825,-49.8227532650012));
#28321=CARTESIAN_POINT('Ctrl Pts',(-8.60451564625954,13.1253379748597,-49.9175682080606));
#28322=CARTESIAN_POINT('Ctrl Pts',(-8.58213843785645,13.2555819259033,-49.9175682080606));
#28323=CARTESIAN_POINT('Origin',(-8.58213843785645,13.2555819259033,-49.6050682080606));
#28324=CARTESIAN_POINT('Origin',(0.0835265683620477,13.4386401876617,-49.6050682080606));
#28325=CARTESIAN_POINT('Origin',(44.4585265683622,13.4386401876617,-49.6050682080606));
#28326=CARTESIAN_POINT('Origin',(26.3424100448454,12.8136401876617,-24.4086847315773));
#28327=CARTESIAN_POINT('Origin',(36.9337491106658,12.8136401876617,-35.0000237973977));
#28328=CARTESIAN_POINT('Origin',(37.8183782124907,-8.24885981233827,-39.4201868051553));
#28329=CARTESIAN_POINT('Origin',(37.8183782124907,-8.24885981233827,-39.4201868051553));
#28330=CARTESIAN_POINT('Origin',(37.8183782124907,-8.24885981233827,-39.4201868051553));
#28331=CARTESIAN_POINT('Origin',(-34.3768787441515,-3.61941807409668,-36.1457404735405));
#28332=CARTESIAN_POINT('Origin',(-34.3768787441515,-3.61941807409668,-36.1457404735405));
#28333=CARTESIAN_POINT('Origin',(-34.9989290209752,12.8136401876617,-36.7677907503642));
#28334=CARTESIAN_POINT('Origin',(-34.9989290209752,12.8136401876617,-36.7677907503642));
#28335=CARTESIAN_POINT('Ctrl Pts',(-8.6201034346928,13.0346110567825,-49.8227532650011));
#28336=CARTESIAN_POINT('Ctrl Pts',(-8.60451564625953,13.1253379748597,-49.9175682080606));
#28337=CARTESIAN_POINT('Ctrl Pts',(-8.58213843785645,13.2555819259033,-49.9175682080606));
#28338=CARTESIAN_POINT('Ctrl Pts',(-8.99338683221866,13.0670184804062,-49.7905479931254));
#28339=CARTESIAN_POINT('Ctrl Pts',(-8.99252376979541,13.1643191174805,-49.9175682080606));
#28340=CARTESIAN_POINT('Ctrl Pts',(-8.95930452222033,13.3203828042395,-49.9175682080606));
#28341=CARTESIAN_POINT('Ctrl Pts',(-9.36803051056639,13.0885197051924,-49.756212524541));
#28342=CARTESIAN_POINT('Ctrl Pts',(-9.37428367693385,13.1804336598308,-49.9175682080606));
#28343=CARTESIAN_POINT('Ctrl Pts',(-9.33908873922842,13.3633992223637,-49.9175682080606));
#28344=CARTESIAN_POINT('Ctrl Pts',(-10.1180295169891,13.1183169307001,-49.6834631932219));
#28345=CARTESIAN_POINT('Ctrl Pts',(-10.1318579424303,13.1821517325912,-49.9175682080606));
#28346=CARTESIAN_POINT('Ctrl Pts',(-10.1016805625987,13.4229936740979,-49.9175682080606));
#28347=CARTESIAN_POINT('Ctrl Pts',(-10.4925362263167,13.1261401876617,-49.6451298663487));
#28348=CARTESIAN_POINT('Ctrl Pts',(-10.5148588400716,13.1638007628797,-49.9175682080606));
#28349=CARTESIAN_POINT('Ctrl Pts',(-10.4837073054091,13.4386401852138,-49.9175682080606));
#28350=CARTESIAN_POINT('Ctrl Pts',(-10.8649863601192,13.1261401876617,-49.6050682080606));
#28351=CARTESIAN_POINT('Ctrl Pts',(-10.8649863601192,13.1261401876617,-49.9175682080606));
#28352=CARTESIAN_POINT('Ctrl Pts',(-10.8649863601192,13.4386401876617,-49.9175682080606));
#28353=CARTESIAN_POINT('Origin',(-10.8649863601192,13.4386401876617,-49.6050682080606));
#28354=CARTESIAN_POINT('Origin',(44.4585265683622,13.4386401876617,-44.2925682080604));
#28355=CARTESIAN_POINT('Origin',(49.7710265683622,13.4386401876617,-44.2925682080604));
#28356=CARTESIAN_POINT('Origin',(36.9337491106658,12.8136401876617,-35.0000237973977));
#28357=CARTESIAN_POINT('Origin',(36.9337491106658,12.8136401876617,-35.0000237973977));
#28358=CARTESIAN_POINT('Origin',(36.9337491106658,12.8136401876617,-35.0000237973977));
#28359=CARTESIAN_POINT('Origin',(39.6373121409847,-8.24885981233827,-41.2391207336493));
#28360=CARTESIAN_POINT('Origin',(0.0835265683620477,-8.24885981233827,0.0824317919394229));
#28361=CARTESIAN_POINT('Ctrl Pts',(21.7919948253812,-8.46983068146548,-49.8076885551764));
#28362=CARTESIAN_POINT('Ctrl Pts',(21.8521423242108,-8.48281912914163,-49.7956815989318));
#28363=CARTESIAN_POINT('Ctrl Pts',(21.9125265915097,-8.49383985404005,-49.7835868143488));
#28364=CARTESIAN_POINT('Ctrl Pts',(21.9730858028217,-8.50331222135622,-49.7714165769901));
#28365=CARTESIAN_POINT('Ctrl Pts',(22.0387999717056,-8.51359090121448,-49.7582103773745));
#28366=CARTESIAN_POINT('Ctrl Pts',(22.1047202451555,-8.52204613529236,-49.7449153215987));
#28367=CARTESIAN_POINT('Ctrl Pts',(22.1707904779483,-8.52915470826165,-49.7315420543742));
#28368=CARTESIAN_POINT('Ctrl Pts',(22.2084677088732,-8.53320844523197,-49.7239158109641));
#28369=CARTESIAN_POINT('Ctrl Pts',(22.2461941051687,-8.53682321976947,-49.7162640419939));
#28370=CARTESIAN_POINT('Ctrl Pts',(22.2839618928278,-8.54008060317762,-49.7085880973647));
#28371=CARTESIAN_POINT('Ctrl Pts',(22.2853194127144,-8.54019768609481,-49.7083121943232));
#28372=CARTESIAN_POINT('Ctrl Pts',(22.2866770266266,-8.54031425987122,-49.7080362514587));
#28373=CARTESIAN_POINT('Ctrl Pts',(22.2880347319652,-8.54043032524655,-49.7077602693195));
#28374=CARTESIAN_POINT('Ctrl Pts',(22.3534462848796,-8.54602212504614,-49.6944639967121));
#28375=CARTESIAN_POINT('Ctrl Pts',(22.4189815616388,-8.55043067995687,-49.681094851513));
#28376=CARTESIAN_POINT('Ctrl Pts',(22.4845845014327,-8.55374151002609,-49.667665924648));
#28377=CARTESIAN_POINT('Ctrl Pts',(22.550095188687,-8.55704768432099,-49.6542558818851));
#28378=CARTESIAN_POINT('Ctrl Pts',(22.6156761216241,-8.55925889971346,-49.6407856528723));
#28379=CARTESIAN_POINT('Ctrl Pts',(22.6812748008842,-8.56041391612642,-49.6272656412831));
#28380=CARTESIAN_POINT('Ctrl Pts',(22.7171068924841,-8.56104482294307,-49.6198805795844));
#28381=CARTESIAN_POINT('Ctrl Pts',(22.7529440968362,-8.56135981233827,-49.6124806680525));
#28382=CARTESIAN_POINT('Ctrl Pts',(22.7887737236329,-8.56135981233827,-49.6050682080606));
#28383=CARTESIAN_POINT('Ctrl Pts',(-37.4986912084115,-8.46983068145905,
-39.2604024894787));
#28384=CARTESIAN_POINT('Ctrl Pts',(-37.7185740154056,-8.46631238203734,
-39.045494006553));
#28385=CARTESIAN_POINT('Ctrl Pts',(-37.8722959448872,-8.24885981233825,
-39.1992159360346));
#28386=CARTESIAN_POINT('Ctrl Pts',(-36.4073256331548,-6.92666471828356,
-38.1688349292187));
#28387=CARTESIAN_POINT('Ctrl Pts',(-36.6274219671529,-6.92339564385727,
-37.9543419582776));
#28388=CARTESIAN_POINT('Ctrl Pts',(-36.7808270652083,-6.7056938484836,-38.1077470563557));
#28389=CARTESIAN_POINT('Ctrl Pts',(-35.3159568179087,-5.38351572788376,
-37.0772471608834));
#28390=CARTESIAN_POINT('Ctrl Pts',(-35.5360656597061,-5.38020745678442,
-36.8629856508611));
#28391=CARTESIAN_POINT('Ctrl Pts',(-35.6893461724156,-5.16254485804107,
-37.016266163563));
#28392=CARTESIAN_POINT('Ctrl Pts',(-34.2245838299083,-3.84038894321748,
-35.9856330592973));
#28393=CARTESIAN_POINT('Ctrl Pts',(-34.4443617566355,-3.83655054711529,
-35.7712817477829));
#28394=CARTESIAN_POINT('Ctrl Pts',(-34.5978496132723,-3.61941807409668,
-35.9247696044197));
#28395=CARTESIAN_POINT('Origin',(-37.6513250757665,-8.24885981233827,-39.4201868051554));
#28396=CARTESIAN_POINT('Origin',(-24.4075899551548,12.8136401876617,-26.1764516845438));
#28397=CARTESIAN_POINT('Origin',(-38.8073463968981,12.8136401876617,-40.576208126287));
#28398=CARTESIAN_POINT('Origin',(0.0835265683620477,13.4386401876617,-49.6050682080606));
#28399=CARTESIAN_POINT('Origin',(-44.2914734316379,13.4386401876617,-49.6050682080606));
#28400=CARTESIAN_POINT('Origin',(49.7710265683621,13.4386401876617,0.0824317919395964));
#28401=CARTESIAN_POINT('Origin',(49.7710265683621,13.4386401876617,-10.8660811365416));
#28402=CARTESIAN_POINT('Origin',(0.0835265683620477,12.8136401876617,0.0824317919394229));
#28403=CARTESIAN_POINT('Ctrl Pts',(49.9887116253026,13.0346110567825,-8.62119821111519));
#28404=CARTESIAN_POINT('Ctrl Pts',(49.9661757048102,13.0572884391283,-8.88240655691535));
#28405=CARTESIAN_POINT('Ctrl Pts',(49.9426352641249,13.0745923805885,-9.14384146257121));
#28406=CARTESIAN_POINT('Ctrl Pts',(49.918105661078,13.0880420719089,-9.40541317909589));
#28407=CARTESIAN_POINT('Ctrl Pts',(49.9075481310961,13.0938308129289,-9.51799352678263));
#28408=CARTESIAN_POINT('Ctrl Pts',(49.8968072588538,13.0989048483046,-9.63059933088929));
#28409=CARTESIAN_POINT('Ctrl Pts',(49.8858838002042,13.1033825850674,-9.74322381006683));
#28410=CARTESIAN_POINT('Ctrl Pts',(49.8858546717335,13.1033945253904,-9.74352413425422));
#28411=CARTESIAN_POINT('Ctrl Pts',(49.8858255419225,13.1034064614893,-9.74382445900064));
#28412=CARTESIAN_POINT('Ctrl Pts',(49.8857964107712,13.1034183933662,-9.74412478430632));
#28413=CARTESIAN_POINT('Ctrl Pts',(49.8621111558389,13.113119676523,-9.98830605051857));
#28414=CARTESIAN_POINT('Ctrl Pts',(49.8375747661617,13.1198333629724,-10.2324983067964));
#28415=CARTESIAN_POINT('Ctrl Pts',(49.8122023193407,13.123330972524,-10.4766688600581));
#28416=CARTESIAN_POINT('Ctrl Pts',(49.7987131033095,13.1251904703945,-10.6064816985539));
#28417=CARTESIAN_POINT('Ctrl Pts',(49.7849874188113,13.1261401876617,-10.7362881913535));
#28418=CARTESIAN_POINT('Ctrl Pts',(49.7710265683621,13.1261401876617,-10.8660811365416));
#28419=CARTESIAN_POINT('Origin',(36.6227242513098,12.3739187291548,-34.6889992126612));
#28420=CARTESIAN_POINT('Origin',(36.3116988338421,11.9341984494202,-34.377973520574));
#28421=CARTESIAN_POINT('Ctrl Pts',(22.7887737236329,-8.87385981233827,-49.9175682080606));
#28422=CARTESIAN_POINT('Ctrl Pts',(22.7887737236329,-8.56135981233826,-49.9175682080606));
#28423=CARTESIAN_POINT('Ctrl Pts',(22.7887737236329,-8.56135981233827,-49.6050682080606));
#28424=CARTESIAN_POINT('Ctrl Pts',(22.6060432734091,-8.87385981115686,-49.9175682080606));
#28425=CARTESIAN_POINT('Ctrl Pts',(22.630506965973,-8.59410214473098,-49.9175682080606));
#28426=CARTESIAN_POINT('Ctrl Pts',(22.6218302886772,-8.56135981233827,-49.6396055907562));
#28427=CARTESIAN_POINT('Ctrl Pts',(22.4199497037722,-8.86016990857446,-49.9175682080606));
#28428=CARTESIAN_POINT('Ctrl Pts',(22.4537595355486,-8.61269267441879,-49.9175682080606));
#28429=CARTESIAN_POINT('Ctrl Pts',(22.4513199439386,-8.55451485837127,-49.6745741172675));
#28430=CARTESIAN_POINT('Ctrl Pts',(22.0556610128347,-8.80243256293693,-49.9175682080606));
#28431=CARTESIAN_POINT('Ctrl Pts',(22.1054332504262,-8.61241087733877,-49.9175682080606));
#28432=CARTESIAN_POINT('Ctrl Pts',(22.1166038668002,-8.52564618972366,-49.7426016210618));
#28433=CARTESIAN_POINT('Ctrl Pts',(21.8765903956183,-8.75973143359561,-49.9175682080606));
#28434=CARTESIAN_POINT('Ctrl Pts',(21.9308811035567,-8.59777411058361,-49.9175682080626));
#28435=CARTESIAN_POINT('Ctrl Pts',(21.9517844512709,-8.50433615795936,-49.7757905000569));
#28436=CARTESIAN_POINT('Ctrl Pts',(21.7038295264605,-8.69080155058829,-49.9175682080606));
#28437=CARTESIAN_POINT('Ctrl Pts',(21.7573153886808,-8.5567486113334,-49.9175682080606));
#28438=CARTESIAN_POINT('Ctrl Pts',(21.7919948253812,-8.46983068146548,-49.8076885551764));
#28439=CARTESIAN_POINT('Origin',(21.7038295264614,-8.69080155057986,-49.6050682080606));
#28440=CARTESIAN_POINT('Origin',(22.7887737236329,-8.87385981233827,-49.6050682080606));
#28441=CARTESIAN_POINT('Origin',(-37.6513250757665,-8.24885981233827,-39.4201868051554));
#28442=CARTESIAN_POINT('Origin',(-37.6513250757665,-8.24885981233827,-39.4201868051554));
#28443=CARTESIAN_POINT('Origin',(-37.6513250757665,-8.24885981233827,-39.4201868051554));
#28444=CARTESIAN_POINT('Origin',(-39.6912298733813,12.8136401876617,-39.6923246498039));
#28445=CARTESIAN_POINT('Origin',(-40.5751133498644,12.8136401876617,-38.8084411733207));
#28446=CARTESIAN_POINT('Origin',(-44.291473431638,13.4386401876617,-44.2925682080606));
#28447=CARTESIAN_POINT('Origin',(-49.603973431638,13.4386401876617,-44.2925682080605));
#28448=CARTESIAN_POINT('Ctrl Pts',(49.9887116253026,13.0346110567825,-8.62119821111519));
#28449=CARTESIAN_POINT('Ctrl Pts',(50.0835265683621,13.1253379748597,-8.60561042268191));
#28450=CARTESIAN_POINT('Ctrl Pts',(50.0835265683621,13.2555819259033,-8.58323321427883));
#28451=CARTESIAN_POINT('Ctrl Pts',(49.956506353427,13.0670184804063,-8.99448160864149));
#28452=CARTESIAN_POINT('Ctrl Pts',(50.0835265683621,13.1643191174749,-8.99361854621833));
#28453=CARTESIAN_POINT('Ctrl Pts',(50.0835265683621,13.3203828042289,-8.96039929864488));
#28454=CARTESIAN_POINT('Ctrl Pts',(49.9221708848413,13.0885197051919,-9.36912528698815));
#28455=CARTESIAN_POINT('Ctrl Pts',(50.0835265683621,13.1804336598305,-9.37537845335551));
#28456=CARTESIAN_POINT('Ctrl Pts',(50.0835265683621,13.363399222363,-9.34018351565049));
#28457=CARTESIAN_POINT('Ctrl Pts',(49.8494215535246,13.1183169307007,-10.1191242934122));
#28458=CARTESIAN_POINT('Ctrl Pts',(50.0835265683621,13.1821517325915,-10.1329527188525));
#28459=CARTESIAN_POINT('Ctrl Pts',(50.0835265683621,13.4229936740986,-10.1027753390215));
#28460=CARTESIAN_POINT('Ctrl Pts',(49.8110882266463,13.1261401876617,-10.4936310027383));
#28461=CARTESIAN_POINT('Ctrl Pts',(50.0835265683621,13.163800762876,-10.5159536164931));
#28462=CARTESIAN_POINT('Ctrl Pts',(50.0835265683621,13.4386401852138,-10.4848020818312));
#28463=CARTESIAN_POINT('Ctrl Pts',(49.7710265683621,13.1261401876617,-10.8660811365416));
#28464=CARTESIAN_POINT('Ctrl Pts',(50.0835265683621,13.1261401876617,-10.8660811365416));
#28465=CARTESIAN_POINT('Ctrl Pts',(50.0835265683621,13.4386401876617,-10.8660811365416));
#28466=CARTESIAN_POINT('Origin',(49.7710265683621,13.2555819259033,-8.58323321427883));
#28467=CARTESIAN_POINT('Origin',(36.3116988338421,11.9341984494201,-34.377973520574));
#28468=CARTESIAN_POINT('Origin',(36.3116988338421,11.9341984494201,-34.377973520574));
#28469=CARTESIAN_POINT('Origin',(36.3116988338421,11.9341984494201,-34.377973520574));
#28470=CARTESIAN_POINT('Origin',(41.4050790939511,-8.24885981233827,-39.4713537806829));
#28471=CARTESIAN_POINT('Origin',(39.586145165457,-8.24885981233827,-37.6524198521889));
#28472=CARTESIAN_POINT('Origin',(0.0835265683620477,-8.87385981233827,-49.6050682080606));
#28473=CARTESIAN_POINT('Origin',(44.4585265683622,-8.87385981233827,-49.6050682080606));
#28474=CARTESIAN_POINT('Ctrl Pts',(21.9120191201608,-8.77420095227338,-49.9175682080606));
#28475=CARTESIAN_POINT('Ctrl Pts',(21.9659793624217,-8.6400331083672,-49.9175682080606));
#28476=CARTESIAN_POINT('Ctrl Pts',(22.0009097439611,-8.55319446848574,-49.8073324854834));
#28477=CARTESIAN_POINT('Ctrl Pts',(18.416083709289,-7.36815837305484,-49.9175682080606));
#28478=CARTESIAN_POINT('Ctrl Pts',(18.4800995730594,-7.24249091494012,-49.9175682080606));
#28479=CARTESIAN_POINT('Ctrl Pts',(18.4930530061579,-7.14715496089317,-49.8125752704599));
#28480=CARTESIAN_POINT('Ctrl Pts',(14.8511163433864,-6.21561709174538,-49.9175682080606));
#28481=CARTESIAN_POINT('Ctrl Pts',(14.9005782180646,-6.08656532545208,-49.9175682080606));
#28482=CARTESIAN_POINT('Ctrl Pts',(14.914458845539,-5.9946085575776,-49.8172935699712));
#28483=CARTESIAN_POINT('Ctrl Pts',(9.39579666290848,-5.02557369219655,-49.9175682080606));
#28484=CARTESIAN_POINT('Ctrl Pts',(9.42266531444727,-4.8958192523429,-49.9175682080606));
#28485=CARTESIAN_POINT('Ctrl Pts',(9.43658922229887,-4.80456526664712,-49.8223359778271));
#28486=CARTESIAN_POINT('Ctrl Pts',(7.57838814645687,-4.71947214408127,-49.9175682080606));
#28487=CARTESIAN_POINT('Ctrl Pts',(7.59939962270635,-4.58961053626329,-49.9175682080606));
#28488=CARTESIAN_POINT('Ctrl Pts',(7.61140680648957,-4.4984637156123,-49.823670236462));
#28489=CARTESIAN_POINT('Ctrl Pts',(4.81242924625007,-4.40691837826564,-49.9175682080606));
#28490=CARTESIAN_POINT('Ctrl Pts',(4.82512043530452,-4.2772572131369,-49.9175682080606));
#28491=CARTESIAN_POINT('Ctrl Pts',(4.8333804099258,-4.18590981848868,-49.8250429970702));
#28492=CARTESIAN_POINT('Ctrl Pts',(3.88371419304163,-4.327158062246,-49.9175682080606));
#28493=CARTESIAN_POINT('Ctrl Pts',(3.89381225256888,-4.19755005843117,-49.9175682080606));
#28494=CARTESIAN_POINT('Ctrl Pts',(3.9005754487046,-4.1061494680653,-49.8253960354399));
#28495=CARTESIAN_POINT('Ctrl Pts',(2.01256027103393,-4.21946011836696,-49.9175682080606));
#28496=CARTESIAN_POINT('Ctrl Pts',(2.01779667868678,-4.08996813964017,-49.9175682080606));
#28497=CARTESIAN_POINT('Ctrl Pts',(2.02114001333537,-3.99845145937632,-49.8258735845114));
#28498=CARTESIAN_POINT('Ctrl Pts',(1.0793230968735,-4.19205938565825,-49.9175682080606));
#28499=CARTESIAN_POINT('Ctrl Pts',(1.08192261688495,-4.06258497561548,-49.9175682080606));
#28500=CARTESIAN_POINT('Ctrl Pts',(1.08375236041024,-3.9710507150754,-49.8259956725485));
#28501=CARTESIAN_POINT('Ctrl Pts',(-3.57528016808697,-4.18598197768416,
-49.9175682080606));
#28502=CARTESIAN_POINT('Ctrl Pts',(-3.58473840334075,-4.05651422028169,
-49.9175682080606));
#28503=CARTESIAN_POINT('Ctrl Pts',(-3.59155443180908,-3.96497330343923,
-49.8260227101939));
#28504=CARTESIAN_POINT('Ctrl Pts',(-7.26155728764166,-4.60394036703586,
-49.9175682080606));
#28505=CARTESIAN_POINT('Ctrl Pts',(-7.29225903965945,-4.47650762043256,
-49.9175682080606));
#28506=CARTESIAN_POINT('Ctrl Pts',(-7.29419220051882,-4.38293092070441,
-49.8241256417463));
#28507=CARTESIAN_POINT('Ctrl Pts',(-11.8283085920387,-5.59091481619605,
-49.9175682080606));
#28508=CARTESIAN_POINT('Ctrl Pts',(-11.8595750836968,-5.46011080390599,
-49.9175682080606));
#28509=CARTESIAN_POINT('Ctrl Pts',(-11.8798541643496,-5.36990690683693,
-49.8199398075984));
#28510=CARTESIAN_POINT('Ctrl Pts',(-12.7389229297277,-5.81129472998947,
-49.9175682080606));
#28511=CARTESIAN_POINT('Ctrl Pts',(-12.7725641377111,-5.68032983292167,
-49.9175682080606));
#28512=CARTESIAN_POINT('Ctrl Pts',(-12.7941716628244,-5.59028691905929,
-49.8190149631812));
#28513=CARTESIAN_POINT('Ctrl Pts',(-14.5390501691854,-6.29050753230873,
-49.9175682080606));
#28514=CARTESIAN_POINT('Ctrl Pts',(-14.5770895837205,-6.15904772772748,
-49.9175682080606));
#28515=CARTESIAN_POINT('Ctrl Pts',(-14.6014698233081,-6.06949999371313,
-49.817034098248));
#28516=CARTESIAN_POINT('Ctrl Pts',(-15.4308544492521,-6.54980455615392,
-49.9175682080606));
#28517=CARTESIAN_POINT('Ctrl Pts',(-15.4711362244083,-6.41814737485005,
-49.9175682080606));
#28518=CARTESIAN_POINT('Ctrl Pts',(-15.4967513843562,-6.32879713522007,
-49.8159761217162));
#28519=CARTESIAN_POINT('Ctrl Pts',(-18.083799066244,-7.38126084278977,-49.9175682080606));
#28520=CARTESIAN_POINT('Ctrl Pts',(-18.133230497015,-7.2496461959732,-49.9175682080606));
#28521=CARTESIAN_POINT('Ctrl Pts',(-18.1597996579572,-7.16025352122019,
-49.8126404346489));
#28522=CARTESIAN_POINT('Ctrl Pts',(-19.8225328933696,-8.00683451480551,
-49.9175682080606));
#28523=CARTESIAN_POINT('Ctrl Pts',(-19.8764542487545,-7.87510646585778,
-49.9175682080606));
#28524=CARTESIAN_POINT('Ctrl Pts',(-19.9048327172755,-7.78582757943561,
-49.8102024034937));
#28525=CARTESIAN_POINT('Ctrl Pts',(-21.5367763897373,-8.69080155057986,
-49.9175682080606));
#28526=CARTESIAN_POINT('Ctrl Pts',(-21.5902754221335,-8.55671560258979,
-49.9175682080606));
#28527=CARTESIAN_POINT('Ctrl Pts',(-21.6249557626307,-8.4697954075151,-49.8076439541995));
#28528=CARTESIAN_POINT('Origin',(-21.5367763897373,-8.69080155057986,-49.6050682080606));
#28529=CARTESIAN_POINT('Origin',(0.0835265683620477,-8.24885981233827,0.0824317919394229));
#28530=CARTESIAN_POINT('Ctrl Pts',(-22.6217205869088,-8.56135981233827,
-49.6050682080606));
#28531=CARTESIAN_POINT('Ctrl Pts',(-22.4870650497075,-8.56135981233827,
-49.632925846288));
#28532=CARTESIAN_POINT('Ctrl Pts',(-22.3526852962314,-8.55702114807138,
-49.660532025143));
#28533=CARTESIAN_POINT('Ctrl Pts',(-22.218611604898,-8.54791555691041,-49.6878806083244));
#28534=CARTESIAN_POINT('Ctrl Pts',(-22.1862325124773,-8.54571653654471,
-49.6944853515339));
#28535=CARTESIAN_POINT('Ctrl Pts',(-22.1538713295352,-8.5432392648958,-49.7010750507536));
#28536=CARTESIAN_POINT('Ctrl Pts',(-22.1215285998496,-8.54047726034825,
-49.7076495796239));
#28537=CARTESIAN_POINT('Ctrl Pts',(-22.1202156261661,-8.54036513501685,
-49.7079164768052));
#28538=CARTESIAN_POINT('Ctrl Pts',(-22.118902733746,-8.54025254469889,-49.7081833384701));
#28539=CARTESIAN_POINT('Ctrl Pts',(-22.117589920377,-8.54013948886801,-49.7084501650743));
#28540=CARTESIAN_POINT('Ctrl Pts',(-22.0560724680956,-8.53484177721648,
-49.7209534601193));
#28541=CARTESIAN_POINT('Ctrl Pts',(-21.9945592187267,-8.5285710544529,-49.733413252321));
#28542=CARTESIAN_POINT('Ctrl Pts',(-21.9331497324827,-8.52099310668472,
-49.7458111112004));
#28543=CARTESIAN_POINT('Ctrl Pts',(-21.8801974450504,-8.51445877961392,
-49.7565015603001));
#28544=CARTESIAN_POINT('Ctrl Pts',(-21.8273216695811,-8.50695259656883,
-49.767146064923));
#28545=CARTESIAN_POINT('Ctrl Pts',(-21.7746031077857,-8.49822768693253,
-49.7777286249897));
#28546=CARTESIAN_POINT('Ctrl Pts',(-21.7245435456955,-8.48994284112497,
-49.7877774257287));
#28547=CARTESIAN_POINT('Ctrl Pts',(-21.6746251818596,-8.48055949752606,
-49.7977704781088));
#28548=CARTESIAN_POINT('Ctrl Pts',(-21.6249416886588,-8.46983068145907,
-49.8076885551783));
#28549=CARTESIAN_POINT('Origin',(-39.4702590042605,-8.24885981233827,-41.2391207336494));
#28550=CARTESIAN_POINT('Origin',(-26.1753569081211,12.8136401876617,-24.4086847315773));
#28551=CARTESIAN_POINT('Origin',(-36.7666959739416,12.8136401876617,-35.0000237973978));
#28552=CARTESIAN_POINT('Origin',(0.0835265683620477,12.8136401876617,0.0824317919394229));
#28553=CARTESIAN_POINT('Ctrl Pts',(-49.603973431638,13.1261401876617,-10.8660811365418));
#28554=CARTESIAN_POINT('Ctrl Pts',(-49.644220100234,13.1261401876617,-10.4919109761389));
#28555=CARTESIAN_POINT('Ctrl Pts',(-49.6825074995808,13.1182694471954,-10.1177151148479));
#28556=CARTESIAN_POINT('Ctrl Pts',(-49.7188065373979,13.1033923474055,-9.74347094847105));
#28557=CARTESIAN_POINT('Ctrl Pts',(-49.718812100481,13.1033900673852,-9.74341359291761));
#28558=CARTESIAN_POINT('Ctrl Pts',(-49.7188176635159,13.1033877872102,-9.74335623737716));
#28559=CARTESIAN_POINT('Ctrl Pts',(-49.7188232265025,13.1033855068804,-9.74329888184971));
#28560=CARTESIAN_POINT('Ctrl Pts',(-49.7399406684873,13.0947292335955,-9.52557374406794));
#28561=CARTESIAN_POINT('Ctrl Pts',(-49.7603774319321,13.0838402503142,-9.30789186800036));
#28562=CARTESIAN_POINT('Ctrl Pts',(-49.7801260723316,13.0698690454478,-9.09033516972605));
#28563=CARTESIAN_POINT('Ctrl Pts',(-49.7943282328449,13.0598217059822,-8.93388008790132));
#28564=CARTESIAN_POINT('Ctrl Pts',(-49.8081743398752,13.0481798478112,-8.77748968268304));
#28565=CARTESIAN_POINT('Ctrl Pts',(-49.8216584885772,13.0346110567867,-8.62119821111491));
#28566=CARTESIAN_POINT('Origin',(-36.7666959739416,12.8136401876617,-35.0000237973978));
#28567=CARTESIAN_POINT('Origin',(-49.603973431638,13.4386401876617,0.0824317919394229));
#28568=CARTESIAN_POINT('Origin',(-49.603973431638,13.4386401876617,-10.8660811365418));
#28569=CARTESIAN_POINT('Ctrl Pts',(49.9887116253026,13.0346110567825,8.78606179499438));
#28570=CARTESIAN_POINT('Ctrl Pts',(50.083526568362,13.1253379748597,8.77047400656112));
#28571=CARTESIAN_POINT('Ctrl Pts',(50.083526568362,13.2555819259033,8.74809679815803));
#28572=CARTESIAN_POINT('Ctrl Pts',(49.9908311071223,12.5435283274362,5.91561885766924));
#28573=CARTESIAN_POINT('Ctrl Pts',(50.083526568362,12.6357570952139,5.91066276265311));
#28574=CARTESIAN_POINT('Ctrl Pts',(50.083526568362,12.7644980954124,5.88980021407049));
#28575=CARTESIAN_POINT('Ctrl Pts',(49.9919944362938,12.2852858973076,3.01901638821139));
#28576=CARTESIAN_POINT('Ctrl Pts',(50.0835265683621,12.3768143018414,3.01363906603581));
#28577=CARTESIAN_POINT('Ctrl Pts',(50.083526568362,12.5062567663973,3.00601459538233));
#28578=CARTESIAN_POINT('Ctrl Pts',(49.9919989292124,12.2842756298938,-1.36854617605777));
#28579=CARTESIAN_POINT('Ctrl Pts',(50.0835265683621,12.3758051232112,-1.36588312104414));
#28580=CARTESIAN_POINT('Ctrl Pts',(50.0835265683621,12.5052464990302,-1.36212193922448));
#28581=CARTESIAN_POINT('Ctrl Pts',(49.9917102361039,12.3489547591789,-2.84244469713244));
#28582=CARTESIAN_POINT('Ctrl Pts',(50.0835265683621,12.4404805872093,-2.83784203918765));
#28583=CARTESIAN_POINT('Ctrl Pts',(50.0835265683621,12.5699256283428,-2.82949528855841));
#28584=CARTESIAN_POINT('Ctrl Pts',(49.9905929379208,12.602124859829,-5.75141479186526));
#28585=CARTESIAN_POINT('Ctrl Pts',(50.0835265683621,12.69337879361,-5.74157443732728));
#28586=CARTESIAN_POINT('Ctrl Pts',(50.0835265683621,12.8230957289067,-5.72573254687836));
#28587=CARTESIAN_POINT('Ctrl Pts',(49.9897665577655,12.7901838029195,-7.19248886629495));
#28588=CARTESIAN_POINT('Ctrl Pts',(50.0835265683621,12.8814125534697,-7.18075767287272));
#28589=CARTESIAN_POINT('Ctrl Pts',(50.0835265683621,13.011154579071,-7.16057213889734));
#28590=CARTESIAN_POINT('Ctrl Pts',(49.9887116253026,13.0346110567825,-8.62119821111519));
#28591=CARTESIAN_POINT('Ctrl Pts',(50.0835265683621,13.1253379748596,-8.60561042268192));
#28592=CARTESIAN_POINT('Ctrl Pts',(50.0835265683621,13.2555819259033,-8.58323321427883));
#28593=CARTESIAN_POINT('Origin',(49.771026568362,13.2555819259033,8.74809679815802));
#28594=CARTESIAN_POINT('Origin',(0.0835265683620477,11.9341984494201,0.0824317919394229));
#28595=CARTESIAN_POINT('Origin',(36.311698833842,11.9341984494201,34.542837104453));
#28596=CARTESIAN_POINT('Origin',(36.3116988338421,11.4830954176946,-34.377973520574));
#28597=CARTESIAN_POINT('Origin',(36.3116988338421,-3.61941807409669,-34.377973520574));
#28598=CARTESIAN_POINT('Ctrl Pts',(39.4263608497803,-8.46983068145906,-37.499785984834));
#28599=CARTESIAN_POINT('Ctrl Pts',(39.2114523668546,-8.46631238203735,-37.7196687918281));
#28600=CARTESIAN_POINT('Ctrl Pts',(39.3651742963362,-8.24885981233826,-37.8733907213097));
#28601=CARTESIAN_POINT('Ctrl Pts',(38.3347932895204,-6.92666471828348,-36.4084204095771));
#28602=CARTESIAN_POINT('Ctrl Pts',(38.120300318573,-6.92339564386607,-36.6285167435691));
#28603=CARTESIAN_POINT('Ctrl Pts',(38.273705416651,-6.70569384849234,-36.7819218416245));
#28604=CARTESIAN_POINT('Ctrl Pts',(37.24320552117,-5.38351572788356,-35.3170515943467));
#28605=CARTESIAN_POINT('Ctrl Pts',(37.0289440111501,-5.38020745678081,-35.5371604361463));
#28606=CARTESIAN_POINT('Ctrl Pts',(37.1822245238672,-5.16254485803749,-35.6904409488406));
#28607=CARTESIAN_POINT('Ctrl Pts',(36.1515914195989,-3.84038894321748,-34.2256786063308));
#28608=CARTESIAN_POINT('Ctrl Pts',(35.9372401080845,-3.8365505471153,-34.445456533058));
#28609=CARTESIAN_POINT('Ctrl Pts',(36.0907279647213,-3.61941807409669,-34.5989443896948));
#28610=CARTESIAN_POINT('Origin',(39.586145165457,-8.24885981233827,-37.6524198521889));
#28611=CARTESIAN_POINT('Origin',(36.3116988338421,-3.61941807409669,-34.377973520574));
#28612=CARTESIAN_POINT('Origin',(39.586145165457,-8.24885981233827,-37.6524198521889));
#28613=CARTESIAN_POINT('Origin',(39.586145165457,-8.24885981233827,-37.6524198521889));
#28614=CARTESIAN_POINT('Origin',(44.4585265683622,-8.87385981233827,-44.2925682080604));
#28615=CARTESIAN_POINT('Origin',(49.7710265683622,-8.87385981233827,-44.2925682080604));
#28616=CARTESIAN_POINT('Ctrl Pts',(-22.6217205869088,-8.56135981233827,
-49.6050682080606));
#28617=CARTESIAN_POINT('Ctrl Pts',(-22.6217205869088,-8.56135981233827,
-49.9175682080606));
#28618=CARTESIAN_POINT('Ctrl Pts',(-22.6217205869088,-8.87385981233827,
-49.9175682080606));
#28619=CARTESIAN_POINT('Ctrl Pts',(-22.4523904056315,-8.56135981233827,
-49.6400993625636));
#28620=CARTESIAN_POINT('Ctrl Pts',(-22.4612973244651,-8.59454828035443,
-49.9175682080606));
#28621=CARTESIAN_POINT('Ctrl Pts',(-22.436382391298,-8.87385980853143,-49.9175682080606));
#28622=CARTESIAN_POINT('Ctrl Pts',(-22.2842585826169,-8.55449257599307,
-49.6745749606216));
#28623=CARTESIAN_POINT('Ctrl Pts',(-22.2866330693819,-8.61264419244103,
-49.9175682080606));
#28624=CARTESIAN_POINT('Ctrl Pts',(-22.2528889951113,-8.86012534447524,
-49.9175682080606));
#28625=CARTESIAN_POINT('Ctrl Pts',(-21.9509213395377,-8.52578588737924,
-49.7423238840037));
#28626=CARTESIAN_POINT('Ctrl Pts',(-21.9397562137707,-8.61245644138935,
-49.9175682080606));
#28627=CARTESIAN_POINT('Ctrl Pts',(-21.8900982070676,-8.80271195759283,
-49.9175682080606));
#28628=CARTESIAN_POINT('Ctrl Pts',(-21.7844807419713,-8.5042820521619,-49.7758405246614));
#28629=CARTESIAN_POINT('Ctrl Pts',(-21.7635637494166,-8.59771167170021,
-49.9175682080606));
#28630=CARTESIAN_POINT('Ctrl Pts',(-21.7092890597639,-8.75963242031969,
-49.9175682080606));
#28631=CARTESIAN_POINT('Ctrl Pts',(-21.6249416886588,-8.46983068145907,
-49.8076885551783));
#28632=CARTESIAN_POINT('Ctrl Pts',(-21.5902622519579,-8.55674861132668,
-49.9175682080606));
#28633=CARTESIAN_POINT('Ctrl Pts',(-21.5367763897373,-8.69080155057986,
-49.9175682080606));
#28634=CARTESIAN_POINT('Origin',(-22.6217205869088,-8.87385981233827,-49.6050682080606));
#28635=CARTESIAN_POINT('Origin',(-36.7666959739416,12.8136401876617,-35.0000237973978));
#28636=CARTESIAN_POINT('Origin',(-36.7666959739416,12.8136401876617,-35.0000237973978));
#28637=CARTESIAN_POINT('Ctrl Pts',(-49.603973431638,13.1261401876617,-10.8660811365418));
#28638=CARTESIAN_POINT('Ctrl Pts',(-49.916473431638,13.1261401876617,-10.8660811365418));
#28639=CARTESIAN_POINT('Ctrl Pts',(-49.916473431638,13.4386401876617,-10.8660811365418));
#28640=CARTESIAN_POINT('Ctrl Pts',(-49.6441532614126,13.1261401876617,-10.4925323714846));
#28641=CARTESIAN_POINT('Ctrl Pts',(-49.916473431638,13.1639055963079,-10.5149789866091));
#28642=CARTESIAN_POINT('Ctrl Pts',(-49.916473431638,13.4386401851022,-10.4836786957547));
#28643=CARTESIAN_POINT('Ctrl Pts',(-49.6824505602016,13.1182927286052,-10.118301392099));
#28644=CARTESIAN_POINT('Ctrl Pts',(-49.9164734316366,13.1821712224823,-10.1321042920214));
#28645=CARTESIAN_POINT('Ctrl Pts',(-49.916473431638,13.4229452699559,-10.1019371937965));
#28646=CARTESIAN_POINT('Ctrl Pts',(-49.7551624447503,13.0884919386939,-9.3686405069943));
#28647=CARTESIAN_POINT('Ctrl Pts',(-49.9164734316392,13.1804128114024,-9.37487243571382));
#28648=CARTESIAN_POINT('Ctrl Pts',(-49.916473431638,13.3633436893187,-9.33969202550905));
#28649=CARTESIAN_POINT('Ctrl Pts',(-49.789510779629,13.066960554456,-8.99381440095842));
#28650=CARTESIAN_POINT('Ctrl Pts',(-49.9164734316379,13.1642472289408,-8.99290301434246));
#28651=CARTESIAN_POINT('Ctrl Pts',(-49.916473431638,13.3202672259813,-8.95972660866116));
#28652=CARTESIAN_POINT('Ctrl Pts',(-49.8216584885772,13.0346110567867,-8.62119821111442));
#28653=CARTESIAN_POINT('Ctrl Pts',(-49.9164734316379,13.125337974864,-8.60561042268131));
#28654=CARTESIAN_POINT('Ctrl Pts',(-49.916473431638,13.2555819259088,-8.5832332142783));
#28655=CARTESIAN_POINT('Origin',(-49.603973431638,13.2555819259033,-8.58323321427904));
#28656=CARTESIAN_POINT('Ctrl Pts',(49.771026568362,13.1261401876617,11.0309447204208));
#28657=CARTESIAN_POINT('Ctrl Pts',(50.083526568362,13.1261401876617,11.0309447204208));
#28658=CARTESIAN_POINT('Ctrl Pts',(50.083526568362,13.4386401876617,11.0309447204208));
#28659=CARTESIAN_POINT('Ctrl Pts',(49.8112063981312,13.1261401876617,10.657395955363));
#28660=CARTESIAN_POINT('Ctrl Pts',(50.083526568362,13.1639055963028,10.6798425704875));
#28661=CARTESIAN_POINT('Ctrl Pts',(50.083526568362,13.4386401851022,10.6485422796337));
#28662=CARTESIAN_POINT('Ctrl Pts',(49.8495036969259,13.1182927286052,10.2831649759781));
#28663=CARTESIAN_POINT('Ctrl Pts',(50.0835265683606,13.1821712224833,10.2969678759003));
#28664=CARTESIAN_POINT('Ctrl Pts',(50.083526568362,13.4229452699559,10.2668007776755));
#28665=CARTESIAN_POINT('Ctrl Pts',(49.9222155814742,13.0884919386938,9.53350409087325));
#28666=CARTESIAN_POINT('Ctrl Pts',(50.0835265683633,13.1804128114014,9.53973601959273));
#28667=CARTESIAN_POINT('Ctrl Pts',(50.083526568362,13.3633436893187,9.50455560938805));
#28668=CARTESIAN_POINT('Ctrl Pts',(49.9565639163529,13.0669605544559,9.15867798483744));
#28669=CARTESIAN_POINT('Ctrl Pts',(50.083526568362,13.1642472289387,9.15776659822167));
#28670=CARTESIAN_POINT('Ctrl Pts',(50.083526568362,13.3202672259815,9.12459019254013));
#28671=CARTESIAN_POINT('Ctrl Pts',(49.9887116253013,13.0346110567867,8.78606179499341));
#28672=CARTESIAN_POINT('Ctrl Pts',(50.083526568362,13.125337974864,8.77047400656029));
#28673=CARTESIAN_POINT('Ctrl Pts',(50.083526568362,13.2555819259088,8.74809679815729));
#28674=CARTESIAN_POINT('Origin',(49.771026568362,13.4386401876617,11.0309447204208));
#28675=CARTESIAN_POINT('Ctrl Pts',(49.9887116253012,13.0346110567867,8.7860617949939));
#28676=CARTESIAN_POINT('Ctrl Pts',(49.9699614074307,13.0534789730025,9.00339098706776));
#28677=CARTESIAN_POINT('Ctrl Pts',(49.9505117180268,13.0686233597236,9.22091083915132));
#28678=CARTESIAN_POINT('Ctrl Pts',(49.930377004077,13.0809296718092,9.4385314775567));
#28679=CARTESIAN_POINT('Ctrl Pts',(49.9158972002272,13.0897797098856,9.59503254162007));
#28680=CARTESIAN_POINT('Ctrl Pts',(49.9010628922511,13.0971603804857,9.7515862513039));
#28681=CARTESIAN_POINT('Ctrl Pts',(49.8858763632264,13.1033855068803,9.90816246572872));
#28682=CARTESIAN_POINT('Ctrl Pts',(49.8858708002398,13.1033877872101,9.90821982125617));
#28683=CARTESIAN_POINT('Ctrl Pts',(49.8858652372049,13.1033900673851,9.90827717679661));
#28684=CARTESIAN_POINT('Ctrl Pts',(49.8858596741218,13.1033923474054,9.90833453235006));
#28685=CARTESIAN_POINT('Ctrl Pts',(49.8495606363048,13.1182694471954,10.282578698727));
#28686=CARTESIAN_POINT('Ctrl Pts',(49.8112732369526,13.1261401876617,10.6567745600179));
#28687=CARTESIAN_POINT('Ctrl Pts',(49.771026568362,13.1261401876617,11.0309447204208));
#28688=CARTESIAN_POINT('Origin',(36.311698833842,11.9341984494201,34.542837104453));
#28689=CARTESIAN_POINT('Origin',(36.311698833842,11.9341984494202,34.542837104453));
#28690=CARTESIAN_POINT('Origin',(36.311698833842,11.9341984494201,34.542837104453));
#28691=CARTESIAN_POINT('Origin',(36.3116988338421,-3.61941807409669,-34.377973520574));
#28692=CARTESIAN_POINT('Origin',(36.3116988338421,-3.61941807409668,-34.377973520574));
#28693=CARTESIAN_POINT('Origin',(0.0835265683620477,-8.24885981233827,0.0824317919394229));
#28694=CARTESIAN_POINT('Ctrl Pts',(49.7710265683621,-8.56135981233827,-22.6228153633312));
#28695=CARTESIAN_POINT('Ctrl Pts',(49.7988842066419,-8.56135981233827,-22.4881598258772));
#28696=CARTESIAN_POINT('Ctrl Pts',(49.8264903855486,-8.55702114805526,-22.3537800721493));
#28697=CARTESIAN_POINT('Ctrl Pts',(49.8538389687804,-8.54791555685928,-22.2197063805655));
#28698=CARTESIAN_POINT('Ctrl Pts',(49.8604437119383,-8.54571653650635,-22.1873272883967));
#28699=CARTESIAN_POINT('Ctrl Pts',(49.8670334111066,-8.54323926487447,-22.1549661057063));
#28700=CARTESIAN_POINT('Ctrl Pts',(49.8736079399258,-8.54047726034837,-22.122623376272));
#28701=CARTESIAN_POINT('Ctrl Pts',(49.8738748371071,-8.54036513501696,-22.1213104025886));
#28702=CARTESIAN_POINT('Ctrl Pts',(49.874141698772,-8.540252544699,-22.1199975101685));
#28703=CARTESIAN_POINT('Ctrl Pts',(49.8744085253762,-8.54013948886812,-22.1186846967995));
#28704=CARTESIAN_POINT('Ctrl Pts',(49.8869118204158,-8.53484177721875,-22.0571672445435));
#28705=CARTESIAN_POINT('Ctrl Pts',(49.8993716126124,-8.52857105445812,-21.9956539952));
#28706=CARTESIAN_POINT('Ctrl Pts',(49.9117694714868,-8.52099310669413,-21.9342445089813));
#28707=CARTESIAN_POINT('Ctrl Pts',(49.9224599205877,-8.51445877962352,-21.881292221543));
#28708=CARTESIAN_POINT('Ctrl Pts',(49.9331044252119,-8.50695259657853,-21.8284164460676));
#28709=CARTESIAN_POINT('Ctrl Pts',(49.9436869852797,-8.49822768694213,-21.7756978842662));
#28710=CARTESIAN_POINT('Ctrl Pts',(49.9537357860226,-8.48994284113222,-21.7256383221565));
#28711=CARTESIAN_POINT('Ctrl Pts',(49.9637288384065,-8.4805594975302,-21.6757199583012));
#28712=CARTESIAN_POINT('Ctrl Pts',(49.9736469154798,-8.46983068145907,-21.6260364650812));
#28713=CARTESIAN_POINT('Origin',(49.7710265683621,-8.87385981233827,0.0824317919395964));
#28714=CARTESIAN_POINT('Origin',(49.7710265683621,-8.87385981233827,-22.6228153633312));
#28715=CARTESIAN_POINT('Origin',(0.0835265683620477,-8.87385981233827,-49.6050682080606));
#28716=CARTESIAN_POINT('Origin',(-44.2914734316379,-8.87385981233827,-49.6050682080606));
#28717=CARTESIAN_POINT('Origin',(-41.2380259572268,-8.24885981233827,-39.4713537806831));
#28718=CARTESIAN_POINT('Origin',(-39.4190920287328,-8.24885981233827,-37.6524198521891));
#28719=CARTESIAN_POINT('Origin',(-36.4556708266332,12.3739193162038,-34.6889986706566));
#28720=CARTESIAN_POINT('Origin',(-36.1446456971179,11.9341984494201,-34.3779735205741));
#28721=CARTESIAN_POINT('Ctrl Pts',(-49.8216584885785,13.0346110567825,-8.62119821111539));
#28722=CARTESIAN_POINT('Ctrl Pts',(-49.916473431638,13.1253379748596,-8.60561042268212));
#28723=CARTESIAN_POINT('Ctrl Pts',(-49.916473431638,13.2555819259033,-8.58323321427904));
#28724=CARTESIAN_POINT('Ctrl Pts',(-49.8237759955599,12.5439858927424,-5.75342980308448));
#28725=CARTESIAN_POINT('Ctrl Pts',(-49.9164734316379,12.6362124110381,-5.74845883635996));
#28726=CARTESIAN_POINT('Ctrl Pts',(-49.916473431638,12.7649555013805,-5.72759890891797));
#28727=CARTESIAN_POINT('Ctrl Pts',(-49.8249470688541,12.2839886353264,-2.84806387820799));
#28728=CARTESIAN_POINT('Ctrl Pts',(-49.916473431638,12.3755184395154,-2.84268189602221));
#28729=CARTESIAN_POINT('Ctrl Pts',(-49.916473431638,12.5049595044998,-2.83508904408025));
#28730=CARTESIAN_POINT('Ctrl Pts',(-49.8249415226426,12.2852357315166,3.03418378172085));
#28731=CARTESIAN_POINT('Ctrl Pts',(-49.9164734316379,12.3767641898923,3.02877807703737));
#28732=CARTESIAN_POINT('Ctrl Pts',(-49.916473431638,12.5062066005848,3.02111483476545));
#28733=CARTESIAN_POINT('Ctrl Pts',(-49.8237672317522,12.5460164567317,5.9301622998315));
#28734=CARTESIAN_POINT('Ctrl Pts',(-49.916473431638,12.6382323220339,5.92512141906298));
#28735=CARTESIAN_POINT('Ctrl Pts',(-49.916473431638,12.7669860817746,5.90428125111807));
#28736=CARTESIAN_POINT('Ctrl Pts',(-49.8216584885785,13.0346110567825,8.78606179499423));
#28737=CARTESIAN_POINT('Ctrl Pts',(-49.9164734316379,13.1253379748596,8.77047400656096));
#28738=CARTESIAN_POINT('Ctrl Pts',(-49.916473431638,13.2555819259033,8.74809679815787));
#28739=CARTESIAN_POINT('Origin',(-49.603973431638,13.2555819259033,8.74809679815787));
#28740=CARTESIAN_POINT('Origin',(49.7710265683621,13.4386401876617,0.0824317919395964));
#28741=CARTESIAN_POINT('Origin',(49.7710265683619,13.4386401876617,36.6697170232579));
#28742=CARTESIAN_POINT('Origin',(0.0835265683620477,12.8136401876617,0.0824317919394229));
#28743=CARTESIAN_POINT('Origin',(36.9337491106657,12.8136401876617,35.1648873812767));
#28744=CARTESIAN_POINT('Origin',(36.6227239633541,12.3739193162048,34.853862254537));
#28745=CARTESIAN_POINT('Origin',(36.9337491106657,12.8136401876617,35.1648873812767));
#28746=CARTESIAN_POINT('Origin',(36.311698833842,11.4830954176946,34.542837104453));
#28747=CARTESIAN_POINT('Origin',(36.311698833842,-3.61941807409668,34.542837104453));
#28748=CARTESIAN_POINT('Origin',(0.0835265683620477,-3.61941807409668,0.0824317919394229));
#28749=CARTESIAN_POINT('Origin',(36.311698833842,-3.61941807409668,34.542837104453));
#28750=CARTESIAN_POINT('Ctrl Pts',(49.7710265683621,-8.56135981233827,-22.6228153633312));
#28751=CARTESIAN_POINT('Ctrl Pts',(50.0835265683621,-8.56135981233826,-22.6228153633312));
#28752=CARTESIAN_POINT('Ctrl Pts',(50.0835265683621,-8.87385981233827,-22.6228153633312));
#28753=CARTESIAN_POINT('Ctrl Pts',(49.8060577228649,-8.56135981233827,-22.453485182054));
#28754=CARTESIAN_POINT('Ctrl Pts',(50.0835265683603,-8.59454828035624,-22.4623921008879));
#28755=CARTESIAN_POINT('Ctrl Pts',(50.0835265683621,-8.87385980853143,-22.4374771677204));
#28756=CARTESIAN_POINT('Ctrl Pts',(49.8405333209238,-8.55449257599331,-22.2853533590394));
#28757=CARTESIAN_POINT('Ctrl Pts',(50.0835265683621,-8.6126441924417,-22.2877278458042));
#28758=CARTESIAN_POINT('Ctrl Pts',(50.0835265683621,-8.86012534447524,-22.2539837715337));
#28759=CARTESIAN_POINT('Ctrl Pts',(49.9082822443045,-8.52578588737901,-21.9520161159601));
#28760=CARTESIAN_POINT('Ctrl Pts',(50.0835265683621,-8.61245644138874,-21.940850990193));
#28761=CARTESIAN_POINT('Ctrl Pts',(50.0835265683621,-8.80271195759284,-21.8911929834901));
#28762=CARTESIAN_POINT('Ctrl Pts',(49.9417988849617,-8.50428205216071,-21.7855755183937));
#28763=CARTESIAN_POINT('Ctrl Pts',(50.0835265683621,-8.59771167170023,-21.7646585258391));
#28764=CARTESIAN_POINT('Ctrl Pts',(50.0835265683621,-8.75963242031947,-21.7103838361864));
#28765=CARTESIAN_POINT('Ctrl Pts',(49.9736469154798,-8.46983068145907,-21.6260364650812));
#28766=CARTESIAN_POINT('Ctrl Pts',(50.0835265683621,-8.55674861132668,-21.5913570283804));
#28767=CARTESIAN_POINT('Ctrl Pts',(50.0835265683621,-8.69080155057987,-21.5378711661598));
#28768=CARTESIAN_POINT('Origin',(49.7710265683621,-8.69080155057986,-21.5378711661598));
#28769=CARTESIAN_POINT('Origin',(-44.291473431638,-8.87385981233827,-44.2925682080606));
#28770=CARTESIAN_POINT('Origin',(-49.603973431638,-8.87385981233827,-44.2925682080605));
#28771=CARTESIAN_POINT('Origin',(-39.4190920287328,-8.24885981233827,-37.6524198521891));
#28772=CARTESIAN_POINT('Origin',(-39.4190920287328,-8.24885981233827,-37.6524198521891));
#28773=CARTESIAN_POINT('Origin',(-39.4190920287328,-8.24885981233827,-37.6524198521891));
#28774=CARTESIAN_POINT('Origin',(-36.1446456971179,11.9341984494201,-34.3779735205741));
#28775=CARTESIAN_POINT('Origin',(-36.1446456971179,11.9341984494201,-34.3779735205741));
#28776=CARTESIAN_POINT('Origin',(-36.1446456971179,11.9341984494202,-34.3779735205741));
#28777=CARTESIAN_POINT('Ctrl Pts',(-49.8216584885785,13.0346110567825,8.78606179499422));
#28778=CARTESIAN_POINT('Ctrl Pts',(-49.9164734316379,13.1253379748597,8.77047400656095));
#28779=CARTESIAN_POINT('Ctrl Pts',(-49.916473431638,13.2555819259033,8.74809679815786));
#28780=CARTESIAN_POINT('Ctrl Pts',(-49.7894532167015,13.0670184804049,9.15934519252001));
#28781=CARTESIAN_POINT('Ctrl Pts',(-49.916473431638,13.1643191174741,9.15848213009695));
#28782=CARTESIAN_POINT('Ctrl Pts',(-49.916473431638,13.3203828042259,9.12526288252385));
#28783=CARTESIAN_POINT('Ctrl Pts',(-49.7551177481173,13.088519705192,9.53398887086785));
#28784=CARTESIAN_POINT('Ctrl Pts',(-49.9164734316379,13.1804336598305,9.5402420372352));
#28785=CARTESIAN_POINT('Ctrl Pts',(-49.916473431638,13.3633992223637,9.50504709953018));
#28786=CARTESIAN_POINT('Ctrl Pts',(-49.6823684168004,13.1183169307006,10.2839878772905));
#28787=CARTESIAN_POINT('Ctrl Pts',(-49.9164734316379,13.1821517325915,10.2978163027309));
#28788=CARTESIAN_POINT('Ctrl Pts',(-49.916473431638,13.4229936740979,10.2676389228998));
#28789=CARTESIAN_POINT('Ctrl Pts',(-49.6440350899221,13.1261401876617,10.6584945866178));
#28790=CARTESIAN_POINT('Ctrl Pts',(-49.9164734316379,13.163800762876,10.6808172003725));
#28791=CARTESIAN_POINT('Ctrl Pts',(-49.916473431638,13.4386401852138,10.6496656657108));
#28792=CARTESIAN_POINT('Ctrl Pts',(-49.603973431638,13.1261401876617,11.0309447204206));
#28793=CARTESIAN_POINT('Ctrl Pts',(-49.9164734316379,13.1261401876617,11.0309447204206));
#28794=CARTESIAN_POINT('Ctrl Pts',(-49.916473431638,13.4386401876617,11.0309447204206));
#28795=CARTESIAN_POINT('Ctrl Pts',(-49.603973431638,13.1261401876617,11.0309447204206));
#28796=CARTESIAN_POINT('Ctrl Pts',(-49.6302329959052,13.1261401876617,10.7868115855527));
#28797=CARTESIAN_POINT('Ctrl Pts',(-49.6556610339887,13.122783140923,10.5426318837783));
#28798=CARTESIAN_POINT('Ctrl Pts',(-49.6802470100602,13.1163230256676,10.2984481491949));
#28799=CARTESIAN_POINT('Ctrl Pts',(-49.6933181003556,13.1128885169226,10.1686283025428));
#28800=CARTESIAN_POINT('Ctrl Pts',(-49.7061510505488,13.1085760632363,10.0388069024177));
#28801=CARTESIAN_POINT('Ctrl Pts',(-49.7187432740471,13.1034183933663,9.90898836818533));
#28802=CARTESIAN_POINT('Ctrl Pts',(-49.7187724051985,13.1034064614893,9.90868804287966));
#28803=CARTESIAN_POINT('Ctrl Pts',(-49.7188015350095,13.1033945253904,9.90838771813324));
#28804=CARTESIAN_POINT('Ctrl Pts',(-49.7188306634802,13.1033825850675,9.90808739394585));
#28805=CARTESIAN_POINT('Ctrl Pts',(-49.7442104734438,13.0929789105763,9.64641314126808));
#28806=CARTESIAN_POINT('Ctrl Pts',(-49.768605180415,13.0793591824316,9.3848393250672));
#28807=CARTESIAN_POINT('Ctrl Pts',(-49.7920029933405,13.0610261308093,9.12345253841242));
#28808=CARTESIAN_POINT('Ctrl Pts',(-49.8020734013628,13.0531355937442,9.01095178453317));
#28809=CARTESIAN_POINT('Ctrl Pts',(-49.8119590386648,13.0443713918135,8.89848574803371));
#28810=CARTESIAN_POINT('Ctrl Pts',(-49.8216584885785,13.0346110567825,8.78606179499422));
#28811=CARTESIAN_POINT('Origin',(-49.603973431638,13.4386401876617,11.0309447204206));
#28812=CARTESIAN_POINT('Origin',(44.4585265683621,13.4386401876617,44.4574317919394));
#28813=CARTESIAN_POINT('Origin',(44.458526568362,13.4386401876617,49.7699317919394));
#28814=CARTESIAN_POINT('Origin',(36.9337491106657,12.8136401876617,35.1648873812767));
#28815=CARTESIAN_POINT('Origin',(36.9337491106657,12.8136401876617,35.1648873812767));
#28816=CARTESIAN_POINT('Origin',(36.311698833842,-3.61941807409668,34.542837104453));
#28817=CARTESIAN_POINT('Origin',(36.311698833842,-3.61941807409669,34.542837104453));
#28818=CARTESIAN_POINT('Ctrl Pts',(50.083526568362,-8.77420095969686,21.9109243621945));
#28819=CARTESIAN_POINT('Ctrl Pts',(50.0835265683628,-8.64003311578147,21.9648846044965));
#28820=CARTESIAN_POINT('Ctrl Pts',(49.9732908457536,-8.55319447590597,21.9998149860589));
#28821=CARTESIAN_POINT('Ctrl Pts',(50.083526568362,-7.36815837710381,18.4149889454167));
#28822=CARTESIAN_POINT('Ctrl Pts',(50.0835265683487,-7.24249091899859,18.4790048093049));
#28823=CARTESIAN_POINT('Ctrl Pts',(49.978533630732,-7.14715496494006,18.4919582423361));
#28824=CARTESIAN_POINT('Ctrl Pts',(50.083526568362,-6.21561709315083,14.8500215734068));
#28825=CARTESIAN_POINT('Ctrl Pts',(50.083526568362,-6.08656532686357,14.8994834481387));
#28826=CARTESIAN_POINT('Ctrl Pts',(49.9832519302634,-5.99460855897936,14.9133640755833));
#28827=CARTESIAN_POINT('Ctrl Pts',(50.083526568362,-5.02557369219655,9.39470188648604));
#28828=CARTESIAN_POINT('Ctrl Pts',(50.083526568362,-4.89581925233923,9.4215705380266));
#28829=CARTESIAN_POINT('Ctrl Pts',(49.9882943381249,-4.80456526664396,9.43549444587848));
#28830=CARTESIAN_POINT('Ctrl Pts',(50.083526568362,-4.71947214408127,7.57729337003443));
#28831=CARTESIAN_POINT('Ctrl Pts',(50.083526568362,-4.58961053625969,7.59830484628597));
#28832=CARTESIAN_POINT('Ctrl Pts',(49.98962859676,-4.49846371560897,7.61031203006756));
#28833=CARTESIAN_POINT('Ctrl Pts',(50.083526568362,-4.40691837826565,4.81133446982763));
#28834=CARTESIAN_POINT('Ctrl Pts',(50.083526568362,-4.27725721313452,4.82402565888155));
#28835=CARTESIAN_POINT('Ctrl Pts',(49.9910013573683,-4.18590981848534,4.83228563350366));
#28836=CARTESIAN_POINT('Ctrl Pts',(50.083526568362,-4.327158062246,3.88261941661919));
#28837=CARTESIAN_POINT('Ctrl Pts',(50.083526568362,-4.19755005842839,3.89271747614665));
#28838=CARTESIAN_POINT('Ctrl Pts',(49.991354395738,-4.10614946806195,3.89948067228241));
#28839=CARTESIAN_POINT('Ctrl Pts',(50.083526568362,-4.21946011836696,2.01146549461149));
#28840=CARTESIAN_POINT('Ctrl Pts',(50.0835265683621,-4.08996813963739,2.01670190226445));
#28841=CARTESIAN_POINT('Ctrl Pts',(49.9918319448095,-3.99845145937297,2.02004523691305));
#28842=CARTESIAN_POINT('Ctrl Pts',(50.0835265683621,-4.19205938565866,1.07822832045126));
#28843=CARTESIAN_POINT('Ctrl Pts',(50.0835265683621,-4.06258497561311,1.08082784046275));
#28844=CARTESIAN_POINT('Ctrl Pts',(49.9919540328468,-3.97105071507225,1.08265758398807));
#28845=CARTESIAN_POINT('Ctrl Pts',(50.0835265683621,-4.18598197768254,-3.57637494451022));
#28846=CARTESIAN_POINT('Ctrl Pts',(50.0835265683621,-4.05651422027729,-3.58583317976415));
#28847=CARTESIAN_POINT('Ctrl Pts',(49.9919810704912,-3.96497330343507,-3.59264920823258));
#28848=CARTESIAN_POINT('Ctrl Pts',(50.0835265683621,-4.60394036703586,-7.26265206407059));
#28849=CARTESIAN_POINT('Ctrl Pts',(50.0835265683621,-4.47650762043161,-7.29335381609307));
#28850=CARTESIAN_POINT('Ctrl Pts',(49.9900840020437,-4.3829309207017,-7.29528697694766));
#28851=CARTESIAN_POINT('Ctrl Pts',(50.0835265683621,-5.59091481619605,-11.8294033684595));
#28852=CARTESIAN_POINT('Ctrl Pts',(50.0835265683621,-5.46011080390277,-11.8606698601175));
#28853=CARTESIAN_POINT('Ctrl Pts',(49.9858981678965,-5.36990690683347,-11.8809489407712));
#28854=CARTESIAN_POINT('Ctrl Pts',(50.0835265683621,-5.81129472998664,-12.7400177061517));
#28855=CARTESIAN_POINT('Ctrl Pts',(50.0835265683589,-5.68032983291523,-12.773658914136));
#28856=CARTESIAN_POINT('Ctrl Pts',(49.9849733234776,-5.59028691905481,-12.7952664392488));
#28857=CARTESIAN_POINT('Ctrl Pts',(50.0835265683621,-6.29050753231155,-14.5401449456062));
#28858=CARTESIAN_POINT('Ctrl Pts',(50.0835265683654,-6.1590477277283,-14.5781843601422));
#28859=CARTESIAN_POINT('Ctrl Pts',(49.9829924585474,-6.06949999371107,-14.6025645997302));
#28860=CARTESIAN_POINT('Ctrl Pts',(50.0835265683621,-6.54980455615391,-15.4319492256746));
#28861=CARTESIAN_POINT('Ctrl Pts',(50.0835265683621,-6.41814737484765,-15.4722310008318));
#28862=CARTESIAN_POINT('Ctrl Pts',(49.9819344820143,-6.32879713521657,-15.497846160778));
#28863=CARTESIAN_POINT('Ctrl Pts',(50.0835265683621,-7.38126084278977,-18.0848938426664));
#28864=CARTESIAN_POINT('Ctrl Pts',(50.0835265683621,-7.24964619596978,-18.1343252734394));
#28865=CARTESIAN_POINT('Ctrl Pts',(49.9785987949462,-7.16025352121745,-18.1608944343837));
#28866=CARTESIAN_POINT('Ctrl Pts',(50.0835265683621,-8.0068345148146,-19.8236276697884));
#28867=CARTESIAN_POINT('Ctrl Pts',(50.0835265683621,-7.87510646586731,-19.8775490251741));
#28868=CARTESIAN_POINT('Ctrl Pts',(49.9761607637979,-7.78582757943672,-19.9059274936949));
#28869=CARTESIAN_POINT('Ctrl Pts',(50.0835265683621,-8.69080155057986,-21.5378711661598));
#28870=CARTESIAN_POINT('Ctrl Pts',(50.0835265683621,-8.55671560258686,-21.5913701985572));
#28871=CARTESIAN_POINT('Ctrl Pts',(49.9736023144971,-8.46979540751197,-21.6260505390544));
#28872=CARTESIAN_POINT('Origin',(49.771026568362,-8.69080155057986,21.702734750039));
#28873=CARTESIAN_POINT('Origin',(-49.603973431638,-8.87385981233827,0.0824317919394229));
#28874=CARTESIAN_POINT('Origin',(-49.603973431638,-8.87385981233827,-22.6228153633314));
#28875=CARTESIAN_POINT('Origin',(0.0835265683620477,-8.24885981233827,0.0824317919394229));
#28876=CARTESIAN_POINT('Ctrl Pts',(-49.8065937787538,-8.46983068146548,
-21.6260364650797));
#28877=CARTESIAN_POINT('Ctrl Pts',(-49.7945868225115,-8.48281912913915,
-21.6861839638978));
#28878=CARTESIAN_POINT('Ctrl Pts',(-49.7824920379308,-8.49383985403581,
-21.7465682311851));
#28879=CARTESIAN_POINT('Ctrl Pts',(-49.7703218005744,-8.50331222135076,
-21.8071274424854));
#28880=CARTESIAN_POINT('Ctrl Pts',(-49.7571156009582,-8.51359090121018,
-21.8728416113725));
#28881=CARTESIAN_POINT('Ctrl Pts',(-49.7438205451818,-8.52204613528895,
-21.9387618848257));
#28882=CARTESIAN_POINT('Ctrl Pts',(-49.7304472779566,-8.52915470825893,
-22.0048321176218));
#28883=CARTESIAN_POINT('Ctrl Pts',(-49.7228210345449,-8.53320844523035,
-22.042509348555));
#28884=CARTESIAN_POINT('Ctrl Pts',(-49.715169265573,-8.53682321976873,-22.0802357448589));
#28885=CARTESIAN_POINT('Ctrl Pts',(-49.707493320942,-8.5400806031776,-22.1180035325263));
#28886=CARTESIAN_POINT('Ctrl Pts',(-49.7072174179006,-8.54019768609479,
-22.119361052413));
#28887=CARTESIAN_POINT('Ctrl Pts',(-49.706941475036,-8.5403142598712,-22.1207186663251));
#28888=CARTESIAN_POINT('Ctrl Pts',(-49.7066654928968,-8.54043032524654,
-22.1220763716637));
#28889=CARTESIAN_POINT('Ctrl Pts',(-49.6933692202904,-8.54602212504574,
-22.1874879245738));
#28890=CARTESIAN_POINT('Ctrl Pts',(-49.680000075092,-8.55043067995626,-22.2530232013284));
#28891=CARTESIAN_POINT('Ctrl Pts',(-49.6665711482279,-8.5537415100254,-22.3186261411179));
#28892=CARTESIAN_POINT('Ctrl Pts',(-49.6531611054658,-8.55704768432024,
-22.3841368283679));
#28893=CARTESIAN_POINT('Ctrl Pts',(-49.6396908764539,-8.55925889971278,
-22.4497177613008));
#28894=CARTESIAN_POINT('Ctrl Pts',(-49.6261708648657,-8.56041391612595,
-22.5153164405566));
#28895=CARTESIAN_POINT('Ctrl Pts',(-49.6187858031651,-8.56104482294291,
-22.5511485321651));
#28896=CARTESIAN_POINT('Ctrl Pts',(-49.6113858916315,-8.56135981233827,
-22.586985736526));
#28897=CARTESIAN_POINT('Ctrl Pts',(-49.603973431638,-8.56135981233827,-22.6228153633314));
#28898=CARTESIAN_POINT('Ctrl Pts',(-39.198121159612,-8.24885981233822,-37.8733907213098));
#28899=CARTESIAN_POINT('Ctrl Pts',(-39.0443992301304,-8.46631238203731,
-37.7196687918282));
#28900=CARTESIAN_POINT('Ctrl Pts',(-39.259307713056,-8.46983068145902,-37.4997859848341));
#28901=CARTESIAN_POINT('Ctrl Pts',(-38.1066522799264,-6.70569384849083,
-36.7819218416243));
#28902=CARTESIAN_POINT('Ctrl Pts',(-37.9532471818597,-6.9233956438646,-36.6285167435576));
#28903=CARTESIAN_POINT('Ctrl Pts',(-38.1677401528067,-6.92666471828269,
-36.408420409565));
#28904=CARTESIAN_POINT('Ctrl Pts',(-37.0151713871357,-5.16254485804652,
-35.6904409488335));
#28905=CARTESIAN_POINT('Ctrl Pts',(-36.8618908744034,-5.38020745678985,
-35.5371604361543));
#28906=CARTESIAN_POINT('Ctrl Pts',(-37.0761523844306,-5.38351572788263,
-35.3170515943614));
#28907=CARTESIAN_POINT('Ctrl Pts',(-35.9236748279971,-3.61941807409667,
-34.5989443896949));
#28908=CARTESIAN_POINT('Ctrl Pts',(-35.7701869713603,-3.83655054711528,
-34.4454565330581));
#28909=CARTESIAN_POINT('Ctrl Pts',(-35.9845382828747,-3.84038894321746,
-34.2256786063309));
#28910=CARTESIAN_POINT('Origin',(-36.1446456971179,-3.61941807409669,-34.3779735205741));
#28911=CARTESIAN_POINT('Origin',(-36.1446456971179,11.4830954176946,-34.3779735205741));
#28912=CARTESIAN_POINT('Origin',(-36.1446456971179,-3.61941807409668,-34.3779735205741));
#28913=CARTESIAN_POINT('Origin',(0.0835265683620477,11.9341984494201,0.0824317919394229));
#28914=CARTESIAN_POINT('Origin',(-36.1446456971182,11.9341984494201,34.5428371044526));
#28915=CARTESIAN_POINT('Origin',(-36.4556711145887,12.3739187291526,34.8538627965404));
#28916=CARTESIAN_POINT('Origin',(-36.7666959739419,12.8136401876617,35.1648873812763));
#28917=CARTESIAN_POINT('Origin',(-36.1446456971182,11.9341984494202,34.5428371044526));
#28918=CARTESIAN_POINT('Origin',(0.0835265683620477,12.8136401876617,0.0824317919394229));
#28919=CARTESIAN_POINT('Origin',(-36.7666959739419,12.8136401876617,35.1648873812763));
#28920=CARTESIAN_POINT('Origin',(-49.603973431638,13.4386401876617,0.0824317919394229));
#28921=CARTESIAN_POINT('Origin',(-49.603973431638,13.4386401876617,44.4574317919389));
#28922=CARTESIAN_POINT('Origin',(0.0835265683620476,13.4386401876617,49.7699317919394));
#28923=CARTESIAN_POINT('Origin',(11.0320394968433,13.4386401876617,49.7699317919394));
#28924=CARTESIAN_POINT('Origin',(26.3424100448452,12.8136401876617,24.5735483154562));
#28925=CARTESIAN_POINT('Ctrl Pts',(39.3651742963362,-8.24885981233836,38.0382543051888));
#28926=CARTESIAN_POINT('Ctrl Pts',(39.2114523668546,-8.46631238203745,37.8845323757072));
#28927=CARTESIAN_POINT('Ctrl Pts',(39.4263608497802,-8.46983068145916,37.6646495687131));
#28928=CARTESIAN_POINT('Ctrl Pts',(38.2737054166549,-6.70569384848682,36.9467854255075));
#28929=CARTESIAN_POINT('Ctrl Pts',(38.1203003185921,-6.92339564386061,36.7933803274371));
#28930=CARTESIAN_POINT('Ctrl Pts',(38.3347932895352,-6.92666471828384,36.5732839934409));
#28931=CARTESIAN_POINT('Ctrl Pts',(37.1822245238622,-5.16254485804367,35.8553045327148));
#28932=CARTESIAN_POINT('Ctrl Pts',(37.0289440111306,-5.38020745678604,35.7020240200362));
#28933=CARTESIAN_POINT('Ctrl Pts',(37.2432055211549,-5.38351572788296,35.4819151782406));
#28934=CARTESIAN_POINT('Ctrl Pts',(36.0907279647212,-3.61941807409668,34.7638079735738));
#28935=CARTESIAN_POINT('Ctrl Pts',(35.9372401080844,-3.83655054711529,34.610320116937));
#28936=CARTESIAN_POINT('Ctrl Pts',(36.1515914195988,-3.84038894321748,34.3905421902098));
#28937=CARTESIAN_POINT('Origin',(39.5861451654569,-8.24885981233827,37.8172834360679));
#28938=CARTESIAN_POINT('Origin',(0.0835265683620477,-8.24885981233827,0.0824317919394229));
#28939=CARTESIAN_POINT('Ctrl Pts',(49.9736469154778,-8.46983068146547,21.7909000489587));
#28940=CARTESIAN_POINT('Ctrl Pts',(49.9616399592362,-8.48281912913843,21.8510475477735));
#28941=CARTESIAN_POINT('Ctrl Pts',(49.949545174656,-8.4938398540346,21.9114318150575));
#28942=CARTESIAN_POINT('Ctrl Pts',(49.9373749373003,-8.50331222134921,21.9719910263544));
#28943=CARTESIAN_POINT('Ctrl Pts',(49.9241687376785,-8.51359090121315,22.0377051952691));
#28944=CARTESIAN_POINT('Ctrl Pts',(49.9108736818965,-8.52204613529488,22.1036254687501));
#28945=CARTESIAN_POINT('Ctrl Pts',(49.8975004146657,-8.52915470826684,22.1696957015741));
#28946=CARTESIAN_POINT('Ctrl Pts',(49.8898741712589,-8.53320844523506,22.2073729324829));
#28947=CARTESIAN_POINT('Ctrl Pts',(49.882222402292,-8.53682321977086,22.2450993287624));
#28948=CARTESIAN_POINT('Ctrl Pts',(49.8745464576661,-8.54008060317762,22.2828671164053));
#28949=CARTESIAN_POINT('Ctrl Pts',(49.8742705546247,-8.54019768609482,22.284224636292));
#28950=CARTESIAN_POINT('Ctrl Pts',(49.8739946117601,-8.54031425987122,22.2855822502041));
#28951=CARTESIAN_POINT('Ctrl Pts',(49.8737186296209,-8.54043032524656,22.2869399555427));
#28952=CARTESIAN_POINT('Ctrl Pts',(49.8604223570134,-8.54602212504619,22.3523515084577));
#28953=CARTESIAN_POINT('Ctrl Pts',(49.8470532118141,-8.55043067995696,22.4178867852175));
#28954=CARTESIAN_POINT('Ctrl Pts',(49.8336242849491,-8.55374151002619,22.4834897250119));
#28955=CARTESIAN_POINT('Ctrl Pts',(49.820214242186,-8.55704768432111,22.5490004122671));
#28956=CARTESIAN_POINT('Ctrl Pts',(49.806744013173,-8.55925889971357,22.6145813452051));
#28957=CARTESIAN_POINT('Ctrl Pts',(49.7932240015836,-8.5604139161265,22.6801800244661));
#28958=CARTESIAN_POINT('Ctrl Pts',(49.7858389398851,-8.5610448229431,22.7160121160645));
#28959=CARTESIAN_POINT('Ctrl Pts',(49.7784390283535,-8.56135981233827,22.7518493204152));
#28960=CARTESIAN_POINT('Ctrl Pts',(49.771026568362,-8.56135981233827,22.7876789472104));
#28961=CARTESIAN_POINT('Origin',(39.5861451654569,-8.24885981233827,37.8172834360679));
#28962=CARTESIAN_POINT('Ctrl Pts',(50.083526568362,-8.87385981233827,22.7876789472104));
#28963=CARTESIAN_POINT('Ctrl Pts',(50.083526568362,-8.56135981233826,22.7876789472104));
#28964=CARTESIAN_POINT('Ctrl Pts',(49.771026568362,-8.56135981233827,22.7876789472104));
#28965=CARTESIAN_POINT('Ctrl Pts',(50.083526568362,-8.87385981115686,22.6049484969869));
#28966=CARTESIAN_POINT('Ctrl Pts',(50.083526568362,-8.59410214473078,22.6294121895504));
#28967=CARTESIAN_POINT('Ctrl Pts',(49.8055639510575,-8.56135981233827,22.6207355122547));
#28968=CARTESIAN_POINT('Ctrl Pts',(50.083526568362,-8.86016990857478,22.4188549273494));
#28969=CARTESIAN_POINT('Ctrl Pts',(50.083526568362,-8.61269267441895,22.4526647591265));
#28970=CARTESIAN_POINT('Ctrl Pts',(49.8405324775689,-8.55451485837129,22.4502251675162));
#28971=CARTESIAN_POINT('Ctrl Pts',(50.083526568362,-8.80243256293661,22.0545662364126));
#28972=CARTESIAN_POINT('Ctrl Pts',(50.083526568362,-8.61241087733861,22.1043384740035));
#28973=CARTESIAN_POINT('Ctrl Pts',(49.9085599813632,-8.52564618972364,22.1155090903777));
#28974=CARTESIAN_POINT('Ctrl Pts',(50.083526568362,-8.75973143359955,21.8754956191941));
#28975=CARTESIAN_POINT('Ctrl Pts',(50.083526568362,-8.59777411058796,21.9297863271335));
#28976=CARTESIAN_POINT('Ctrl Pts',(49.9417488603592,-8.50433615796023,21.9506896748485));
#28977=CARTESIAN_POINT('Ctrl Pts',(50.083526568362,-8.69080155058829,21.7027347500381));
#28978=CARTESIAN_POINT('Ctrl Pts',(50.083526568362,-8.55674861133339,21.7562206122583));
#28979=CARTESIAN_POINT('Ctrl Pts',(49.9736469154778,-8.46983068146547,21.7909000489587));
#28980=CARTESIAN_POINT('Origin',(49.771026568362,-8.87385981233827,22.7876789472104));
#28981=CARTESIAN_POINT('Ctrl Pts',(-49.916473431638,-8.87385981233827,-22.6228153633314));
#28982=CARTESIAN_POINT('Ctrl Pts',(-49.9164734316379,-8.56135981233827,
-22.6228153633314));
#28983=CARTESIAN_POINT('Ctrl Pts',(-49.603973431638,-8.56135981233827,-22.6228153633314));
#28984=CARTESIAN_POINT('Ctrl Pts',(-49.916473431638,-8.87385981115686,-22.4400849131078));
#28985=CARTESIAN_POINT('Ctrl Pts',(-49.916473431638,-8.59410214473059,-22.4645486056717));
#28986=CARTESIAN_POINT('Ctrl Pts',(-49.638510814333,-8.56135981233827,-22.4558719283758));
#28987=CARTESIAN_POINT('Ctrl Pts',(-49.916473431638,-8.86016990857445,-22.2539913434704));
#28988=CARTESIAN_POINT('Ctrl Pts',(-49.9164734316379,-8.61269267441878,
-22.2878011752468));
#28989=CARTESIAN_POINT('Ctrl Pts',(-49.6734793408449,-8.55451485837122,
-22.2853615836368));
#28990=CARTESIAN_POINT('Ctrl Pts',(-49.916473431638,-8.80243256293692,-21.8897026525336));
#28991=CARTESIAN_POINT('Ctrl Pts',(-49.9164734316379,-8.61241087733876,
-21.9394748901251));
#28992=CARTESIAN_POINT('Ctrl Pts',(-49.7415068446392,-8.5256461897237,-21.950645506499));
#28993=CARTESIAN_POINT('Ctrl Pts',(-49.916473431638,-8.75973143359542,-21.7106320353166));
#28994=CARTESIAN_POINT('Ctrl Pts',(-49.9164734316379,-8.59777411058377,
-21.764922743255));
#28995=CARTESIAN_POINT('Ctrl Pts',(-49.7746957236346,-8.5043361579596,-21.7858260909692));
#28996=CARTESIAN_POINT('Ctrl Pts',(-49.916473431638,-8.6908015505883,-21.5378711661591));
#28997=CARTESIAN_POINT('Ctrl Pts',(-49.916473431638,-8.5567486113334,-21.5913570283793));
#28998=CARTESIAN_POINT('Ctrl Pts',(-49.8065937787538,-8.46983068146548,
-21.6260364650797));
#28999=CARTESIAN_POINT('Origin',(-49.603973431638,-8.69080155057987,-21.5378711661599));
#29000=CARTESIAN_POINT('Origin',(-36.1446456971179,-3.61941807409668,-34.3779735205741));
#29001=CARTESIAN_POINT('Origin',(-36.1446456971179,-3.61941807409668,-34.3779735205741));
#29002=CARTESIAN_POINT('Origin',(-36.1446456971182,11.9341984494201,34.5428371044526));
#29003=CARTESIAN_POINT('Origin',(-36.1446456971182,11.9341984494201,34.5428371044526));
#29004=CARTESIAN_POINT('Origin',(-36.7666959739419,12.8136401876617,35.1648873812763));
#29005=CARTESIAN_POINT('Origin',(-36.7666959739419,12.8136401876617,35.1648873812763));
#29006=CARTESIAN_POINT('Origin',(-44.2914734316384,13.4386401876617,44.457431791939));
#29007=CARTESIAN_POINT('Origin',(-44.2914734316384,13.4386401876617,49.769931791939));
#29008=CARTESIAN_POINT('Ctrl Pts',(8.7871565714169,13.0346110567825,49.98761684888));
#29009=CARTESIAN_POINT('Ctrl Pts',(8.77156878298363,13.1253379748597,50.0824317919394));
#29010=CARTESIAN_POINT('Ctrl Pts',(8.74919157458054,13.2555819259033,50.0824317919394));
#29011=CARTESIAN_POINT('Ctrl Pts',(9.16043996894276,13.0670184804062,49.9554115770043));
#29012=CARTESIAN_POINT('Ctrl Pts',(9.15957690651951,13.1643191174805,50.0824317919394));
#29013=CARTESIAN_POINT('Ctrl Pts',(9.12635765894441,13.3203828042395,50.0824317919394));
#29014=CARTESIAN_POINT('Ctrl Pts',(9.53508364729048,13.0885197051924,49.9210761084199));
#29015=CARTESIAN_POINT('Ctrl Pts',(9.54133681365794,13.1804336598308,50.0824317919394));
#29016=CARTESIAN_POINT('Ctrl Pts',(9.50614187595252,13.3633992223637,50.0824317919394));
#29017=CARTESIAN_POINT('Ctrl Pts',(10.2850826537132,13.1183169307001,49.8483267771008));
#29018=CARTESIAN_POINT('Ctrl Pts',(10.2989110791544,13.1821517325912,50.0824317919394));
#29019=CARTESIAN_POINT('Ctrl Pts',(10.2687336993228,13.4229936740979,50.0824317919394));
#29020=CARTESIAN_POINT('Ctrl Pts',(10.6595893630408,13.1261401876617,49.8099934502275));
#29021=CARTESIAN_POINT('Ctrl Pts',(10.6819119767957,13.1638007628797,50.0824317919394));
#29022=CARTESIAN_POINT('Ctrl Pts',(10.6507604421332,13.4386401852138,50.0824317919394));
#29023=CARTESIAN_POINT('Ctrl Pts',(11.0320394968433,13.1261401876617,49.7699317919394));
#29024=CARTESIAN_POINT('Ctrl Pts',(11.0320394968433,13.1261401876617,50.0824317919394));
#29025=CARTESIAN_POINT('Ctrl Pts',(11.0320394968433,13.4386401876617,50.0824317919394));
#29026=CARTESIAN_POINT('Origin',(8.74919157458055,13.2555819259033,49.7699317919394));
#29027=CARTESIAN_POINT('Ctrl Pts',(11.0320394968433,13.1261401876617,49.7699317919394));
#29028=CARTESIAN_POINT('Ctrl Pts',(10.7879063626455,13.1261401876617,49.7961913561371));
#29029=CARTESIAN_POINT('Ctrl Pts',(10.5437266615415,13.1227831409413,49.8216193941525));
#29030=CARTESIAN_POINT('Ctrl Pts',(10.2995429276285,13.1163230257208,49.8462053701604));
#29031=CARTESIAN_POINT('Ctrl Pts',(10.1697230803061,13.1128885169672,49.8592764605253));
#29032=CARTESIAN_POINT('Ctrl Pts',(10.0399016795106,13.1085760632631,49.8721094107857));
#29033=CARTESIAN_POINT('Ctrl Pts',(9.91008314460798,13.1034183933665,49.8847016343491));
#29034=CARTESIAN_POINT('Ctrl Pts',(9.9097828193023,13.1034064614895,49.8847307655005));
#29035=CARTESIAN_POINT('Ctrl Pts',(9.90948249455588,13.1033945253906,49.8847598953115));
#29036=CARTESIAN_POINT('Ctrl Pts',(9.90918217036849,13.1033825850677,49.8847890237822));
#29037=CARTESIAN_POINT('Ctrl Pts',(9.64750791812301,13.0929789105939,49.9101688337043));
#29038=CARTESIAN_POINT('Ctrl Pts',(9.38593410235409,13.0793591824768,49.9345635406361));
#29039=CARTESIAN_POINT('Ctrl Pts',(9.12454731613055,13.0610261309002,49.9579613535261));
#29040=CARTESIAN_POINT('Ctrl Pts',(9.01204656181922,13.0531355938115,49.9680317615884));
#29041=CARTESIAN_POINT('Ctrl Pts',(8.89958052488792,13.044371391851,49.977917398929));
#29042=CARTESIAN_POINT('Ctrl Pts',(8.7871565714169,13.0346110567825,49.98761684888));
#29043=CARTESIAN_POINT('Origin',(39.5861451654569,-8.24885981233827,37.8172834360679));
#29044=CARTESIAN_POINT('Origin',(39.5861451654569,-8.24885981233827,37.8172834360679));
#29045=CARTESIAN_POINT('Origin',(49.7710265683621,-8.87385981233827,0.0824317919395964));
#29046=CARTESIAN_POINT('Origin',(49.7710265683619,-8.87385981233827,36.6697170232579));
#29047=CARTESIAN_POINT('Ctrl Pts',(-49.806390285198,-8.51742571162867,21.9103807300632));
#29048=CARTESIAN_POINT('Ctrl Pts',(-49.9164734316379,-8.60429852763446,
21.8755587571809));
#29049=CARTESIAN_POINT('Ctrl Pts',(-49.916473431638,-8.73841680848988,21.821799675756));
#29050=CARTESIAN_POINT('Ctrl Pts',(-49.8090085275553,-7.81611845087935,
20.1547534124056));
#29051=CARTESIAN_POINT('Ctrl Pts',(-49.9164734316379,-7.905452447202,20.1264636503561));
#29052=CARTESIAN_POINT('Ctrl Pts',(-49.916473431638,-8.03710989934276,20.0721563037169));
#29053=CARTESIAN_POINT('Ctrl Pts',(-49.811505080355,-7.17497856296609,18.3722381388645));
#29054=CARTESIAN_POINT('Ctrl Pts',(-49.916473431638,-7.26440945854389,18.3457771808587));
#29055=CARTESIAN_POINT('Ctrl Pts',(-49.916473431638,-7.39597034001919,18.2960666122331));
#29056=CARTESIAN_POINT('Ctrl Pts',(-49.8148908786805,-6.33083548943257,
15.6694891089486));
#29057=CARTESIAN_POINT('Ctrl Pts',(-49.916473431638,-6.42018164708939,15.643863548684));
#29058=CARTESIAN_POINT('Ctrl Pts',(-49.916473431638,-6.55182731464684,15.6035705286288));
#29059=CARTESIAN_POINT('Ctrl Pts',(-49.8159488661239,-6.07147275224007,
14.7743893106039));
#29060=CARTESIAN_POINT('Ctrl Pts',(-49.9164734316379,-6.1610167959071,14.7499995971314));
#29061=CARTESIAN_POINT('Ctrl Pts',(-49.916473431638,-6.29246464497438,14.7119466567203));
#29062=CARTESIAN_POINT('Ctrl Pts',(-49.8179305761161,-5.59194595832842,
12.9667362137106));
#29063=CARTESIAN_POINT('Ctrl Pts',(-49.9164734316379,-5.68198529154953,
12.9451192661143));
#29064=CARTESIAN_POINT('Ctrl Pts',(-49.916473431638,-5.81293800731357,12.9114646652259));
#29065=CARTESIAN_POINT('Ctrl Pts',(-49.818851928498,-5.37235566849251,12.0558730479342));
#29066=CARTESIAN_POINT('Ctrl Pts',(-49.9164734316379,-5.46255331592529,
12.0355704304617));
#29067=CARTESIAN_POINT('Ctrl Pts',(-49.916473431638,-5.5933477731877,12.0042902846947));
#29068=CARTESIAN_POINT('Ctrl Pts',(-49.8230168203026,-4.39003165639685,
7.49797183341572));
#29069=CARTESIAN_POINT('Ctrl Pts',(-49.916473431638,-4.48357391698338,7.49584681502986));
#29070=CARTESIAN_POINT('Ctrl Pts',(-49.916473431638,-4.6110246353903,7.46517834582782));
#29071=CARTESIAN_POINT('Ctrl Pts',(-49.8249248580392,-3.9693070073482,3.81016121038314));
#29072=CARTESIAN_POINT('Ctrl Pts',(-49.916473431638,-4.0608403985703,3.8033166949147));
#29073=CARTESIAN_POINT('Ctrl Pts',(-49.916473431638,-4.19029955013506,3.79365499210425));
#29074=CARTESIAN_POINT('Ctrl Pts',(-49.8249220643427,-3.96993507524447,
-0.857931554581411));
#29075=CARTESIAN_POINT('Ctrl Pts',(-49.916473431638,-4.06146778743525,-0.85620740371108));
#29076=CARTESIAN_POINT('Ctrl Pts',(-49.916473431638,-4.19092761786416,-0.853767668538309));
#29077=CARTESIAN_POINT('Ctrl Pts',(-49.8248043537542,-3.99635691345978,
-1.79721876196628));
#29078=CARTESIAN_POINT('Ctrl Pts',(-49.9164734316379,-4.08787247118437,
-1.793974725638));
#29079=CARTESIAN_POINT('Ctrl Pts',(-49.916473431638,-4.21734944964593,-1.78889590701665));
#29080=CARTESIAN_POINT('Ctrl Pts',(-49.8243398235277,-4.10112063979829,
-3.66632558149043));
#29081=CARTESIAN_POINT('Ctrl Pts',(-49.916473431638,-4.19252330504738,-3.65967940853563));
#29082=CARTESIAN_POINT('Ctrl Pts',(-49.916473431638,-4.32211313978211,-3.64976555244737));
#29083=CARTESIAN_POINT('Ctrl Pts',(-49.8239941455949,-4.17921237910952,
-4.59529073762686));
#29084=CARTESIAN_POINT('Ctrl Pts',(-49.916473431638,-4.270562939551,-4.58715350637057));
#29085=CARTESIAN_POINT('Ctrl Pts',(-49.916473431638,-4.40020485981034,-4.57465641978639));
#29086=CARTESIAN_POINT('Ctrl Pts',(-49.8226424366985,-4.48691998515858,
-7.36617052593359));
#29087=CARTESIAN_POINT('Ctrl Pts',(-49.916473431638,-4.57807108938205,-7.3542734158373));
#29088=CARTESIAN_POINT('Ctrl Pts',(-49.916473431638,-4.7079123912234,-7.33349441387557));
#29089=CARTESIAN_POINT('Ctrl Pts',(-49.8213206429539,-4.79002518529142,
-9.19205418037808));
#29090=CARTESIAN_POINT('Ctrl Pts',(-49.9164734316379,-4.88128811498848,
-9.17826244785312));
#29091=CARTESIAN_POINT('Ctrl Pts',(-49.916473431638,-5.01101759107685,-9.15159463779479));
#29092=CARTESIAN_POINT('Ctrl Pts',(-49.8180136507671,-5.57013492024956,
-12.8056466912206));
#29093=CARTESIAN_POINT('Ctrl Pts',(-49.916473431638,-5.66058104929807,-12.7859604123856));
#29094=CARTESIAN_POINT('Ctrl Pts',(-49.916473431638,-5.79112706648838,-12.7502963145487));
#29095=CARTESIAN_POINT('Ctrl Pts',(-49.8160298017131,-6.04706234041287,
-14.5933718646951));
#29096=CARTESIAN_POINT('Ctrl Pts',(-49.916473431638,-6.13757065813332,-14.5718489152074));
#29097=CARTESIAN_POINT('Ctrl Pts',(-49.916473431638,-6.26805446129722,-14.5309143455853));
#29098=CARTESIAN_POINT('Ctrl Pts',(-49.8115462443468,-7.16453247036129,
-18.1766274992858));
#29099=CARTESIAN_POINT('Ctrl Pts',(-49.916473431638,-7.25396587946009,-18.1501885883301));
#29100=CARTESIAN_POINT('Ctrl Pts',(-49.916473431638,-7.3855242488532,-18.1005692862277));
#29101=CARTESIAN_POINT('Ctrl Pts',(-49.8090319587906,-7.80982710888312,
-19.9742784910252));
#29102=CARTESIAN_POINT('Ctrl Pts',(-49.916473431638,-7.89920232384119,-19.9460959591859));
#29103=CARTESIAN_POINT('Ctrl Pts',(-49.916473431638,-8.03081819453224,-19.8917334283858));
#29104=CARTESIAN_POINT('Ctrl Pts',(-49.8063885873382,-8.51788060322345,
-21.7466537855478));
#29105=CARTESIAN_POINT('Ctrl Pts',(-49.916473431638,-8.60475296695841,-21.7118303962669));
#29106=CARTESIAN_POINT('Ctrl Pts',(-49.916473431638,-8.73887172590212,-21.6580689256479));
#29107=CARTESIAN_POINT('Origin',(-49.603973431638,-8.69080155057986,21.7027347500388));
#29108=CARTESIAN_POINT('Origin',(0.0835265683620477,-3.61941807409668,0.0824317919394229));
#29109=CARTESIAN_POINT('Origin',(-36.1446456971182,-3.61941807409668,34.5428371044526));
#29110=CARTESIAN_POINT('Origin',(-36.1446456971182,11.4830954176946,34.5428371044526));
#29111=CARTESIAN_POINT('Origin',(-36.1446456971182,-3.61941807409669,34.5428371044526));
#29112=CARTESIAN_POINT('Origin',(-26.1753569081214,12.8136401876617,24.573548315456));
#29113=CARTESIAN_POINT('Origin',(0.0835265683620476,13.4386401876617,49.7699317919394));
#29114=CARTESIAN_POINT('Origin',(-10.8649863601191,13.4386401876617,49.7699317919394));
#29115=CARTESIAN_POINT('Ctrl Pts',(-8.62010343469276,13.0346110567825,49.98761684888));
#29116=CARTESIAN_POINT('Ctrl Pts',(-8.60451564625949,13.1253379748597,50.0824317919394));
#29117=CARTESIAN_POINT('Ctrl Pts',(-8.58213843785641,13.2555819259033,50.0824317919394));
#29118=CARTESIAN_POINT('Ctrl Pts',(-5.74966049737118,12.5435283274364,49.9897363306993));
#29119=CARTESIAN_POINT('Ctrl Pts',(-5.74470440235702,12.6357570952065,50.0824317919394));
#29120=CARTESIAN_POINT('Ctrl Pts',(-5.72384185377314,12.7644980954123,50.0824317919394));
#29121=CARTESIAN_POINT('Ctrl Pts',(-2.85305802790577,12.2852858973025,49.9908996598662));
#29122=CARTESIAN_POINT('Ctrl Pts',(-2.84768070573019,12.3768143018313,50.0824317919394));
#29123=CARTESIAN_POINT('Ctrl Pts',(-2.84005623507672,12.5062567663872,50.0824317919394));
#29124=CARTESIAN_POINT('Ctrl Pts',(1.53450453635747,12.2842756298963,49.9909041527923));
#29125=CARTESIAN_POINT('Ctrl Pts',(1.53184148134384,12.3758051232163,50.0824317919394));
#29126=CARTESIAN_POINT('Ctrl Pts',(1.52808029952419,12.5052464990352,50.0824317919394));
#29127=CARTESIAN_POINT('Ctrl Pts',(3.00840305743394,12.3489547591764,49.9906154596787));
#29128=CARTESIAN_POINT('Ctrl Pts',(3.00380039949013,12.4404805872018,50.0824317919394));
#29129=CARTESIAN_POINT('Ctrl Pts',(2.99545364886012,12.5699256283378,50.0824317919394));
#29130=CARTESIAN_POINT('Ctrl Pts',(5.91737315216722,12.6021248598315,49.9894981615007));
#29131=CARTESIAN_POINT('Ctrl Pts',(5.90753279762978,12.6933787936176,50.0824317919394));
#29132=CARTESIAN_POINT('Ctrl Pts',(5.89169090718009,12.8230957289117,50.0824317919394));
#29133=CARTESIAN_POINT('Ctrl Pts',(7.35844722659859,12.7901838029052,49.9886717813281));
#29134=CARTESIAN_POINT('Ctrl Pts',(7.34671603317829,12.8814125534449,50.0824317919394));
#29135=CARTESIAN_POINT('Ctrl Pts',(7.32653049920342,13.0111545790419,50.0824317919394));
#29136=CARTESIAN_POINT('Ctrl Pts',(8.7871565714169,13.0346110567825,49.98761684888));
#29137=CARTESIAN_POINT('Ctrl Pts',(8.77156878298363,13.1253379748597,50.0824317919394));
#29138=CARTESIAN_POINT('Ctrl Pts',(8.74919157458054,13.2555819259033,50.0824317919394));
#29139=CARTESIAN_POINT('Origin',(-8.58213843785641,13.2555819259033,49.7699317919394));
#29140=CARTESIAN_POINT('Origin',(0.0835265683620477,12.8136401876617,0.0824317919394229));
#29141=CARTESIAN_POINT('Origin',(35.1659821576993,12.8136401876617,36.932654334243));
#29142=CARTESIAN_POINT('Origin',(24.5746430918789,12.8136401876617,26.3413152684227));
#29143=CARTESIAN_POINT('Origin',(35.1659821576993,12.8136401876617,36.932654334243));
#29144=CARTESIAN_POINT('Origin',(41.4050790939509,-8.24885981233827,39.6362173645619));
#29145=CARTESIAN_POINT('Origin',(40.7421664865885,-8.24885981233827,38.9733047571995));
#29146=CARTESIAN_POINT('Origin',(44.4585265683621,-8.87385981233827,44.4574317919394));
#29147=CARTESIAN_POINT('Origin',(44.458526568362,-8.87385981233827,49.7699317919394));
#29148=CARTESIAN_POINT('Ctrl Pts',(-49.603973431638,-8.56135981233827,22.7876789472102));
#29149=CARTESIAN_POINT('Ctrl Pts',(-49.9164734316379,-8.56135981233827,
22.7876789472102));
#29150=CARTESIAN_POINT('Ctrl Pts',(-49.916473431638,-8.87385981233827,22.7876789472102));
#29151=CARTESIAN_POINT('Ctrl Pts',(-49.6390045861426,-8.56135981233827,
22.6183487659333));
#29152=CARTESIAN_POINT('Ctrl Pts',(-49.916473431638,-8.59454828035616,22.6272556847667));
#29153=CARTESIAN_POINT('Ctrl Pts',(-49.916473431638,-8.87385980853143,22.6023407515994));
#29154=CARTESIAN_POINT('Ctrl Pts',(-49.6734801841997,-8.55449257599332,
22.4502169429184));
#29155=CARTESIAN_POINT('Ctrl Pts',(-49.916473431638,-8.61264419244186,22.4525914296835));
#29156=CARTESIAN_POINT('Ctrl Pts',(-49.916473431638,-8.86012534447556,22.4188473554127));
#29157=CARTESIAN_POINT('Ctrl Pts',(-49.7412291075803,-8.52578588737898,
22.1168796998391));
#29158=CARTESIAN_POINT('Ctrl Pts',(-49.916473431638,-8.61245644138859,22.1057145740718));
#29159=CARTESIAN_POINT('Ctrl Pts',(-49.916473431638,-8.80271195759251,22.0560565673691));
#29160=CARTESIAN_POINT('Ctrl Pts',(-49.7747457482377,-8.50428205216085,
21.9504391022727));
#29161=CARTESIAN_POINT('Ctrl Pts',(-49.916473431636,-8.59771167170006,21.9295221097184));
#29162=CARTESIAN_POINT('Ctrl Pts',(-49.916473431638,-8.75963242031971,21.8752474200655));
#29163=CARTESIAN_POINT('Ctrl Pts',(-49.8065937787556,-8.46983068145906,
21.7909000489602));
#29164=CARTESIAN_POINT('Ctrl Pts',(-49.916473431638,-8.55674861132667,21.7562206122594));
#29165=CARTESIAN_POINT('Ctrl Pts',(-49.916473431638,-8.69080155057985,21.7027347500388));
#29166=CARTESIAN_POINT('Origin',(-49.603973431638,-8.87385981233827,22.7876789472102));
#29167=CARTESIAN_POINT('Ctrl Pts',(-49.8065937787556,-8.46983068145906,
21.7909000489602));
#29168=CARTESIAN_POINT('Ctrl Pts',(-49.7963235078174,-8.48094048097799,
21.8423478177927));
#29169=CARTESIAN_POINT('Ctrl Pts',(-49.7859728826426,-8.49060780497133,
21.8940472511784));
#29170=CARTESIAN_POINT('Ctrl Pts',(-49.775563128702,-8.49910612137133,21.9458948974734));
#29171=CARTESIAN_POINT('Ctrl Pts',(-49.764379289321,-8.50823638575309,22.0015980151221));
#29172=CARTESIAN_POINT('Ctrl Pts',(-49.7531270731297,-8.51601690934008,
22.0574729005677));
#29173=CARTESIAN_POINT('Ctrl Pts',(-49.741824971166,-8.52273612856652,22.1134260010429));
#29174=CARTESIAN_POINT('Ctrl Pts',(-49.7303817060214,-8.52953927079792,
22.1700779553834));
#29175=CARTESIAN_POINT('Ctrl Pts',(-49.7188870758208,-8.53525345256675,
22.2268112355569));
#29176=CARTESIAN_POINT('Ctrl Pts',(-49.7073553886521,-8.54013948886813,
22.2835482806785));
#29177=CARTESIAN_POINT('Ctrl Pts',(-49.7070885620479,-8.54025254469902,
22.2848610940475));
#29178=CARTESIAN_POINT('Ctrl Pts',(-49.706821700383,-8.54036513501698,22.2861739864676));
#29179=CARTESIAN_POINT('Ctrl Pts',(-49.7065548032017,-8.54047726034838,
22.287486960151));
#29180=CARTESIAN_POINT('Ctrl Pts',(-49.6793313303115,-8.55191402751557,
22.4214100810567));
#29181=CARTESIAN_POINT('Ctrl Pts',(-49.6518481112244,-8.5584728839653,22.5556485348429));
#29182=CARTESIAN_POINT('Ctrl Pts',(-49.6241123555729,-8.56059423319272,
22.6901689000943));
#29183=CARTESIAN_POINT('Ctrl Pts',(-49.6174141089786,-8.56110654374291,
22.7226558670884));
#29184=CARTESIAN_POINT('Ctrl Pts',(-49.6107011130711,-8.56135981233827,
22.7551593362476));
#29185=CARTESIAN_POINT('Ctrl Pts',(-49.603973431638,-8.56135981233827,22.7876789472102));
#29186=CARTESIAN_POINT('Origin',(-36.1446456971182,-3.61941807409668,34.5428371044526));
#29187=CARTESIAN_POINT('Origin',(-36.1446456971182,-3.61941807409668,34.5428371044526));
#29188=CARTESIAN_POINT('Ctrl Pts',(-10.8649863601191,13.1261401876617,49.7699317919394));
#29189=CARTESIAN_POINT('Ctrl Pts',(-10.8649863601191,13.1261401876617,50.0824317919394));
#29190=CARTESIAN_POINT('Ctrl Pts',(-10.8649863601191,13.4386401876617,50.0824317919394));
#29191=CARTESIAN_POINT('Ctrl Pts',(-10.4914375950611,13.1261401876617,49.8101116217086));
#29192=CARTESIAN_POINT('Ctrl Pts',(-10.5138842101856,13.1639055963027,50.0824317919394));
#29193=CARTESIAN_POINT('Ctrl Pts',(-10.4825839193318,13.4386401851022,50.0824317919394));
#29194=CARTESIAN_POINT('Ctrl Pts',(-10.1172066156767,13.1182927286051,49.8484089205029));
#29195=CARTESIAN_POINT('Ctrl Pts',(-10.1310095155991,13.1821712224816,50.0824317919381));
#29196=CARTESIAN_POINT('Ctrl Pts',(-10.1008424173742,13.4229452699553,50.0824317919394));
#29197=CARTESIAN_POINT('Ctrl Pts',(-9.36754573057138,13.0884919386939,49.921120805052));
#29198=CARTESIAN_POINT('Ctrl Pts',(-9.37377765929087,13.180412811403,50.0824317919407));
#29199=CARTESIAN_POINT('Ctrl Pts',(-9.33859724908609,13.3633436893193,50.0824317919394));
#29200=CARTESIAN_POINT('Ctrl Pts',(-8.99271962453602,13.0669605544565,49.955469139931));
#29201=CARTESIAN_POINT('Ctrl Pts',(-8.99180823791993,13.1642472289417,50.0824317919394));
#29202=CARTESIAN_POINT('Ctrl Pts',(-8.95863183223867,13.3202672259815,50.0824317919394));
#29203=CARTESIAN_POINT('Ctrl Pts',(-8.62010343469179,13.0346110567867,49.9876168488787));
#29204=CARTESIAN_POINT('Ctrl Pts',(-8.60451564625867,13.125337974864,50.0824317919394));
#29205=CARTESIAN_POINT('Ctrl Pts',(-8.58213843785567,13.2555819259088,50.0824317919394));
#29206=CARTESIAN_POINT('Ctrl Pts',(-8.62010343469228,13.0346110567867,49.9876168488786));
#29207=CARTESIAN_POINT('Ctrl Pts',(-8.83743262669382,13.0534789729962,49.9688666310144));
#29208=CARTESIAN_POINT('Ctrl Pts',(-9.05495247870489,13.0686233597136,49.9494169416172));
#29209=CARTESIAN_POINT('Ctrl Pts',(-9.27257311703778,13.0809296717971,49.9292822276746));
#29210=CARTESIAN_POINT('Ctrl Pts',(-9.42907418117352,13.0897797098789,49.9148024238186));
#29211=CARTESIAN_POINT('Ctrl Pts',(-9.5856278909298,13.0971603804829,49.8999681158358));
#29212=CARTESIAN_POINT('Ctrl Pts',(-9.74220410542708,13.1033855068804,49.884781586804));
#29213=CARTESIAN_POINT('Ctrl Pts',(-9.74226146095453,13.1033877872102,49.8847760238175));
#29214=CARTESIAN_POINT('Ctrl Pts',(-9.74231881649497,13.1033900673852,49.8847704607826));
#29215=CARTESIAN_POINT('Ctrl Pts',(-9.74237617204842,13.1033923474055,49.8847648976995));
#29216=CARTESIAN_POINT('Ctrl Pts',(-10.1166203384253,13.1182694471954,49.8484658598822));
#29217=CARTESIAN_POINT('Ctrl Pts',(-10.4908161997162,13.1261401876617,49.8101784605299));
#29218=CARTESIAN_POINT('Ctrl Pts',(-10.8649863601191,13.1261401876617,49.7699317919394));
#29219=CARTESIAN_POINT('Origin',(35.1659821576993,12.8136401876617,36.932654334243));
#29220=CARTESIAN_POINT('Origin',(35.1659821576993,12.8136401876617,36.932654334243));
#29221=CARTESIAN_POINT('Origin',(39.8582830101054,-8.24885981233827,39.8571882336827));
#29222=CARTESIAN_POINT('Origin',(38.9743995336222,-8.24885981233827,40.7410717101659));
#29223=CARTESIAN_POINT('Origin',(0.0835265683620476,-8.87385981233827,49.7699317919394));
#29224=CARTESIAN_POINT('Origin',(22.7887737236329,-8.87385981233827,49.7699317919394));
#29225=CARTESIAN_POINT('Origin',(-49.603973431638,-8.87385981233827,0.0824317919394229));
#29226=CARTESIAN_POINT('Origin',(-49.603973431638,-8.87385981233827,44.4574317919389));
#29227=CARTESIAN_POINT('Origin',(0.0835265683620477,-8.24885981233827,0.0824317919394229));
#29228=CARTESIAN_POINT('Origin',(-39.4190920287332,-8.24885981233827,37.8172834360675));
#29229=CARTESIAN_POINT('Ctrl Pts',(-39.2593077130565,-8.4698306814591,37.6646495687126));
#29230=CARTESIAN_POINT('Ctrl Pts',(-39.0443992301308,-8.46631238203738,
37.8845323757067));
#29231=CARTESIAN_POINT('Ctrl Pts',(-39.1981211596124,-8.2488598123383,38.0382543051883));
#29232=CARTESIAN_POINT('Ctrl Pts',(-38.1677401528071,-6.92666471828265,
36.5732839934435));
#29233=CARTESIAN_POINT('Ctrl Pts',(-37.9532471818617,-6.9233956438625,36.7933803274376));
#29234=CARTESIAN_POINT('Ctrl Pts',(-38.1066522799251,-6.70569384849333,
36.946785425501));
#29235=CARTESIAN_POINT('Ctrl Pts',(-37.0761523844497,-5.38351572788325,
35.4819151782211));
#29236=CARTESIAN_POINT('Ctrl Pts',(-36.8618908744297,-5.38020745678036,
35.7020240200208));
#29237=CARTESIAN_POINT('Ctrl Pts',(-37.0151713871424,-5.16254485803799,
35.8553045327183));
#29238=CARTESIAN_POINT('Ctrl Pts',(-35.984538282875,-3.84038894321749,34.3905421902094));
#29239=CARTESIAN_POINT('Ctrl Pts',(-35.7701869713607,-3.8365505471153,34.6103201169366));
#29240=CARTESIAN_POINT('Ctrl Pts',(-35.9236748279975,-3.61941807409669,
34.7638079735734));
#29241=CARTESIAN_POINT('Origin',(-39.4190920287332,-8.24885981233827,37.8172834360675));
#29242=CARTESIAN_POINT('Origin',(-24.407589955155,12.8136401876617,26.3413152684223));
#29243=CARTESIAN_POINT('Origin',(-34.9989290209756,12.8136401876617,36.9326543342427));
#29244=CARTESIAN_POINT('Origin',(0.0835265683620477,12.8136401876617,0.0824317919394229));
#29245=CARTESIAN_POINT('Origin',(-34.9989290209756,12.8136401876617,36.9326543342427));
#29246=CARTESIAN_POINT('Origin',(34.8549575729643,12.3739187291566,36.6216294748833));
#29247=CARTESIAN_POINT('Origin',(34.5439318808756,11.9341984494202,36.3106040574193));
#29248=CARTESIAN_POINT('Origin',(39.6373121409846,-8.24885981233827,41.4039843175283));
#29249=CARTESIAN_POINT('Origin',(37.8183782124906,-8.24885981233827,39.5850503890343));
#29250=CARTESIAN_POINT('Origin',(0.0835265683620477,-8.24885981233827,0.0824317919394229));
#29251=CARTESIAN_POINT('Ctrl Pts',(22.7887737236329,-8.56135981233827,49.7699317919394));
#29252=CARTESIAN_POINT('Ctrl Pts',(22.6541181864147,-8.56135981233827,49.7977894301704));
#29253=CARTESIAN_POINT('Ctrl Pts',(22.5197384329217,-8.55702114807029,49.8253956090288));
#29254=CARTESIAN_POINT('Ctrl Pts',(22.3856647415717,-8.54791555690698,49.8527441922136));
#29255=CARTESIAN_POINT('Ctrl Pts',(22.3532856491678,-8.54571653654214,49.8593489354196));
#29256=CARTESIAN_POINT('Ctrl Pts',(22.3209244662425,-8.54323926489437,49.8659386346358));
#29257=CARTESIAN_POINT('Ctrl Pts',(22.2885817365737,-8.54047726034825,49.8725131635028));
#29258=CARTESIAN_POINT('Ctrl Pts',(22.2872687628902,-8.54036513501685,49.872780060684));
#29259=CARTESIAN_POINT('Ctrl Pts',(22.2859558704701,-8.54025254469889,49.873046922349));
#29260=CARTESIAN_POINT('Ctrl Pts',(22.2846430571011,-8.54013948886801,49.8733137489532));
#29261=CARTESIAN_POINT('Ctrl Pts',(22.22312560482,-8.5348417772165,49.8858170439981));
#29262=CARTESIAN_POINT('Ctrl Pts',(22.1616123554514,-8.52857105445296,49.8982768361997));
#29263=CARTESIAN_POINT('Ctrl Pts',(22.1002028692077,-8.52099310668482,49.9106746950791));
#29264=CARTESIAN_POINT('Ctrl Pts',(22.0472505817754,-8.51445877961403,49.9213651441788));
#29265=CARTESIAN_POINT('Ctrl Pts',(21.994374806306,-8.50695259656895,49.9320096488017));
#29266=CARTESIAN_POINT('Ctrl Pts',(21.9416562445106,-8.49822768693266,49.9425922088684));
#29267=CARTESIAN_POINT('Ctrl Pts',(21.8915966824201,-8.48994284112507,49.9526410096075));
#29268=CARTESIAN_POINT('Ctrl Pts',(21.8416783185839,-8.48055949752612,49.9626340619876));
#29269=CARTESIAN_POINT('Ctrl Pts',(21.7919948253829,-8.46983068145907,49.9725521390571));
#29270=CARTESIAN_POINT('Origin',(37.8183782124906,-8.24885981233827,39.5850503890343));
#29271=CARTESIAN_POINT('Ctrl Pts',(22.7887737236329,-8.56135981233827,49.7699317919394));
#29272=CARTESIAN_POINT('Ctrl Pts',(22.7887737236329,-8.56135981233827,50.0824317919394));
#29273=CARTESIAN_POINT('Ctrl Pts',(22.7887737236329,-8.87385981233827,50.0824317919394));
#29274=CARTESIAN_POINT('Ctrl Pts',(22.6194435423556,-8.56135981233827,49.8049629464425));
#29275=CARTESIAN_POINT('Ctrl Pts',(22.6283504611892,-8.59454828035467,50.0824317919394));
#29276=CARTESIAN_POINT('Ctrl Pts',(22.6034355280221,-8.87385980853143,50.0824317919394));
#29277=CARTESIAN_POINT('Ctrl Pts',(22.451311719341,-8.55449257599307,49.8394385445005));
#29278=CARTESIAN_POINT('Ctrl Pts',(22.453686206106,-8.61264419244103,50.0824317919394));
#29279=CARTESIAN_POINT('Ctrl Pts',(22.4199421318354,-8.86012534447524,50.0824317919394));
#29280=CARTESIAN_POINT('Ctrl Pts',(22.1179744762618,-8.52578588737924,49.9071874678825));
#29281=CARTESIAN_POINT('Ctrl Pts',(22.1068093504948,-8.61245644138935,50.0824317919394));
#29282=CARTESIAN_POINT('Ctrl Pts',(22.0571513437917,-8.80271195759283,50.0824317919394));
#29283=CARTESIAN_POINT('Ctrl Pts',(21.9515338786954,-8.5042820521619,49.9407041085403));
#29284=CARTESIAN_POINT('Ctrl Pts',(21.930616886141,-8.59771167169906,50.0824317919394));
#29285=CARTESIAN_POINT('Ctrl Pts',(21.876342196488,-8.75963242031969,50.0824317919394));
#29286=CARTESIAN_POINT('Ctrl Pts',(21.7919948253829,-8.46983068145907,49.9725521390571));
#29287=CARTESIAN_POINT('Ctrl Pts',(21.757315388682,-8.55674861132668,50.0824317919394));
#29288=CARTESIAN_POINT('Ctrl Pts',(21.7038295264614,-8.69080155057986,50.0824317919394));
#29289=CARTESIAN_POINT('Origin',(21.7038295264614,-8.69080155057986,49.7699317919394));
#29290=CARTESIAN_POINT('Origin',(-44.2914734316384,-8.87385981233827,44.457431791939));
#29291=CARTESIAN_POINT('Origin',(-44.2914734316384,-8.87385981233827,49.769931791939));
#29292=CARTESIAN_POINT('Origin',(-39.4190920287332,-8.24885981233827,37.8172834360675));
#29293=CARTESIAN_POINT('Origin',(-39.4190920287332,-8.24885981233827,37.8172834360675));
#29294=CARTESIAN_POINT('Origin',(-34.9989290209756,12.8136401876617,36.9326543342427));
#29295=CARTESIAN_POINT('Origin',(-34.9989290209756,12.8136401876617,36.9326543342427));
#29296=CARTESIAN_POINT('Origin',(34.5439318808756,11.9341984494201,36.3106040574193));
#29297=CARTESIAN_POINT('Origin',(34.5439318808756,11.9341984494201,36.3106040574193));
#29298=CARTESIAN_POINT('Origin',(37.8183782124906,-8.24885981233827,39.5850503890343));
#29299=CARTESIAN_POINT('Origin',(37.8183782124906,-8.24885981233827,39.5850503890343));
#29300=CARTESIAN_POINT('Ctrl Pts',(-21.7449659867426,-8.77420095360317,
50.0824317919394));
#29301=CARTESIAN_POINT('Ctrl Pts',(-21.798926229011,-8.64003310969503,50.0824317919394));
#29302=CARTESIAN_POINT('Ctrl Pts',(-21.8338566105543,-8.55319446981481,
49.9721960693566));
#29303=CARTESIAN_POINT('Ctrl Pts',(-18.2490305748135,-7.36815837377856,
50.0824317919394));
#29304=CARTESIAN_POINT('Ctrl Pts',(-18.3130464386012,-7.24249091567042,
50.0824317919394));
#29305=CARTESIAN_POINT('Ctrl Pts',(-18.3259998716927,-7.14715496161882,
49.9774388543335));
#29306=CARTESIAN_POINT('Ctrl Pts',(-14.6840632078164,-6.21561709199713,
50.0824317919394));
#29307=CARTESIAN_POINT('Ctrl Pts',(-14.7335250825033,-6.08656532570595,
50.0824317919394));
#29308=CARTESIAN_POINT('Ctrl Pts',(-14.7474057099706,-5.99460855782839,
49.9821571538487));
#29309=CARTESIAN_POINT('Ctrl Pts',(-9.22874352618438,-5.02557369219655,
50.0824317919394));
#29310=CARTESIAN_POINT('Ctrl Pts',(-9.25561217772287,-4.89581925234152,
50.0824317919394));
#29311=CARTESIAN_POINT('Ctrl Pts',(-9.26953608557641,-4.8045652666467,49.9871995617052));
#29312=CARTESIAN_POINT('Ctrl Pts',(-7.41133500973276,-4.71947214408047,
50.0824317919394));
#29313=CARTESIAN_POINT('Ctrl Pts',(-7.43234648598233,-4.58961053626118,
50.0824317919394));
#29314=CARTESIAN_POINT('Ctrl Pts',(-7.44435366976549,-4.4984637156113,49.9885338203398));
#29315=CARTESIAN_POINT('Ctrl Pts',(-4.64537610952596,-4.40691837826605,
50.0824317919394));
#29316=CARTESIAN_POINT('Ctrl Pts',(-4.65806729858047,-4.27725721313721,
50.0824317919394));
#29317=CARTESIAN_POINT('Ctrl Pts',(-4.66632727320178,-4.18590981848828,
49.9899065809487));
#29318=CARTESIAN_POINT('Ctrl Pts',(-3.71666105631754,-4.327158062246,50.0824317919394));
#29319=CARTESIAN_POINT('Ctrl Pts',(-3.72675911584482,-4.19755005843067,
50.0824317919394));
#29320=CARTESIAN_POINT('Ctrl Pts',(-3.73352231198055,-4.1061494680647,49.9902596193181));
#29321=CARTESIAN_POINT('Ctrl Pts',(-1.84550713430984,-4.21946011836696,
50.0824317919394));
#29322=CARTESIAN_POINT('Ctrl Pts',(-1.8507435419627,-4.08996813963968,50.0824317919394));
#29323=CARTESIAN_POINT('Ctrl Pts',(-1.85408687661129,-3.99845145937572,
49.9907371683897));
#29324=CARTESIAN_POINT('Ctrl Pts',(-0.912269960149392,-4.19205938565825,
50.0824317919394));
#29325=CARTESIAN_POINT('Ctrl Pts',(-0.914869480160837,-4.06258497561498,
50.0824317919394));
#29326=CARTESIAN_POINT('Ctrl Pts',(-0.91669922368614,-3.9710507150748,49.9908592564268));
#29327=CARTESIAN_POINT('Ctrl Pts',(3.74233330481107,-4.18598197768416,50.0824317919394));
#29328=CARTESIAN_POINT('Ctrl Pts',(3.75179154006485,-4.05651422028119,50.0824317919394));
#29329=CARTESIAN_POINT('Ctrl Pts',(3.75860756853322,-3.96497330343863,49.9908862940722));
#29330=CARTESIAN_POINT('Ctrl Pts',(7.42861042436576,-4.60394036704883,50.0824317919394));
#29331=CARTESIAN_POINT('Ctrl Pts',(7.45931217637961,-4.47650762044643,50.0824317919394));
#29332=CARTESIAN_POINT('Ctrl Pts',(7.46124533724433,-4.38293092071028,49.9889892256309));
#29333=CARTESIAN_POINT('Ctrl Pts',(11.9953617287628,-5.59091481619281,50.0824317919394));
#29334=CARTESIAN_POINT('Ctrl Pts',(12.0266282204217,-5.46011080390181,50.0824317919394));
#29335=CARTESIAN_POINT('Ctrl Pts',(12.0469073010734,-5.36990690683472,49.984803391475));
#29336=CARTESIAN_POINT('Ctrl Pts',(12.9059760664518,-5.81129472998947,50.0824317919394));
#29337=CARTESIAN_POINT('Ctrl Pts',(12.9396172744353,-5.68032983292117,50.0824317919394));
#29338=CARTESIAN_POINT('Ctrl Pts',(12.9612247995486,-5.59028691905869,49.9838785470594));
#29339=CARTESIAN_POINT('Ctrl Pts',(14.7061033059095,-6.29050753230872,50.0824317919394));
#29340=CARTESIAN_POINT('Ctrl Pts',(14.7441427204447,-6.15904772772697,50.0824317919394));
#29341=CARTESIAN_POINT('Ctrl Pts',(14.7685229600323,-6.06949999371254,49.9818976821262));
#29342=CARTESIAN_POINT('Ctrl Pts',(15.5979075859762,-6.54980455615392,50.0824317919394));
#29343=CARTESIAN_POINT('Ctrl Pts',(15.6381893611325,-6.41814737484953,50.0824317919394));
#29344=CARTESIAN_POINT('Ctrl Pts',(15.6638045210804,-6.32879713521949,49.9808397055944));
#29345=CARTESIAN_POINT('Ctrl Pts',(18.2508522029681,-7.38126084278977,50.0824317919394));
#29346=CARTESIAN_POINT('Ctrl Pts',(18.3002836337393,-7.24964619597268,50.0824317919394));
#29347=CARTESIAN_POINT('Ctrl Pts',(18.3268527946815,-7.16025352121961,49.9775040185271));
#29348=CARTESIAN_POINT('Ctrl Pts',(19.9895860300914,-8.00683451481104,50.0824317919394));
#29349=CARTESIAN_POINT('Ctrl Pts',(20.043507385477,-7.87510646586172,50.0824317919394));
#29350=CARTESIAN_POINT('Ctrl Pts',(20.0718858539989,-7.78582757943738,49.9750659873749));
#29351=CARTESIAN_POINT('Ctrl Pts',(21.7038295264614,-8.69080155057986,50.0824317919394));
#29352=CARTESIAN_POINT('Ctrl Pts',(21.7573285588578,-8.55671560258926,50.0824317919394));
#29353=CARTESIAN_POINT('Ctrl Pts',(21.7920088993551,-8.46979540751453,49.9725075380777));
#29354=CARTESIAN_POINT('Origin',(-21.5367763897373,-8.69080155057986,49.7699317919394));
#29355=CARTESIAN_POINT('Origin',(0.0835265683620476,-8.87385981233827,49.7699317919394));
#29356=CARTESIAN_POINT('Origin',(-22.6217205869088,-8.87385981233827,49.7699317919394));
#29357=CARTESIAN_POINT('Origin',(-41.2380259572272,-8.24885981233827,39.6362173645615));
#29358=CARTESIAN_POINT('Origin',(-40.5751133498648,-8.24885981233827,38.9733047571991));
#29359=CARTESIAN_POINT('Origin',(-34.6879038942329,12.3739193162068,36.621629186931));
#29360=CARTESIAN_POINT('Origin',(-34.3768787441519,11.9341984494201,36.310604057419));
#29361=CARTESIAN_POINT('Origin',(34.5439318808756,11.4830954176946,36.3106040574193));
#29362=CARTESIAN_POINT('Origin',(34.5439318808756,-3.61941807409669,36.3106040574193));
#29363=CARTESIAN_POINT('Ctrl Pts',(37.6657443451356,-8.46983068145905,39.4252660733575));
#29364=CARTESIAN_POINT('Ctrl Pts',(37.8856271521297,-8.46631238203734,39.2103575904319));
#29365=CARTESIAN_POINT('Ctrl Pts',(38.0393490816113,-8.24885981233825,39.3640795199135));
#29366=CARTESIAN_POINT('Ctrl Pts',(36.5743787698899,-6.92666471828331,38.3336985130867));
#29367=CARTESIAN_POINT('Ctrl Pts',(36.7944751038716,-6.92339564388109,38.1192055421283));
#29368=CARTESIAN_POINT('Ctrl Pts',(36.9478802019155,-6.70569384850732,38.2726106402177));
#29369=CARTESIAN_POINT('Ctrl Pts',(35.4830099546367,-5.38351572788366,37.2421107447585));
#29370=CARTESIAN_POINT('Ctrl Pts',(35.7031187964357,-5.38020745678172,37.0278492347378));
#29371=CARTESIAN_POINT('Ctrl Pts',(35.8563993091415,-5.16254485803843,37.1811297474436));
#29372=CARTESIAN_POINT('Ctrl Pts',(34.3916369666324,-3.84038894321749,36.1504966431761));
#29373=CARTESIAN_POINT('Ctrl Pts',(34.6114148933596,-3.8365505471153,35.9361453316618));
#29374=CARTESIAN_POINT('Ctrl Pts',(34.7649027499964,-3.61941807409669,36.0896331882986));
#29375=CARTESIAN_POINT('Origin',(34.5439318808756,-3.61941807409668,36.3106040574193));
#29376=CARTESIAN_POINT('Ctrl Pts',(-22.6217205869088,-8.87385981233827,
50.0824317919394));
#29377=CARTESIAN_POINT('Ctrl Pts',(-22.6217205869088,-8.56135981233826,
50.0824317919394));
#29378=CARTESIAN_POINT('Ctrl Pts',(-22.6217205869088,-8.56135981233827,
49.7699317919394));
#29379=CARTESIAN_POINT('Ctrl Pts',(-22.438990136685,-8.87385981115686,50.0824317919394));
#29380=CARTESIAN_POINT('Ctrl Pts',(-22.4634538292487,-8.59410214473108,
50.0824317919394));
#29381=CARTESIAN_POINT('Ctrl Pts',(-22.4547771519531,-8.56135981233827,
49.8044691746351));
#29382=CARTESIAN_POINT('Ctrl Pts',(-22.2528965670481,-8.86016990857445,
50.0824317919394));
#29383=CARTESIAN_POINT('Ctrl Pts',(-22.2867063988249,-8.61269267441879,
50.0824317919388));
#29384=CARTESIAN_POINT('Ctrl Pts',(-22.2842668072145,-8.55451485837127,
49.8394377011463));
#29385=CARTESIAN_POINT('Ctrl Pts',(-21.8886078761106,-8.80243256293693,
50.0824317919394));
#29386=CARTESIAN_POINT('Ctrl Pts',(-21.9383801137018,-8.61241087733877,
50.08243179194));
#29387=CARTESIAN_POINT('Ctrl Pts',(-21.9495507300761,-8.52564618972366,
49.9074652049407));
#29388=CARTESIAN_POINT('Ctrl Pts',(-21.7095372588941,-8.7597314335958,50.0824317919394));
#29389=CARTESIAN_POINT('Ctrl Pts',(-21.7638279668325,-8.59777411058506,
50.0824317919414));
#29390=CARTESIAN_POINT('Ctrl Pts',(-21.7847313145468,-8.50433615796108,
49.9406540839376));
#29391=CARTESIAN_POINT('Ctrl Pts',(-21.5367763897364,-8.69080155058829,
50.0824317919394));
#29392=CARTESIAN_POINT('Ctrl Pts',(-21.5902622519567,-8.5567486113334,50.0824317919394));
#29393=CARTESIAN_POINT('Ctrl Pts',(-21.624941688657,-8.46983068146548,49.9725521390553));
#29394=CARTESIAN_POINT('Ctrl Pts',(-22.6217205869088,-8.56135981233827,
49.7699317919394));
#29395=CARTESIAN_POINT('Ctrl Pts',(-22.5570649108185,-8.56135981233827,
49.7833078065708));
#29396=CARTESIAN_POINT('Ctrl Pts',(-22.4923868342644,-8.56033639109561,
49.7966425973418));
#29397=CARTESIAN_POINT('Ctrl Pts',(-22.4277520323567,-8.55827526792405,
49.8099240615446));
#29398=CARTESIAN_POINT('Ctrl Pts',(-22.3612333428163,-8.55615406992689,
49.8235926358711));
#29399=CARTESIAN_POINT('Ctrl Pts',(-22.2947577095333,-8.552934288094,49.8372053106334));
#29400=CARTESIAN_POINT('Ctrl Pts',(-22.2283761570625,-8.54855443110404,
49.8507510984659));
#29401=CARTESIAN_POINT('Ctrl Pts',(-22.1925472882174,-8.5461904411729,49.8580623202977));
#29402=CARTESIAN_POINT('Ctrl Pts',(-22.1567457285975,-8.54348767314343,
49.8653540415904));
#29403=CARTESIAN_POINT('Ctrl Pts',(-22.1209815952407,-8.54043032524651,
49.8726238531984));
#29404=CARTESIAN_POINT('Ctrl Pts',(-22.1196238899022,-8.54031425987119,
49.8728998353376));
#29405=CARTESIAN_POINT('Ctrl Pts',(-22.1182662759902,-8.54019768609479,
49.8731757782021));
#29406=CARTESIAN_POINT('Ctrl Pts',(-22.1169087561037,-8.54008060317761,
49.8734516812435));
#29407=CARTESIAN_POINT('Ctrl Pts',(-22.0497247180194,-8.53428613692706,
49.8871061997702));
#29408=CARTESIAN_POINT('Ctrl Pts',(-21.9826706468966,-8.5273633766299,49.9006844600952));
#29409=CARTESIAN_POINT('Ctrl Pts',(-21.9157941683003,-8.51884310578637,
49.914177934353));
#29410=CARTESIAN_POINT('Ctrl Pts',(-21.8545644066734,-8.51104224420251,
49.9265320868094));
#29411=CARTESIAN_POINT('Ctrl Pts',(-21.7934834053665,-8.50190252011177,
49.9388151779388));
#29412=CARTESIAN_POINT('Ctrl Pts',(-21.7326032971608,-8.49102344833061,
49.9510170411214));
#29413=CARTESIAN_POINT('Ctrl Pts',(-21.6966410620796,-8.48459711716286,
49.9582247528869));
#29414=CARTESIAN_POINT('Ctrl Pts',(-21.6607492307147,-8.47756307924556,
49.9654040514526));
#29415=CARTESIAN_POINT('Ctrl Pts',(-21.624941688657,-8.46983068146548,49.9725521390553));
#29416=CARTESIAN_POINT('Origin',(-39.6912298733817,-8.24885981233827,39.8571882336823));
#29417=CARTESIAN_POINT('Origin',(-38.8073463968985,-8.24885981233827,40.7410717101655));
#29418=CARTESIAN_POINT('Origin',(-34.3768787441519,11.9341984494201,36.310604057419));
#29419=CARTESIAN_POINT('Origin',(-34.3768787441519,11.9341984494202,36.310604057419));
#29420=CARTESIAN_POINT('Origin',(34.5439318808756,-3.61941807409668,36.3106040574193));
#29421=CARTESIAN_POINT('Origin',(0.0835265683620477,-8.24885981233827,0.0824317919394229));
#29422=CARTESIAN_POINT('Origin',(-37.6513250757669,-8.24885981233827,39.5850503890339));
#29423=CARTESIAN_POINT('Origin',(-39.4702590042609,-8.24885981233827,41.4039843175279));
#29424=CARTESIAN_POINT('Origin',(-37.6513250757669,-8.24885981233827,39.5850503890339));
#29425=CARTESIAN_POINT('Origin',(-34.3768787441519,11.4830954176946,36.310604057419));
#29426=CARTESIAN_POINT('Origin',(-34.3768787441519,-3.61941807409668,36.310604057419));
#29427=CARTESIAN_POINT('Origin',(-37.6513250757669,-8.24885981233827,39.5850503890339));
#29428=CARTESIAN_POINT('Origin',(-37.6513250757669,-8.24885981233827,39.5850503890339));
#29429=CARTESIAN_POINT('Origin',(-34.3768787441519,-3.61941807409668,36.310604057419));
#29430=CARTESIAN_POINT('Origin',(-34.3768787441519,-3.61941807409669,36.310604057419));
#29431=CARTESIAN_POINT('Ctrl Pts',(-37.8722959448876,-8.24885981233824,
39.3640795199131));
#29432=CARTESIAN_POINT('Ctrl Pts',(-37.718574015406,-8.46631238203733,39.2103575904315));
#29433=CARTESIAN_POINT('Ctrl Pts',(-37.4986912084119,-8.46983068145904,
39.4252660733572));
#29434=CARTESIAN_POINT('Ctrl Pts',(-36.7808270651937,-6.70569384850457,
38.2726106402191));
#29435=CARTESIAN_POINT('Ctrl Pts',(-36.6274219671306,-6.92339564387865,
38.1192055421485));
#29436=CARTESIAN_POINT('Ctrl Pts',(-36.40732563317,-6.92666471828328,38.3336985130827));
#29437=CARTESIAN_POINT('Ctrl Pts',(-35.6893461724109,-5.16254485804842,
37.1811297474364));
#29438=CARTESIAN_POINT('Ctrl Pts',(-35.536065659707,-5.38020745680514,37.0278492347098));
#29439=CARTESIAN_POINT('Ctrl Pts',(-35.3159568179278,-5.38351572788345,
37.2421107447437));
#29440=CARTESIAN_POINT('Ctrl Pts',(-34.5978496132727,-3.61941807409668,
36.0896331882982));
#29441=CARTESIAN_POINT('Ctrl Pts',(-34.4443617566359,-3.83655054711529,
35.9361453316614));
#29442=CARTESIAN_POINT('Ctrl Pts',(-34.2245838299087,-3.84038894321747,
36.1504966431758));
#29443=CARTESIAN_POINT('Ctrl Pts',(0.0835265683646154,11.4728541727075,
48.5199460669665));
#29444=CARTESIAN_POINT('Ctrl Pts',(0.434571873652948,11.47819221482,48.5199461833401));
#29445=CARTESIAN_POINT('Ctrl Pts',(0.78544120302723,11.4874426767152,48.5184889915191));
#29446=CARTESIAN_POINT('Ctrl Pts',(1.48685396299278,11.5143737377395,48.5151613829998));
#29447=CARTESIAN_POINT('Ctrl Pts',(1.83739739358405,11.5320543368685,48.5132909663016));
#29448=CARTESIAN_POINT('Ctrl Pts',(2.88857791675096,11.598649286609,48.5108119661593));
#29449=CARTESIAN_POINT('Ctrl Pts',(3.59085027393415,11.6392592214975,48.506118103167));
#29450=CARTESIAN_POINT('Ctrl Pts',(4.29256572527697,11.6756605207451,48.4959174422581));
#29451=CARTESIAN_POINT('Ctrl Pts',(0.0835265683646867,11.4942063411577,
48.5199465324602));
#29452=CARTESIAN_POINT('Ctrl Pts',(0.356369924468222,11.4971000233707,48.5198869612823));
#29453=CARTESIAN_POINT('Ctrl Pts',(0.651973539440871,11.5031786713304,48.5195752074941));
#29454=CARTESIAN_POINT('Ctrl Pts',(1.2945339969987,11.5255419633083,48.5183112784645));
#29455=CARTESIAN_POINT('Ctrl Pts',(1.64148768476021,11.5418711528752,48.5173741424329));
#29456=CARTESIAN_POINT('Ctrl Pts',(2.76813631993237,11.6120206208596,48.5172046544328));
#29457=CARTESIAN_POINT('Ctrl Pts',(3.51890802363922,11.6580360440938,48.5141149281054));
#29458=CARTESIAN_POINT('Ctrl Pts',(4.29124902552725,11.6996409410751,48.5059136087032));
#29459=CARTESIAN_POINT('Ctrl Pts',(0.0835265683659855,11.5200575082527,
48.5195892904601));
#29460=CARTESIAN_POINT('Ctrl Pts',(0.356156584738792,11.5200113925674,48.5195869596123));
#29461=CARTESIAN_POINT('Ctrl Pts',(0.651610340351263,11.5245005081763,48.5196902430686));
#29462=CARTESIAN_POINT('Ctrl Pts',(1.29397444549905,11.5448479357178,48.5193460059354));
#29463=CARTESIAN_POINT('Ctrl Pts',(1.6408816402107,11.5607507931991,48.5189135245556));
#29464=CARTESIAN_POINT('Ctrl Pts',(2.76751045405255,11.6290600690807,48.5194534619891));
#29465=CARTESIAN_POINT('Ctrl Pts',(3.51790722899464,11.6785648284704,48.5175683502971));
#29466=CARTESIAN_POINT('Ctrl Pts',(4.28995382479,11.7229366511906,48.5119171961236));
#29467=CARTESIAN_POINT('Ctrl Pts',(0.0835265683637358,11.5731362269332,
48.5213546907495));
#29468=CARTESIAN_POINT('Ctrl Pts',(0.394869806429155,11.5731490589917,48.5213559145826));
#29469=CARTESIAN_POINT('Ctrl Pts',(0.717676140691825,11.5776504745527,48.5214911613194));
#29470=CARTESIAN_POINT('Ctrl Pts',(1.38907005436015,11.5959692446123,48.5214366576315));
#29471=CARTESIAN_POINT('Ctrl Pts',(1.73765605635396,11.6098088718851,48.5212544268118));
#29472=CARTESIAN_POINT('Ctrl Pts',(2.82637284200128,11.6658592241826,48.5212339924692));
#29473=CARTESIAN_POINT('Ctrl Pts',(3.55158573922134,11.7135824344715,48.5204767822115));
#29474=CARTESIAN_POINT('Ctrl Pts',(4.2874400917096,11.7642258753785,48.5189262877417));
#29475=CARTESIAN_POINT('Ctrl Pts',(0.0835265683629213,11.5876793312944,
48.5199317919394));
#29476=CARTESIAN_POINT('Ctrl Pts',(0.433796367851579,11.5876793312944,48.5199317919394));
#29477=CARTESIAN_POINT('Ctrl Pts',(0.784105140124401,11.5930695682598,48.5199317919388));
#29478=CARTESIAN_POINT('Ctrl Pts',(1.48472521472274,11.6126245374907,48.5199317919371));
#29479=CARTESIAN_POINT('Ctrl Pts',(1.83503651704826,11.6267892697562,48.5199317919361));
#29480=CARTESIAN_POINT('Ctrl Pts',(2.88586109583041,11.6794362415569,48.5199317919341));
#29481=CARTESIAN_POINT('Ctrl Pts',(3.58626504409264,11.728071256096,48.5199317919341));
#29482=CARTESIAN_POINT('Ctrl Pts',(4.28622155936646,11.7822193894509,48.5199317919394));
#29483=CARTESIAN_POINT('Ctrl Pts',(0.0835265683619702,11.6131136241746,
48.5199317919394));
#29484=CARTESIAN_POINT('Ctrl Pts',(0.433874220973474,11.6131136241746,48.5199317919394));
#29485=CARTESIAN_POINT('Ctrl Pts',(0.784221873584978,11.6169153282063,48.5199317919388));
#29486=CARTESIAN_POINT('Ctrl Pts',(1.48483467245502,11.6321221443329,48.5199317919372));
#29487=CARTESIAN_POINT('Ctrl Pts',(1.83509981871355,11.6435272564279,48.5199317919363));
#29488=CARTESIAN_POINT('Ctrl Pts',(2.88564773843024,11.689147704808,48.5199317919344));
#29489=CARTESIAN_POINT('Ctrl Pts',(3.58568299282948,11.734768153188,48.5199317919344));
#29490=CARTESIAN_POINT('Ctrl Pts',(4.28505819640496,11.7955954176946,48.5199317919394));
#29491=CARTESIAN_POINT('',(0.0835265683646154,11.4728541727075,48.5199460669665));
#29492=CARTESIAN_POINT('Ctrl Pts',(0.0835265683619702,11.6131136241746,
48.5199317919394));
#29493=CARTESIAN_POINT('Ctrl Pts',(0.0835265683629213,11.5876793312944,
48.5199317919394));
#29494=CARTESIAN_POINT('Ctrl Pts',(0.0835265683637358,11.5731362269332,
48.5213546907495));
#29495=CARTESIAN_POINT('Ctrl Pts',(0.0835265683659855,11.5200575082527,
48.5195892904601));
#29496=CARTESIAN_POINT('Ctrl Pts',(0.0835265683646867,11.4942063411577,
48.5199465324602));
#29497=CARTESIAN_POINT('Ctrl Pts',(0.0835265683646154,11.4728541727075,
48.5199460669665));
#29498=CARTESIAN_POINT('',(4.29256572406856,11.6756605346477,48.4959174087471));
#29499=CARTESIAN_POINT('Ctrl Pts',(4.28505819640497,11.7955954176945,48.5199317919394));
#29500=CARTESIAN_POINT('Ctrl Pts',(4.28563987788572,11.7889074035727,48.5199317866933));
#29501=CARTESIAN_POINT('Ctrl Pts',(4.2862286391617,11.7811426004669,48.51971728124));
#29502=CARTESIAN_POINT('Ctrl Pts',(4.28683031455212,11.7724551591809,48.5190688938798));
#29503=CARTESIAN_POINT('Ctrl Pts',(4.28737989743217,11.7645198686933,48.5184766433099));
#29504=CARTESIAN_POINT('Ctrl Pts',(4.28794027744316,11.7558145072651,48.5175204898844));
#29505=CARTESIAN_POINT('Ctrl Pts',(4.28851223325202,11.746498740511,48.516032617158));
#29506=CARTESIAN_POINT('Ctrl Pts',(4.2890564340326,11.7376350355518,48.5146169457257));
#29507=CARTESIAN_POINT('Ctrl Pts',(4.28961108824049,11.7282190174497,48.5127184771679));
#29508=CARTESIAN_POINT('Ctrl Pts',(4.29017342238365,11.7184280696926,48.510215157354));
#29509=CARTESIAN_POINT('Ctrl Pts',(4.29070902472487,11.7091025563741,48.5078308384051));
#29510=CARTESIAN_POINT('Ctrl Pts',(4.2912515217908,11.6994377386552,48.5048968999018));
#29511=CARTESIAN_POINT('Ctrl Pts',(4.29179604392015,11.6896156896679,48.5013453462893));
#29512=CARTESIAN_POINT('Ctrl Pts',(4.29205239342601,11.6849916766688,48.4996733499378));
#29513=CARTESIAN_POINT('Ctrl Pts',(4.29230916168589,11.6803331677637,48.4978651076034));
#29514=CARTESIAN_POINT('Ctrl Pts',(4.29256572165175,11.675660562453,48.4959173417252));
#29515=CARTESIAN_POINT('Ctrl Pts',(4.29256572527696,11.6756605207451,48.4959174422581));
#29516=CARTESIAN_POINT('Ctrl Pts',(3.59085027393415,11.6392592214975,48.506118103167));
#29517=CARTESIAN_POINT('Ctrl Pts',(2.88857791675096,11.598649286609,48.5108119661593));
#29518=CARTESIAN_POINT('Ctrl Pts',(1.48700388586174,11.5098560202884,48.5141172996824));
#29519=CARTESIAN_POINT('Ctrl Pts',(0.78561717894128,11.4835302569325,48.5199462997137));
#29520=CARTESIAN_POINT('Ctrl Pts',(0.0835265683646154,11.4728541727075,
48.5199460669665));
#29521=CARTESIAN_POINT('Ctrl Pts',(0.0835265683646154,11.4728541727075,
48.5199460669665));
#29522=CARTESIAN_POINT('Ctrl Pts',(0.434571873652913,11.4675161305949,48.5199459505932));
#29523=CARTESIAN_POINT('Ctrl Pts',(0.785669116598665,11.4659265087691,48.5184885224499));
#29524=CARTESIAN_POINT('Ctrl Pts',(1.48799468015646,11.464396632877,48.5087577020976));
#29525=CARTESIAN_POINT('Ctrl Pts',(1.83922300076851,11.4644563788108,48.5004843098885));
#29526=CARTESIAN_POINT('Ctrl Pts',(2.89314538263116,11.4583384590299,48.4595881763738));
#29527=CARTESIAN_POINT('Ctrl Pts',(3.59439815510967,11.4609474762041,48.4163876002293));
#29528=CARTESIAN_POINT('Ctrl Pts',(4.29550794737987,11.4732422824941,48.3603316468569));
#29529=CARTESIAN_POINT('Ctrl Pts',(0.434571873652948,11.47819221482,48.5199461833401));
#29530=CARTESIAN_POINT('Ctrl Pts',(0.707588293934062,11.474986089803,48.5190043349166));
#29531=CARTESIAN_POINT('Ctrl Pts',(0.998676156497516,11.4745419834778,48.5169166777059));
#29532=CARTESIAN_POINT('Ctrl Pts',(1.6137782469759,11.4744825705815,48.5070409830049));
#29533=CARTESIAN_POINT('Ctrl Pts',(1.93779750982841,11.4748353413217,48.4992338111971));
#29534=CARTESIAN_POINT('Ctrl Pts',(2.9544266533864,11.4700074930207,48.4591554550249));
#29535=CARTESIAN_POINT('Ctrl Pts',(3.63137389791096,11.4731609516944,48.4176356670413));
#29536=CARTESIAN_POINT('Ctrl Pts',(4.29556063459987,11.4851966459098,48.3652975204339));
#29537=CARTESIAN_POINT('Ctrl Pts',(0.78544120302723,11.4874426767152,48.5184889915191));
#29538=CARTESIAN_POINT('Ctrl Pts',(0.998330962591659,11.484480312248,48.5172889554747));
#29539=CARTESIAN_POINT('Ctrl Pts',(1.24336152271846,11.4840908039498,48.514900881629));
#29540=CARTESIAN_POINT('Ctrl Pts',(1.78770682159394,11.4843329006938,48.5050013605299));
#29541=CARTESIAN_POINT('Ctrl Pts',(2.08702911274898,11.4849166217029,48.4974612118004));
#29542=CARTESIAN_POINT('Ctrl Pts',(3.05143599908222,11.4818828006799,48.4585450693865));
#29543=CARTESIAN_POINT('Ctrl Pts',(3.69355131246621,11.4863352799679,48.4189800886588));
#29544=CARTESIAN_POINT('Ctrl Pts',(4.29569371583977,11.497472006951,48.3719827330256));
#29545=CARTESIAN_POINT('Ctrl Pts',(1.48685396299278,11.5143737377395,48.5151613829998));
#29546=CARTESIAN_POINT('Ctrl Pts',(1.61221600332869,11.5105174196343,48.5134046445916));
#29547=CARTESIAN_POINT('Ctrl Pts',(1.78640027442033,11.5090816899187,48.5103147764347));
#29548=CARTESIAN_POINT('Ctrl Pts',(2.21034412033182,11.5079260458442,48.4999506929245));
#29549=CARTESIAN_POINT('Ctrl Pts',(2.4601131356596,11.5081462764441,48.4926406007259));
#29550=CARTESIAN_POINT('Ctrl Pts',(3.28969174892232,11.5065304546904,48.456544560029));
#29551=CARTESIAN_POINT('Ctrl Pts',(3.8387134471824,11.5121367174565,48.4216081073346));
#29552=CARTESIAN_POINT('Ctrl Pts',(4.29625434599571,11.5208685373805,48.3864516772668));
#29553=CARTESIAN_POINT('Ctrl Pts',(1.83739739358405,11.5320543368685,48.5132909663016));
#29554=CARTESIAN_POINT('Ctrl Pts',(1.93535675584129,11.5270830007426,48.5112385621713));
#29555=CARTESIAN_POINT('Ctrl Pts',(2.08475123055101,11.5245577996658,48.5077487408488));
#29556=CARTESIAN_POINT('Ctrl Pts',(2.45904980776384,11.5217114161952,48.4969449897084));
#29557=CARTESIAN_POINT('Ctrl Pts',(2.68396272140769,11.5213343690961,48.489597574835));
#29558=CARTESIAN_POINT('Ctrl Pts',(3.43093653349979,11.5193254972085,48.455157285331));
#29559=CARTESIAN_POINT('Ctrl Pts',(3.92169816734333,11.5247638266718,48.4228917043929));
#29560=CARTESIAN_POINT('Ctrl Pts',(4.29668189491177,11.5319897067687,48.3942354089164));
#29561=CARTESIAN_POINT('Ctrl Pts',(2.88857791675096,11.598649286609,48.5108119661593));
#29562=CARTESIAN_POINT('Ctrl Pts',(2.9488036240303,11.5919036248663,48.507599134787));
#29563=CARTESIAN_POINT('Ctrl Pts',(3.0457795460293,11.5859418512212,48.5025662258368));
#29564=CARTESIAN_POINT('Ctrl Pts',(3.28508025551021,11.5755468354636,48.4895414183257));
#29565=CARTESIAN_POINT('Ctrl Pts',(3.42741007792968,11.5710816706623,48.4815303854473));
#29566=CARTESIAN_POINT('Ctrl Pts',(3.8802020832709,11.5598336028535,48.4510874244428));
#29567=CARTESIAN_POINT('Ctrl Pts',(4.15746922938128,11.5581209387927,48.4262709574734));
#29568=CARTESIAN_POINT('Ctrl Pts',(4.29860676262873,11.5609276470972,48.4157241439942));
#29569=CARTESIAN_POINT('Ctrl Pts',(3.59085027393415,11.6392592214975,48.506118103167));
#29570=CARTESIAN_POINT('Ctrl Pts',(3.62682139908161,11.6298708101994,48.5021196906978));
#29571=CARTESIAN_POINT('Ctrl Pts',(3.68879009436557,11.6209827896646,48.4962278199978));
#29572=CARTESIAN_POINT('Ctrl Pts',(3.83438595526553,11.6050189470302,48.4820050859842));
#29573=CARTESIAN_POINT('Ctrl Pts',(3.91801312088154,11.5979431249305,48.4736742226707));
#29574=CARTESIAN_POINT('Ctrl Pts',(4.15587731831616,11.5806510816468,48.447045029582));
#29575=CARTESIAN_POINT('Ctrl Pts',(4.29707247281346,11.5743267261738,48.4278950754016));
#29576=CARTESIAN_POINT('Ctrl Pts',(4.30074630239845,11.5743188502015,48.4275666875517));
#29577=CARTESIAN_POINT('Ctrl Pts',(4.29256572527697,11.6756605207451,48.4959174422581));
#29578=CARTESIAN_POINT('Ctrl Pts',(4.29322407515183,11.6636703105801,48.4909193590355));
#29579=CARTESIAN_POINT('Ctrl Pts',(4.29389281459049,11.6514649415886,48.4847891628829));
#29580=CARTESIAN_POINT('Ctrl Pts',(4.29532858886799,11.6282480883359,48.4713889284475));
#29581=CARTESIAN_POINT('Ctrl Pts',(4.29609562370683,11.6172366040747,48.4641188901648));
#29582=CARTESIAN_POINT('Ctrl Pts',(4.29866044573254,11.588429281961,48.4422855877167));
#29583=CARTESIAN_POINT('Ctrl Pts',(4.30071410004355,11.5746245276893,48.4278763391902));
#29584=CARTESIAN_POINT('Ctrl Pts',(4.30427685533877,11.5746245485738,48.4275653153946));
#29585=CARTESIAN_POINT('Ctrl Pts',(4.29256572527696,11.6756605207451,48.4959174422581));
#29586=CARTESIAN_POINT('Ctrl Pts',(4.2938824250267,11.6516801004151,48.485921275813));
#29587=CARTESIAN_POINT('Ctrl Pts',(4.29524068303159,11.6268390447792,48.4713966576475));
#29588=CARTESIAN_POINT('Ctrl Pts',(4.29866044573254,11.588429281961,48.4422855877167));
#29589=CARTESIAN_POINT('Ctrl Pts',(4.30071410004355,11.5746245276893,48.4278763391902));
#29590=CARTESIAN_POINT('Ctrl Pts',(4.30427685533877,11.5746245485738,48.4275653153946));
#29591=CARTESIAN_POINT('',(4.29550794737987,11.4732422824942,48.360331646857));
#29592=CARTESIAN_POINT('Ctrl Pts',(4.30427685533877,11.5746245485738,48.4275653153946));
#29593=CARTESIAN_POINT('Ctrl Pts',(4.29721574945814,11.5740131518292,48.4275680597088));
#29594=CARTESIAN_POINT('Ctrl Pts',(4.29571869625989,11.5210597361567,48.3801951411647));
#29595=CARTESIAN_POINT('Ctrl Pts',(4.29550794737987,11.4732422824942,48.360331646857));
#29596=CARTESIAN_POINT('Ctrl Pts',(4.29550794737987,11.4732422824942,48.360331646857));
#29597=CARTESIAN_POINT('Ctrl Pts',(3.59439815510967,11.4609474762041,48.4163876002292));
#29598=CARTESIAN_POINT('Ctrl Pts',(2.89314538263116,11.4583384590299,48.4595881763737));
#29599=CARTESIAN_POINT('Ctrl Pts',(1.48791554014763,11.4664956854044,48.5141163543934));
#29600=CARTESIAN_POINT('Ctrl Pts',(0.785617178941208,11.4621780884822,48.5199458342199));
#29601=CARTESIAN_POINT('Ctrl Pts',(0.0835265683646154,11.4728541727075,
48.5199460669665));
#29602=CARTESIAN_POINT('Ctrl Pts',(0.0835265683646154,11.4728541727075,
48.5199460669665));
#29603=CARTESIAN_POINT('Ctrl Pts',(0.0835265683645438,11.4515020042572,
48.5199456014727));
#29604=CARTESIAN_POINT('Ctrl Pts',(0.0835265683631205,11.4284235901226,
48.5195872927698));
#29605=CARTESIAN_POINT('Ctrl Pts',(0.0835265683628376,11.3941472536996,
48.5154826406219));
#29606=CARTESIAN_POINT('Ctrl Pts',(0.0835265683627773,11.3720285904897,
48.5199317919394));
#29607=CARTESIAN_POINT('Ctrl Pts',(0.0835265683619676,11.353653679453,48.5199317919394));
#29608=CARTESIAN_POINT('Ctrl Pts',(0.434571873652913,11.4675161305949,48.5199459505932));
#29609=CARTESIAN_POINT('Ctrl Pts',(0.356716052822661,11.4488974993902,48.51988591043));
#29610=CARTESIAN_POINT('Ctrl Pts',(0.339530012993789,11.4285976962987,48.5196215918845));
#29611=CARTESIAN_POINT('Ctrl Pts',(0.361332410433279,11.3940705712691,48.5154600081738));
#29612=CARTESIAN_POINT('Ctrl Pts',(0.400320847700618,11.3720285904897,48.5199317919394));
#29613=CARTESIAN_POINT('Ctrl Pts',(0.434813981059838,11.353653679453,48.5199317919394));
#29614=CARTESIAN_POINT('Ctrl Pts',(0.785669116598665,11.4659265087691,48.5184885224499));
#29615=CARTESIAN_POINT('Ctrl Pts',(0.652301278511543,11.447718516688,48.5186918880708));
#29616=CARTESIAN_POINT('Ctrl Pts',(0.626534465182239,11.428587933622,48.5182575867036));
#29617=CARTESIAN_POINT('Ctrl Pts',(0.667559641505308,11.3934281614349,48.5133469042742));
#29618=CARTESIAN_POINT('Ctrl Pts',(0.734351631156823,11.3718199008203,48.5168141308044));
#29619=CARTESIAN_POINT('Ctrl Pts',(0.786101399028862,11.353653679453,48.5161104362146));
#29620=CARTESIAN_POINT('Ctrl Pts',(1.48799468015646,11.464396632877,48.5087577020976));
#29621=CARTESIAN_POINT('Ctrl Pts',(1.29495517067291,11.4452664260876,48.5103258778886));
#29622=CARTESIAN_POINT('Ctrl Pts',(1.26276365300082,11.4271829834973,48.5091673912096));
#29623=CARTESIAN_POINT('Ctrl Pts',(1.32724155706699,11.39130385313,48.5020950494664));
#29624=CARTESIAN_POINT('Ctrl Pts',(1.42391097880467,11.3711415135622,48.5026532295396));
#29625=CARTESIAN_POINT('Ctrl Pts',(1.48859334813903,11.353653679453,48.50082319184));
#29626=CARTESIAN_POINT('Ctrl Pts',(1.83922300076851,11.4644563788108,48.5004843098885));
#29627=CARTESIAN_POINT('Ctrl Pts',(1.64203235159374,11.443938017789,48.5030276183437));
#29628=CARTESIAN_POINT('Ctrl Pts',(1.61199486709086,11.425732495649,48.5013148775259));
#29629=CARTESIAN_POINT('Ctrl Pts',(1.68069642943966,11.389794304459,48.4928930593065));
#29630=CARTESIAN_POINT('Ctrl Pts',(1.7794354762909,11.3706718159735,48.491609885926));
#29631=CARTESIAN_POINT('Ctrl Pts',(1.83979788982311,11.353653679453,48.489357302818));
#29632=CARTESIAN_POINT('Ctrl Pts',(2.54183792201028,11.4603777656235,48.4732202208787));
#29633=CARTESIAN_POINT('Ctrl Pts',(2.39436890042523,11.4381382649983,48.4746917382113));
#29634=CARTESIAN_POINT('Ctrl Pts',(2.37286182154143,11.4203247666438,48.4721918658361));
#29635=CARTESIAN_POINT('Ctrl Pts',(2.42513999639859,11.3861758639155,48.4637155121672));
#29636=CARTESIAN_POINT('Ctrl Pts',(2.49892525013932,11.3696277842964,48.4610292841198));
#29637=CARTESIAN_POINT('Ctrl Pts',(2.54204089380268,11.353653679453,48.4587755322629));
#29638=CARTESIAN_POINT('Ctrl Pts',(2.89280484544034,11.4600103666203,48.4556040545901));
#29639=CARTESIAN_POINT('Ctrl Pts',(2.76993041129963,11.4370088609558,48.4559496852932));
#29640=CARTESIAN_POINT('Ctrl Pts',(2.75490259059407,11.4187667259072,48.4528734061814));
#29641=CARTESIAN_POINT('Ctrl Pts',(2.80138061725977,11.3847952022384,48.4445443128281));
#29642=CARTESIAN_POINT('Ctrl Pts',(2.86288646463088,11.369053450208,48.4414922321744));
#29643=CARTESIAN_POINT('Ctrl Pts',(2.89307936664307,11.353653679453,48.439659649984));
#29644=CARTESIAN_POINT('Ctrl Pts',(3.59436241005759,11.4633689234831,48.4131737559223));
#29645=CARTESIAN_POINT('Ctrl Pts',(3.52670827169875,11.4394032486783,48.4096766577646));
#29646=CARTESIAN_POINT('Ctrl Pts',(3.5225115642211,11.4193327724023,48.4051808771548));
#29647=CARTESIAN_POINT('Ctrl Pts',(3.55227792535516,11.3835624194323,48.3973032871378));
#29648=CARTESIAN_POINT('Ctrl Pts',(3.58624099396685,11.3679565169509,48.3944770846954));
#29649=CARTESIAN_POINT('Ctrl Pts',(3.59490640778659,11.353653679453,48.3937688119853));
#29650=CARTESIAN_POINT('Ctrl Pts',(3.94495305124477,11.4670948793491,48.3883596235431));
#29651=CARTESIAN_POINT('Ctrl Pts',(3.90792462122347,11.4429270404433,48.3821456831541));
#29652=CARTESIAN_POINT('Ctrl Pts',(3.90807774441525,11.4214568596339,48.3768070662869));
#29653=CARTESIAN_POINT('Ctrl Pts',(3.9269305664659,11.3837102983034,48.3692339775144));
#29654=CARTESIAN_POINT('Ctrl Pts',(3.94563026532478,11.3674339177823,48.3669995056091));
#29655=CARTESIAN_POINT('Ctrl Pts',(3.94569498663766,11.353653679453,48.3669938551438));
#29656=CARTESIAN_POINT('Ctrl Pts',(4.29550794737987,11.4732422824941,48.3603316468569));
#29657=CARTESIAN_POINT('Ctrl Pts',(4.29540257293986,11.4493335556629,48.3503998997031));
#29658=CARTESIAN_POINT('Ctrl Pts',(4.29560464263433,11.4261172510677,48.3444127441005));
#29659=CARTESIAN_POINT('Ctrl Pts',(4.29606146924328,11.384958159128,48.3374043064722));
#29660=CARTESIAN_POINT('Ctrl Pts',(4.29631622615776,11.3670153717833,48.3363830244465));
#29661=CARTESIAN_POINT('Ctrl Pts',(4.29631622615776,11.353653679453,48.3363830244465));
#29662=CARTESIAN_POINT('Ctrl Pts',(4.29550794737987,11.4732422824942,48.360331646857));
#29663=CARTESIAN_POINT('Ctrl Pts',(4.29546091471024,11.4625708971931,48.3558987257173));
#29664=CARTESIAN_POINT('Ctrl Pts',(4.29547085992706,11.4520014357867,48.3522029429309));
#29665=CARTESIAN_POINT('Ctrl Pts',(4.29551799962758,11.4417444398151,48.3491738175902));
#29666=CARTESIAN_POINT('Ctrl Pts',(4.29556841690108,11.4307742858786,48.3459340804028));
#29667=CARTESIAN_POINT('Ctrl Pts',(4.29566133560236,11.420162601422,48.3434563976416));
#29668=CARTESIAN_POINT('Ctrl Pts',(4.29576766490653,11.4101434346418,48.341598642047));
#29669=CARTESIAN_POINT('Ctrl Pts',(4.29588042424243,11.3995183806997,48.3396285427527));
#29670=CARTESIAN_POINT('Ctrl Pts',(4.29600813145325,11.3895604073049,48.338354073489));
#29671=CARTESIAN_POINT('Ctrl Pts',(4.29611218230524,11.3805081454716,48.3375612325113));
#29672=CARTESIAN_POINT('Ctrl Pts',(4.29622934837385,11.3703148802493,48.3366684569251));
#29673=CARTESIAN_POINT('Ctrl Pts',(4.29631622615776,11.3612705067707,48.3363830244465));
#29674=CARTESIAN_POINT('Ctrl Pts',(4.29631622615776,11.353653679453,48.3363830244465));
#29675=CARTESIAN_POINT('Ctrl Pts',(0.0835265683619891,11.353653679453,48.5199317919394));
#29676=CARTESIAN_POINT('Ctrl Pts',(0.0835265683627773,11.3720285904897,
48.5199317919394));
#29677=CARTESIAN_POINT('Ctrl Pts',(0.0835265683628376,11.3941472536996,
48.5154826406219));
#29678=CARTESIAN_POINT('Ctrl Pts',(0.0835265683631205,11.4284235901226,
48.5195872927698));
#29679=CARTESIAN_POINT('Ctrl Pts',(0.0835265683645438,11.4515020042572,
48.5199456014727));
#29680=CARTESIAN_POINT('Ctrl Pts',(0.0835265683646154,11.4728541727075,
48.5199460669665));
#29681=CARTESIAN_POINT('Ctrl Pts',(0.0835265683646154,11.4728541727075,
48.5199460669665));
#29682=CARTESIAN_POINT('Ctrl Pts',(-0.267518736923717,11.4675161305949,
48.5199459505928));
#29683=CARTESIAN_POINT('Ctrl Pts',(-0.61861597986895,11.4659265087692,48.5184885224493));
#29684=CARTESIAN_POINT('Ctrl Pts',(-1.32094154342462,11.4643966328772,48.5087577020968));
#29685=CARTESIAN_POINT('Ctrl Pts',(-1.67216986403505,11.4644563788108,48.5004843098878));
#29686=CARTESIAN_POINT('Ctrl Pts',(-2.37478478527252,11.4603777656235,48.4732202208791));
#29687=CARTESIAN_POINT('Ctrl Pts',(-2.72575170870462,11.4600103666202,48.4556040545906));
#29688=CARTESIAN_POINT('Ctrl Pts',(-3.4273092733279,11.463368923483,48.4131737559227));
#29689=CARTESIAN_POINT('Ctrl Pts',(-3.77789991451908,11.4670948793491,48.3883596235432));
#29690=CARTESIAN_POINT('Ctrl Pts',(-4.12845481065596,11.4732422824942,48.3603316468569));
#29691=CARTESIAN_POINT('Ctrl Pts',(0.0835265683645438,11.4515020042572,
48.5199456014727));
#29692=CARTESIAN_POINT('Ctrl Pts',(-0.189662916093927,11.4488974993903,
48.5198859104297));
#29693=CARTESIAN_POINT('Ctrl Pts',(-0.485248141782668,11.4477185166882,
48.5186918880704));
#29694=CARTESIAN_POINT('Ctrl Pts',(-1.12790203394243,11.4452664260878,48.5103258778881));
#29695=CARTESIAN_POINT('Ctrl Pts',(-1.47497921486181,11.4439380177892,48.5030276183433));
#29696=CARTESIAN_POINT('Ctrl Pts',(-2.22731576368872,11.4381382649983,48.4746917382118));
#29697=CARTESIAN_POINT('Ctrl Pts',(-2.60287727456489,11.4370088609558,48.4559496852938));
#29698=CARTESIAN_POINT('Ctrl Pts',(-3.35965513496952,11.4394032486783,48.409676657765));
#29699=CARTESIAN_POINT('Ctrl Pts',(-3.74087148449797,11.4429270404433,48.3821456831542));
#29700=CARTESIAN_POINT('Ctrl Pts',(-4.12834943621596,11.4493335556629,48.3503998997031));
#29701=CARTESIAN_POINT('Ctrl Pts',(0.0835265683631205,11.4284235901226,
48.5195872927698));
#29702=CARTESIAN_POINT('Ctrl Pts',(-0.172476876267548,11.4285976962988,
48.5196215918844));
#29703=CARTESIAN_POINT('Ctrl Pts',(-0.459481328455685,11.4285879336221,
48.5182575867033));
#29704=CARTESIAN_POINT('Ctrl Pts',(-1.0957105162727,11.4271829834975,48.5091673912093));
#29705=CARTESIAN_POINT('Ctrl Pts',(-1.44494173036149,11.4257324956491,48.5013148775256));
#29706=CARTESIAN_POINT('Ctrl Pts',(-2.20580868480827,11.4203247666438,48.4721918658365));
#29707=CARTESIAN_POINT('Ctrl Pts',(-2.58784945386211,11.4187667259072,48.4528734061819));
#29708=CARTESIAN_POINT('Ctrl Pts',(-3.35545842749311,11.4193327724023,48.4051808771551));
#29709=CARTESIAN_POINT('Ctrl Pts',(-3.74102460769006,11.4214568596339,48.376807066287));
#29710=CARTESIAN_POINT('Ctrl Pts',(-4.12855150591043,11.4261172510678,48.3444127441005));
#29711=CARTESIAN_POINT('Ctrl Pts',(0.0835265683628376,11.3941472536996,
48.5154826406219));
#29712=CARTESIAN_POINT('Ctrl Pts',(-0.194279273707604,11.3940705712692,
48.5154600081738));
#29713=CARTESIAN_POINT('Ctrl Pts',(-0.500506504779572,11.393428161435,48.5133469042742));
#29714=CARTESIAN_POINT('Ctrl Pts',(-1.16018842034084,11.39130385313,48.5020950494664));
#29715=CARTESIAN_POINT('Ctrl Pts',(-1.51364329271317,11.3897943044591,48.4928930593065));
#29716=CARTESIAN_POINT('Ctrl Pts',(-2.25808685967095,11.3861758639155,48.4637155121674));
#29717=CARTESIAN_POINT('Ctrl Pts',(-2.6343274805326,11.3847952022384,48.4445443128283));
#29718=CARTESIAN_POINT('Ctrl Pts',(-3.38522478862952,11.3835624194324,48.3973032871379));
#29719=CARTESIAN_POINT('Ctrl Pts',(-3.75987742974135,11.3837102983034,48.3692339775145));
#29720=CARTESIAN_POINT('Ctrl Pts',(-4.12900833251936,11.384958159128,48.3374043064722));
#29721=CARTESIAN_POINT('Ctrl Pts',(0.0835265683627773,11.3720285904897,
48.5199317919394));
#29722=CARTESIAN_POINT('Ctrl Pts',(-0.233267710975063,11.3720285904897,
48.5199317919394));
#29723=CARTESIAN_POINT('Ctrl Pts',(-0.567298494431303,11.3718199008203,
48.5168141308044));
#29724=CARTESIAN_POINT('Ctrl Pts',(-1.25685784207929,11.3711415135622,48.5026532295397));
#29725=CARTESIAN_POINT('Ctrl Pts',(-1.61238233956562,11.3706718159735,48.491609885926));
#29726=CARTESIAN_POINT('Ctrl Pts',(-2.33187211341431,11.3696277842964,48.4610292841198));
#29727=CARTESIAN_POINT('Ctrl Pts',(-2.69583332790602,11.369053450208,48.4414922321744));
#29728=CARTESIAN_POINT('Ctrl Pts',(-3.41918785724238,11.3679565169509,48.3944770846954));
#29729=CARTESIAN_POINT('Ctrl Pts',(-3.77857712860057,11.3674339177823,48.3669995056091));
#29730=CARTESIAN_POINT('Ctrl Pts',(-4.12926308943382,11.3670153717833,48.3363830244465));
#29731=CARTESIAN_POINT('Ctrl Pts',(0.0835265683619676,11.353653679453,48.5199317919394));
#29732=CARTESIAN_POINT('Ctrl Pts',(-0.267760844335902,11.353653679453,48.5199317919394));
#29733=CARTESIAN_POINT('Ctrl Pts',(-0.619048262304927,11.3536536794531,
48.5161104362146));
#29734=CARTESIAN_POINT('Ctrl Pts',(-1.32154021141509,11.3536536794531,48.50082319184));
#29735=CARTESIAN_POINT('Ctrl Pts',(-1.67274475309917,11.3536536794531,48.489357302818));
#29736=CARTESIAN_POINT('Ctrl Pts',(-2.37498775707875,11.3536536794531,48.4587755322629));
#29737=CARTESIAN_POINT('Ctrl Pts',(-2.72602622991912,11.3536536794531,48.439659649984));
#29738=CARTESIAN_POINT('Ctrl Pts',(-3.42785327106262,11.3536536794531,48.3937688119853));
#29739=CARTESIAN_POINT('Ctrl Pts',(-3.77864184991372,11.3536536794531,48.3669938551438));
#29740=CARTESIAN_POINT('Ctrl Pts',(-4.12926308943382,11.3536536794531,48.3363830244465));
#29741=CARTESIAN_POINT('',(-4.12845481065596,11.4732422824942,48.360331646857));
#29742=CARTESIAN_POINT('Ctrl Pts',(-4.12926308943382,11.3536536794531,48.3363830244465));
#29743=CARTESIAN_POINT('Ctrl Pts',(-4.12926308943382,11.3608560447969,48.3363830244465));
#29744=CARTESIAN_POINT('Ctrl Pts',(-4.12918541418972,11.3693343502548,48.3366383003061));
#29745=CARTESIAN_POINT('Ctrl Pts',(-4.12907789424658,11.3788543868427,48.3374208419226));
#29746=CARTESIAN_POINT('Ctrl Pts',(-4.1289785687574,11.3876488696476,48.338143743429));
#29747=CARTESIAN_POINT('Ctrl Pts',(-4.12885398245303,11.3973323098416,48.339318986334));
#29748=CARTESIAN_POINT('Ctrl Pts',(-4.12874104374852,11.4076804802594,48.3411521533193));
#29749=CARTESIAN_POINT('Ctrl Pts',(-4.12863183371979,11.4176870054229,48.3429247982243));
#29750=CARTESIAN_POINT('Ctrl Pts',(-4.12853365126042,11.428314631214,48.3453142106815));
#29751=CARTESIAN_POINT('Ctrl Pts',(-4.12847668203915,11.4393255986458,48.3484700316399));
#29752=CARTESIAN_POINT('Ctrl Pts',(-4.12842391816255,11.4495237602834,48.3513928967225));
#29753=CARTESIAN_POINT('Ctrl Pts',(-4.1284065446436,11.460049829507,48.354973634109));
#29754=CARTESIAN_POINT('Ctrl Pts',(-4.12844464232628,11.4706948755439,48.3592865236346));
#29755=CARTESIAN_POINT('Ctrl Pts',(-4.12844767875758,11.4715432985642,48.3596302661365));
#29756=CARTESIAN_POINT('Ctrl Pts',(-4.12845106522601,11.4723924705143,48.3599786327558));
#29757=CARTESIAN_POINT('Ctrl Pts',(-4.12845481065596,11.4732422824942,48.3603316468569));
#29758=CARTESIAN_POINT('Ctrl Pts',(-4.12845481065596,11.4732422824942,48.360331646857));
#29759=CARTESIAN_POINT('Ctrl Pts',(-3.4273450183822,11.4609474762041,48.4163876002295));
#29760=CARTESIAN_POINT('Ctrl Pts',(-2.72609224589126,11.4583384590298,48.4595881763747));
#29761=CARTESIAN_POINT('Ctrl Pts',(-1.32086240341632,11.4664956854045,48.5141163543922));
#29762=CARTESIAN_POINT('Ctrl Pts',(-0.618564042212051,11.4621780884824,
48.5199458342193));
#29763=CARTESIAN_POINT('Ctrl Pts',(0.0835265683646154,11.4728541727075,
48.5199460669665));
#29764=CARTESIAN_POINT('Ctrl Pts',(0.0835265683646154,11.4728541727075,
48.5199460669665));
#29765=CARTESIAN_POINT('Ctrl Pts',(-0.267518736923682,11.47819221482,48.5199461833397));
#29766=CARTESIAN_POINT('Ctrl Pts',(-0.618388066296979,11.4874426767151,
48.5184889915183));
#29767=CARTESIAN_POINT('Ctrl Pts',(-1.31980082625865,11.5143737377389,48.5151613829986));
#29768=CARTESIAN_POINT('Ctrl Pts',(-1.67034425684702,11.5320543368675,48.5132909663004));
#29769=CARTESIAN_POINT('Ctrl Pts',(-2.72152478000237,11.5986492866067,48.5108119661587));
#29770=CARTESIAN_POINT('Ctrl Pts',(-3.42379713716555,11.6392592214936,48.5061181031666));
#29771=CARTESIAN_POINT('Ctrl Pts',(-4.12551258849121,11.6756605207398,48.4959174422581));
#29772=CARTESIAN_POINT('Ctrl Pts',(-0.267518736923717,11.4675161305949,
48.5199459505928));
#29773=CARTESIAN_POINT('Ctrl Pts',(-0.540535157204295,11.4749860898031,
48.5190043349159));
#29774=CARTESIAN_POINT('Ctrl Pts',(-0.831277825861035,11.4844803122479,
48.5172889554738));
#29775=CARTESIAN_POINT('Ctrl Pts',(-1.44516286659434,11.5105174196336,48.5134046445902));
#29776=CARTESIAN_POINT('Ctrl Pts',(-1.76830361910408,11.5270830007414,48.5112385621698));
#29777=CARTESIAN_POINT('Ctrl Pts',(-2.78175048727934,11.5919036248635,48.5075991347862));
#29778=CARTESIAN_POINT('Ctrl Pts',(-3.45976826230679,11.6298708101947,48.5021196906972));
#29779=CARTESIAN_POINT('Ctrl Pts',(-4.12617093834983,11.6636703105734,48.4909193590356));
#29780=CARTESIAN_POINT('Ctrl Pts',(-0.61861597986895,11.4659265087692,48.5184885224493));
#29781=CARTESIAN_POINT('Ctrl Pts',(-0.831623019767032,11.4745419834779,
48.5169166777051));
#29782=CARTESIAN_POINT('Ctrl Pts',(-1.07630838598628,11.4840908039496,48.5149008816279));
#29783=CARTESIAN_POINT('Ctrl Pts',(-1.6193471376818,11.5090816899177,48.5103147764332));
#29784=CARTESIAN_POINT('Ctrl Pts',(-1.91769809380781,11.5245577996642,48.5077487408472));
#29785=CARTESIAN_POINT('Ctrl Pts',(-2.87872640926596,11.5859418512174,48.5025662258359));
#29786=CARTESIAN_POINT('Ctrl Pts',(-3.52173695757365,11.6209827896584,48.496227819997));
#29787=CARTESIAN_POINT('Ctrl Pts',(-4.12683967776745,11.6514649415801,48.4847891628829));
#29788=CARTESIAN_POINT('Ctrl Pts',(-1.32094154342462,11.4643966328772,48.5087577020968));
#29789=CARTESIAN_POINT('Ctrl Pts',(-1.4467251102432,11.4744825705815,48.507040983004));
#29790=CARTESIAN_POINT('Ctrl Pts',(-1.6206536848576,11.4843329006934,48.5050013605288));
#29791=CARTESIAN_POINT('Ctrl Pts',(-2.04329098358324,11.5079260458424,48.499950692923));
#29792=CARTESIAN_POINT('Ctrl Pts',(-2.29199667100668,11.5217114161924,48.4969449897068));
#29793=CARTESIAN_POINT('Ctrl Pts',(-3.1180271187208,11.5755468354576,48.4895414183245));
#29794=CARTESIAN_POINT('Ctrl Pts',(-3.66733281844084,11.6050189470212,48.4820050859833));
#29795=CARTESIAN_POINT('Ctrl Pts',(-4.12827545201166,11.6282480883245,48.4713889284476));
#29796=CARTESIAN_POINT('Ctrl Pts',(-1.67216986403505,11.4644563788108,48.5004843098878));
#29797=CARTESIAN_POINT('Ctrl Pts',(-1.7707443730942,11.4748353413217,48.4992338111963));
#29798=CARTESIAN_POINT('Ctrl Pts',(-1.91997597601002,11.4849166217024,48.4974612117994));
#29799=CARTESIAN_POINT('Ctrl Pts',(-2.29305999890518,11.5081462764419,48.4926406007247));
#29800=CARTESIAN_POINT('Ctrl Pts',(-2.51690958464257,11.5213343690928,48.4895975748336));
#29801=CARTESIAN_POINT('Ctrl Pts',(-3.2603569411266,11.5710816706553,48.4815303854461));
#29802=CARTESIAN_POINT('Ctrl Pts',(-3.75095998404117,11.5979431249203,48.4736742226698));
#29803=CARTESIAN_POINT('Ctrl Pts',(-4.12904248683824,11.6172366040622,48.4641188901649));
#29804=CARTESIAN_POINT('Ctrl Pts',(-2.72609224589126,11.4583384590298,48.4595881763747));
#29805=CARTESIAN_POINT('Ctrl Pts',(-2.78737351664595,11.4700074930205,48.4591554550258));
#29806=CARTESIAN_POINT('Ctrl Pts',(-2.88438286233575,11.4818828006791,48.4585450693872));
#29807=CARTESIAN_POINT('Ctrl Pts',(-3.12263861215733,11.5065304546877,48.4565445600294));
#29808=CARTESIAN_POINT('Ctrl Pts',(-3.26388339672229,11.5193254972046,48.4551572853311));
#29809=CARTESIAN_POINT('Ctrl Pts',(-3.71314894645291,11.5598336028455,48.4510874244425));
#29810=CARTESIAN_POINT('Ctrl Pts',(-3.98882418146572,11.5806510816358,48.4470450295816));
#29811=CARTESIAN_POINT('Ctrl Pts',(-4.13160730886785,11.5884292819489,48.4422855877167));
#29812=CARTESIAN_POINT('Ctrl Pts',(-3.4273450183822,11.4609474762041,48.4163876002295));
#29813=CARTESIAN_POINT('Ctrl Pts',(-3.46432076118331,11.4731609516943,48.4176356670416));
#29814=CARTESIAN_POINT('Ctrl Pts',(-3.52649817573868,11.4863352799677,48.4189800886591));
#29815=CARTESIAN_POINT('Ctrl Pts',(-3.67166031045544,11.5121367174564,48.4216081073348));
#29816=CARTESIAN_POINT('Ctrl Pts',(-3.75464503061683,11.5247638266717,48.422891704393));
#29817=CARTESIAN_POINT('Ctrl Pts',(-3.99041609265622,11.5581209387927,48.4262709574735));
#29818=CARTESIAN_POINT('Ctrl Pts',(-4.13001933608946,11.5743267261738,48.4278950754016));
#29819=CARTESIAN_POINT('Ctrl Pts',(-4.13366096331961,11.5746245276893,48.4278763391902));
#29820=CARTESIAN_POINT('Ctrl Pts',(-4.12845481065596,11.4732422824942,48.3603316468569));
#29821=CARTESIAN_POINT('Ctrl Pts',(-4.12850749787596,11.4851966459098,48.3652975204339));
#29822=CARTESIAN_POINT('Ctrl Pts',(-4.12864057911585,11.4974720069511,48.3719827330256));
#29823=CARTESIAN_POINT('Ctrl Pts',(-4.12920120927179,11.5208685373805,48.3864516772668));
#29824=CARTESIAN_POINT('Ctrl Pts',(-4.12962875818784,11.5319897067687,48.3942354089164));
#29825=CARTESIAN_POINT('Ctrl Pts',(-4.13155362590479,11.5609276470972,48.4157241439943));
#29826=CARTESIAN_POINT('Ctrl Pts',(-4.13369316567451,11.5743188502015,48.4275666875517));
#29827=CARTESIAN_POINT('Ctrl Pts',(-4.13722371861482,11.5746245485739,48.4275653153946));
#29828=CARTESIAN_POINT('Ctrl Pts',(-4.12845481065596,11.4732422824942,48.360331646857));
#29829=CARTESIAN_POINT('Ctrl Pts',(-4.12866555953595,11.5210597361567,48.3801951411646));
#29830=CARTESIAN_POINT('Ctrl Pts',(-4.13016261273423,11.5740131518293,48.4275680597092));
#29831=CARTESIAN_POINT('Ctrl Pts',(-4.13722371861483,11.5746245485739,48.4275653153946));
#29832=CARTESIAN_POINT('',(-4.12551258849077,11.6756605207468,48.495917442261));
#29833=CARTESIAN_POINT('Ctrl Pts',(-4.12551258849121,11.6756605207397,48.4959174422581));
#29834=CARTESIAN_POINT('Ctrl Pts',(-4.1258953594032,11.6686892977337,48.4930115088121));
#29835=CARTESIAN_POINT('Ctrl Pts',(-4.12627095135831,11.661843965821,48.4898115000955));
#29836=CARTESIAN_POINT('Ctrl Pts',(-4.12665447322118,11.6551189469296,48.4863820761544));
#29837=CARTESIAN_POINT('Ctrl Pts',(-4.1269487006233,11.649959697799,48.4837511166327));
#29838=CARTESIAN_POINT('Ctrl Pts',(-4.12724744290251,11.6448712703663,48.4809834473072));
#29839=CARTESIAN_POINT('Ctrl Pts',(-4.12755756488955,11.6398565149523,48.4780890456653));
#29840=CARTESIAN_POINT('Ctrl Pts',(-4.12790255670227,11.6342779051378,48.4748692002144));
#29841=CARTESIAN_POINT('Ctrl Pts',(-4.12826137312859,11.6287898949969,48.4714928657208));
#29842=CARTESIAN_POINT('Ctrl Pts',(-4.12864636713521,11.6234078109081,48.4679547934975));
#29843=CARTESIAN_POINT('Ctrl Pts',(-4.12882718134101,11.6208800903635,48.4662931216062));
#29844=CARTESIAN_POINT('Ctrl Pts',(-4.12901382912469,11.6183759600391,48.4645955090256));
#29845=CARTESIAN_POINT('Ctrl Pts',(-4.12920813507089,11.6158985300687,48.4628595640575));
#29846=CARTESIAN_POINT('Ctrl Pts',(-4.1293455880544,11.6141459839037,48.4616315480357));
#29847=CARTESIAN_POINT('Ctrl Pts',(-4.12948687798054,11.6124070235617,48.4603843962804));
#29848=CARTESIAN_POINT('Ctrl Pts',(-4.12963227160581,11.6106893807938,48.4591215269354));
#29849=CARTESIAN_POINT('Ctrl Pts',(-4.1297189685603,11.609665165347,48.4583684889261));
#29850=CARTESIAN_POINT('Ctrl Pts',(-4.12980723187199,11.6086472141289,48.457608922056));
#29851=CARTESIAN_POINT('Ctrl Pts',(-4.12989742751478,11.6076341633577,48.4568411226821));
#29852=CARTESIAN_POINT('Ctrl Pts',(-4.13014206460896,11.6048864719033,48.4547586251031));
#29853=CARTESIAN_POINT('Ctrl Pts',(-4.13040049692275,11.60216730197,48.4526172688089));
#29854=CARTESIAN_POINT('Ctrl Pts',(-4.1306843553102,11.599476279665,48.4504226933436));
#29855=CARTESIAN_POINT('Ctrl Pts',(-4.13087962948455,11.5976250496786,48.4489129831114));
#29856=CARTESIAN_POINT('Ctrl Pts',(-4.13108698032367,11.5957876815349,48.4473783076307));
#29857=CARTESIAN_POINT('Ctrl Pts',(-4.13131145786228,11.593976786229,48.4458307104849));
#29858=CARTESIAN_POINT('Ctrl Pts',(-4.13153926000086,11.5921390708566,48.4442601928212));
#29859=CARTESIAN_POINT('Ctrl Pts',(-4.13178482689973,11.5903229945745,48.442671860598));
#29860=CARTESIAN_POINT('Ctrl Pts',(-4.13206214386908,11.5885243391444,48.4410617399059));
#29861=CARTESIAN_POINT('Ctrl Pts',(-4.13233279400564,11.5867689242525,48.4394903272866));
#29862=CARTESIAN_POINT('Ctrl Pts',(-4.13263186492608,11.5850314713388,48.4378995371871));
#29863=CARTESIAN_POINT('Ctrl Pts',(-4.13299116528337,11.5833150139726,48.4362882720692));
#29864=CARTESIAN_POINT('Ctrl Pts',(-4.13323220081251,11.5821635338777,48.4352073598675));
#29865=CARTESIAN_POINT('Ctrl Pts',(-4.1334993953209,11.5810211498778,48.4341169808742));
#29866=CARTESIAN_POINT('Ctrl Pts',(-4.13382303553132,11.5798920643606,48.433017017294));
#29867=CARTESIAN_POINT('Ctrl Pts',(-4.13401325610055,11.5792284407351,48.4323705101802));
#29868=CARTESIAN_POINT('Ctrl Pts',(-4.13422283309914,11.5785688892838,48.4317201905913));
#29869=CARTESIAN_POINT('Ctrl Pts',(-4.13447082538378,11.577917245021,48.431067393103));
#29870=CARTESIAN_POINT('Ctrl Pts',(-4.13463747005405,11.5774793562235,48.4306287293665));
#29871=CARTESIAN_POINT('Ctrl Pts',(-4.13482261192084,11.5770415637595,48.4301854309067));
#29872=CARTESIAN_POINT('Ctrl Pts',(-4.13503924470767,11.576616631166,48.4297484868059));
#29873=CARTESIAN_POINT('Ctrl Pts',(-4.13517769151791,11.5763450630299,48.4294692422931));
#29874=CARTESIAN_POINT('Ctrl Pts',(-4.13533045467977,11.576074686727,48.429188484864));
#29875=CARTESIAN_POINT('Ctrl Pts',(-4.13551152790242,11.5758096277524,48.4289088568648));
#29876=CARTESIAN_POINT('Ctrl Pts',(-4.13563658855657,11.5756265612103,48.42871572803));
#29877=CARTESIAN_POINT('Ctrl Pts',(-4.13577439313221,11.5754472102307,48.4285243589121));
#29878=CARTESIAN_POINT('Ctrl Pts',(-4.13593295017201,11.5752795116543,48.4283419921649));
#29879=CARTESIAN_POINT('Ctrl Pts',(-4.13600396520959,11.5752044022759,48.4282603131589));
#29880=CARTESIAN_POINT('Ctrl Pts',(-4.13608017351886,11.5751304213442,48.4281791399513));
#29881=CARTESIAN_POINT('Ctrl Pts',(-4.13616638889705,11.5750574234697,48.4280978870178));
#29882=CARTESIAN_POINT('Ctrl Pts',(-4.13623123833384,11.5750025159677,48.42803677023));
#29883=CARTESIAN_POINT('Ctrl Pts',(-4.13629784753377,11.574949303433,48.427977124616));
#29884=CARTESIAN_POINT('Ctrl Pts',(-4.13639939779102,11.5748837650914,48.4279017477846));
#29885=CARTESIAN_POINT('Ctrl Pts',(-4.13645017291964,11.5748509959206,48.4278640593689));
#29886=CARTESIAN_POINT('Ctrl Pts',(-4.13650742313086,11.5748147554917,48.4278222495093));
#29887=CARTESIAN_POINT('Ctrl Pts',(-4.13660866417317,11.5747669664098,48.4277647101541));
#29888=CARTESIAN_POINT('Ctrl Pts',(-4.13665928465917,11.5747430718855,48.4277359404965));
#29889=CARTESIAN_POINT('Ctrl Pts',(-4.13671884717098,11.5747164083803,48.4277035354777));
#29890=CARTESIAN_POINT('Ctrl Pts',(-4.13681243800998,11.5746874268168,48.4276657143528));
#29891=CARTESIAN_POINT('Ctrl Pts',(-4.13689467272046,11.5746619618193,48.4276324823688));
#29892=CARTESIAN_POINT('Ctrl Pts',(-4.13700306041443,11.5746336393858,48.4275939402689));
#29893=CARTESIAN_POINT('Ctrl Pts',(-4.13715717683536,11.5746261598313,48.4275727843802));
#29894=CARTESIAN_POINT('Ctrl Pts',(-4.13717845940415,11.5746251269489,48.4275698628768));
#29895=CARTESIAN_POINT('Ctrl Pts',(-4.13720062027767,11.5746245484517,48.4275673318624));
#29896=CARTESIAN_POINT('Ctrl Pts',(-4.13722371782189,11.5746245485739,48.4275653154638));
#29897=CARTESIAN_POINT('Ctrl Pts',(-4.12551258849121,11.6756605207397,48.4959174422581));
#29898=CARTESIAN_POINT('Ctrl Pts',(-3.42379713716555,11.6392592214936,48.5061181031666));
#29899=CARTESIAN_POINT('Ctrl Pts',(-2.72152478000237,11.5986492866067,48.5108119661587));
#29900=CARTESIAN_POINT('Ctrl Pts',(-1.31995074912857,11.5098560202878,48.5141172996809));
#29901=CARTESIAN_POINT('Ctrl Pts',(-0.618564042211977,11.4835302569326,
48.5199462997129));
#29902=CARTESIAN_POINT('Ctrl Pts',(0.0835265683646154,11.4728541727075,
48.5199460669665));
#29903=CARTESIAN_POINT('Ctrl Pts',(48.5210408433891,11.4728541727075,0.0824317919368853));
#29904=CARTESIAN_POINT('Ctrl Pts',(48.5210413088829,11.4942063411577,0.0824317919368136));
#29905=CARTESIAN_POINT('Ctrl Pts',(48.5206840668827,11.5200575082527,0.082431791935498));
#29906=CARTESIAN_POINT('Ctrl Pts',(48.5224494671721,11.5731362269333,0.0824317919377551));
#29907=CARTESIAN_POINT('Ctrl Pts',(48.521026568362,11.5876793312944,0.082431791938572));
#29908=CARTESIAN_POINT('Ctrl Pts',(48.521026568362,11.6131136241746,0.0824317919395203));
#29909=CARTESIAN_POINT('Ctrl Pts',(48.5210409597623,11.4781922148201,0.4334770972252));
#29910=CARTESIAN_POINT('Ctrl Pts',(48.5209817377046,11.4971000233707,0.355275148040153));
#29911=CARTESIAN_POINT('Ctrl Pts',(48.5206817360346,11.5200113925674,0.355061808308312));
#29912=CARTESIAN_POINT('Ctrl Pts',(48.5224506910052,11.5731490589917,0.393775030003177));
#29913=CARTESIAN_POINT('Ctrl Pts',(48.521026568362,11.5876793312944,0.432701591427231));
#29914=CARTESIAN_POINT('Ctrl Pts',(48.521026568362,11.6131136241746,0.432779444551026));
#29915=CARTESIAN_POINT('Ctrl Pts',(48.5195837679409,11.4874426767152,0.784346426598513));
#29916=CARTESIAN_POINT('Ctrl Pts',(48.5206699839161,11.5031786713302,0.650878763011595));
#29917=CARTESIAN_POINT('Ctrl Pts',(48.520785019491,11.5245005081761,0.650515563920166));
#29918=CARTESIAN_POINT('Ctrl Pts',(48.5225859377424,11.5776504745526,0.716581364265669));
#29919=CARTESIAN_POINT('Ctrl Pts',(48.521026568362,11.5930695682598,0.783010363700175));
#29920=CARTESIAN_POINT('Ctrl Pts',(48.521026568362,11.6169153282063,0.783127097162531));
#29921=CARTESIAN_POINT('Ctrl Pts',(48.5162561594212,11.5143737377389,1.48575918656021));
#29922=CARTESIAN_POINT('Ctrl Pts',(48.5194060548862,11.5255419633077,1.29343922056592));
#29923=CARTESIAN_POINT('Ctrl Pts',(48.520440782358,11.5448479357173,1.29287966906623));
#29924=CARTESIAN_POINT('Ctrl Pts',(48.5225314340558,11.595969244612,1.38797527793364));
#29925=CARTESIAN_POINT('Ctrl Pts',(48.5210265683621,11.6126245374907,1.48363043829888));
#29926=CARTESIAN_POINT('Ctrl Pts',(48.5210265683621,11.632122144333,1.48373989603257));
#29927=CARTESIAN_POINT('Ctrl Pts',(48.5143857427228,11.5320543368676,1.83630261714859));
#29928=CARTESIAN_POINT('Ctrl Pts',(48.5184689188545,11.5418711528743,1.64039290832512));
#29929=CARTESIAN_POINT('Ctrl Pts',(48.5200083009784,11.5607507931985,1.63978686377675));
#29930=CARTESIAN_POINT('Ctrl Pts',(48.5223492032368,11.6098088718849,1.73656127992728));
#29931=CARTESIAN_POINT('Ctrl Pts',(48.5210265683621,11.6267892697561,1.83394174062464));
#29932=CARTESIAN_POINT('Ctrl Pts',(48.5210265683621,11.643527256428,1.83400504229111));
#29933=CARTESIAN_POINT('Ctrl Pts',(48.5119067425813,11.5986492866067,2.88748314030395));
#29934=CARTESIAN_POINT('Ctrl Pts',(48.5182994308552,11.612020620858,2.7670415434901));
#29935=CARTESIAN_POINT('Ctrl Pts',(48.5205482384131,11.6290600690796,2.76641567761564));
#29936=CARTESIAN_POINT('Ctrl Pts',(48.522328768896,11.6658592241822,2.82527806557464));
#29937=CARTESIAN_POINT('Ctrl Pts',(48.521026568362,11.6794362415567,2.88476631940751));
#29938=CARTESIAN_POINT('Ctrl Pts',(48.521026568362,11.689147704808,2.8845529620078));
#29939=CARTESIAN_POINT('Ctrl Pts',(48.5072128795892,11.6392592214936,3.58975549746708));
#29940=CARTESIAN_POINT('Ctrl Pts',(48.5152097045281,11.6580360440914,3.51781324718459));
#29941=CARTESIAN_POINT('Ctrl Pts',(48.5186631267213,11.6785648284689,3.51681245255117));
#29942=CARTESIAN_POINT('Ctrl Pts',(48.5215715586383,11.7135824344711,3.55049096279398));
#29943=CARTESIAN_POINT('Ctrl Pts',(48.521026568362,11.7280712560958,3.58517026767022));
#29944=CARTESIAN_POINT('Ctrl Pts',(48.521026568362,11.734768153188,3.58458821640705));
#29945=CARTESIAN_POINT('Ctrl Pts',(48.4970122186807,11.6756605207398,4.29147094879272));
#29946=CARTESIAN_POINT('Ctrl Pts',(48.5070083851258,11.6996409410726,4.29015424907548));
#29947=CARTESIAN_POINT('Ctrl Pts',(48.5130119725461,11.7229366511894,4.28885904835369));
#29948=CARTESIAN_POINT('Ctrl Pts',(48.5200210641643,11.7642258753785,4.28634531528796));
#29949=CARTESIAN_POINT('Ctrl Pts',(48.521026568362,11.7822193894509,4.28512678294403));
#29950=CARTESIAN_POINT('Ctrl Pts',(48.521026568362,11.7955954176946,4.28396341998253));
#29951=CARTESIAN_POINT('',(48.4970121852286,11.675660534618,4.29147094758644));
#29952=CARTESIAN_POINT('',(48.5210408433891,11.4728541727075,0.0824317919368853));
#29953=CARTESIAN_POINT('Ctrl Pts',(48.4970122186807,11.6756605207397,4.29147094879272));
#29954=CARTESIAN_POINT('Ctrl Pts',(48.5072128795892,11.6392592214936,3.58975549746708));
#29955=CARTESIAN_POINT('Ctrl Pts',(48.5119067425813,11.5986492866067,2.88748314030395));
#29956=CARTESIAN_POINT('Ctrl Pts',(48.5152120761034,11.5098560202879,1.48590910943014));
#29957=CARTESIAN_POINT('Ctrl Pts',(48.5210410761356,11.4835302569327,0.784522402513517));
#29958=CARTESIAN_POINT('Ctrl Pts',(48.5210408433891,11.4728541727075,0.0824317919368853));
#29959=CARTESIAN_POINT('Ctrl Pts',(48.4970121183243,11.6756605623744,4.29147094517387));
#29960=CARTESIAN_POINT('Ctrl Pts',(48.5011284587564,11.6855354834088,4.29092874030659));
#29961=CARTESIAN_POINT('Ctrl Pts',(48.5046183464519,11.6953464500614,4.29038568916614));
#29962=CARTESIAN_POINT('Ctrl Pts',(48.5075262052002,11.7049048876128,4.28984737507277));
#29963=CARTESIAN_POINT('Ctrl Pts',(48.5106115103027,11.7150466099943,4.28927621142185));
#29964=CARTESIAN_POINT('Ctrl Pts',(48.5130422894378,11.7249027978756,4.28871048915178));
#29965=CARTESIAN_POINT('Ctrl Pts',(48.5149248520449,11.734276287982,4.2881544780866));
#29966=CARTESIAN_POINT('Ctrl Pts',(48.5168934367235,11.7440780916189,4.28757306057625));
#29967=CARTESIAN_POINT('Ctrl Pts',(48.5182641071096,11.7533514160685,4.28700232059462));
#29968=CARTESIAN_POINT('Ctrl Pts',(48.5191968155257,11.7619163369651,4.2864432162865));
#29969=CARTESIAN_POINT('Ctrl Pts',(48.5202107580794,11.7712272187112,4.28583541684976));
#29970=CARTESIAN_POINT('Ctrl Pts',(48.5207093509836,11.779700856982,4.28524137620842));
#29971=CARTESIAN_POINT('Ctrl Pts',(48.5209120861297,11.787166042447,4.28465712816846));
#29972=CARTESIAN_POINT('Ctrl Pts',(48.5209927949347,11.7901379306939,4.28442453918706));
#29973=CARTESIAN_POINT('Ctrl Pts',(48.5210265662916,11.7929506159592,4.28419344823332));
#29974=CARTESIAN_POINT('Ctrl Pts',(48.5210265683619,11.7955954176946,4.28396341998252));
#29975=CARTESIAN_POINT('Ctrl Pts',(48.5210265683621,11.6131136241746,0.0824317919395203));
#29976=CARTESIAN_POINT('Ctrl Pts',(48.521026568362,11.5876793312944,0.082431791938572));
#29977=CARTESIAN_POINT('Ctrl Pts',(48.5224494671721,11.5731362269333,0.0824317919377551));
#29978=CARTESIAN_POINT('Ctrl Pts',(48.5206840668827,11.5200575082527,0.082431791935498));
#29979=CARTESIAN_POINT('Ctrl Pts',(48.5210413088829,11.4942063411577,0.0824317919368136));
#29980=CARTESIAN_POINT('Ctrl Pts',(48.5210408433891,11.4728541727075,0.0824317919368853));
#29981=CARTESIAN_POINT('Ctrl Pts',(48.5210408433891,11.4728541727075,0.0824317919368853));
#29982=CARTESIAN_POINT('Ctrl Pts',(48.5210409597627,11.4781922148199,-0.268613513351465));
#29983=CARTESIAN_POINT('Ctrl Pts',(48.5195837679418,11.4874426767152,-0.619482842725758));
#29984=CARTESIAN_POINT('Ctrl Pts',(48.5162561594226,11.5143737377394,-1.32089560269132));
#29985=CARTESIAN_POINT('Ctrl Pts',(48.5143857427244,11.5320543368685,-1.67143903328259));
#29986=CARTESIAN_POINT('Ctrl Pts',(48.5119067425819,11.598649286609,-2.72261955644951));
#29987=CARTESIAN_POINT('Ctrl Pts',(48.5072128795897,11.6392592214975,-3.42489191363272));
#29988=CARTESIAN_POINT('Ctrl Pts',(48.4970122186807,11.6756605207451,-4.1266073649755));
#29989=CARTESIAN_POINT('Ctrl Pts',(48.5210413088829,11.4942063411577,0.0824317919368136));
#29990=CARTESIAN_POINT('Ctrl Pts',(48.520981737705,11.4971000233707,-0.190411564166736));
#29991=CARTESIAN_POINT('Ctrl Pts',(48.5206699839168,11.5031786713304,-0.486015179139394));
#29992=CARTESIAN_POINT('Ctrl Pts',(48.5194060548872,11.5255419633083,-1.12857563669724));
#29993=CARTESIAN_POINT('Ctrl Pts',(48.5184689188556,11.5418711528751,-1.47552932445875));
#29994=CARTESIAN_POINT('Ctrl Pts',(48.5182994308554,11.6120206208596,-2.6021779596309));
#29995=CARTESIAN_POINT('Ctrl Pts',(48.5152097045281,11.6580360440938,-3.35294966333778));
#29996=CARTESIAN_POINT('Ctrl Pts',(48.5070083851259,11.6996409410751,-4.12529066522578));
#29997=CARTESIAN_POINT('Ctrl Pts',(48.5206840668827,11.5200575082527,0.082431791935498));
#29998=CARTESIAN_POINT('Ctrl Pts',(48.5206817360349,11.5200113925674,-0.190198224437316));
#29999=CARTESIAN_POINT('Ctrl Pts',(48.5207850194913,11.5245005081763,-0.485651980049793));
#30000=CARTESIAN_POINT('Ctrl Pts',(48.5204407823581,11.5448479357178,-1.12801608519759));
#30001=CARTESIAN_POINT('Ctrl Pts',(48.5200083009782,11.5607507931991,-1.47492327990924));
#30002=CARTESIAN_POINT('Ctrl Pts',(48.5205482384117,11.6290600690807,-2.60155209375108));
#30003=CARTESIAN_POINT('Ctrl Pts',(48.5186631267198,11.6785648284704,-3.35194886869318));
#30004=CARTESIAN_POINT('Ctrl Pts',(48.5130119725462,11.7229366511906,-4.12399546448852));
#30005=CARTESIAN_POINT('Ctrl Pts',(48.5224494671721,11.5731362269333,0.0824317919377551));
#30006=CARTESIAN_POINT('Ctrl Pts',(48.5224506910053,11.5731490589917,-0.228911446127667));
#30007=CARTESIAN_POINT('Ctrl Pts',(48.5225859377421,11.5776504745527,-0.551717780390339));
#30008=CARTESIAN_POINT('Ctrl Pts',(48.5225314340542,11.5959692446123,-1.22311169405866));
#30009=CARTESIAN_POINT('Ctrl Pts',(48.5223492032345,11.6098088718852,-1.57169769605248));
#30010=CARTESIAN_POINT('Ctrl Pts',(48.5223287688919,11.6658592241826,-2.6604144816998));
#30011=CARTESIAN_POINT('Ctrl Pts',(48.5215715586341,11.7135824344715,-3.38562737891988));
#30012=CARTESIAN_POINT('Ctrl Pts',(48.5200210641643,11.7642258753785,-4.12148173140813));
#30013=CARTESIAN_POINT('Ctrl Pts',(48.521026568362,11.5876793312944,0.082431791938572));
#30014=CARTESIAN_POINT('Ctrl Pts',(48.521026568362,11.5876793312944,-0.267838007550087));
#30015=CARTESIAN_POINT('Ctrl Pts',(48.5210265683614,11.5930695682598,-0.618146779822911));
#30016=CARTESIAN_POINT('Ctrl Pts',(48.5210265683597,11.6126245374908,-1.31876685442126));
#30017=CARTESIAN_POINT('Ctrl Pts',(48.5210265683587,11.6267892697563,-1.66907815674678));
#30018=CARTESIAN_POINT('Ctrl Pts',(48.5210265683567,11.6794362415569,-2.71990273552893));
#30019=CARTESIAN_POINT('Ctrl Pts',(48.5210265683567,11.728071256096,-3.42030668379117));
#30020=CARTESIAN_POINT('Ctrl Pts',(48.5210265683621,11.7822193894509,-4.12026319906499));
#30021=CARTESIAN_POINT('Ctrl Pts',(48.521026568362,11.6131136241746,0.0824317919395203));
#30022=CARTESIAN_POINT('Ctrl Pts',(48.521026568362,11.6131136241746,-0.267915860671985));
#30023=CARTESIAN_POINT('Ctrl Pts',(48.5210265683614,11.6169153282063,-0.618263513283491));
#30024=CARTESIAN_POINT('Ctrl Pts',(48.5210265683599,11.6321221443329,-1.31887631215353));
#30025=CARTESIAN_POINT('Ctrl Pts',(48.5210265683589,11.643527256428,-1.66914145841207));
#30026=CARTESIAN_POINT('Ctrl Pts',(48.521026568357,11.689147704808,-2.71968937812876));
#30027=CARTESIAN_POINT('Ctrl Pts',(48.521026568357,11.734768153188,-3.41972463252801));
#30028=CARTESIAN_POINT('Ctrl Pts',(48.5210265683621,11.7955954176946,-4.11909983610349));
#30029=CARTESIAN_POINT('',(48.4970121851698,11.6756605346477,-4.12660736376709));
#30030=CARTESIAN_POINT('Ctrl Pts',(48.521026568362,11.7955954176945,-4.11909983610349));
#30031=CARTESIAN_POINT('Ctrl Pts',(48.5210265631159,11.7889074035727,-4.11968151758424));
#30032=CARTESIAN_POINT('Ctrl Pts',(48.5208120576626,11.7811426004669,-4.12027027886023));
#30033=CARTESIAN_POINT('Ctrl Pts',(48.5201636703024,11.7724551591809,-4.12087195425065));
#30034=CARTESIAN_POINT('Ctrl Pts',(48.5195714197326,11.7645198686933,-4.12142153713069));
#30035=CARTESIAN_POINT('Ctrl Pts',(48.5186152663071,11.7558145072651,-4.12198191714169));
#30036=CARTESIAN_POINT('Ctrl Pts',(48.5171273935807,11.746498740511,-4.12255387295054));
#30037=CARTESIAN_POINT('Ctrl Pts',(48.5157117221484,11.7376350355518,-4.12309807373113));
#30038=CARTESIAN_POINT('Ctrl Pts',(48.5138132535906,11.7282190174497,-4.12365272793901));
#30039=CARTESIAN_POINT('Ctrl Pts',(48.5113099337767,11.7184280696927,-4.12421506208217));
#30040=CARTESIAN_POINT('Ctrl Pts',(48.5089256148278,11.7091025563742,-4.12475066442339));
#30041=CARTESIAN_POINT('Ctrl Pts',(48.5059916763245,11.6994377386554,-4.12529316148933));
#30042=CARTESIAN_POINT('Ctrl Pts',(48.502440122712,11.6896156896681,-4.12583768361868));
#30043=CARTESIAN_POINT('Ctrl Pts',(48.5007681263605,11.6849916766689,-4.12609403312455));
#30044=CARTESIAN_POINT('Ctrl Pts',(48.4989598840261,11.6803331677638,-4.12635080138442));
#30045=CARTESIAN_POINT('Ctrl Pts',(48.4970121181478,11.675660562453,-4.12660736135028));
#30046=CARTESIAN_POINT('Ctrl Pts',(48.4970122186807,11.6756605207451,-4.12660736497549));
#30047=CARTESIAN_POINT('Ctrl Pts',(48.5072128795897,11.6392592214975,-3.42489191363272));
#30048=CARTESIAN_POINT('Ctrl Pts',(48.5119067425819,11.598649286609,-2.72261955644951));
#30049=CARTESIAN_POINT('Ctrl Pts',(48.5152120761052,11.5098560202883,-1.32104552556029));
#30050=CARTESIAN_POINT('Ctrl Pts',(48.5210410761364,11.4835302569324,-0.619658818639818));
#30051=CARTESIAN_POINT('Ctrl Pts',(48.5210408433891,11.4728541727075,0.0824317919368853));
#30052=CARTESIAN_POINT('Ctrl Pts',(48.5210408433891,11.4728541727075,0.0824317919368853));
#30053=CARTESIAN_POINT('Ctrl Pts',(48.5210407270158,11.4675161305948,-0.268613513351429));
#30054=CARTESIAN_POINT('Ctrl Pts',(48.5195832988726,11.465926508769,-0.619710756297191));
#30055=CARTESIAN_POINT('Ctrl Pts',(48.5098524785203,11.464396632877,-1.32203631985499));
#30056=CARTESIAN_POINT('Ctrl Pts',(48.5015790863112,11.4644563788107,-1.67326464046703));
#30057=CARTESIAN_POINT('Ctrl Pts',(48.4606829527964,11.4583384590299,-2.72718702232965));
#30058=CARTESIAN_POINT('Ctrl Pts',(48.4174823766519,11.4609474762042,-3.42843979480817));
#30059=CARTESIAN_POINT('Ctrl Pts',(48.3614264232796,11.4732422824942,-4.1295495870784));
#30060=CARTESIAN_POINT('Ctrl Pts',(48.5210409597627,11.4781922148199,-0.268613513351465));
#30061=CARTESIAN_POINT('Ctrl Pts',(48.5200991113392,11.474986089803,-0.541629933632588));
#30062=CARTESIAN_POINT('Ctrl Pts',(48.5180114541286,11.4745419834777,-0.832717796196048));
#30063=CARTESIAN_POINT('Ctrl Pts',(48.5081357594276,11.4744825705814,-1.44781988667443));
#30064=CARTESIAN_POINT('Ctrl Pts',(48.5003285876198,11.4748353413217,-1.77183914952693));
#30065=CARTESIAN_POINT('Ctrl Pts',(48.4602502314476,11.4700074930207,-2.78846829308488));
#30066=CARTESIAN_POINT('Ctrl Pts',(48.4187304434639,11.4731609516944,-3.46541553760946));
#30067=CARTESIAN_POINT('Ctrl Pts',(48.3663922968565,11.4851966459098,-4.1296022742984));
#30068=CARTESIAN_POINT('Ctrl Pts',(48.5195837679418,11.4874426767152,-0.619482842725758));
#30069=CARTESIAN_POINT('Ctrl Pts',(48.5183837318974,11.4844803122479,-0.832372602290194));
#30070=CARTESIAN_POINT('Ctrl Pts',(48.5159956580517,11.4840908039498,-1.077403162417));
#30071=CARTESIAN_POINT('Ctrl Pts',(48.5060961369527,11.4843329006937,-1.62174846129248));
#30072=CARTESIAN_POINT('Ctrl Pts',(48.4985559882231,11.4849166217029,-1.92107075244751));
#30073=CARTESIAN_POINT('Ctrl Pts',(48.4596398458091,11.4818828006799,-2.8854776387807));
#30074=CARTESIAN_POINT('Ctrl Pts',(48.4200748650815,11.4863352799679,-3.52759295216471));
#30075=CARTESIAN_POINT('Ctrl Pts',(48.3730775094482,11.4974720069511,-4.1297353555383));
#30076=CARTESIAN_POINT('Ctrl Pts',(48.5162561594226,11.5143737377394,-1.32089560269132));
#30077=CARTESIAN_POINT('Ctrl Pts',(48.5144994210143,11.5105174196342,-1.44625764302723));
#30078=CARTESIAN_POINT('Ctrl Pts',(48.5114095528574,11.5090816899186,-1.62044191411888));
#30079=CARTESIAN_POINT('Ctrl Pts',(48.5010454693472,11.5079260458441,-2.04438576003036));
#30080=CARTESIAN_POINT('Ctrl Pts',(48.4937353771487,11.5081462764441,-2.29415477535813));
#30081=CARTESIAN_POINT('Ctrl Pts',(48.4576393364517,11.5065304546904,-3.12373338862082));
#30082=CARTESIAN_POINT('Ctrl Pts',(48.4227028837573,11.5121367174566,-3.6727550868809));
#30083=CARTESIAN_POINT('Ctrl Pts',(48.3875464536895,11.5208685373805,-4.13029598569424));
#30084=CARTESIAN_POINT('Ctrl Pts',(48.5143857427244,11.5320543368685,-1.67143903328259));
#30085=CARTESIAN_POINT('Ctrl Pts',(48.512333338594,11.5270830007425,-1.76939839553984));
#30086=CARTESIAN_POINT('Ctrl Pts',(48.5088435172715,11.5245577996658,-1.91879287024956));
#30087=CARTESIAN_POINT('Ctrl Pts',(48.4980397661311,11.5217114161951,-2.29309144746239));
#30088=CARTESIAN_POINT('Ctrl Pts',(48.4906923512577,11.5213343690961,-2.51800436110623));
#30089=CARTESIAN_POINT('Ctrl Pts',(48.4562520617536,11.5193254972085,-3.26497817319829));
#30090=CARTESIAN_POINT('Ctrl Pts',(48.4239864808155,11.5247638266718,-3.75573980704184));
#30091=CARTESIAN_POINT('Ctrl Pts',(48.395330185339,11.5319897067687,-4.13072353461029));
#30092=CARTESIAN_POINT('Ctrl Pts',(48.5119067425819,11.598649286609,-2.72261955644951));
#30093=CARTESIAN_POINT('Ctrl Pts',(48.5086939112097,11.5919036248663,-2.78284526372885));
#30094=CARTESIAN_POINT('Ctrl Pts',(48.5036610022595,11.5859418512212,-2.87982118572785));
#30095=CARTESIAN_POINT('Ctrl Pts',(48.4906361947483,11.5755468354635,-3.11912189520875));
#30096=CARTESIAN_POINT('Ctrl Pts',(48.4826251618699,11.5710816706623,-3.26145171762822));
#30097=CARTESIAN_POINT('Ctrl Pts',(48.4521822008654,11.5598336028535,-3.71424372296942));
#30098=CARTESIAN_POINT('Ctrl Pts',(48.4273657338961,11.5581209387927,-3.9915108690798));
#30099=CARTESIAN_POINT('Ctrl Pts',(48.4168189204169,11.5609276470972,-4.13264840232726));
#30100=CARTESIAN_POINT('Ctrl Pts',(48.5072128795897,11.6392592214975,-3.42489191363272));
#30101=CARTESIAN_POINT('Ctrl Pts',(48.5032144671204,11.6298708101994,-3.46086303878018));
#30102=CARTESIAN_POINT('Ctrl Pts',(48.4973225964204,11.6209827896646,-3.52283173406414));
#30103=CARTESIAN_POINT('Ctrl Pts',(48.4830998624069,11.6050189470302,-3.6684275949641));
#30104=CARTESIAN_POINT('Ctrl Pts',(48.4747689990933,11.5979431249305,-3.75205476058009));
#30105=CARTESIAN_POINT('Ctrl Pts',(48.4481398060047,11.5806510816468,-3.9899189580147));
#30106=CARTESIAN_POINT('Ctrl Pts',(48.4289898518242,11.5743267261738,-4.13111411251199));
#30107=CARTESIAN_POINT('Ctrl Pts',(48.4286614639744,11.5743188502015,-4.13478794209698));
#30108=CARTESIAN_POINT('Ctrl Pts',(48.4970122186807,11.6756605207451,-4.1266073649755));
#30109=CARTESIAN_POINT('Ctrl Pts',(48.4920141354582,11.6636703105801,-4.12726571485037));
#30110=CARTESIAN_POINT('Ctrl Pts',(48.4858839393056,11.6514649415887,-4.12793445428902));
#30111=CARTESIAN_POINT('Ctrl Pts',(48.4724837048702,11.6282480883359,-4.12937022856651));
#30112=CARTESIAN_POINT('Ctrl Pts',(48.4652136665875,11.6172366040747,-4.13013726340536));
#30113=CARTESIAN_POINT('Ctrl Pts',(48.4433803641393,11.588429281961,-4.13270208543106));
#30114=CARTESIAN_POINT('Ctrl Pts',(48.4289711156128,11.5746245276893,-4.13475573974208));
#30115=CARTESIAN_POINT('Ctrl Pts',(48.4286600918172,11.5746245485739,-4.13831849503729));
#30116=CARTESIAN_POINT('Ctrl Pts',(48.4970122186807,11.6756605207451,-4.12660736497549));
#30117=CARTESIAN_POINT('Ctrl Pts',(48.4870160522356,11.6516801004151,-4.12792406472524));
#30118=CARTESIAN_POINT('Ctrl Pts',(48.4724914340702,11.6268390447793,-4.12928232273011));
#30119=CARTESIAN_POINT('Ctrl Pts',(48.4433803641393,11.588429281961,-4.13270208543106));
#30120=CARTESIAN_POINT('Ctrl Pts',(48.4289711156128,11.5746245276893,-4.13475573974208));
#30121=CARTESIAN_POINT('Ctrl Pts',(48.4286600918172,11.5746245485739,-4.13831849503729));
#30122=CARTESIAN_POINT('',(48.3614264232796,11.4732422824942,-4.1295495870784));
#30123=CARTESIAN_POINT('Ctrl Pts',(48.4286600918172,11.5746245485739,-4.13831849503729));
#30124=CARTESIAN_POINT('Ctrl Pts',(48.4286628361315,11.5740131518292,-4.13125738915667));
#30125=CARTESIAN_POINT('Ctrl Pts',(48.3812899175873,11.5210597361567,-4.12976033595841));
#30126=CARTESIAN_POINT('Ctrl Pts',(48.3614264232796,11.4732422824942,-4.1295495870784));
#30127=CARTESIAN_POINT('Ctrl Pts',(48.3614264232796,11.4732422824942,-4.1295495870784));
#30128=CARTESIAN_POINT('Ctrl Pts',(48.4174823766519,11.4609474762041,-3.42843979480816));
#30129=CARTESIAN_POINT('Ctrl Pts',(48.4606829527965,11.45833845903,-2.72718702232965));
#30130=CARTESIAN_POINT('Ctrl Pts',(48.5152111308162,11.4664956854043,-1.32195717984616));
#30131=CARTESIAN_POINT('Ctrl Pts',(48.5210406106426,11.4621780884822,-0.619658818639743));
#30132=CARTESIAN_POINT('Ctrl Pts',(48.5210408433891,11.4728541727075,0.0824317919368853));
#30133=CARTESIAN_POINT('Ctrl Pts',(48.5210408433891,11.4728541727075,0.0824317919368853));
#30134=CARTESIAN_POINT('Ctrl Pts',(48.5210403778953,11.4515020042572,0.0824317919369568));
#30135=CARTESIAN_POINT('Ctrl Pts',(48.5206820691924,11.4284235901226,0.0824317919383984));
#30136=CARTESIAN_POINT('Ctrl Pts',(48.5165774170445,11.3941472536996,0.0824317919386741));
#30137=CARTESIAN_POINT('Ctrl Pts',(48.521026568362,11.3720285904897,0.0824317919387195));
#30138=CARTESIAN_POINT('Ctrl Pts',(48.521026568362,11.353653679453,0.0824317919395275));
#30139=CARTESIAN_POINT('Ctrl Pts',(48.5210407270158,11.4675161305948,-0.268613513351429));
#30140=CARTESIAN_POINT('Ctrl Pts',(48.5209806868526,11.4488974993901,-0.19075769252117));
#30141=CARTESIAN_POINT('Ctrl Pts',(48.5207163683071,11.4285976962987,-0.173571652692277));
#30142=CARTESIAN_POINT('Ctrl Pts',(48.5165547845964,11.3940705712691,-0.195374050131769));
#30143=CARTESIAN_POINT('Ctrl Pts',(48.521026568362,11.3720285904897,-0.234362487399122));
#30144=CARTESIAN_POINT('Ctrl Pts',(48.521026568362,11.353653679453,-0.268855620758342));
#30145=CARTESIAN_POINT('Ctrl Pts',(48.5195832988726,11.465926508769,-0.619710756297191));
#30146=CARTESIAN_POINT('Ctrl Pts',(48.5197866644935,11.447718516688,-0.486342918210061));
#30147=CARTESIAN_POINT('Ctrl Pts',(48.5193523631262,11.428587933622,-0.460576104880735));
#30148=CARTESIAN_POINT('Ctrl Pts',(48.5144416806968,11.3934281614349,-0.501601281203803));
#30149=CARTESIAN_POINT('Ctrl Pts',(48.517908907227,11.3718199008203,-0.568393270855329));
#30150=CARTESIAN_POINT('Ctrl Pts',(48.5172052126372,11.3536536794531,-0.620143038727369));
#30151=CARTESIAN_POINT('Ctrl Pts',(48.5098524785203,11.464396632877,-1.32203631985499));
#30152=CARTESIAN_POINT('Ctrl Pts',(48.5114206543114,11.4452664260876,-1.12899681037143));
#30153=CARTESIAN_POINT('Ctrl Pts',(48.5102621676323,11.4271829834973,-1.09680529269933));
#30154=CARTESIAN_POINT('Ctrl Pts',(48.503189825889,11.3913038531299,-1.16128319676548));
#30155=CARTESIAN_POINT('Ctrl Pts',(48.5037480059623,11.3711415135622,-1.25795261850317));
#30156=CARTESIAN_POINT('Ctrl Pts',(48.5019179682627,11.3536536794531,-1.32263498783753));
#30157=CARTESIAN_POINT('Ctrl Pts',(48.5015790863112,11.4644563788107,-1.67326464046703));
#30158=CARTESIAN_POINT('Ctrl Pts',(48.5041223947664,11.443938017789,-1.47607399129227));
#30159=CARTESIAN_POINT('Ctrl Pts',(48.5024096539486,11.4257324956489,-1.44603650678937));
#30160=CARTESIAN_POINT('Ctrl Pts',(48.4939878357291,11.389794304459,-1.51473806913817));
#30161=CARTESIAN_POINT('Ctrl Pts',(48.4927046623486,11.3706718159735,-1.61347711598941));
#30162=CARTESIAN_POINT('Ctrl Pts',(48.4904520792406,11.3536536794531,-1.67383952952162));
#30163=CARTESIAN_POINT('Ctrl Pts',(48.4743149973013,11.4603777656235,-2.37587956170877));
#30164=CARTESIAN_POINT('Ctrl Pts',(48.475786514634,11.4381382649982,-2.22841054012373));
#30165=CARTESIAN_POINT('Ctrl Pts',(48.4732866422588,11.4203247666438,-2.20690346123993));
#30166=CARTESIAN_POINT('Ctrl Pts',(48.4648102885898,11.3861758639155,-2.25918163609709));
#30167=CARTESIAN_POINT('Ctrl Pts',(48.4621240605424,11.3696277842964,-2.33296688983783));
#30168=CARTESIAN_POINT('Ctrl Pts',(48.4598703086856,11.3536536794531,-2.3760825335012));
#30169=CARTESIAN_POINT('Ctrl Pts',(48.4566988310128,11.4600103666203,-2.72684648513884));
#30170=CARTESIAN_POINT('Ctrl Pts',(48.4570444617159,11.4370088609558,-2.60397205099813));
#30171=CARTESIAN_POINT('Ctrl Pts',(48.4539681826041,11.4187667259072,-2.58894423029257));
#30172=CARTESIAN_POINT('Ctrl Pts',(48.4456390892507,11.3847952022384,-2.63542225695827));
#30173=CARTESIAN_POINT('Ctrl Pts',(48.442587008597,11.369053450208,-2.69692810432937));
#30174=CARTESIAN_POINT('Ctrl Pts',(48.4407544264067,11.3536536794531,-2.72712100634157));
#30175=CARTESIAN_POINT('Ctrl Pts',(48.4142685323449,11.4633689234831,-3.42840404975609));
#30176=CARTESIAN_POINT('Ctrl Pts',(48.4107714341872,11.4394032486783,-3.36074991139726));
#30177=CARTESIAN_POINT('Ctrl Pts',(48.4062756535774,11.4193327724023,-3.3565532039196));
#30178=CARTESIAN_POINT('Ctrl Pts',(48.3983980635604,11.3835624194323,-3.38631956505366));
#30179=CARTESIAN_POINT('Ctrl Pts',(48.395571861118,11.3679565169509,-3.42028263366534));
#30180=CARTESIAN_POINT('Ctrl Pts',(48.3948635884079,11.3536536794531,-3.42894804748508));
#30181=CARTESIAN_POINT('Ctrl Pts',(48.3894543999657,11.4670948793492,-3.77899469094328));
#30182=CARTESIAN_POINT('Ctrl Pts',(48.3832404595767,11.4429270404433,-3.74196626092199));
#30183=CARTESIAN_POINT('Ctrl Pts',(48.3779018427096,11.4214568596339,-3.74211938411377));
#30184=CARTESIAN_POINT('Ctrl Pts',(48.3703287539371,11.3837102983034,-3.76097220616443));
#30185=CARTESIAN_POINT('Ctrl Pts',(48.3680942820317,11.3674339177823,-3.7796719050233));
#30186=CARTESIAN_POINT('Ctrl Pts',(48.3680886315664,11.3536536794531,-3.77973662633619));
#30187=CARTESIAN_POINT('Ctrl Pts',(48.3614264232796,11.4732422824942,-4.1295495870784));
#30188=CARTESIAN_POINT('Ctrl Pts',(48.3514946761257,11.4493335556629,-4.12944421263839));
#30189=CARTESIAN_POINT('Ctrl Pts',(48.3455075205231,11.4261172510678,-4.12964628233286));
#30190=CARTESIAN_POINT('Ctrl Pts',(48.3384990828948,11.384958159128,-4.13010310894181));
#30191=CARTESIAN_POINT('Ctrl Pts',(48.3374778008691,11.3670153717833,-4.13035786585628));
#30192=CARTESIAN_POINT('Ctrl Pts',(48.3374778008691,11.3536536794531,-4.13035786585628));
#30193=CARTESIAN_POINT('Ctrl Pts',(48.3614264232796,11.4732422824942,-4.1295495870784));
#30194=CARTESIAN_POINT('Ctrl Pts',(48.35699350214,11.4625708971931,-4.12950255440878));
#30195=CARTESIAN_POINT('Ctrl Pts',(48.3532977193535,11.4520014357868,-4.12951249962561));
#30196=CARTESIAN_POINT('Ctrl Pts',(48.3502685940128,11.4417444398152,-4.12955963932613));
#30197=CARTESIAN_POINT('Ctrl Pts',(48.3470288568254,11.4307742858787,-4.12961005659963));
#30198=CARTESIAN_POINT('Ctrl Pts',(48.3445511740643,11.4201626014222,-4.12970297530091));
#30199=CARTESIAN_POINT('Ctrl Pts',(48.3426934184697,11.410143434642,-4.12980930460507));
#30200=CARTESIAN_POINT('Ctrl Pts',(48.3407233191754,11.3995183806998,-4.12992206394097));
#30201=CARTESIAN_POINT('Ctrl Pts',(48.3394488499117,11.389560407305,-4.13004977115178));
#30202=CARTESIAN_POINT('Ctrl Pts',(48.3386560089339,11.3805081454717,-4.13015382200378));
#30203=CARTESIAN_POINT('Ctrl Pts',(48.3377632333477,11.3703148802494,-4.13027098807239));
#30204=CARTESIAN_POINT('Ctrl Pts',(48.3374778008691,11.3612705067707,-4.13035786585628));
#30205=CARTESIAN_POINT('Ctrl Pts',(48.3374778008691,11.3536536794531,-4.13035786585629));
#30206=CARTESIAN_POINT('Ctrl Pts',(48.5210265683621,11.353653679453,0.0824317919395275));
#30207=CARTESIAN_POINT('Ctrl Pts',(48.521026568362,11.3720285904897,0.0824317919387195));
#30208=CARTESIAN_POINT('Ctrl Pts',(48.5165774170445,11.3941472536996,0.0824317919386741));
#30209=CARTESIAN_POINT('Ctrl Pts',(48.5206820691924,11.4284235901226,0.0824317919383984));
#30210=CARTESIAN_POINT('Ctrl Pts',(48.5210403778953,11.4515020042572,0.0824317919369568));
#30211=CARTESIAN_POINT('Ctrl Pts',(48.5210408433891,11.4728541727075,0.0824317919368853));
#30212=CARTESIAN_POINT('Ctrl Pts',(48.5210408433891,11.4728541727075,0.0824317919368853));
#30213=CARTESIAN_POINT('Ctrl Pts',(48.5210407270154,11.467516130595,0.433477097225236));
#30214=CARTESIAN_POINT('Ctrl Pts',(48.5195832988718,11.4659265087693,0.784574340170486));
#30215=CARTESIAN_POINT('Ctrl Pts',(48.5098524785193,11.4643966328772,1.48689990372619));
#30216=CARTESIAN_POINT('Ctrl Pts',(48.5015790863104,11.4644563788109,1.83812822433663));
#30217=CARTESIAN_POINT('Ctrl Pts',(48.4743149973016,11.4603777656235,2.54074314557413));
#30218=CARTESIAN_POINT('Ctrl Pts',(48.4566988310132,11.4600103666202,2.89171006900623));
#30219=CARTESIAN_POINT('Ctrl Pts',(48.4142685323453,11.463368923483,3.59326763362947));
#30220=CARTESIAN_POINT('Ctrl Pts',(48.3894543999659,11.4670948793491,3.94385827482061));
#30221=CARTESIAN_POINT('Ctrl Pts',(48.3614264232796,11.4732422824942,4.29441317095744));
#30222=CARTESIAN_POINT('Ctrl Pts',(48.5210403778953,11.4515020042572,0.0824317919369568));
#30223=CARTESIAN_POINT('Ctrl Pts',(48.5209806868523,11.4488974993903,0.355621276395441));
#30224=CARTESIAN_POINT('Ctrl Pts',(48.519786664493,11.4477185166882,0.651206502084196));
#30225=CARTESIAN_POINT('Ctrl Pts',(48.5114206543107,11.4452664260879,1.29386039424399));
#30226=CARTESIAN_POINT('Ctrl Pts',(48.5041223947658,11.4439380177892,1.64093757516338));
#30227=CARTESIAN_POINT('Ctrl Pts',(48.4757865146344,11.4381382649983,2.39327412399031));
#30228=CARTESIAN_POINT('Ctrl Pts',(48.4570444617164,11.4370088609558,2.76883563486649));
#30229=CARTESIAN_POINT('Ctrl Pts',(48.4107714341876,11.4394032486783,3.52561349527108));
#30230=CARTESIAN_POINT('Ctrl Pts',(48.3832404595769,11.4429270404433,3.90682984479949));
#30231=CARTESIAN_POINT('Ctrl Pts',(48.3514946761257,11.4493335556629,4.29430779651743));
#30232=CARTESIAN_POINT('Ctrl Pts',(48.5206820691924,11.4284235901226,0.0824317919383984));
#30233=CARTESIAN_POINT('Ctrl Pts',(48.5207163683069,11.4285976962988,0.338435236569074));
#30234=CARTESIAN_POINT('Ctrl Pts',(48.5193523631259,11.4285879336221,0.62543968875722));
#30235=CARTESIAN_POINT('Ctrl Pts',(48.5102621676319,11.4271829834975,1.26166887657425));
#30236=CARTESIAN_POINT('Ctrl Pts',(48.5024096539482,11.4257324956491,1.61090009066305));
#30237=CARTESIAN_POINT('Ctrl Pts',(48.4732866422591,11.4203247666438,2.37176704510986));
#30238=CARTESIAN_POINT('Ctrl Pts',(48.4539681826045,11.4187667259072,2.75380781416369));
#30239=CARTESIAN_POINT('Ctrl Pts',(48.4062756535777,11.4193327724023,3.52141678779466));
#30240=CARTESIAN_POINT('Ctrl Pts',(48.3779018427096,11.4214568596339,3.90698296799157));
#30241=CARTESIAN_POINT('Ctrl Pts',(48.3455075205231,11.4261172510677,4.2945098662119));
#30242=CARTESIAN_POINT('Ctrl Pts',(48.5165774170445,11.3941472536996,0.0824317919386741));
#30243=CARTESIAN_POINT('Ctrl Pts',(48.5165547845964,11.3940705712691,0.360237634009118));
#30244=CARTESIAN_POINT('Ctrl Pts',(48.5144416806968,11.393428161435,0.666464865081089));
#30245=CARTESIAN_POINT('Ctrl Pts',(48.503189825889,11.39130385313,1.32614678064237));
#30246=CARTESIAN_POINT('Ctrl Pts',(48.4939878357291,11.389794304459,1.6796016530147));
#30247=CARTESIAN_POINT('Ctrl Pts',(48.46481028859,11.3861758639155,2.42404521997249));
#30248=CARTESIAN_POINT('Ctrl Pts',(48.4456390892509,11.3847952022384,2.80028584083416));
#30249=CARTESIAN_POINT('Ctrl Pts',(48.3983980635606,11.3835624194323,3.55118314893107));
#30250=CARTESIAN_POINT('Ctrl Pts',(48.3703287539371,11.3837102983034,3.92583579004287));
#30251=CARTESIAN_POINT('Ctrl Pts',(48.3384990828948,11.384958159128,4.29496669282085));
#30252=CARTESIAN_POINT('Ctrl Pts',(48.521026568362,11.3720285904897,0.0824317919387195));
#30253=CARTESIAN_POINT('Ctrl Pts',(48.5210265683621,11.3720285904897,0.399226071276561));
#30254=CARTESIAN_POINT('Ctrl Pts',(48.517908907227,11.3718199008203,0.733256854732802));
#30255=CARTESIAN_POINT('Ctrl Pts',(48.5037480059623,11.3711415135622,1.42281620238079));
#30256=CARTESIAN_POINT('Ctrl Pts',(48.4927046623486,11.3706718159735,1.77834069986712));
#30257=CARTESIAN_POINT('Ctrl Pts',(48.4621240605424,11.3696277842964,2.49783047371582));
#30258=CARTESIAN_POINT('Ctrl Pts',(48.4425870085971,11.369053450208,2.86179168820756));
#30259=CARTESIAN_POINT('Ctrl Pts',(48.395571861118,11.3679565169509,3.58514621754392));
#30260=CARTESIAN_POINT('Ctrl Pts',(48.3680942820317,11.3674339177823,3.94453548890209));
#30261=CARTESIAN_POINT('Ctrl Pts',(48.3374778008691,11.3670153717833,4.29522144973533));
#30262=CARTESIAN_POINT('Ctrl Pts',(48.521026568362,11.353653679453,0.0824317919395275));
#30263=CARTESIAN_POINT('Ctrl Pts',(48.521026568362,11.353653679453,0.433719204637397));
#30264=CARTESIAN_POINT('Ctrl Pts',(48.5172052126372,11.353653679453,0.785006622606423));
#30265=CARTESIAN_POINT('Ctrl Pts',(48.5019179682626,11.353653679453,1.48749857171659));
#30266=CARTESIAN_POINT('Ctrl Pts',(48.4904520792406,11.353653679453,1.83870311340066));
#30267=CARTESIAN_POINT('Ctrl Pts',(48.4598703086855,11.353653679453,2.54094611738025));
#30268=CARTESIAN_POINT('Ctrl Pts',(48.4407544264066,11.353653679453,2.89198459022065));
#30269=CARTESIAN_POINT('Ctrl Pts',(48.3948635884079,11.353653679453,3.59381163136416));
#30270=CARTESIAN_POINT('Ctrl Pts',(48.3680886315664,11.353653679453,3.94460021021523));
#30271=CARTESIAN_POINT('Ctrl Pts',(48.3374778008691,11.353653679453,4.29522144973533));
#30272=CARTESIAN_POINT('',(48.3614264232796,11.4732422824942,4.29441317095745));
#30273=CARTESIAN_POINT('Origin',(48.6500773750264,11.3534224546478,4.32103607292982));
#30274=CARTESIAN_POINT('Ctrl Pts',(48.3614264232796,11.4732422824942,4.29441317095745));
#30275=CARTESIAN_POINT('Ctrl Pts',(48.4174823766521,11.4609474762041,3.59330337868377));
#30276=CARTESIAN_POINT('Ctrl Pts',(48.4606829527973,11.4583384590298,2.89205060619289));
#30277=CARTESIAN_POINT('Ctrl Pts',(48.5152111308147,11.4664956854046,1.48682076371788));
#30278=CARTESIAN_POINT('Ctrl Pts',(48.5210406106418,11.4621780884825,0.784522402513595));
#30279=CARTESIAN_POINT('Ctrl Pts',(48.5210408433891,11.4728541727075,0.0824317919368853));
#30280=CARTESIAN_POINT('Ctrl Pts',(-48.353987706665,11.4728541727075,0.0824317919420715));
#30281=CARTESIAN_POINT('Ctrl Pts',(-48.3539875902914,11.4675161305949,-0.268613513346274));
#30282=CARTESIAN_POINT('Ctrl Pts',(-48.3525301621478,11.4659265087692,-0.619710756291519));
#30283=CARTESIAN_POINT('Ctrl Pts',(-48.3427993417953,11.4643966328771,-1.32203631984721));
#30284=CARTESIAN_POINT('Ctrl Pts',(-48.3345259495864,11.4644563788108,-1.67326464045766));
#30285=CARTESIAN_POINT('Ctrl Pts',(-48.3072618605776,11.4603777656235,-2.37587956169515));
#30286=CARTESIAN_POINT('Ctrl Pts',(-48.2896456942891,11.4600103666202,-2.72684648512726));
#30287=CARTESIAN_POINT('Ctrl Pts',(-48.2472153956212,11.463368923483,-3.42840404975053));
#30288=CARTESIAN_POINT('Ctrl Pts',(-48.2224012632418,11.4670948793491,-3.77899469094169));
#30289=CARTESIAN_POINT('Ctrl Pts',(-48.1943732865555,11.4732422824942,-4.12954958707854));
#30290=CARTESIAN_POINT('Ctrl Pts',(-48.3539872411712,11.4515020042572,0.0824317919420012));
#30291=CARTESIAN_POINT('Ctrl Pts',(-48.3539275501283,11.4488974993903,-0.19075769251648));
#30292=CARTESIAN_POINT('Ctrl Pts',(-48.352733527769,11.4477185166882,-0.486342918205233));
#30293=CARTESIAN_POINT('Ctrl Pts',(-48.3443675175867,11.4452664260878,-1.12899681036502));
#30294=CARTESIAN_POINT('Ctrl Pts',(-48.3370692580418,11.4439380177892,-1.47607399128441));
#30295=CARTESIAN_POINT('Ctrl Pts',(-48.3087333779103,11.4381382649983,-2.22841054011135));
#30296=CARTESIAN_POINT('Ctrl Pts',(-48.2899913249923,11.4370088609558,-2.60397205098753));
#30297=CARTESIAN_POINT('Ctrl Pts',(-48.2437182974635,11.4394032486783,-3.36074991139214));
#30298=CARTESIAN_POINT('Ctrl Pts',(-48.2161873228528,11.4429270404433,-3.74196626092057));
#30299=CARTESIAN_POINT('Ctrl Pts',(-48.1844415394016,11.4493335556629,-4.12944421263853));
#30300=CARTESIAN_POINT('Ctrl Pts',(-48.3536289324683,11.4284235901226,0.0824317919405622));
#30301=CARTESIAN_POINT('Ctrl Pts',(-48.3536632315829,11.4285976962988,-0.173571652690114));
#30302=CARTESIAN_POINT('Ctrl Pts',(-48.3522992264019,11.4285879336221,-0.460576104878249));
#30303=CARTESIAN_POINT('Ctrl Pts',(-48.3432090309079,11.4271829834975,-1.09680529269528));
#30304=CARTESIAN_POINT('Ctrl Pts',(-48.3353565172242,11.4257324956491,-1.4460365067841));
#30305=CARTESIAN_POINT('Ctrl Pts',(-48.3062335055351,11.4203247666438,-2.20690346123091));
#30306=CARTESIAN_POINT('Ctrl Pts',(-48.2869150458804,11.4187667259072,-2.58894423028474));
#30307=CARTESIAN_POINT('Ctrl Pts',(-48.2392225168536,11.4193327724023,-3.35655320391572));
#30308=CARTESIAN_POINT('Ctrl Pts',(-48.2108487059856,11.4214568596339,-3.74211938411265));
#30309=CARTESIAN_POINT('Ctrl Pts',(-48.178454383799,11.4261172510678,-4.129646282333));
#30310=CARTESIAN_POINT('Ctrl Pts',(-48.3495242803204,11.3941472536996,0.0824317919402862));
#30311=CARTESIAN_POINT('Ctrl Pts',(-48.3495016478723,11.3940705712692,-0.195374050130163));
#30312=CARTESIAN_POINT('Ctrl Pts',(-48.3473885439727,11.393428161435,-0.501601281202104));
#30313=CARTESIAN_POINT('Ctrl Pts',(-48.3361366891649,11.39130385313,-1.16128319676337));
#30314=CARTESIAN_POINT('Ctrl Pts',(-48.326934699005,11.3897943044591,-1.51473806913577));
#30315=CARTESIAN_POINT('Ctrl Pts',(-48.2977571518659,11.3861758639155,-2.25918163609357));
#30316=CARTESIAN_POINT('Ctrl Pts',(-48.2785859525268,11.3847952022384,-2.6354222569552));
#30317=CARTESIAN_POINT('Ctrl Pts',(-48.2313449268365,11.3835624194323,-3.38631956505211));
#30318=CARTESIAN_POINT('Ctrl Pts',(-48.203275617213,11.3837102983034,-3.76097220616396));
#30319=CARTESIAN_POINT('Ctrl Pts',(-48.1714459461707,11.384958159128,-4.13010310894195));
#30320=CARTESIAN_POINT('Ctrl Pts',(-48.3539734316379,11.3720285904897,0.08243179194024));
#30321=CARTESIAN_POINT('Ctrl Pts',(-48.353973431638,11.3720285904897,-0.234362487397608));
#30322=CARTESIAN_POINT('Ctrl Pts',(-48.350855770503,11.3718199008203,-0.56839327085381));
#30323=CARTESIAN_POINT('Ctrl Pts',(-48.3366948692382,11.3711415135622,-1.25795261850178));
#30324=CARTESIAN_POINT('Ctrl Pts',(-48.3256515256246,11.3706718159735,-1.6134771159882));
#30325=CARTESIAN_POINT('Ctrl Pts',(-48.2950709238183,11.3696277842964,-2.33296688983691));
#30326=CARTESIAN_POINT('Ctrl Pts',(-48.275533871873,11.369053450208,-2.69692810432859));
#30327=CARTESIAN_POINT('Ctrl Pts',(-48.2285187243939,11.3679565169509,-3.42028263366496));
#30328=CARTESIAN_POINT('Ctrl Pts',(-48.2010411453076,11.3674339177823,-3.77967190502318));
#30329=CARTESIAN_POINT('Ctrl Pts',(-48.170424664145,11.3670153717833,-4.13035786585643));
#30330=CARTESIAN_POINT('Ctrl Pts',(-48.3539734316379,11.3536536794531,0.0824317919394318));
#30331=CARTESIAN_POINT('Ctrl Pts',(-48.3539734316379,11.3536536794531,-0.268855620758443));
#30332=CARTESIAN_POINT('Ctrl Pts',(-48.3501520759131,11.3536536794531,-0.620143038727429));
#30333=CARTESIAN_POINT('Ctrl Pts',(-48.3348648315386,11.3536536794531,-1.32263498783758));
#30334=CARTESIAN_POINT('Ctrl Pts',(-48.3233989425165,11.3536536794531,-1.67383952952175));
#30335=CARTESIAN_POINT('Ctrl Pts',(-48.2928171719614,11.3536536794531,-2.37608253350134));
#30336=CARTESIAN_POINT('Ctrl Pts',(-48.2737012896825,11.3536536794531,-2.72712100634169));
#30337=CARTESIAN_POINT('Ctrl Pts',(-48.2278104516838,11.3536536794531,-3.42894804748519));
#30338=CARTESIAN_POINT('Ctrl Pts',(-48.2010354948423,11.3536536794531,-3.77973662633633));
#30339=CARTESIAN_POINT('Ctrl Pts',(-48.170424664145,11.3536536794531,-4.13035786585643));
#30340=CARTESIAN_POINT('',(-48.353987706665,11.4728541727075,0.0824317919420715));
#30341=CARTESIAN_POINT('Ctrl Pts',(-48.3539734316379,11.3536536794531,0.0824317919394318));
#30342=CARTESIAN_POINT('Ctrl Pts',(-48.3539734316379,11.3720285904897,0.08243179194024));
#30343=CARTESIAN_POINT('Ctrl Pts',(-48.3495242803204,11.3941472536996,0.0824317919402862));
#30344=CARTESIAN_POINT('Ctrl Pts',(-48.3536289324683,11.4284235901226,0.0824317919405622));
#30345=CARTESIAN_POINT('Ctrl Pts',(-48.3539872411712,11.4515020042572,0.0824317919420012));
#30346=CARTESIAN_POINT('Ctrl Pts',(-48.353987706665,11.4728541727075,0.0824317919420715));
#30347=CARTESIAN_POINT('',(-48.1943732865555,11.4732422824942,-4.1295495870785));
#30348=CARTESIAN_POINT('Ctrl Pts',(-48.170424664145,11.3536536794531,-4.13035786585642));
#30349=CARTESIAN_POINT('Ctrl Pts',(-48.170424664145,11.3608560447969,-4.13035786585642));
#30350=CARTESIAN_POINT('Ctrl Pts',(-48.1706799400046,11.3693343502548,-4.13028019061231));
#30351=CARTESIAN_POINT('Ctrl Pts',(-48.1714624816211,11.3788543868427,-4.13017267066916));
#30352=CARTESIAN_POINT('Ctrl Pts',(-48.1721853831276,11.3876488696476,-4.13007334517998));
#30353=CARTESIAN_POINT('Ctrl Pts',(-48.1733606260326,11.3973323098415,-4.12994875887561));
#30354=CARTESIAN_POINT('Ctrl Pts',(-48.1751937930179,11.4076804802593,-4.12983582017109));
#30355=CARTESIAN_POINT('Ctrl Pts',(-48.1769664379229,11.4176870054229,-4.12972661014235));
#30356=CARTESIAN_POINT('Ctrl Pts',(-48.1793558503801,11.428314631214,-4.12962842768296));
#30357=CARTESIAN_POINT('Ctrl Pts',(-48.1825116713384,11.4393255986458,-4.12957145846169));
#30358=CARTESIAN_POINT('Ctrl Pts',(-48.1854345364211,11.4495237602833,-4.12951869458509));
#30359=CARTESIAN_POINT('Ctrl Pts',(-48.1890152738075,11.4600498295069,-4.12950132106614));
#30360=CARTESIAN_POINT('Ctrl Pts',(-48.1933281633331,11.4706948755438,-4.12953941874883));
#30361=CARTESIAN_POINT('Ctrl Pts',(-48.193671905835,11.4715432985641,-4.12954245518013));
#30362=CARTESIAN_POINT('Ctrl Pts',(-48.1940202724543,11.4723924705143,-4.12954584164855));
#30363=CARTESIAN_POINT('Ctrl Pts',(-48.1943732865555,11.4732422824942,-4.1295495870785));
#30364=CARTESIAN_POINT('Ctrl Pts',(-48.1943732865555,11.4732422824942,-4.1295495870785));
#30365=CARTESIAN_POINT('Ctrl Pts',(-48.2504292399281,11.4609474762041,-3.42843979480483));
#30366=CARTESIAN_POINT('Ctrl Pts',(-48.2936298160732,11.4583384590298,-2.7271870223139));
#30367=CARTESIAN_POINT('Ctrl Pts',(-48.3481579940908,11.4664956854045,-1.32195717983891));
#30368=CARTESIAN_POINT('Ctrl Pts',(-48.3539874739178,11.4621780884824,-0.619658818634619));
#30369=CARTESIAN_POINT('Ctrl Pts',(-48.353987706665,11.4728541727075,0.0824317919420715));
#30370=CARTESIAN_POINT('Ctrl Pts',(-48.353987706665,11.4728541727075,0.0824317919420715));
#30371=CARTESIAN_POINT('Ctrl Pts',(-48.3539878230383,11.47819221482,-0.268613513346239));
#30372=CARTESIAN_POINT('Ctrl Pts',(-48.3525306312169,11.4874426767151,-0.619482842719547));
#30373=CARTESIAN_POINT('Ctrl Pts',(-48.3492030226972,11.5143737377389,-1.32089560268123));
#30374=CARTESIAN_POINT('Ctrl Pts',(-48.3473326059989,11.5320543368675,-1.67143903326961));
#30375=CARTESIAN_POINT('Ctrl Pts',(-48.3448536058572,11.5986492866067,-2.72261955642498));
#30376=CARTESIAN_POINT('Ctrl Pts',(-48.3401597428651,11.6392592214936,-3.42489191358813));
#30377=CARTESIAN_POINT('Ctrl Pts',(-48.3299590819566,11.6756605207398,-4.12660736491379));
#30378=CARTESIAN_POINT('Ctrl Pts',(-48.3539875902914,11.4675161305949,-0.268613513346274));
#30379=CARTESIAN_POINT('Ctrl Pts',(-48.3530459746145,11.4749860898031,-0.541629933626861));
#30380=CARTESIAN_POINT('Ctrl Pts',(-48.3513305951723,11.4844803122479,-0.832372602283611));
#30381=CARTESIAN_POINT('Ctrl Pts',(-48.3474462842888,11.5105174196336,-1.44625764301694));
#30382=CARTESIAN_POINT('Ctrl Pts',(-48.3452802018684,11.5270830007414,-1.76939839552668));
#30383=CARTESIAN_POINT('Ctrl Pts',(-48.3416407744847,11.5919036248635,-2.78284526370196));
#30384=CARTESIAN_POINT('Ctrl Pts',(-48.3361613303957,11.6298708101947,-3.46086303872938));
#30385=CARTESIAN_POINT('Ctrl Pts',(-48.3249609987341,11.6636703105734,-4.12726571477241));
#30386=CARTESIAN_POINT('Ctrl Pts',(-48.3525301621478,11.4659265087692,-0.619710756291519));
#30387=CARTESIAN_POINT('Ctrl Pts',(-48.3509583174037,11.4745419834778,-0.832717796189608));
#30388=CARTESIAN_POINT('Ctrl Pts',(-48.3489425213265,11.4840908039496,-1.07740316240887));
#30389=CARTESIAN_POINT('Ctrl Pts',(-48.3443564161318,11.5090816899176,-1.62044191410439));
#30390=CARTESIAN_POINT('Ctrl Pts',(-48.3417903805458,11.5245577996642,-1.91879287023042));
#30391=CARTESIAN_POINT('Ctrl Pts',(-48.3366078655344,11.5859418512174,-2.87982118568858));
#30392=CARTESIAN_POINT('Ctrl Pts',(-48.3302694596955,11.6209827896584,-3.52283173399625));
#30393=CARTESIAN_POINT('Ctrl Pts',(-48.3188308025814,11.6514649415801,-4.12793445419003));
#30394=CARTESIAN_POINT('Ctrl Pts',(-48.3427993417953,11.4643966328771,-1.32203631984721));
#30395=CARTESIAN_POINT('Ctrl Pts',(-48.3410826227025,11.4744825705815,-1.44781988666579));
#30396=CARTESIAN_POINT('Ctrl Pts',(-48.3390430002274,11.4843329006933,-1.62174846128019));
#30397=CARTESIAN_POINT('Ctrl Pts',(-48.3339923326216,11.5079260458424,-2.04438576000585));
#30398=CARTESIAN_POINT('Ctrl Pts',(-48.3309866294054,11.5217114161924,-2.29309144742929));
#30399=CARTESIAN_POINT('Ctrl Pts',(-48.323583058023,11.5755468354576,-3.11912189514342));
#30400=CARTESIAN_POINT('Ctrl Pts',(-48.3160467256819,11.6050189470212,-3.66842759486343));
#30401=CARTESIAN_POINT('Ctrl Pts',(-48.3054305681461,11.6282480883245,-4.12937022843424));
#30402=CARTESIAN_POINT('Ctrl Pts',(-48.3345259495864,11.4644563788108,-1.67326464045766));
#30403=CARTESIAN_POINT('Ctrl Pts',(-48.3332754508949,11.4748353413217,-1.7718391495168));
#30404=CARTESIAN_POINT('Ctrl Pts',(-48.331502851498,11.4849166217024,-1.92107075243263));
#30405=CARTESIAN_POINT('Ctrl Pts',(-48.3266822404233,11.5081462764419,-2.29415477532779));
#30406=CARTESIAN_POINT('Ctrl Pts',(-48.3236392145321,11.5213343690928,-2.51800436106519));
#30407=CARTESIAN_POINT('Ctrl Pts',(-48.3155720251447,11.5710816706553,-3.26145171754922));
#30408=CARTESIAN_POINT('Ctrl Pts',(-48.3077158623684,11.5979431249203,-3.75205476046376));
#30409=CARTESIAN_POINT('Ctrl Pts',(-48.2981605298634,11.6172366040622,-4.13013726326082));
#30410=CARTESIAN_POINT('Ctrl Pts',(-48.2936298160732,11.4583384590298,-2.7271870223139));
#30411=CARTESIAN_POINT('Ctrl Pts',(-48.2931970947244,11.4700074930205,-2.7884682930686));
#30412=CARTESIAN_POINT('Ctrl Pts',(-48.2925867090858,11.481882800679,-2.88547763875839));
#30413=CARTESIAN_POINT('Ctrl Pts',(-48.2905861997279,11.5065304546877,-3.12373338857996));
#30414=CARTESIAN_POINT('Ctrl Pts',(-48.2891989250297,11.5193254972046,-3.26497817314492));
#30415=CARTESIAN_POINT('Ctrl Pts',(-48.2851290641411,11.5598336028455,-3.71424372287552));
#30416=CARTESIAN_POINT('Ctrl Pts',(-48.2810866692801,11.5806510816358,-3.98991895788831));
#30417=CARTESIAN_POINT('Ctrl Pts',(-48.2763272274152,11.5884292819489,-4.13270208529043));
#30418=CARTESIAN_POINT('Ctrl Pts',(-48.2504292399281,11.4609474762041,-3.42843979480483));
#30419=CARTESIAN_POINT('Ctrl Pts',(-48.2516773067401,11.4731609516943,-3.46541553760594));
#30420=CARTESIAN_POINT('Ctrl Pts',(-48.2530217283576,11.4863352799677,-3.52759295216131));
#30421=CARTESIAN_POINT('Ctrl Pts',(-48.2556497470334,11.5121367174564,-3.67275508687807));
#30422=CARTESIAN_POINT('Ctrl Pts',(-48.2569333440916,11.5247638266717,-3.75573980703945));
#30423=CARTESIAN_POINT('Ctrl Pts',(-48.260312597172,11.5581209387927,-3.99151086907883));
#30424=CARTESIAN_POINT('Ctrl Pts',(-48.2619367151001,11.5743267261738,-4.13111411251207));
#30425=CARTESIAN_POINT('Ctrl Pts',(-48.2619179788887,11.5746245276893,-4.13475573974222));
#30426=CARTESIAN_POINT('Ctrl Pts',(-48.1943732865555,11.4732422824942,-4.12954958707854));
#30427=CARTESIAN_POINT('Ctrl Pts',(-48.1993391601324,11.4851966459098,-4.12960227429855));
#30428=CARTESIAN_POINT('Ctrl Pts',(-48.2060243727241,11.4974720069511,-4.12973535553844));
#30429=CARTESIAN_POINT('Ctrl Pts',(-48.2204933169654,11.5208685373805,-4.13029598569439));
#30430=CARTESIAN_POINT('Ctrl Pts',(-48.2282770486149,11.5319897067687,-4.13072353461044));
#30431=CARTESIAN_POINT('Ctrl Pts',(-48.2497657836928,11.5609276470972,-4.1326484023274));
#30432=CARTESIAN_POINT('Ctrl Pts',(-48.2616083272502,11.5743188502015,-4.13478794209711));
#30433=CARTESIAN_POINT('Ctrl Pts',(-48.2616069550931,11.5746245485739,-4.13831849503743));
#30434=CARTESIAN_POINT('Ctrl Pts',(-48.1943732865555,11.4732422824942,-4.1295495870785));
#30435=CARTESIAN_POINT('Ctrl Pts',(-48.2142367808631,11.5210597361567,-4.1297603359587));
#30436=CARTESIAN_POINT('Ctrl Pts',(-48.2616096994078,11.5740131518293,-4.13125738915642));
#30437=CARTESIAN_POINT('Ctrl Pts',(-48.2616069550931,11.5746245485739,-4.13831849503741));
#30438=CARTESIAN_POINT('',(-48.3299590485044,11.675660534618,-4.12660736370751));
#30439=CARTESIAN_POINT('Ctrl Pts',(-48.2616069550931,11.5746245485739,-4.13831849503741));
#30440=CARTESIAN_POINT('Ctrl Pts',(-48.2619179788887,11.5746245276893,-4.13475573974222));
#30441=CARTESIAN_POINT('Ctrl Pts',(-48.2763272274152,11.5884292819489,-4.13270208529043));
#30442=CARTESIAN_POINT('Ctrl Pts',(-48.3054382973461,11.6268390447666,-4.12928232258428));
#30443=CARTESIAN_POINT('Ctrl Pts',(-48.3199629155115,11.6516801004069,-4.12792406463103));
#30444=CARTESIAN_POINT('Ctrl Pts',(-48.3299590819566,11.6756605207397,-4.1266073649138));
#30445=CARTESIAN_POINT('Ctrl Pts',(-48.3299590819566,11.6756605207397,-4.1266073649138));
#30446=CARTESIAN_POINT('Ctrl Pts',(-48.3401597428651,11.6392592214936,-3.42489191358813));
#30447=CARTESIAN_POINT('Ctrl Pts',(-48.3448536058572,11.5986492866067,-2.72261955642498));
#30448=CARTESIAN_POINT('Ctrl Pts',(-48.3481589393795,11.5098560202878,-1.32104552555116));
#30449=CARTESIAN_POINT('Ctrl Pts',(-48.3539879394116,11.4835302569326,-0.619658818634546));
#30450=CARTESIAN_POINT('Ctrl Pts',(-48.353987706665,11.4728541727075,0.0824317919420715));
#30451=CARTESIAN_POINT('Ctrl Pts',(-48.353987706665,11.4728541727075,0.0824317919420715));
#30452=CARTESIAN_POINT('Ctrl Pts',(-48.3539881721588,11.4942063411577,0.082431791942142));
#30453=CARTESIAN_POINT('Ctrl Pts',(-48.3536309301586,11.5200575082527,0.0824317919434549));
#30454=CARTESIAN_POINT('Ctrl Pts',(-48.355396330448,11.5731362269333,0.0824317919411931));
#30455=CARTESIAN_POINT('Ctrl Pts',(-48.3539734316379,11.5876793312944,0.0824317919403744));
#30456=CARTESIAN_POINT('Ctrl Pts',(-48.3539734316379,11.6131136241746,0.0824317919394229));
#30457=CARTESIAN_POINT('Ctrl Pts',(-48.3539878230383,11.47819221482,-0.268613513346239));
#30458=CARTESIAN_POINT('Ctrl Pts',(-48.3539286009805,11.4971000233706,-0.190411564161195));
#30459=CARTESIAN_POINT('Ctrl Pts',(-48.3536285993105,11.5200113925673,-0.190198224429358));
#30460=CARTESIAN_POINT('Ctrl Pts',(-48.3553975542811,11.5731490589916,-0.228911446124229));
#30461=CARTESIAN_POINT('Ctrl Pts',(-48.3539734316379,11.5876793312944,-0.267838007548286));
#30462=CARTESIAN_POINT('Ctrl Pts',(-48.3539734316379,11.6131136241746,-0.267915860672084));
#30463=CARTESIAN_POINT('Ctrl Pts',(-48.3525306312169,11.4874426767151,-0.619482842719547));
#30464=CARTESIAN_POINT('Ctrl Pts',(-48.3536168471921,11.5031786713302,-0.486015179132629));
#30465=CARTESIAN_POINT('Ctrl Pts',(-48.353731882767,11.524500508176,-0.485651980041206));
#30466=CARTESIAN_POINT('Ctrl Pts',(-48.3555328010184,11.5776504745526,-0.55171778038672));
#30467=CARTESIAN_POINT('Ctrl Pts',(-48.3539734316379,11.5930695682598,-0.618146779821232));
#30468=CARTESIAN_POINT('Ctrl Pts',(-48.3539734316379,11.6169153282063,-0.61826351328359));
#30469=CARTESIAN_POINT('Ctrl Pts',(-48.3492030226972,11.5143737377389,-1.32089560268123));
#30470=CARTESIAN_POINT('Ctrl Pts',(-48.3523529181622,11.5255419633076,-1.12857563668694));
#30471=CARTESIAN_POINT('Ctrl Pts',(-48.3533876456339,11.5448479357173,-1.12801608518725));
#30472=CARTESIAN_POINT('Ctrl Pts',(-48.3554782973317,11.595969244612,-1.22311169405469));
#30473=CARTESIAN_POINT('Ctrl Pts',(-48.3539734316379,11.6126245374907,-1.31876685441994));
#30474=CARTESIAN_POINT('Ctrl Pts',(-48.3539734316379,11.632122144333,-1.31887631215363));
#30475=CARTESIAN_POINT('Ctrl Pts',(-48.3473326059989,11.5320543368675,-1.67143903326961));
#30476=CARTESIAN_POINT('Ctrl Pts',(-48.3514157821305,11.5418711528743,-1.47552932444613));
#30477=CARTESIAN_POINT('Ctrl Pts',(-48.3529551642544,11.5607507931984,-1.47492327989778));
#30478=CARTESIAN_POINT('Ctrl Pts',(-48.3552960665127,11.6098088718848,-1.57169769604833));
#30479=CARTESIAN_POINT('Ctrl Pts',(-48.353973431638,11.6267892697561,-1.6690781567457));
#30480=CARTESIAN_POINT('Ctrl Pts',(-48.353973431638,11.643527256428,-1.66914145841217));
#30481=CARTESIAN_POINT('Ctrl Pts',(-48.3448536058572,11.5986492866067,-2.72261955642498));
#30482=CARTESIAN_POINT('Ctrl Pts',(-48.3512462941311,11.612020620858,-2.6021779596111));
#30483=CARTESIAN_POINT('Ctrl Pts',(-48.353495101689,11.6290600690796,-2.60155209373665));
#30484=CARTESIAN_POINT('Ctrl Pts',(-48.3552756321719,11.6658592241822,-2.66041448169569));
#30485=CARTESIAN_POINT('Ctrl Pts',(-48.353973431638,11.6794362415567,-2.71990273552858));
#30486=CARTESIAN_POINT('Ctrl Pts',(-48.353973431638,11.689147704808,-2.71968937812887));
#30487=CARTESIAN_POINT('Ctrl Pts',(-48.3401597428651,11.6392592214936,-3.42489191358813));
#30488=CARTESIAN_POINT('Ctrl Pts',(-48.348156567804,11.6580360440914,-3.35294966330561));
#30489=CARTESIAN_POINT('Ctrl Pts',(-48.3516099899972,11.6785648284689,-3.3519488686722));
#30490=CARTESIAN_POINT('Ctrl Pts',(-48.3545184219142,11.7135824344711,-3.38562737891504));
#30491=CARTESIAN_POINT('Ctrl Pts',(-48.353973431638,11.7280712560958,-3.42030668379129));
#30492=CARTESIAN_POINT('Ctrl Pts',(-48.353973431638,11.734768153188,-3.41972463252812));
#30493=CARTESIAN_POINT('Ctrl Pts',(-48.3299590819566,11.6756605207398,-4.12660736491379));
#30494=CARTESIAN_POINT('Ctrl Pts',(-48.3399552484017,11.6996409410726,-4.12529066519656));
#30495=CARTESIAN_POINT('Ctrl Pts',(-48.3459588358221,11.7229366511894,-4.12399546447476));
#30496=CARTESIAN_POINT('Ctrl Pts',(-48.3529679274402,11.7642258753786,-4.12148173140903));
#30497=CARTESIAN_POINT('Ctrl Pts',(-48.3539734316379,11.7822193894509,-4.1202631990651));
#30498=CARTESIAN_POINT('Ctrl Pts',(-48.3539734316379,11.7955954176946,-4.1190998361036));
#30499=CARTESIAN_POINT('Ctrl Pts',(-48.3299589815999,11.6756605623745,-4.12660736129494));
#30500=CARTESIAN_POINT('Ctrl Pts',(-48.334075322032,11.685535483409,-4.12606515642765));
#30501=CARTESIAN_POINT('Ctrl Pts',(-48.3375652097276,11.6953464500616,-4.12552210528721));
#30502=CARTESIAN_POINT('Ctrl Pts',(-48.3404730684758,11.704904887613,-4.12498379119384));
#30503=CARTESIAN_POINT('Ctrl Pts',(-48.3435583735783,11.7150466099945,-4.12441262754291));
#30504=CARTESIAN_POINT('Ctrl Pts',(-48.3459891527135,11.7249027978758,-4.12384690527284));
#30505=CARTESIAN_POINT('Ctrl Pts',(-48.3478717153206,11.7342762879822,-4.12329089420766));
#30506=CARTESIAN_POINT('Ctrl Pts',(-48.3498402999992,11.7440780916192,-4.12270947669732));
#30507=CARTESIAN_POINT('Ctrl Pts',(-48.3512109703853,11.7533514160688,-4.12213873671569));
#30508=CARTESIAN_POINT('Ctrl Pts',(-48.3521436788015,11.7619163369653,-4.12157963240757));
#30509=CARTESIAN_POINT('Ctrl Pts',(-48.3531576213552,11.7712272187115,-4.12097183297083));
#30510=CARTESIAN_POINT('Ctrl Pts',(-48.3536562142594,11.7797008569823,-4.12037779232948));
#30511=CARTESIAN_POINT('Ctrl Pts',(-48.3538589494056,11.7871660424472,-4.11979354428953));
#30512=CARTESIAN_POINT('Ctrl Pts',(-48.3539396582106,11.7901379306941,-4.11956095530813));
#30513=CARTESIAN_POINT('Ctrl Pts',(-48.3539734295675,11.7929506159593,-4.1193298643544));
#30514=CARTESIAN_POINT('Ctrl Pts',(-48.3539734316378,11.7955954176947,-4.11909983610361));
#30515=CARTESIAN_POINT('Ctrl Pts',(-48.3539734316379,11.6131136241746,0.0824317919394229));
#30516=CARTESIAN_POINT('Ctrl Pts',(-48.3539734316379,11.5876793312944,0.0824317919403744));
#30517=CARTESIAN_POINT('Ctrl Pts',(-48.355396330448,11.5731362269333,0.0824317919411931));
#30518=CARTESIAN_POINT('Ctrl Pts',(-48.3536309301586,11.5200575082527,0.0824317919434549));
#30519=CARTESIAN_POINT('Ctrl Pts',(-48.3539881721588,11.4942063411577,0.082431791942142));
#30520=CARTESIAN_POINT('Ctrl Pts',(-48.353987706665,11.4728541727075,0.0824317919420715));
#30521=CARTESIAN_POINT('Ctrl Pts',(-48.353987706665,11.4728541727075,0.0824317919420715));
#30522=CARTESIAN_POINT('Ctrl Pts',(-48.3539878230386,11.47819221482,0.433477097230417));
#30523=CARTESIAN_POINT('Ctrl Pts',(-48.3525306312176,11.4874426767153,0.784346426604709));
#30524=CARTESIAN_POINT('Ctrl Pts',(-48.3492030226983,11.5143737377395,1.48575918657027));
#30525=CARTESIAN_POINT('Ctrl Pts',(-48.3473326060001,11.5320543368686,1.83630261716154));
#30526=CARTESIAN_POINT('Ctrl Pts',(-48.3448536058578,11.5986492866091,2.88748314032846));
#30527=CARTESIAN_POINT('Ctrl Pts',(-48.3401597428655,11.6392592214975,3.58975549751167));
#30528=CARTESIAN_POINT('Ctrl Pts',(-48.3299590819566,11.6756605207451,4.29147094885445));
#30529=CARTESIAN_POINT('Ctrl Pts',(-48.3539881721588,11.4942063411577,0.082431791942142));
#30530=CARTESIAN_POINT('Ctrl Pts',(-48.3539286009808,11.4971000233708,0.355275148045688));
#30531=CARTESIAN_POINT('Ctrl Pts',(-48.3536168471926,11.5031786713304,0.650878763018348));
#30532=CARTESIAN_POINT('Ctrl Pts',(-48.352352918163,11.5255419633083,1.2934392205762));
#30533=CARTESIAN_POINT('Ctrl Pts',(-48.3514157821314,11.5418711528752,1.64039290833772));
#30534=CARTESIAN_POINT('Ctrl Pts',(-48.3512462941313,11.6120206208596,2.76704154350989));
#30535=CARTESIAN_POINT('Ctrl Pts',(-48.348156567804,11.6580360440938,3.51781324721676));
#30536=CARTESIAN_POINT('Ctrl Pts',(-48.3399552484018,11.6996409410751,4.29015424910472));
#30537=CARTESIAN_POINT('Ctrl Pts',(-48.3536309301586,11.5200575082527,0.0824317919434549));
#30538=CARTESIAN_POINT('Ctrl Pts',(-48.3536285993108,11.5200113925675,0.355061808316268));
#30539=CARTESIAN_POINT('Ctrl Pts',(-48.3537318827671,11.5245005081763,0.650515563928747));
#30540=CARTESIAN_POINT('Ctrl Pts',(-48.3533876456339,11.5448479357178,1.29287966907655));
#30541=CARTESIAN_POINT('Ctrl Pts',(-48.352955164254,11.5607507931992,1.63978686378821));
#30542=CARTESIAN_POINT('Ctrl Pts',(-48.3534951016876,11.6290600690807,2.76641567763006));
#30543=CARTESIAN_POINT('Ctrl Pts',(-48.3516099899957,11.6785648284704,3.51681245257216));
#30544=CARTESIAN_POINT('Ctrl Pts',(-48.3459588358221,11.7229366511906,4.28885904836748));
#30545=CARTESIAN_POINT('Ctrl Pts',(-48.355396330448,11.5731362269333,0.0824317919411931));
#30546=CARTESIAN_POINT('Ctrl Pts',(-48.3553975542812,11.5731490589917,0.393775030006615));
#30547=CARTESIAN_POINT('Ctrl Pts',(-48.355532801018,11.5776504745527,0.716581364269289));
#30548=CARTESIAN_POINT('Ctrl Pts',(-48.35547829733,11.5959692446123,1.38797527793762));
#30549=CARTESIAN_POINT('Ctrl Pts',(-48.3552960665103,11.6098088718852,1.73656127993144));
#30550=CARTESIAN_POINT('Ctrl Pts',(-48.3552756321677,11.6658592241826,2.82527806557877));
#30551=CARTESIAN_POINT('Ctrl Pts',(-48.35451842191,11.7135824344715,3.55049096279885));
#30552=CARTESIAN_POINT('Ctrl Pts',(-48.3529679274402,11.7642258753785,4.28634531528709));
#30553=CARTESIAN_POINT('Ctrl Pts',(-48.3539734316379,11.5876793312944,0.0824317919403744));
#30554=CARTESIAN_POINT('Ctrl Pts',(-48.3539734316379,11.5876793312944,0.432701591429034));
#30555=CARTESIAN_POINT('Ctrl Pts',(-48.3539734316373,11.5930695682598,0.783010363701859));
#30556=CARTESIAN_POINT('Ctrl Pts',(-48.3539734316356,11.6126245374908,1.48363043830021));
#30557=CARTESIAN_POINT('Ctrl Pts',(-48.3539734316346,11.6267892697563,1.83394174062573));
#30558=CARTESIAN_POINT('Ctrl Pts',(-48.3539734316326,11.6794362415569,2.88476631940789));
#30559=CARTESIAN_POINT('Ctrl Pts',(-48.3539734316326,11.728071256096,3.58517026767012));
#30560=CARTESIAN_POINT('Ctrl Pts',(-48.3539734316379,11.7822193894509,4.28512678294395));
#30561=CARTESIAN_POINT('Ctrl Pts',(-48.3539734316379,11.6131136241746,0.0824317919394229));
#30562=CARTESIAN_POINT('Ctrl Pts',(-48.3539734316379,11.6131136241746,0.432779444550929));
#30563=CARTESIAN_POINT('Ctrl Pts',(-48.3539734316373,11.6169153282063,0.783127097162436));
#30564=CARTESIAN_POINT('Ctrl Pts',(-48.3539734316357,11.632122144333,1.48373989603248));
#30565=CARTESIAN_POINT('Ctrl Pts',(-48.3539734316348,11.643527256428,1.83400504229102));
#30566=CARTESIAN_POINT('Ctrl Pts',(-48.3539734316329,11.689147704808,2.88455296200771));
#30567=CARTESIAN_POINT('Ctrl Pts',(-48.3539734316329,11.734768153188,3.58458821640696));
#30568=CARTESIAN_POINT('Ctrl Pts',(-48.3539734316379,11.7955954176946,4.28396341998245));
#30569=CARTESIAN_POINT('',(-48.3299590484456,11.6756605346478,4.29147094764604));
#30570=CARTESIAN_POINT('Ctrl Pts',(-48.3539734316379,11.7955954176946,4.28396341998245));
#30571=CARTESIAN_POINT('Ctrl Pts',(-48.3539734263918,11.7889074035727,4.2845451014632));
#30572=CARTESIAN_POINT('Ctrl Pts',(-48.3537589209384,11.781142600467,4.28513386273919));
#30573=CARTESIAN_POINT('Ctrl Pts',(-48.3531105335782,11.7724551591809,4.28573553812961));
#30574=CARTESIAN_POINT('Ctrl Pts',(-48.3525182830083,11.7645198686933,4.28628512100966));
#30575=CARTESIAN_POINT('Ctrl Pts',(-48.3515621295827,11.7558145072651,4.28684550102065));
#30576=CARTESIAN_POINT('Ctrl Pts',(-48.3500742568563,11.7464987405109,4.2874174568295));
#30577=CARTESIAN_POINT('Ctrl Pts',(-48.348658585424,11.7376350355516,4.28796165761009));
#30578=CARTESIAN_POINT('Ctrl Pts',(-48.3467601168661,11.7282190174495,4.28851631181798));
#30579=CARTESIAN_POINT('Ctrl Pts',(-48.3442567970522,11.7184280696924,4.28907864596114));
#30580=CARTESIAN_POINT('Ctrl Pts',(-48.3418724781032,11.7091025563739,4.28961424830237));
#30581=CARTESIAN_POINT('Ctrl Pts',(-48.3389385395999,11.6994377386549,4.2901567453683));
#30582=CARTESIAN_POINT('Ctrl Pts',(-48.3353869859874,11.6896156896676,4.29070126749766));
#30583=CARTESIAN_POINT('Ctrl Pts',(-48.3337149896359,11.6849916766686,4.29095761700351));
#30584=CARTESIAN_POINT('Ctrl Pts',(-48.3319067473016,11.6803331677637,4.29121438526338));
#30585=CARTESIAN_POINT('Ctrl Pts',(-48.3299589814234,11.6756605624531,4.29147094522923));
#30586=CARTESIAN_POINT('Ctrl Pts',(-48.3299590819566,11.6756605207451,4.29147094885445));
#30587=CARTESIAN_POINT('Ctrl Pts',(-48.3401597428655,11.6392592214975,3.58975549751167));
#30588=CARTESIAN_POINT('Ctrl Pts',(-48.3448536058578,11.5986492866091,2.88748314032846));
#30589=CARTESIAN_POINT('Ctrl Pts',(-48.3481589393809,11.5098560202884,1.48590910943924));
#30590=CARTESIAN_POINT('Ctrl Pts',(-48.3539879394121,11.4835302569326,0.784522402518766));
#30591=CARTESIAN_POINT('Ctrl Pts',(-48.353987706665,11.4728541727075,0.0824317919420715));
#30592=CARTESIAN_POINT('Ctrl Pts',(-48.353987706665,11.4728541727075,0.0824317919420715));
#30593=CARTESIAN_POINT('Ctrl Pts',(-48.3539875902917,11.4675161305949,0.433477097230381));
#30594=CARTESIAN_POINT('Ctrl Pts',(-48.3525301621484,11.4659265087691,0.784574340176142));
#30595=CARTESIAN_POINT('Ctrl Pts',(-48.3427993417961,11.4643966328771,1.48689990373394));
#30596=CARTESIAN_POINT('Ctrl Pts',(-48.334525949587,11.4644563788108,1.83812822434599));
#30597=CARTESIAN_POINT('Ctrl Pts',(-48.2936298160723,11.4583384590299,2.89205060620861));
#30598=CARTESIAN_POINT('Ctrl Pts',(-48.2504292399278,11.4609474762042,3.59330337868711));
#30599=CARTESIAN_POINT('Ctrl Pts',(-48.1943732865555,11.4732422824942,4.29441317095732));
#30600=CARTESIAN_POINT('Ctrl Pts',(-48.3539878230386,11.47819221482,0.433477097230417));
#30601=CARTESIAN_POINT('Ctrl Pts',(-48.3530459746151,11.4749860898031,0.706493517511539));
#30602=CARTESIAN_POINT('Ctrl Pts',(-48.3509583174044,11.4745419834778,0.997581380074998));
#30603=CARTESIAN_POINT('Ctrl Pts',(-48.3410826227033,11.4744825705815,1.61268347055339));
#30604=CARTESIAN_POINT('Ctrl Pts',(-48.3332754508955,11.4748353413218,1.93670273340589));
#30605=CARTESIAN_POINT('Ctrl Pts',(-48.2931970947235,11.4700074930207,2.95333187696386));
#30606=CARTESIAN_POINT('Ctrl Pts',(-48.2516773067399,11.4731609516944,3.63027912148841));
#30607=CARTESIAN_POINT('Ctrl Pts',(-48.1993391601324,11.4851966459098,4.29446585817733));
#30608=CARTESIAN_POINT('Ctrl Pts',(-48.3525306312176,11.4874426767153,0.784346426604709));
#30609=CARTESIAN_POINT('Ctrl Pts',(-48.3513305951732,11.484480312248,0.997236186169142));
#30610=CARTESIAN_POINT('Ctrl Pts',(-48.3489425213275,11.4840908039499,1.24226674629595));
#30611=CARTESIAN_POINT('Ctrl Pts',(-48.3390430002284,11.4843329006938,1.78661204517143));
#30612=CARTESIAN_POINT('Ctrl Pts',(-48.3315028514989,11.484916621703,2.08593433632647));
#30613=CARTESIAN_POINT('Ctrl Pts',(-48.292586709085,11.4818828006799,3.05034122265968));
#30614=CARTESIAN_POINT('Ctrl Pts',(-48.2530217283574,11.4863352799679,3.69245653604367));
#30615=CARTESIAN_POINT('Ctrl Pts',(-48.2060243727241,11.4974720069511,4.29459893941723));
#30616=CARTESIAN_POINT('Ctrl Pts',(-48.3492030226983,11.5143737377395,1.48575918657027));
#30617=CARTESIAN_POINT('Ctrl Pts',(-48.34744628429,11.5105174196344,1.61112122690618));
#30618=CARTESIAN_POINT('Ctrl Pts',(-48.3443564161332,11.5090816899187,1.78530549799782));
#30619=CARTESIAN_POINT('Ctrl Pts',(-48.3339923326229,11.5079260458442,2.2092493439093));
#30620=CARTESIAN_POINT('Ctrl Pts',(-48.3266822404244,11.5081462764441,2.45901835923708));
#30621=CARTESIAN_POINT('Ctrl Pts',(-48.2905861997275,11.5065304546904,3.28859697249979));
#30622=CARTESIAN_POINT('Ctrl Pts',(-48.2556497470331,11.5121367174566,3.83761867075986));
#30623=CARTESIAN_POINT('Ctrl Pts',(-48.2204933169654,11.5208685373805,4.29515956957318));
#30624=CARTESIAN_POINT('Ctrl Pts',(-48.3473326060001,11.5320543368686,1.83630261716154));
#30625=CARTESIAN_POINT('Ctrl Pts',(-48.3452802018698,11.5270830007426,1.93426197941878));
#30626=CARTESIAN_POINT('Ctrl Pts',(-48.3417903805473,11.5245577996659,2.08365645412851));
#30627=CARTESIAN_POINT('Ctrl Pts',(-48.3309866294069,11.5217114161952,2.45795503134133));
#30628=CARTESIAN_POINT('Ctrl Pts',(-48.3236392145334,11.5213343690961,2.68286794498518));
#30629=CARTESIAN_POINT('Ctrl Pts',(-48.2891989250295,11.5193254972085,3.42984175707725));
#30630=CARTESIAN_POINT('Ctrl Pts',(-48.2569333440914,11.5247638266718,3.9206033909208));
#30631=CARTESIAN_POINT('Ctrl Pts',(-48.2282770486149,11.5319897067687,4.29558711848924));
#30632=CARTESIAN_POINT('Ctrl Pts',(-48.3448536058578,11.5986492866091,2.88748314032846));
#30633=CARTESIAN_POINT('Ctrl Pts',(-48.3416407744856,11.5919036248663,2.94770884760779));
#30634=CARTESIAN_POINT('Ctrl Pts',(-48.3366078655353,11.5859418512212,3.04468476960679));
#30635=CARTESIAN_POINT('Ctrl Pts',(-48.3235830580242,11.5755468354636,3.28398547908769));
#30636=CARTESIAN_POINT('Ctrl Pts',(-48.3155720251457,11.5710816706623,3.42631530150717));
#30637=CARTESIAN_POINT('Ctrl Pts',(-48.2851290641413,11.5598336028535,3.87910730684837));
#30638=CARTESIAN_POINT('Ctrl Pts',(-48.260312597172,11.5581209387927,4.15637445295875));
#30639=CARTESIAN_POINT('Ctrl Pts',(-48.2497657836928,11.5609276470972,4.29751198620621));
#30640=CARTESIAN_POINT('Ctrl Pts',(-48.3401597428655,11.6392592214975,3.58975549751167));
#30641=CARTESIAN_POINT('Ctrl Pts',(-48.3361613303963,11.6298708101994,3.62572662265912));
#30642=CARTESIAN_POINT('Ctrl Pts',(-48.3302694596963,11.6209827896646,3.68769531794308));
#30643=CARTESIAN_POINT('Ctrl Pts',(-48.3160467256828,11.6050189470302,3.83329117884303));
#30644=CARTESIAN_POINT('Ctrl Pts',(-48.3077158623693,11.5979431249306,3.91691834445902));
#30645=CARTESIAN_POINT('Ctrl Pts',(-48.2810866692805,11.5806510816468,4.15478254189364));
#30646=CARTESIAN_POINT('Ctrl Pts',(-48.2619367151001,11.5743267261738,4.29597769639093));
#30647=CARTESIAN_POINT('Ctrl Pts',(-48.2616083272502,11.5743188502015,4.29965152597593));
#30648=CARTESIAN_POINT('Ctrl Pts',(-48.3299590819566,11.6756605207451,4.29147094885445));
#30649=CARTESIAN_POINT('Ctrl Pts',(-48.3249609987341,11.6636703105801,4.29212929872931));
#30650=CARTESIAN_POINT('Ctrl Pts',(-48.3188308025814,11.6514649415887,4.29279803816797));
#30651=CARTESIAN_POINT('Ctrl Pts',(-48.3054305681461,11.6282480883359,4.29423381244547));
#30652=CARTESIAN_POINT('Ctrl Pts',(-48.2981605298634,11.6172366040747,4.29500084728431));
#30653=CARTESIAN_POINT('Ctrl Pts',(-48.2763272274152,11.588429281961,4.29756566931001));
#30654=CARTESIAN_POINT('Ctrl Pts',(-48.2619179788887,11.5746245276893,4.29961932362103));
#30655=CARTESIAN_POINT('Ctrl Pts',(-48.2616069550931,11.5746245485739,4.30318207891624));
#30656=CARTESIAN_POINT('Ctrl Pts',(-48.3299590819566,11.6756605207451,4.29147094885445));
#30657=CARTESIAN_POINT('Ctrl Pts',(-48.3199629155115,11.6516801004151,4.29278764860417));
#30658=CARTESIAN_POINT('Ctrl Pts',(-48.3054382973461,11.6268390447792,4.29414590660908));
#30659=CARTESIAN_POINT('Ctrl Pts',(-48.2763272274152,11.588429281961,4.29756566931001));
#30660=CARTESIAN_POINT('Ctrl Pts',(-48.2619179788887,11.5746245276893,4.29961932362103));
#30661=CARTESIAN_POINT('Ctrl Pts',(-48.2616069550931,11.5746245485739,4.30318207891625));
#30662=CARTESIAN_POINT('',(-48.1943732865555,11.4732422824942,4.29441317095733));
#30663=CARTESIAN_POINT('Ctrl Pts',(-48.1943732865555,11.4732422824942,4.29441317095732));
#30664=CARTESIAN_POINT('Ctrl Pts',(-48.196487864659,11.4783327131562,4.29443560633351));
#30665=CARTESIAN_POINT('Ctrl Pts',(-48.1988424763931,11.4833192247691,4.29447185544362));
#30666=CARTESIAN_POINT('Ctrl Pts',(-48.2013545801683,11.4882155712552,4.2945249560433));
#30667=CARTESIAN_POINT('Ctrl Pts',(-48.204468050974,11.4942840434216,4.29459076827944));
#30668=CARTESIAN_POINT('Ctrl Pts',(-48.2078249701059,11.5002159027501,4.29468221538989));
#30669=CARTESIAN_POINT('Ctrl Pts',(-48.2113461926006,11.5060421521798,4.29480804329398));
#30670=CARTESIAN_POINT('Ctrl Pts',(-48.2119784181535,11.5070882388083,4.29483063533874));
#30671=CARTESIAN_POINT('Ctrl Pts',(-48.2126160717519,11.5081308970756,4.29485434887851));
#30672=CARTESIAN_POINT('Ctrl Pts',(-48.2132588448447,11.5091702721658,4.29487925449521));
#30673=CARTESIAN_POINT('Ctrl Pts',(-48.2172981689735,11.5157019284025,4.29503576673815));
#30674=CARTESIAN_POINT('Ctrl Pts',(-48.2215368905597,11.5221052410797,4.29523764753415));
#30675=CARTESIAN_POINT('Ctrl Pts',(-48.2259211554775,11.5284062451254,4.29551276580963));
#30676=CARTESIAN_POINT('Ctrl Pts',(-48.2290245093856,11.5328663418341,4.29570750526799));
#30677=CARTESIAN_POINT('Ctrl Pts',(-48.2322009933063,11.5372739115821,4.29593860844117));
#30678=CARTESIAN_POINT('Ctrl Pts',(-48.2354399603075,11.5416356868782,4.29622874106156));
#30679=CARTESIAN_POINT('Ctrl Pts',(-48.2381803964523,11.5453261124591,4.29647421744937));
#30680=CARTESIAN_POINT('Ctrl Pts',(-48.2409650173885,11.5489827466928,4.29676073668963));
#30681=CARTESIAN_POINT('Ctrl Pts',(-48.2437875269064,11.5526057362471,4.29712165145316));
#30682=CARTESIAN_POINT('Ctrl Pts',(-48.2458021197089,11.5551916792292,4.29737925777134));
#30683=CARTESIAN_POINT('Ctrl Pts',(-48.2478368856971,11.5577614675671,4.29767390515738));
#30684=CARTESIAN_POINT('Ctrl Pts',(-48.2498887314464,11.5603135612093,4.29803922268809));
#30685=CARTESIAN_POINT('Ctrl Pts',(-48.2513195940382,11.5620932736095,4.29829397828509));
#30686=CARTESIAN_POINT('Ctrl Pts',(-48.2527589064005,11.5638644687507,4.29858198823371));
#30687=CARTESIAN_POINT('Ctrl Pts',(-48.254204885756,11.5656264211453,4.29893754450221));
#30688=CARTESIAN_POINT('Ctrl Pts',(-48.2551766147946,11.5668104908209,4.29917648591561));
#30689=CARTESIAN_POINT('Ctrl Pts',(-48.256151771226,11.5679907811658,4.29944485081465));
#30690=CARTESIAN_POINT('Ctrl Pts',(-48.257126565722,11.5691644697714,4.29977599704979));
#30691=CARTESIAN_POINT('Ctrl Pts',(-48.2577142195889,11.5698720267494,4.29997562821966));
#30692=CARTESIAN_POINT('Ctrl Pts',(-48.2583022378277,11.5705777201803,4.30019764216591));
#30693=CARTESIAN_POINT('Ctrl Pts',(-48.2588872441424,11.5712791301838,4.30046624970369));
#30694=CARTESIAN_POINT('Ctrl Pts',(-48.2592662088748,11.5717335007565,4.30064025258387));
#30695=CARTESIAN_POINT('Ctrl Pts',(-48.2596450908386,11.572187424288,4.30083381477504));
#30696=CARTESIAN_POINT('Ctrl Pts',(-48.2600166453457,11.5726339419601,4.30106614290028));
#30697=CARTESIAN_POINT('Ctrl Pts',(-48.2602186580187,11.5728767118007,4.30119245875618));
#30698=CARTESIAN_POINT('Ctrl Pts',(-48.2604197722893,11.5731188229199,4.3013312052759));
#30699=CARTESIAN_POINT('Ctrl Pts',(-48.2606142273849,11.5733542339528,4.30148923677993));
#30700=CARTESIAN_POINT('Ctrl Pts',(-48.2607720584956,11.5735453072939,4.30161750437682));
#30701=CARTESIAN_POINT('Ctrl Pts',(-48.2609257038798,11.5737321635395,4.30175813254586));
#30702=CARTESIAN_POINT('Ctrl Pts',(-48.2610695236536,11.5739092744934,4.30192109628311));
#30703=CARTESIAN_POINT('Ctrl Pts',(-48.2611414335404,11.5739978299704,4.30200257815174));
#30704=CARTESIAN_POINT('Ctrl Pts',(-48.2612094962467,11.5740821529245,4.30208695578815));
#30705=CARTESIAN_POINT('Ctrl Pts',(-48.261281040375,11.5741721054102,4.30219266734828));
#30706=CARTESIAN_POINT('Ctrl Pts',(-48.2613168124392,11.5742170816531,4.30224552312834));
#30707=CARTESIAN_POINT('Ctrl Pts',(-48.2613523347546,11.5742618826269,4.30229992241309));
#30708=CARTESIAN_POINT('Ctrl Pts',(-48.2614004758006,11.5743239422312,4.30239026429631));
#30709=CARTESIAN_POINT('Ctrl Pts',(-48.2614245463109,11.574354972017,4.30243543521408));
#30710=CARTESIAN_POINT('Ctrl Pts',(-48.2614593265161,11.5743996848319,4.30249945951758));
#30711=CARTESIAN_POINT('Ctrl Pts',(-48.2615035948095,11.5744597225481,4.30261831732649));
#30712=CARTESIAN_POINT('Ctrl Pts',(-48.2615361811056,11.5745039168608,4.30270580964811));
#30713=CARTESIAN_POINT('Ctrl Pts',(-48.2615743374215,11.5745568559738,4.30282296938909));
#30714=CARTESIAN_POINT('Ctrl Pts',(-48.2615948384317,11.5745940265263,4.30298682659291));
#30715=CARTESIAN_POINT('Ctrl Pts',(-48.2616021879244,11.5746073519527,4.30304556844533));
#30716=CARTESIAN_POINT('Ctrl Pts',(-48.2616069829336,11.5746183373345,4.30311034495461));
#30717=CARTESIAN_POINT('Ctrl Pts',(-48.2616069550935,11.5746245484993,4.30318207805534));
#30718=CARTESIAN_POINT('Ctrl Pts',(-48.1943732865555,11.4732422824942,4.29441317095733));
#30719=CARTESIAN_POINT('Ctrl Pts',(-48.2504292399278,11.4609474762042,3.59330337868711));
#30720=CARTESIAN_POINT('Ctrl Pts',(-48.2936298160723,11.4583384590299,2.89205060620861));
#30721=CARTESIAN_POINT('Ctrl Pts',(-48.3481579940919,11.4664956854044,1.48682076372511));
#30722=CARTESIAN_POINT('Ctrl Pts',(-48.3539874739184,11.4621780884823,0.78452240251869));
#30723=CARTESIAN_POINT('Ctrl Pts',(-48.353987706665,11.4728541727075,0.0824317919420715));
#30724=CARTESIAN_POINT('Ctrl Pts',(0.0835265683594526,11.4728541727075,
-48.3550824830876));
#30725=CARTESIAN_POINT('Ctrl Pts',(0.0835265683593817,11.4942063411577,
-48.3550829485814));
#30726=CARTESIAN_POINT('Ctrl Pts',(0.0835265683580835,11.5200575082527,
-48.3547257065812));
#30727=CARTESIAN_POINT('Ctrl Pts',(0.0835265683603323,11.5731362269333,
-48.3564911068706));
#30728=CARTESIAN_POINT('Ctrl Pts',(0.0835265683611482,11.5876793312944,
-48.3550682080606));
#30729=CARTESIAN_POINT('Ctrl Pts',(0.0835265683620996,11.6131136241746,
-48.3550682080606));
#30730=CARTESIAN_POINT('Ctrl Pts',(0.434571873647755,11.4781922148201,-48.3550825994612));
#30731=CARTESIAN_POINT('Ctrl Pts',(0.356369924462715,11.4971000233707,-48.3550233774034));
#30732=CARTESIAN_POINT('Ctrl Pts',(0.356156584730894,11.5200113925674,-48.3547233757333));
#30733=CARTESIAN_POINT('Ctrl Pts',(0.394869806425756,11.5731490589917,-48.3564923307038));
#30734=CARTESIAN_POINT('Ctrl Pts',(0.433796367849811,11.5876793312944,-48.3550682080606));
#30735=CARTESIAN_POINT('Ctrl Pts',(0.433874220973609,11.6131136241746,-48.3550682080606));
#30736=CARTESIAN_POINT('Ctrl Pts',(0.785441203021056,11.4874426767152,-48.3536254076401));
#30737=CARTESIAN_POINT('Ctrl Pts',(0.651973539434153,11.5031786713302,-48.3547116236151));
#30738=CARTESIAN_POINT('Ctrl Pts',(0.651610340342747,11.5245005081761,-48.3548266591899));
#30739=CARTESIAN_POINT('Ctrl Pts',(0.717676140688252,11.5776504745526,-48.3566275774411));
#30740=CARTESIAN_POINT('Ctrl Pts',(0.78410514012276,11.5930695682598,-48.3550682080606));
#30741=CARTESIAN_POINT('Ctrl Pts',(0.784221873585119,11.6169153282063,-48.3550682080606));
#30742=CARTESIAN_POINT('Ctrl Pts',(1.48685396298274,11.5143737377389,-48.3502977991207));
#30743=CARTESIAN_POINT('Ctrl Pts',(1.29453399698848,11.5255419633077,-48.3534476945855));
#30744=CARTESIAN_POINT('Ctrl Pts',(1.29397444548881,11.5448479357173,-48.354482422057));
#30745=CARTESIAN_POINT('Ctrl Pts',(1.38907005435624,11.5959692446121,-48.3565730737545));
#30746=CARTESIAN_POINT('Ctrl Pts',(1.48472521472147,11.6126245374907,-48.3550682080606));
#30747=CARTESIAN_POINT('Ctrl Pts',(1.48483467245517,11.632122144333,-48.3550682080606));
#30748=CARTESIAN_POINT('Ctrl Pts',(1.83739739357112,11.5320543368675,-48.3484273824224));
#30749=CARTESIAN_POINT('Ctrl Pts',(1.64148768474769,11.5418711528743,-48.3525105585539));
#30750=CARTESIAN_POINT('Ctrl Pts',(1.64088164019935,11.5607507931985,-48.3540499406775));
#30751=CARTESIAN_POINT('Ctrl Pts',(1.73765605634988,11.6098088718849,-48.3563908429355));
#30752=CARTESIAN_POINT('Ctrl Pts',(1.83503651704724,11.6267892697561,-48.3550682080606));
#30753=CARTESIAN_POINT('Ctrl Pts',(1.83509981871371,11.643527256428,-48.3550682080606));
#30754=CARTESIAN_POINT('Ctrl Pts',(2.88857791672651,11.5986492866067,-48.3459483822799));
#30755=CARTESIAN_POINT('Ctrl Pts',(2.7681363199127,11.612020620858,-48.3523410705538));
#30756=CARTESIAN_POINT('Ctrl Pts',(2.76751045403826,11.6290600690796,-48.3545898781116));
#30757=CARTESIAN_POINT('Ctrl Pts',(2.82637284199726,11.6658592241822,-48.3563704085945));
#30758=CARTESIAN_POINT('Ctrl Pts',(2.88586109583013,11.6794362415567,-48.3550682080606));
#30759=CARTESIAN_POINT('Ctrl Pts',(2.88564773843041,11.689147704808,-48.3550682080606));
#30760=CARTESIAN_POINT('Ctrl Pts',(3.59085027388967,11.6392592214936,-48.3412545192878));
#30761=CARTESIAN_POINT('Ctrl Pts',(3.51890802360723,11.6580360440914,-48.3492513442266));
#30762=CARTESIAN_POINT('Ctrl Pts',(3.51790722897382,11.6785648284689,-48.3527047664198));
#30763=CARTESIAN_POINT('Ctrl Pts',(3.55158573921662,11.7135824344711,-48.3556131983368));
#30764=CARTESIAN_POINT('Ctrl Pts',(3.58626504409284,11.7280712560958,-48.3550682080606));
#30765=CARTESIAN_POINT('Ctrl Pts',(3.58568299282967,11.734768153188,-48.3550682080606));
#30766=CARTESIAN_POINT('Ctrl Pts',(4.29256572521535,11.6756605207398,-48.3310538583792));
#30767=CARTESIAN_POINT('Ctrl Pts',(4.29124902549811,11.6996409410726,-48.3410500248244));
#30768=CARTESIAN_POINT('Ctrl Pts',(4.28995382477632,11.7229366511894,-48.3470536122447));
#30769=CARTESIAN_POINT('Ctrl Pts',(4.28744009171059,11.7642258753786,-48.3540627038628));
#30770=CARTESIAN_POINT('Ctrl Pts',(4.28622155936666,11.7822193894509,-48.3550682080606));
#30771=CARTESIAN_POINT('Ctrl Pts',(4.28505819640515,11.7955954176946,-48.3550682080606));
#30772=CARTESIAN_POINT('',(4.29256572400907,11.675660534618,-48.3310538249271));
#30773=CARTESIAN_POINT('',(0.0835265683594526,11.4728541727075,-48.3550824830876));
#30774=CARTESIAN_POINT('Ctrl Pts',(4.29256572521535,11.6756605207397,-48.3310538583792));
#30775=CARTESIAN_POINT('Ctrl Pts',(3.59085027388967,11.6392592214936,-48.3412545192878));
#30776=CARTESIAN_POINT('Ctrl Pts',(2.88857791672651,11.5986492866067,-48.3459483822799));
#30777=CARTESIAN_POINT('Ctrl Pts',(1.48700388585266,11.5098560202878,-48.3492537158032));
#30778=CARTESIAN_POINT('Ctrl Pts',(0.785617178936058,11.4835302569327,-48.3550827158346));
#30779=CARTESIAN_POINT('Ctrl Pts',(0.0835265683594526,11.4728541727075,
-48.3550824830876));
#30780=CARTESIAN_POINT('Ctrl Pts',(4.2925657215965,11.6756605623744,-48.3310537580229));
#30781=CARTESIAN_POINT('Ctrl Pts',(4.29202351672922,11.6855354834088,-48.3351700984549));
#30782=CARTESIAN_POINT('Ctrl Pts',(4.29148046558877,11.6953464500614,-48.3386599861505));
#30783=CARTESIAN_POINT('Ctrl Pts',(4.2909421514954,11.7049048876128,-48.3415678448987));
#30784=CARTESIAN_POINT('Ctrl Pts',(4.29037098784448,11.7150466099943,-48.3446531500012));
#30785=CARTESIAN_POINT('Ctrl Pts',(4.28980526557442,11.7249027978756,-48.3470839291363));
#30786=CARTESIAN_POINT('Ctrl Pts',(4.28924925450923,11.734276287982,-48.3489664917434));
#30787=CARTESIAN_POINT('Ctrl Pts',(4.28866783699889,11.7440780916189,-48.350935076422));
#30788=CARTESIAN_POINT('Ctrl Pts',(4.28809709701726,11.7533514160685,-48.3523057468082));
#30789=CARTESIAN_POINT('Ctrl Pts',(4.28753799270913,11.7619163369651,-48.3532384552243));
#30790=CARTESIAN_POINT('Ctrl Pts',(4.28693019327239,11.7712272187112,-48.3542523977779));
#30791=CARTESIAN_POINT('Ctrl Pts',(4.28633615263105,11.779700856982,-48.3547509906821));
#30792=CARTESIAN_POINT('Ctrl Pts',(4.28575190459109,11.7871660424469,-48.3549537258283));
#30793=CARTESIAN_POINT('Ctrl Pts',(4.28551931560969,11.7901379306939,-48.3550344346333));
#30794=CARTESIAN_POINT('Ctrl Pts',(4.28528822465595,11.7929506159592,-48.3550682059901));
#30795=CARTESIAN_POINT('Ctrl Pts',(4.28505819640516,11.7955954176946,-48.3550682080605));
#30796=CARTESIAN_POINT('Ctrl Pts',(0.0835265683620996,11.6131136241746,
-48.3550682080606));
#30797=CARTESIAN_POINT('Ctrl Pts',(0.0835265683611482,11.5876793312944,
-48.3550682080606));
#30798=CARTESIAN_POINT('Ctrl Pts',(0.0835265683603323,11.5731362269333,
-48.3564911068706));
#30799=CARTESIAN_POINT('Ctrl Pts',(0.0835265683580835,11.5200575082527,
-48.3547257065812));
#30800=CARTESIAN_POINT('Ctrl Pts',(0.0835265683593817,11.4942063411577,
-48.3550829485814));
#30801=CARTESIAN_POINT('Ctrl Pts',(0.0835265683594526,11.4728541727075,
-48.3550824830876));
#30802=CARTESIAN_POINT('Ctrl Pts',(0.0835265683594526,11.4728541727075,
-48.3550824830876));
#30803=CARTESIAN_POINT('Ctrl Pts',(-0.267518736928885,11.47819221482,-48.3550825994609));
#30804=CARTESIAN_POINT('Ctrl Pts',(-0.618388066303173,11.4874426767152,
-48.3536254076396));
#30805=CARTESIAN_POINT('Ctrl Pts',(-1.31980082626874,11.5143737377395,-48.3502977991201));
#30806=CARTESIAN_POINT('Ctrl Pts',(-1.67034425686001,11.5320543368685,-48.3484273824219));
#30807=CARTESIAN_POINT('Ctrl Pts',(-2.72152478002693,11.598649286609,-48.3459483822804));
#30808=CARTESIAN_POINT('Ctrl Pts',(-3.42379713721014,11.6392592214975,-48.3412545192881));
#30809=CARTESIAN_POINT('Ctrl Pts',(-4.12551258855296,11.6756605207451,-48.3310538583792));
#30810=CARTESIAN_POINT('Ctrl Pts',(0.0835265683593817,11.4942063411577,
-48.3550829485814));
#30811=CARTESIAN_POINT('Ctrl Pts',(-0.189316787744158,11.4971000233707,
-48.3550233774032));
#30812=CARTESIAN_POINT('Ctrl Pts',(-0.484920402716805,11.5031786713304,
-48.3547116236149));
#30813=CARTESIAN_POINT('Ctrl Pts',(-1.12748086027463,11.5255419633083,-48.353447694585));
#30814=CARTESIAN_POINT('Ctrl Pts',(-1.47443454803614,11.5418711528751,-48.3525105585533));
#30815=CARTESIAN_POINT('Ctrl Pts',(-2.60108318320828,11.6120206208596,-48.3523410705539));
#30816=CARTESIAN_POINT('Ctrl Pts',(-3.35185488691515,11.6580360440938,-48.3492513442266));
#30817=CARTESIAN_POINT('Ctrl Pts',(-4.12419588880323,11.6996409410751,-48.3410500248244));
#30818=CARTESIAN_POINT('Ctrl Pts',(0.0835265683580835,11.5200575082527,
-48.3547257065812));
#30819=CARTESIAN_POINT('Ctrl Pts',(-0.189103448014727,11.5200113925675,
-48.3547233757333));
#30820=CARTESIAN_POINT('Ctrl Pts',(-0.484557203627196,11.5245005081763,
-48.3548266591895));
#30821=CARTESIAN_POINT('Ctrl Pts',(-1.12692130877498,11.5448479357178,-48.354482422056));
#30822=CARTESIAN_POINT('Ctrl Pts',(-1.47382850348662,11.5607507931991,-48.3540499406762));
#30823=CARTESIAN_POINT('Ctrl Pts',(-2.60045731732845,11.6290600690807,-48.3545898781102));
#30824=CARTESIAN_POINT('Ctrl Pts',(-3.35085409227056,11.6785648284704,-48.3527047664183));
#30825=CARTESIAN_POINT('Ctrl Pts',(-4.12290068806598,11.7229366511906,-48.3470536122447));
#30826=CARTESIAN_POINT('Ctrl Pts',(0.0835265683603323,11.5731362269333,
-48.3564911068706));
#30827=CARTESIAN_POINT('Ctrl Pts',(-0.227816669705091,11.5731490589917,
-48.3564923307038));
#30828=CARTESIAN_POINT('Ctrl Pts',(-0.550623003967762,11.5776504745528,
-48.3566275774405));
#30829=CARTESIAN_POINT('Ctrl Pts',(-1.22201691763608,11.5959692446123,-48.3565730737525));
#30830=CARTESIAN_POINT('Ctrl Pts',(-1.5706029196299,11.6098088718852,-48.3563908429328));
#30831=CARTESIAN_POINT('Ctrl Pts',(-2.65931970527722,11.6658592241826,-48.3563704085904));
#30832=CARTESIAN_POINT('Ctrl Pts',(-3.3845326024973,11.7135824344715,-48.3556131983326));
#30833=CARTESIAN_POINT('Ctrl Pts',(-4.12038695498559,11.7642258753785,-48.3540627038628));
#30834=CARTESIAN_POINT('Ctrl Pts',(0.0835265683611482,11.5876793312944,
-48.3550682080606));
#30835=CARTESIAN_POINT('Ctrl Pts',(-0.266743231127515,11.5876793312944,
-48.3550682080606));
#30836=CARTESIAN_POINT('Ctrl Pts',(-0.617052003400343,11.5930695682598,
-48.3550682080599));
#30837=CARTESIAN_POINT('Ctrl Pts',(-1.31767207799869,11.6126245374908,-48.3550682080582));
#30838=CARTESIAN_POINT('Ctrl Pts',(-1.66798338032422,11.6267892697563,-48.3550682080572));
#30839=CARTESIAN_POINT('Ctrl Pts',(-2.71880795910639,11.6794362415569,-48.3550682080552));
#30840=CARTESIAN_POINT('Ctrl Pts',(-3.41921190736862,11.728071256096,-48.3550682080552));
#30841=CARTESIAN_POINT('Ctrl Pts',(-4.11916842264246,11.7822193894509,-48.3550682080606));
#30842=CARTESIAN_POINT('Ctrl Pts',(0.0835265683620996,11.6131136241746,
-48.3550682080606));
#30843=CARTESIAN_POINT('Ctrl Pts',(-0.26682108424941,11.6131136241746,-48.3550682080606));
#30844=CARTESIAN_POINT('Ctrl Pts',(-0.617168736860919,11.6169153282063,
-48.35506820806));
#30845=CARTESIAN_POINT('Ctrl Pts',(-1.31778153573097,11.632122144333,-48.3550682080584));
#30846=CARTESIAN_POINT('Ctrl Pts',(-1.66804668198951,11.643527256428,-48.3550682080574));
#30847=CARTESIAN_POINT('Ctrl Pts',(-2.71859460170621,11.689147704808,-48.3550682080555));
#30848=CARTESIAN_POINT('Ctrl Pts',(-3.41862985610546,11.734768153188,-48.3550682080555));
#30849=CARTESIAN_POINT('Ctrl Pts',(-4.11800505968095,11.7955954176946,-48.3550682080606));
#30850=CARTESIAN_POINT('',(-4.12551258734455,11.6756605346478,-48.3310538248682));
#30851=CARTESIAN_POINT('Ctrl Pts',(-4.11800505968096,11.7955954176946,-48.3550682080605));
#30852=CARTESIAN_POINT('Ctrl Pts',(-4.11858674116171,11.7889074035727,-48.3550682028144));
#30853=CARTESIAN_POINT('Ctrl Pts',(-4.1191755024377,11.7811426004669,-48.3548536973611));
#30854=CARTESIAN_POINT('Ctrl Pts',(-4.11977717782812,11.7724551591809,-48.3542053100008));
#30855=CARTESIAN_POINT('Ctrl Pts',(-4.12032676070816,11.7645198686933,-48.353613059431));
#30856=CARTESIAN_POINT('Ctrl Pts',(-4.12088714071915,11.7558145072651,-48.3526569060054));
#30857=CARTESIAN_POINT('Ctrl Pts',(-4.121459096528,11.746498740511,-48.351169033279));
#30858=CARTESIAN_POINT('Ctrl Pts',(-4.12200329730859,11.7376350355518,-48.3497533618467));
#30859=CARTESIAN_POINT('Ctrl Pts',(-4.12255795151647,11.7282190174497,-48.3478548932889));
#30860=CARTESIAN_POINT('Ctrl Pts',(-4.12312028565963,11.7184280696927,-48.345351573475));
#30861=CARTESIAN_POINT('Ctrl Pts',(-4.12365588800086,11.7091025563741,-48.342967254526));
#30862=CARTESIAN_POINT('Ctrl Pts',(-4.12419838506679,11.6994377386552,-48.3400333160227));
#30863=CARTESIAN_POINT('Ctrl Pts',(-4.12474290719614,11.689615689668,-48.3364817624102));
#30864=CARTESIAN_POINT('Ctrl Pts',(-4.124999256702,11.6849916766689,-48.3348097660587));
#30865=CARTESIAN_POINT('Ctrl Pts',(-4.12525602496188,11.6803331677638,-48.3330015237243));
#30866=CARTESIAN_POINT('Ctrl Pts',(-4.12551258492773,11.6756605624531,-48.3310537578461));
#30867=CARTESIAN_POINT('Ctrl Pts',(-4.12551258855296,11.6756605207451,-48.3310538583792));
#30868=CARTESIAN_POINT('Ctrl Pts',(-3.42379713721014,11.6392592214975,-48.3412545192881));
#30869=CARTESIAN_POINT('Ctrl Pts',(-2.72152478002693,11.598649286609,-48.3459483822803));
#30870=CARTESIAN_POINT('Ctrl Pts',(-1.3199507491377,11.5098560202884,-48.3492537158024));
#30871=CARTESIAN_POINT('Ctrl Pts',(-0.618564042217223,11.4835302569325,
-48.3550827158344));
#30872=CARTESIAN_POINT('Ctrl Pts',(0.0835265683594526,11.4728541727075,
-48.3550824830876));
#30873=CARTESIAN_POINT('Ctrl Pts',(0.0835265683594526,11.4728541727075,
-48.3550824830876));
#30874=CARTESIAN_POINT('Ctrl Pts',(-0.267518736928849,11.4675161305949,
-48.355082366714));
#30875=CARTESIAN_POINT('Ctrl Pts',(-0.618615979874604,11.4659265087691,
-48.3536249385705));
#30876=CARTESIAN_POINT('Ctrl Pts',(-1.32094154343241,11.464396632877,-48.3438941182179));
#30877=CARTESIAN_POINT('Ctrl Pts',(-1.67216986404445,11.4644563788108,-48.3356207260088));
#30878=CARTESIAN_POINT('Ctrl Pts',(-2.7260922459071,11.4583384590299,-48.2947245924949));
#30879=CARTESIAN_POINT('Ctrl Pts',(-3.42734501838564,11.4609474762042,-48.2515240163504));
#30880=CARTESIAN_POINT('Ctrl Pts',(-4.12845481065586,11.4732422824942,-48.1954680629781));
#30881=CARTESIAN_POINT('Ctrl Pts',(-0.267518736928885,11.47819221482,-48.3550825994609));
#30882=CARTESIAN_POINT('Ctrl Pts',(-0.540535157210003,11.474986089803,-48.3541407510372));
#30883=CARTESIAN_POINT('Ctrl Pts',(-0.831623019773455,11.4745419834778,
-48.3520530938263));
#30884=CARTESIAN_POINT('Ctrl Pts',(-1.44672511025184,11.4744825705814,-48.3421773991251));
#30885=CARTESIAN_POINT('Ctrl Pts',(-1.77074437310434,11.4748353413217,-48.3343702273172));
#30886=CARTESIAN_POINT('Ctrl Pts',(-2.78737351666232,11.4700074930206,-48.294291871146));
#30887=CARTESIAN_POINT('Ctrl Pts',(-3.4643207611869,11.4731609516944,-48.2527720831625));
#30888=CARTESIAN_POINT('Ctrl Pts',(-4.12850749787586,11.4851966459098,-48.200433936555));
#30889=CARTESIAN_POINT('Ctrl Pts',(-0.618388066303173,11.4874426767152,
-48.3536254076396));
#30890=CARTESIAN_POINT('Ctrl Pts',(-0.831277825867611,11.484480312248,-48.3524253715951));
#30891=CARTESIAN_POINT('Ctrl Pts',(-1.07630838599441,11.4840908039498,-48.3500372977493));
#30892=CARTESIAN_POINT('Ctrl Pts',(-1.62065368486988,11.4843329006937,-48.3401377766501));
#30893=CARTESIAN_POINT('Ctrl Pts',(-1.91997597602491,11.4849166217029,-48.3325976279206));
#30894=CARTESIAN_POINT('Ctrl Pts',(-2.88438286235813,11.4818828006798,-48.2936814855076));
#30895=CARTESIAN_POINT('Ctrl Pts',(-3.52649817574215,11.4863352799679,-48.25411650478));
#30896=CARTESIAN_POINT('Ctrl Pts',(-4.12864057911575,11.497472006951,-48.2071191491468));
#30897=CARTESIAN_POINT('Ctrl Pts',(-1.31980082626874,11.5143737377395,-48.3502977991201));
#30898=CARTESIAN_POINT('Ctrl Pts',(-1.44516286660466,11.5105174196343,-48.3485410607117));
#30899=CARTESIAN_POINT('Ctrl Pts',(-1.61934713769631,11.5090816899187,-48.3454511925548));
#30900=CARTESIAN_POINT('Ctrl Pts',(-2.04329098360778,11.5079260458441,-48.3350871090446));
#30901=CARTESIAN_POINT('Ctrl Pts',(-2.29305999893556,11.508146276444,-48.3277770168462));
#30902=CARTESIAN_POINT('Ctrl Pts',(-3.12263861219824,11.5065304546903,-48.29168097615));
#30903=CARTESIAN_POINT('Ctrl Pts',(-3.67166031045832,11.5121367174565,-48.2567445234558));
#30904=CARTESIAN_POINT('Ctrl Pts',(-4.1292012092717,11.5208685373805,-48.221588093388));
#30905=CARTESIAN_POINT('Ctrl Pts',(-1.67034425686001,11.5320543368685,-48.3484273824219));
#30906=CARTESIAN_POINT('Ctrl Pts',(-1.76830361911727,11.5270830007426,-48.3463749782915));
#30907=CARTESIAN_POINT('Ctrl Pts',(-1.917698093827,11.5245577996658,-48.342885156969));
#30908=CARTESIAN_POINT('Ctrl Pts',(-2.29199667103983,11.5217114161951,-48.3320814058286));
#30909=CARTESIAN_POINT('Ctrl Pts',(-2.51690958468367,11.521334369096,-48.3247339909552));
#30910=CARTESIAN_POINT('Ctrl Pts',(-3.26388339677572,11.5193254972085,-48.290293701452));
#30911=CARTESIAN_POINT('Ctrl Pts',(-3.75464503061926,11.5247638266718,-48.258028120514));
#30912=CARTESIAN_POINT('Ctrl Pts',(-4.12962875818775,11.5319897067687,-48.2293718250375));
#30913=CARTESIAN_POINT('Ctrl Pts',(-2.72152478002693,11.598649286609,-48.3459483822803));
#30914=CARTESIAN_POINT('Ctrl Pts',(-2.7817504873063,11.5919036248662,-48.3427355509081));
#30915=CARTESIAN_POINT('Ctrl Pts',(-2.87872640930532,11.5859418512212,-48.3377026419578));
#30916=CARTESIAN_POINT('Ctrl Pts',(-3.11802711878623,11.5755468354635,-48.3246778344466));
#30917=CARTESIAN_POINT('Ctrl Pts',(-3.2603569412057,11.5710816706623,-48.3166668015682));
#30918=CARTESIAN_POINT('Ctrl Pts',(-3.71314894654688,11.5598336028535,-48.2862238405639));
#30919=CARTESIAN_POINT('Ctrl Pts',(-3.99041609265724,11.5581209387927,-48.2614073735946));
#30920=CARTESIAN_POINT('Ctrl Pts',(-4.13155362590472,11.5609276470972,-48.2508605601154));
#30921=CARTESIAN_POINT('Ctrl Pts',(-3.42379713721014,11.6392592214975,-48.3412545192881));
#30922=CARTESIAN_POINT('Ctrl Pts',(-3.45976826235763,11.6298708101994,-48.3372561068189));
#30923=CARTESIAN_POINT('Ctrl Pts',(-3.52173695764161,11.6209827896646,-48.3313642361189));
#30924=CARTESIAN_POINT('Ctrl Pts',(-3.66733281854159,11.6050189470302,-48.3171415021054));
#30925=CARTESIAN_POINT('Ctrl Pts',(-3.75095998415758,11.5979431249306,-48.3088106387919));
#30926=CARTESIAN_POINT('Ctrl Pts',(-3.98882418159218,11.5806510816468,-48.2821814457032));
#30927=CARTESIAN_POINT('Ctrl Pts',(-4.13001933608944,11.5743267261738,-48.2630314915227));
#30928=CARTESIAN_POINT('Ctrl Pts',(-4.13369316567444,11.5743188502015,-48.2627031036729));
#30929=CARTESIAN_POINT('Ctrl Pts',(-4.12551258855296,11.6756605207451,-48.3310538583792));
#30930=CARTESIAN_POINT('Ctrl Pts',(-4.12617093842782,11.6636703105801,-48.3260557751567));
#30931=CARTESIAN_POINT('Ctrl Pts',(-4.12683967786648,11.6514649415886,-48.319925579004));
#30932=CARTESIAN_POINT('Ctrl Pts',(-4.12827545214397,11.6282480883359,-48.3065253445687));
#30933=CARTESIAN_POINT('Ctrl Pts',(-4.12904248698282,11.6172366040747,-48.299255306286));
#30934=CARTESIAN_POINT('Ctrl Pts',(-4.13160730900852,11.588429281961,-48.2774220038378));
#30935=CARTESIAN_POINT('Ctrl Pts',(-4.13366096331954,11.5746245276893,-48.2630127553113));
#30936=CARTESIAN_POINT('Ctrl Pts',(-4.13722371861475,11.5746245485739,-48.2627017315157));
#30937=CARTESIAN_POINT('Ctrl Pts',(-4.12551258855296,11.6756605207451,-48.3310538583792));
#30938=CARTESIAN_POINT('Ctrl Pts',(-4.12682928830268,11.6516801004151,-48.3210576919341));
#30939=CARTESIAN_POINT('Ctrl Pts',(-4.12818754630759,11.6268390447792,-48.3065330737686));
#30940=CARTESIAN_POINT('Ctrl Pts',(-4.13160730900852,11.588429281961,-48.2774220038378));
#30941=CARTESIAN_POINT('Ctrl Pts',(-4.13366096331954,11.5746245276893,-48.2630127553113));
#30942=CARTESIAN_POINT('Ctrl Pts',(-4.13722371861476,11.5746245485739,-48.2627017315157));
#30943=CARTESIAN_POINT('',(-4.12845481065586,11.4732422824942,-48.1954680629781));
#30944=CARTESIAN_POINT('Ctrl Pts',(-4.12845481065586,11.4732422824942,-48.1954680629781));
#30945=CARTESIAN_POINT('Ctrl Pts',(-4.12847724604266,11.4783327155669,-48.197582642083));
#30946=CARTESIAN_POINT('Ctrl Pts',(-4.12851349517641,11.4833192294908,-48.1999372550416));
#30947=CARTESIAN_POINT('Ctrl Pts',(-4.12856659581727,11.4882155782114,-48.2024493601598));
#30948=CARTESIAN_POINT('Ctrl Pts',(-4.1286324082246,11.4942840642271,-48.2055628383147));
#30949=CARTESIAN_POINT('Ctrl Pts',(-4.12872385562462,11.5002159367925,-48.2089197658545));
#30950=CARTESIAN_POINT('Ctrl Pts',(-4.12884968400471,11.5060421990484,-48.2124409973493));
#30951=CARTESIAN_POINT('Ctrl Pts',(-4.12887227574559,11.5070882699516,-48.2130732136224));
#30952=CARTESIAN_POINT('Ctrl Pts',(-4.12889598894898,11.5081309125981,-48.213710857774));
#30953=CARTESIAN_POINT('Ctrl Pts',(-4.12892089419373,11.5091702721658,-48.2143536212674));
#30954=CARTESIAN_POINT('Ctrl Pts',(-4.12907740654552,11.515701932945,-48.2183929482053));
#30955=CARTESIAN_POINT('Ctrl Pts',(-4.12927928751034,11.5221052499854,-48.2226316728729));
#30956=CARTESIAN_POINT('Ctrl Pts',(-4.12955440608205,11.5284062582695,-48.2270159410459));
#30957=CARTESIAN_POINT('Ctrl Pts',(-4.12974914542339,11.5328663504957,-48.2301192920516));
#30958=CARTESIAN_POINT('Ctrl Pts',(-4.1299802484247,11.5372739158669,-48.2332957729108));
#30959=CARTESIAN_POINT('Ctrl Pts',(-4.13027038076007,11.5416356868782,-48.2365347367302));
#30960=CARTESIAN_POINT('Ctrl Pts',(-4.13051330836706,11.545287794778,-48.2392467189322));
#30961=CARTESIAN_POINT('Ctrl Pts',(-4.13079649629707,11.5489068236642,-48.2420019879108));
#30962=CARTESIAN_POINT('Ctrl Pts',(-4.13115207407033,11.5524928731301,-48.2447943975055));
#30963=CARTESIAN_POINT('Ctrl Pts',(-4.13140677308046,11.5550615467591,-48.2467945899054));
#30964=CARTESIAN_POINT('Ctrl Pts',(-4.13169781691591,11.5576142914133,-48.2488147085002));
#30965=CARTESIAN_POINT('Ctrl Pts',(-4.13205749655601,11.5601495956737,-48.2508517250196));
#30966=CARTESIAN_POINT('Ctrl Pts',(-4.13230907506287,11.5619229183452,-48.2522765195236));
#30967=CARTESIAN_POINT('Ctrl Pts',(-4.13259322084644,11.5636878343141,-48.253709749953));
#30968=CARTESIAN_POINT('Ctrl Pts',(-4.13294254831288,11.5654435821136,-48.2551496626094));
#30969=CARTESIAN_POINT('Ctrl Pts',(-4.13317705493165,11.5666222311447,-48.2561162887147));
#30970=CARTESIAN_POINT('Ctrl Pts',(-4.13343997566705,11.5677969692623,-48.2570861853592));
#30971=CARTESIAN_POINT('Ctrl Pts',(-4.13376223323209,11.5689658159629,-48.2580563995925));
#30972=CARTESIAN_POINT('Ctrl Pts',(-4.13395686573063,11.5696717592159,-48.2586423756589));
#30973=CARTESIAN_POINT('Ctrl Pts',(-4.13417293995391,11.5703762086922,-48.2592290531955));
#30974=CARTESIAN_POINT('Ctrl Pts',(-4.13443138997987,11.5710757337678,-48.259812391898));
#30975=CARTESIAN_POINT('Ctrl Pts',(-4.13461059905206,11.5715607839794,-48.2602168785575));
#30976=CARTESIAN_POINT('Ctrl Pts',(-4.13481062697808,11.5720464962208,-48.2606223555231));
#30977=CARTESIAN_POINT('Ctrl Pts',(-4.13505139716509,11.5725238643872,-48.2610197986288));
#30978=CARTESIAN_POINT('Ctrl Pts',(-4.13521808348396,11.5728543485863,-48.261294950337));
#30979=CARTESIAN_POINT('Ctrl Pts',(-4.13540552833946,11.5731846562113,-48.2615695100043));
#30980=CARTESIAN_POINT('Ctrl Pts',(-4.1356319850481,11.5734998993923,-48.2618291616974));
#30981=CARTESIAN_POINT('Ctrl Pts',(-4.13573263391391,11.5736400094769,-48.2619445641006));
#30982=CARTESIAN_POINT('Ctrl Pts',(-4.13584148560198,11.5737774981193,-48.2620572934349));
#30983=CARTESIAN_POINT('Ctrl Pts',(-4.13596273598079,11.5739092744925,-48.2621643000755));
#30984=CARTESIAN_POINT('Ctrl Pts',(-4.13604421784951,11.5739978299696,-48.2622362099625));
#30985=CARTESIAN_POINT('Ctrl Pts',(-4.13612859548604,11.5740821529239,-48.2623042726689));
#30986=CARTESIAN_POINT('Ctrl Pts',(-4.13623430704625,11.5741721054098,-48.2623758167973));
#30987=CARTESIAN_POINT('Ctrl Pts',(-4.13628716282636,11.5742170816527,-48.2624115888615));
#30988=CARTESIAN_POINT('Ctrl Pts',(-4.13634156211114,11.5742618826266,-48.2624471111769));
#30989=CARTESIAN_POINT('Ctrl Pts',(-4.13643190399437,11.5743239422309,-48.262495252223));
#30990=CARTESIAN_POINT('Ctrl Pts',(-4.13647707491214,11.5743549720167,-48.2625193227333));
#30991=CARTESIAN_POINT('Ctrl Pts',(-4.13654109921554,11.5743996848316,-48.2625541029385));
#30992=CARTESIAN_POINT('Ctrl Pts',(-4.13665995702445,11.5744597225478,-48.2625983712319));
#30993=CARTESIAN_POINT('Ctrl Pts',(-4.13674744934593,11.5745039168605,-48.262630957528));
#30994=CARTESIAN_POINT('Ctrl Pts',(-4.13686460908674,11.5745568559735,-48.2626691138439));
#30995=CARTESIAN_POINT('Ctrl Pts',(-4.13702846629035,11.5745940265261,-48.2626896148542));
#30996=CARTESIAN_POINT('Ctrl Pts',(-4.13708720814305,11.5746073519526,-48.2626969643469));
#30997=CARTESIAN_POINT('Ctrl Pts',(-4.13715198465268,11.5746183373345,-48.2627017593562));
#30998=CARTESIAN_POINT('Ctrl Pts',(-4.13722371775385,11.5746245484993,-48.2627017315161));
#30999=CARTESIAN_POINT('Ctrl Pts',(-4.12845481065586,11.4732422824942,-48.1954680629781));
#31000=CARTESIAN_POINT('Ctrl Pts',(-3.42734501838564,11.4609474762041,-48.2515240163504));
#31001=CARTESIAN_POINT('Ctrl Pts',(-2.7260922459071,11.45833845903,-48.2947245924949));
#31002=CARTESIAN_POINT('Ctrl Pts',(-1.32086240342357,11.4664956854044,-48.3492527705134));
#31003=CARTESIAN_POINT('Ctrl Pts',(-0.618564042217151,11.4621780884823,
-48.3550822503405));
#31004=CARTESIAN_POINT('Ctrl Pts',(0.0835265683594526,11.4728541727075,
-48.3550824830876));
#31005=CARTESIAN_POINT('Ctrl Pts',(0.0835265683594526,11.4728541727075,
-48.3550824830876));
#31006=CARTESIAN_POINT('Ctrl Pts',(0.0835265683595233,11.4515020042572,
-48.3550820175938));
#31007=CARTESIAN_POINT('Ctrl Pts',(0.0835265683609461,11.4284235901226,
-48.3547237088909));
#31008=CARTESIAN_POINT('Ctrl Pts',(0.083526568361231,11.3941472536996,-48.350619056743));
#31009=CARTESIAN_POINT('Ctrl Pts',(0.0835265683612866,11.3720285904897,
-48.3550682080606));
#31010=CARTESIAN_POINT('Ctrl Pts',(0.0835265683620956,11.3536536794531,
-48.3550682080606));
#31011=CARTESIAN_POINT('Ctrl Pts',(-0.267518736928849,11.4675161305949,
-48.355082366714));
#31012=CARTESIAN_POINT('Ctrl Pts',(-0.189662916098598,11.4488974993902,
-48.3550223265509));
#31013=CARTESIAN_POINT('Ctrl Pts',(-0.172476876269728,11.4285976962987,
-48.3547580080055));
#31014=CARTESIAN_POINT('Ctrl Pts',(-0.19427927370922,11.3940705712691,-48.3505964242949));
#31015=CARTESIAN_POINT('Ctrl Pts',(-0.233267710976564,11.3720285904897,
-48.3550682080606));
#31016=CARTESIAN_POINT('Ctrl Pts',(-0.26776084433578,11.3536536794531,-48.3550682080606));
#31017=CARTESIAN_POINT('Ctrl Pts',(-0.618615979874604,11.4659265087691,
-48.3536249385705));
#31018=CARTESIAN_POINT('Ctrl Pts',(-0.485248141787488,11.447718516688,-48.3538283041916));
#31019=CARTESIAN_POINT('Ctrl Pts',(-0.459481328458187,11.428587933622,-48.3533940028244));
#31020=CARTESIAN_POINT('Ctrl Pts',(-0.500506504781256,11.3934281614349,
-48.3484833203952));
#31021=CARTESIAN_POINT('Ctrl Pts',(-0.567298494432773,11.3718199008203,
-48.3519505469255));
#31022=CARTESIAN_POINT('Ctrl Pts',(-0.619048262304807,11.3536536794531,
-48.3512468523357));
#31023=CARTESIAN_POINT('Ctrl Pts',(-1.32094154343241,11.464396632877,-48.3438941182179));
#31024=CARTESIAN_POINT('Ctrl Pts',(-1.12790203394888,11.4452664260876,-48.3454622940091));
#31025=CARTESIAN_POINT('Ctrl Pts',(-1.09571051627679,11.4271829834973,-48.3443038073303));
#31026=CARTESIAN_POINT('Ctrl Pts',(-1.16018842034295,11.3913038531299,-48.3372314655874));
#31027=CARTESIAN_POINT('Ctrl Pts',(-1.25685784208063,11.3711415135622,-48.3377896456608));
#31028=CARTESIAN_POINT('Ctrl Pts',(-1.32154021141497,11.3536536794531,-48.3359596079612));
#31029=CARTESIAN_POINT('Ctrl Pts',(-1.67216986404445,11.4644563788108,-48.3356207260088));
#31030=CARTESIAN_POINT('Ctrl Pts',(-1.47497921486972,11.443938017789,-48.3381640344641));
#31031=CARTESIAN_POINT('Ctrl Pts',(-1.44494173036685,11.4257324956489,-48.3364512936465));
#31032=CARTESIAN_POINT('Ctrl Pts',(-1.51364329271565,11.389794304459,-48.3280294754275));
#31033=CARTESIAN_POINT('Ctrl Pts',(-1.61238233956687,11.3706718159735,-48.3267463020471));
#31034=CARTESIAN_POINT('Ctrl Pts',(-1.67274475309907,11.3536536794531,-48.3244937189391));
#31035=CARTESIAN_POINT('Ctrl Pts',(-2.37478478528622,11.4603777656235,-48.3083566369995));
#31036=CARTESIAN_POINT('Ctrl Pts',(-2.22731576370123,11.4381382649982,-48.3098281543322));
#31037=CARTESIAN_POINT('Ctrl Pts',(-2.20580868481744,11.4203247666437,-48.307328281957));
#31038=CARTESIAN_POINT('Ctrl Pts',(-2.25808685967459,11.3861758639155,-48.2988519282882));
#31039=CARTESIAN_POINT('Ctrl Pts',(-2.3318721134153,11.3696277842964,-48.2961657002409));
#31040=CARTESIAN_POINT('Ctrl Pts',(-2.37498775707866,11.3536536794531,-48.2939119483841));
#31041=CARTESIAN_POINT('Ctrl Pts',(-2.7257517087163,11.4600103666203,-48.2907404707111));
#31042=CARTESIAN_POINT('Ctrl Pts',(-2.60287727457564,11.4370088609558,-48.2910861014142));
#31043=CARTESIAN_POINT('Ctrl Pts',(-2.58784945387008,11.4187667259072,-48.2880098223025));
#31044=CARTESIAN_POINT('Ctrl Pts',(-2.63432748053576,11.3847952022384,-48.2796807289492));
#31045=CARTESIAN_POINT('Ctrl Pts',(-2.69583332790684,11.369053450208,-48.2766286482955));
#31046=CARTESIAN_POINT('Ctrl Pts',(-2.72602622991903,11.3536536794531,-48.2747960661052));
#31047=CARTESIAN_POINT('Ctrl Pts',(-3.42730927333356,11.4633689234831,-48.2483101720435));
#31048=CARTESIAN_POINT('Ctrl Pts',(-3.35965513497476,11.4394032486783,-48.2448130738858));
#31049=CARTESIAN_POINT('Ctrl Pts',(-3.35545842749711,11.4193327724023,-48.2403172932759));
#31050=CARTESIAN_POINT('Ctrl Pts',(-3.38522478863114,11.3835624194323,-48.232439703259));
#31051=CARTESIAN_POINT('Ctrl Pts',(-3.4191878572428,11.3679565169509,-48.2296135008165));
#31052=CARTESIAN_POINT('Ctrl Pts',(-3.42785327106255,11.3536536794531,-48.2289052281065));
#31053=CARTESIAN_POINT('Ctrl Pts',(-3.77789991452075,11.4670948793492,-48.2234960396643));
#31054=CARTESIAN_POINT('Ctrl Pts',(-3.74087148449948,11.4429270404433,-48.2172820992753));
#31055=CARTESIAN_POINT('Ctrl Pts',(-3.74102460769126,11.4214568596339,-48.2119434824081));
#31056=CARTESIAN_POINT('Ctrl Pts',(-3.7598774297419,11.3837102983034,-48.2043703936356));
#31057=CARTESIAN_POINT('Ctrl Pts',(-3.77857712860076,11.3674339177823,-48.2021359217303));
#31058=CARTESIAN_POINT('Ctrl Pts',(-3.77864184991365,11.3536536794531,-48.2021302712649));
#31059=CARTESIAN_POINT('Ctrl Pts',(-4.12845481065586,11.4732422824942,-48.1954680629781));
#31060=CARTESIAN_POINT('Ctrl Pts',(-4.12834943621585,11.4493335556629,-48.1855363158243));
#31061=CARTESIAN_POINT('Ctrl Pts',(-4.12855150591032,11.4261172510677,-48.1795491602216));
#31062=CARTESIAN_POINT('Ctrl Pts',(-4.12900833251927,11.384958159128,-48.1725407225933));
#31063=CARTESIAN_POINT('Ctrl Pts',(-4.12926308943375,11.3670153717833,-48.1715194405676));
#31064=CARTESIAN_POINT('Ctrl Pts',(-4.12926308943375,11.3536536794531,-48.1715194405676));
#31065=CARTESIAN_POINT('Origin',(-4.155077712629,11.3534224546477,-48.4841190147253));
#31066=CARTESIAN_POINT('Ctrl Pts',(0.0835265683620358,11.3536536794531,
-48.3550682080606));
#31067=CARTESIAN_POINT('Ctrl Pts',(0.0835265683612866,11.3720285904897,
-48.3550682080606));
#31068=CARTESIAN_POINT('Ctrl Pts',(0.083526568361231,11.3941472536996,-48.350619056743));
#31069=CARTESIAN_POINT('Ctrl Pts',(0.0835265683609461,11.4284235901226,
-48.3547237088909));
#31070=CARTESIAN_POINT('Ctrl Pts',(0.0835265683595233,11.4515020042572,
-48.3550820175938));
#31071=CARTESIAN_POINT('Ctrl Pts',(0.0835265683594526,11.4728541727075,
-48.3550824830876));
#31072=CARTESIAN_POINT('Ctrl Pts',(0.0835265683594526,11.4728541727075,
-48.3550824830876));
#31073=CARTESIAN_POINT('Ctrl Pts',(0.43457187364779,11.467516130595,-48.3550823667143));
#31074=CARTESIAN_POINT('Ctrl Pts',(0.785669116593031,11.4659265087692,-48.353624938571));
#31075=CARTESIAN_POINT('Ctrl Pts',(1.48799468014872,11.4643966328772,-48.3438941182188));
#31076=CARTESIAN_POINT('Ctrl Pts',(1.83922300075916,11.4644563788109,-48.3356207260099));
#31077=CARTESIAN_POINT('Ctrl Pts',(2.54183792199666,11.4603777656235,-48.3083566370006));
#31078=CARTESIAN_POINT('Ctrl Pts',(2.89280484542876,11.4600103666202,-48.2907404707119));
#31079=CARTESIAN_POINT('Ctrl Pts',(3.59436241005202,11.463368923483,-48.2483101720439));
#31080=CARTESIAN_POINT('Ctrl Pts',(3.94495305124318,11.4670948793491,-48.2234960396644));
#31081=CARTESIAN_POINT('Ctrl Pts',(4.29550794738005,11.4732422824942,-48.1954680629781));
#31082=CARTESIAN_POINT('Ctrl Pts',(0.0835265683595233,11.4515020042572,
-48.3550820175938));
#31083=CARTESIAN_POINT('Ctrl Pts',(0.356716052817998,11.4488974993903,-48.3550223265511));
#31084=CARTESIAN_POINT('Ctrl Pts',(0.652301278506739,11.4477185166882,-48.353828304192));
#31085=CARTESIAN_POINT('Ctrl Pts',(1.2949551706665,11.4452664260879,-48.34546229401));
#31086=CARTESIAN_POINT('Ctrl Pts',(1.64203235158588,11.4439380177893,-48.3381640344652));
#31087=CARTESIAN_POINT('Ctrl Pts',(2.39436890041279,11.4381382649983,-48.3098281543332));
#31088=CARTESIAN_POINT('Ctrl Pts',(2.76993041128897,11.4370088609558,-48.2910861014151));
#31089=CARTESIAN_POINT('Ctrl Pts',(3.52670827169359,11.4394032486783,-48.2448130738862));
#31090=CARTESIAN_POINT('Ctrl Pts',(3.90792462122203,11.4429270404433,-48.2172820992754));
#31091=CARTESIAN_POINT('Ctrl Pts',(4.29540257294004,11.4493335556629,-48.1855363158243));
#31092=CARTESIAN_POINT('Ctrl Pts',(0.0835265683609461,11.4284235901226,
-48.3547237088909));
#31093=CARTESIAN_POINT('Ctrl Pts',(0.33953001299162,11.4285976962988,-48.3547580080057));
#31094=CARTESIAN_POINT('Ctrl Pts',(0.626534465179757,11.4285879336221,-48.3533940028248));
#31095=CARTESIAN_POINT('Ctrl Pts',(1.26276365299677,11.4271829834975,-48.344303807331));
#31096=CARTESIAN_POINT('Ctrl Pts',(1.61199486708556,11.4257324956492,-48.3364512936473));
#31097=CARTESIAN_POINT('Ctrl Pts',(2.37286182153235,11.4203247666439,-48.3073282819579));
#31098=CARTESIAN_POINT('Ctrl Pts',(2.75490259058618,11.4187667259073,-48.2880098223032));
#31099=CARTESIAN_POINT('Ctrl Pts',(3.52251156421718,11.4193327724023,-48.2403172932763));
#31100=CARTESIAN_POINT('Ctrl Pts',(3.90807774441412,11.4214568596339,-48.2119434824082));
#31101=CARTESIAN_POINT('Ctrl Pts',(4.29560464263451,11.4261172510678,-48.1795491602216));
#31102=CARTESIAN_POINT('Ctrl Pts',(0.083526568361231,11.3941472536996,-48.350619056743));
#31103=CARTESIAN_POINT('Ctrl Pts',(0.361332410431682,11.3940705712691,-48.350596424295));
#31104=CARTESIAN_POINT('Ctrl Pts',(0.667559641503652,11.393428161435,-48.3484833203954));
#31105=CARTESIAN_POINT('Ctrl Pts',(1.32724155706492,11.39130385313,-48.3372314655877));
#31106=CARTESIAN_POINT('Ctrl Pts',(1.68069642943727,11.3897943044591,-48.3280294754278));
#31107=CARTESIAN_POINT('Ctrl Pts',(2.42513999639505,11.3861758639155,-48.2988519282886));
#31108=CARTESIAN_POINT('Ctrl Pts',(2.8013806172567,11.3847952022384,-48.2796807289495));
#31109=CARTESIAN_POINT('Ctrl Pts',(3.55227792535362,11.3835624194324,-48.2324397032591));
#31110=CARTESIAN_POINT('Ctrl Pts',(3.92693056646546,11.3837102983034,-48.2043703936356));
#31111=CARTESIAN_POINT('Ctrl Pts',(4.29606146924347,11.384958159128,-48.1725407225933));
#31112=CARTESIAN_POINT('Ctrl Pts',(0.0835265683612866,11.3720285904897,
-48.3550682080606));
#31113=CARTESIAN_POINT('Ctrl Pts',(0.400320847699137,11.3720285904897,-48.3550682080606));
#31114=CARTESIAN_POINT('Ctrl Pts',(0.734351631155381,11.3718199008203,-48.3519505469256));
#31115=CARTESIAN_POINT('Ctrl Pts',(1.42391097880337,11.3711415135622,-48.3377896456608));
#31116=CARTESIAN_POINT('Ctrl Pts',(1.77943547628973,11.3706718159735,-48.3267463020472));
#31117=CARTESIAN_POINT('Ctrl Pts',(2.49892525013843,11.3696277842964,-48.296165700241));
#31118=CARTESIAN_POINT('Ctrl Pts',(2.86288646463014,11.369053450208,-48.2766286482956));
#31119=CARTESIAN_POINT('Ctrl Pts',(3.58624099396651,11.3679565169509,-48.2296135008166));
#31120=CARTESIAN_POINT('Ctrl Pts',(3.9456302653247,11.3674339177823,-48.2021359217302));
#31121=CARTESIAN_POINT('Ctrl Pts',(4.29631622615795,11.3670153717833,-48.1715194405676));
#31122=CARTESIAN_POINT('Ctrl Pts',(0.0835265683620956,11.3536536794531,
-48.3550682080606));
#31123=CARTESIAN_POINT('Ctrl Pts',(0.434813981059971,11.3536536794531,-48.3550682080606));
#31124=CARTESIAN_POINT('Ctrl Pts',(0.786101399028999,11.3536536794531,-48.3512468523357));
#31125=CARTESIAN_POINT('Ctrl Pts',(1.48859334813917,11.3536536794531,-48.3359596079612));
#31126=CARTESIAN_POINT('Ctrl Pts',(1.83979788982327,11.3536536794531,-48.3244937189391));
#31127=CARTESIAN_POINT('Ctrl Pts',(2.54204089380286,11.3536536794531,-48.293911948384));
#31128=CARTESIAN_POINT('Ctrl Pts',(2.89307936664324,11.3536536794531,-48.2747960661052));
#31129=CARTESIAN_POINT('Ctrl Pts',(3.59490640778675,11.3536536794531,-48.2289052281065));
#31130=CARTESIAN_POINT('Ctrl Pts',(3.94569498663785,11.353653679453,-48.2021302712649));
#31131=CARTESIAN_POINT('Ctrl Pts',(4.29631622615795,11.353653679453,-48.1715194405676));
#31132=CARTESIAN_POINT('',(4.29550794738005,11.4732422824942,-48.1954680629781));
#31133=CARTESIAN_POINT('Origin',(4.32213084935235,11.3534224546478,-48.484119014725));
#31134=CARTESIAN_POINT('Ctrl Pts',(4.29550794738005,11.4732422824942,-48.1954680629781));
#31135=CARTESIAN_POINT('Ctrl Pts',(3.59439815510631,11.4609474762041,-48.2515240163507));
#31136=CARTESIAN_POINT('Ctrl Pts',(2.89314538261541,11.4583384590298,-48.2947245924959));
#31137=CARTESIAN_POINT('Ctrl Pts',(1.48791554014041,11.4664956854045,-48.3492527705145));
#31138=CARTESIAN_POINT('Ctrl Pts',(0.785617178936127,11.4621780884824,-48.355082250341));
#31139=CARTESIAN_POINT('Ctrl Pts',(0.0835265683594526,11.4728541727075,
-48.3550824830876));
#31140=CARTESIAN_POINT('Origin',(-44.291473431638,16.1705954176946,-48.6675682080606));
#31141=CARTESIAN_POINT('Origin',(21.5192211643356,16.1705954176946,-48.6675682080606));
#31142=CARTESIAN_POINT('Origin',(-21.3521680276115,16.1705954176946,-48.6675682080606));
#31143=CARTESIAN_POINT('Ctrl Pts',(21.5192211643355,16.1705954176947,-48.3550682080606));
#31144=CARTESIAN_POINT('Ctrl Pts',(21.5192211643355,16.4830954176946,-48.3550682080606));
#31145=CARTESIAN_POINT('Ctrl Pts',(21.5192211643356,16.4830954176946,-48.6675682080606));
#31146=CARTESIAN_POINT('Ctrl Pts',(21.7183268789094,16.2080049077902,-48.3550682080606));
#31147=CARTESIAN_POINT('Ctrl Pts',(21.7071386526689,16.4830954176967,-48.3903755582775));
#31148=CARTESIAN_POINT('Ctrl Pts',(21.7335478130473,16.4830954176946,-48.6675682080621));
#31149=CARTESIAN_POINT('Ctrl Pts',(21.9153131059641,16.2453260884688,-48.3475889909109));
#31150=CARTESIAN_POINT('Ctrl Pts',(21.911211102576,16.4830954176946,-48.4095570299751));
#31151=CARTESIAN_POINT('Ctrl Pts',(21.9460469728313,16.4830954176946,-48.6526097807597));
#31152=CARTESIAN_POINT('Ctrl Pts',(22.3039820967341,16.3195276817373,-48.3137123018963));
#31153=CARTESIAN_POINT('Ctrl Pts',(22.314923637338,16.4830954176946,-48.4038409245796));
#31154=CARTESIAN_POINT('Ctrl Pts',(22.3661671540024,16.4830954176946,-48.5848563887335));
#31155=CARTESIAN_POINT('Ctrl Pts',(22.4984290660376,16.3569498947425,-48.2880700344635));
#31156=CARTESIAN_POINT('Ctrl Pts',(22.5211470257103,16.4830954176957,-48.3840049109222));
#31157=CARTESIAN_POINT('Ctrl Pts',(22.5772011717386,16.4830954176946,-48.5333831751917));
#31158=CARTESIAN_POINT('Ctrl Pts',(22.6771142305796,16.3915662868148,-48.2427418189135));
#31159=CARTESIAN_POINT('Ctrl Pts',(22.7158795095401,16.4830954176946,-48.3256564433572));
#31160=CARTESIAN_POINT('Ctrl Pts',(22.7707018927952,16.4830954176946,-48.4429154297649));
#31161=CARTESIAN_POINT('Ctrl Pts',(22.6771142305791,16.3915662868147,-48.2427418189136));
#31162=CARTESIAN_POINT('Ctrl Pts',(22.6378911635743,16.3839676712799,-48.2526917941307));
#31163=CARTESIAN_POINT('Ctrl Pts',(22.5984148180719,16.3763319926651,-48.2615688372914));
#31164=CARTESIAN_POINT('Ctrl Pts',(22.558782775705,16.3686778876808,-48.2695704658023));
#31165=CARTESIAN_POINT('Ctrl Pts',(22.5150421675873,16.3602302986439,-48.2784016053575));
#31166=CARTESIAN_POINT('Ctrl Pts',(22.4711116392402,16.3517602066248,-48.286166399441));
#31167=CARTESIAN_POINT('Ctrl Pts',(22.4270762160408,16.3432839722952,-48.2930847735754));
#31168=CARTESIAN_POINT('Ctrl Pts',(22.3795404288295,16.3341339643659,-48.3005530874194));
#31169=CARTESIAN_POINT('Ctrl Pts',(22.3318815956323,16.3249766329787,-48.3070346785341));
#31170=CARTESIAN_POINT('Ctrl Pts',(22.2841643538499,16.3158247537669,-48.312759037465));
#31171=CARTESIAN_POINT('Ctrl Pts',(22.2260558231734,16.3046798880107,-48.3197299786618));
#31172=CARTESIAN_POINT('Ctrl Pts',(22.1678592205032,16.2935427876854,-48.325577982882));
#31173=CARTESIAN_POINT('Ctrl Pts',(22.1096477331681,16.2824290454295,-48.330651463777));
#31174=CARTESIAN_POINT('Ctrl Pts',(22.1068105242813,16.2818873652606,-48.3308987435793));
#31175=CARTESIAN_POINT('Ctrl Pts',(22.1039726872235,16.2813456246246,-48.3311440122853));
#31176=CARTESIAN_POINT('Ctrl Pts',(22.1011341818606,16.2808038159101,-48.3313872793092));
#31177=CARTESIAN_POINT('Ctrl Pts',(21.9836165992224,16.2583722745758,-48.3414588306834));
#31178=CARTESIAN_POINT('Ctrl Pts',(21.8658458886457,16.2359974207799,-48.3480286392735));
#31179=CARTESIAN_POINT('Ctrl Pts',(21.7478614729999,16.2136898071046,-48.3516402651633));
#31180=CARTESIAN_POINT('Ctrl Pts',(21.6717488808251,16.199299005635,-48.3539701509108));
#31181=CARTESIAN_POINT('Ctrl Pts',(21.5955470434192,16.1849361189663,-48.3550678012165));
#31182=CARTESIAN_POINT('Ctrl Pts',(21.5192635553992,16.1706033824536,-48.3550682079476));
#31183=CARTESIAN_POINT('Origin',(22.7707018927938,16.1705954176946,-48.4429154297618));
#31184=CARTESIAN_POINT('Ctrl Pts',(-21.2235932570288,16.4830953098781,-48.6660549524581));
#31185=CARTESIAN_POINT('Ctrl Pts',(-21.2332870627948,16.4833744495148,-48.3301033390522));
#31186=CARTESIAN_POINT('Ctrl Pts',(-21.2326795856286,16.1481826330634,-48.35418182094));
#31187=CARTESIAN_POINT('Ctrl Pts',(-21.4809214109692,16.483095324294,-48.6730692758819));
#31188=CARTESIAN_POINT('Ctrl Pts',(-21.4530298656609,16.483319828549,-48.3811888777417));
#31189=CARTESIAN_POINT('Ctrl Pts',(-21.4719110727632,16.1929802521112,-48.3576973104808));
#31190=CARTESIAN_POINT('Ctrl Pts',(-21.7374879541375,16.4830953387802,-48.6595262778593));
#31191=CARTESIAN_POINT('Ctrl Pts',(-21.7001920947721,16.483273583025,-48.4102189210674));
#31192=CARTESIAN_POINT('Ctrl Pts',(-21.7098307047766,16.2379895254129,-48.3509368618739));
#31193=CARTESIAN_POINT('Ctrl Pts',(-22.2406226301952,16.4830953673845,-48.5783465526032));
#31194=CARTESIAN_POINT('Ctrl Pts',(-22.1840696711221,16.4831976839894,-48.4033925316084));
#31195=CARTESIAN_POINT('Ctrl Pts',(-22.1752787584643,16.3268490737816,-48.3103713569693));
#31196=CARTESIAN_POINT('Ctrl Pts',(-22.4910901849638,16.4830953816853,-48.5139692904343));
#31197=CARTESIAN_POINT('Ctrl Pts',(-22.4296943202957,16.4831654080667,-48.377041868324));
#31198=CARTESIAN_POINT('Ctrl Pts',(-22.405734464261,16.3712675955696,-48.2783677938984));
#31199=CARTESIAN_POINT('Ctrl Pts',(-22.719770248326,16.4830953949244,-48.3828323956905));
#31200=CARTESIAN_POINT('Ctrl Pts',(-22.6621435906265,16.483138027882,-48.2869031393868));
#31201=CARTESIAN_POINT('Ctrl Pts',(-22.6173710027542,16.4123847430247,-48.2125473910278));
#31202=CARTESIAN_POINT('Origin',(-22.6036487560697,16.1705954176946,-48.4429154297618));
#31203=CARTESIAN_POINT('Ctrl Pts',(-21.3522103060312,16.1706033612892,-48.3550682079475));
#31204=CARTESIAN_POINT('Ctrl Pts',(-21.4500468132788,16.1889856471426,-48.3550676843655));
#31205=CARTESIAN_POINT('Ctrl Pts',(-21.547817703659,16.2074307865434,-48.3532530208503));
#31206=CARTESIAN_POINT('Ctrl Pts',(-21.6454352010438,16.2259200040857,-48.3493520545576));
#31207=CARTESIAN_POINT('Ctrl Pts',(-21.7419037370204,16.2441916028814,-48.3454970027766));
#31208=CARTESIAN_POINT('Ctrl Pts',(-21.8382231430226,16.2625063923369,-48.3396050349912));
#31209=CARTESIAN_POINT('Ctrl Pts',(-21.9342849222553,16.2808424439029,-48.3313696581645));
#31210=CARTESIAN_POINT('Ctrl Pts',(-21.937041977193,16.2813687042107,-48.3311332958306));
#31211=CARTESIAN_POINT('Ctrl Pts',(-21.9397986145587,16.2818949414479,-48.3308950166343));
#31212=CARTESIAN_POINT('Ctrl Pts',(-21.9425548449769,16.2824211576432,-48.3306548123709));
#31213=CARTESIAN_POINT('Ctrl Pts',(-22.0014746788088,16.2936700614286,-48.3255199748789));
#31214=CARTESIAN_POINT('Ctrl Pts',(-22.0603976620597,16.3049460203245,-48.3196239637247));
#31215=CARTESIAN_POINT('Ctrl Pts',(-22.1192165044416,16.3162274856631,-48.3125646537137));
#31216=CARTESIAN_POINT('Ctrl Pts',(-22.1732048838581,16.3265824672713,-48.3060850854009));
#31217=CARTESIAN_POINT('Ctrl Pts',(-22.2271060462257,16.3369421989594,-48.2986260138347));
#31218=CARTESIAN_POINT('Ctrl Pts',(-22.2808168332591,16.3472864072055,-48.2898397095524));
#31219=CARTESIAN_POINT('Ctrl Pts',(-22.3299129238807,16.3567418669654,-48.2818083025465));
#31220=CARTESIAN_POINT('Ctrl Pts',(-22.3788501680607,16.3661844046855,-48.2726681344544));
#31221=CARTESIAN_POINT('Ctrl Pts',(-22.4275274387716,16.3755943695789,-48.2621166834727));
#31222=CARTESIAN_POINT('Ctrl Pts',(-22.4551301771965,16.3809303466323,-48.2561334198839));
#31223=CARTESIAN_POINT('Ctrl Pts',(-22.4826488894981,16.3862557688533,-48.2496956543661));
#31224=CARTESIAN_POINT('Ctrl Pts',(-22.5100610938539,16.3915662868154,-48.2427418189112));
#31225=CARTESIAN_POINT('Ctrl Pts',(-23.0849210718625,16.8990456385831,-48.3550682080606));
#31226=CARTESIAN_POINT('Ctrl Pts',(-23.1434946548348,16.7639536069274,-48.3550682080606));
#31227=CARTESIAN_POINT('Ctrl Pts',(-23.1808194403678,16.6779610607098,-48.241518966339));
#31228=CARTESIAN_POINT('Ctrl Pts',(-19.9713351701806,15.5488264548572,-48.3550682080606));
#31229=CARTESIAN_POINT('Ctrl Pts',(-20.0384527840987,15.4217541149126,-48.3550682080606));
#31230=CARTESIAN_POINT('Ctrl Pts',(-20.0567638409257,15.3277344947597,-48.2465561452514));
#31231=CARTESIAN_POINT('Ctrl Pts',(-16.7812848361363,14.382877194386,-48.3550682080606));
#31232=CARTESIAN_POINT('Ctrl Pts',(-16.8373508296582,14.2535943294201,-48.3550682080606));
#31233=CARTESIAN_POINT('Ctrl Pts',(-16.8547673953945,14.1617844335495,-48.2513064297563));
#31234=CARTESIAN_POINT('Ctrl Pts',(-11.9276124411326,13.0662924545649,-48.3550682080606));
#31235=CARTESIAN_POINT('Ctrl Pts',(-11.962050470773,12.935869085436,-48.3550682080606));
#31236=CARTESIAN_POINT('Ctrl Pts',(-11.9812252105756,12.8452005633123,-48.2569136015784));
#31237=CARTESIAN_POINT('Ctrl Pts',(-10.3466638904053,12.7052707111053,-48.3550682080606));
#31238=CARTESIAN_POINT('Ctrl Pts',(-10.3762902134349,12.5748662546358,-48.3550682080606));
#31239=CARTESIAN_POINT('Ctrl Pts',(-10.3935551174996,12.4841786131398,-48.2584966737937));
#31240=CARTESIAN_POINT('Ctrl Pts',(-6.98178065400343,12.0967706273038,-48.3550682080606));
#31241=CARTESIAN_POINT('Ctrl Pts',(-7.00312169292105,11.9671239022574,-48.3550682080606));
#31242=CARTESIAN_POINT('Ctrl Pts',(-7.01396478862274,11.8756772034364,-48.2612025886206));
#31243=CARTESIAN_POINT('Ctrl Pts',(-5.19039787585605,11.86730628845,-48.3550682080606));
#31244=CARTESIAN_POINT('Ctrl Pts',(-5.20558538253443,11.7375302402796,-48.3550682080606));
#31245=CARTESIAN_POINT('Ctrl Pts',(-5.21452165327191,11.6462129991553,-48.2622498619779));
#31246=CARTESIAN_POINT('Ctrl Pts',(-3.39047527149618,11.7377723175973,-48.3550682080606));
#31247=CARTESIAN_POINT('Ctrl Pts',(-3.39980751503421,11.608092893254,-48.3550682080606));
#31248=CARTESIAN_POINT('Ctrl Pts',(-3.40639346140351,11.5166787176219,-48.2628417377604));
#31249=CARTESIAN_POINT('Ctrl Pts',(22.9214777263312,16.4951170325608,-48.2422982426787));
#31250=CARTESIAN_POINT('Ctrl Pts',(22.8846548346438,16.581294328644,-48.3550682080606));
#31251=CARTESIAN_POINT('Ctrl Pts',(22.8270439774155,16.7161293233258,-48.3550682080606));
#31252=CARTESIAN_POINT('Ctrl Pts',(19.9326035269438,15.2224248692786,-48.2470767173395));
#31253=CARTESIAN_POINT('Ctrl Pts',(19.9130757495238,15.3157731473117,-48.3550682080606));
#31254=CARTESIAN_POINT('Ctrl Pts',(19.8482783897377,15.4434377872993,-48.3550682080606));
#31255=CARTESIAN_POINT('Ctrl Pts',(16.8711181780395,14.121138883407,-48.2515673091557));
#31256=CARTESIAN_POINT('Ctrl Pts',(16.8528533641736,14.2126904008502,-48.3550682080606));
#31257=CARTESIAN_POINT('Ctrl Pts',(16.7982643163788,14.3421540062504,-48.3550682080606));
#31258=CARTESIAN_POINT('Ctrl Pts',(12.1478906017067,12.8451845281753,-48.2569973005878));
#31259=CARTESIAN_POINT('Ctrl Pts',(12.1287157575068,12.9358419174557,-48.3550682080606));
#31260=CARTESIAN_POINT('Ctrl Pts',(12.0942956535457,13.066199446441,-48.3550682080606));
#31261=CARTESIAN_POINT('Ctrl Pts',(10.5602837555011,12.484193948824,-48.2585790241695));
#31262=CARTESIAN_POINT('Ctrl Pts',(10.5430188516445,12.5748700381595,-48.3550682080606));
#31263=CARTESIAN_POINT('Ctrl Pts',(10.5134085414344,12.7052089420493,-48.3550682080606));
#31264=CARTESIAN_POINT('Ctrl Pts',(7.33455208025131,11.9034070992466,-48.2611597032935));
#31265=CARTESIAN_POINT('Ctrl Pts',(7.32304238738767,11.9947391319378,-48.3550682080606));
#31266=CARTESIAN_POINT('Ctrl Pts',(7.30170908809363,12.1244225199508,-48.3550682080606));
#31267=CARTESIAN_POINT('Ctrl Pts',(5.69014026513413,11.6863324002422,-48.2621466998951));
#31268=CARTESIAN_POINT('Ctrl Pts',(5.68056395331838,11.7776141662045,-48.3550682080606));
#31269=CARTESIAN_POINT('Ctrl Pts',(5.66464372163471,11.9073477694537,-48.3550682080606));
#31270=CARTESIAN_POINT('Ctrl Pts',(4.03844270956242,11.5522837221933,-48.2627582883049));
#31271=CARTESIAN_POINT('Ctrl Pts',(4.03099382678731,11.6436417585081,-48.3550682080606));
#31272=CARTESIAN_POINT('Ctrl Pts',(4.02042267392571,11.7732992288254,-48.3550682080606));
#31273=CARTESIAN_POINT('Ctrl Pts',(4.30427685533896,11.5746245485739,-48.2627017315157));
#31274=CARTESIAN_POINT('Ctrl Pts',(4.30071410004375,11.5746245276893,-48.2630127553113));
#31275=CARTESIAN_POINT('Ctrl Pts',(4.29866044559197,11.5884292819489,-48.2774220038378));
#31276=CARTESIAN_POINT('Ctrl Pts',(4.29524068288583,11.6268390447666,-48.3065330737687));
#31277=CARTESIAN_POINT('Ctrl Pts',(4.29388242493259,11.651680100407,-48.3210576919341));
#31278=CARTESIAN_POINT('Ctrl Pts',(4.29256572521535,11.6756605207397,-48.3310538583792));
#31279=CARTESIAN_POINT('Origin',(0.0835265683620477,16.1705954176946,0.0824317919394229));
#31280=CARTESIAN_POINT('Origin',(48.6088737900633,16.1705954176946,-22.6047435324922));
#31281=CARTESIAN_POINT('Origin',(48.8335265683622,16.1705954176946,-44.2925682080603));
#31282=CARTESIAN_POINT('Origin',(48.833526568362,16.1705954176946,21.5181263879131));
#31283=CARTESIAN_POINT('Origin',(48.8335265683621,16.1705954176946,-21.353262804034));
#31284=CARTESIAN_POINT('Origin',(0.0835265683620477,16.1705954176946,0.0824317919394229));
#31285=CARTESIAN_POINT('Origin',(-48.4418206533391,16.1705954176946,-22.6047435324924));
#31286=CARTESIAN_POINT('Ctrl Pts',(0.0835265683594526,11.4728541727075,
-48.3550824830876));
#31287=CARTESIAN_POINT('Ctrl Pts',(0.434571873647755,11.4781922148201,-48.3550825994612));
#31288=CARTESIAN_POINT('Ctrl Pts',(0.785441203021056,11.4874426767152,-48.3536254076401));
#31289=CARTESIAN_POINT('Ctrl Pts',(1.48685396298274,11.5143737377389,-48.3502977991207));
#31290=CARTESIAN_POINT('Ctrl Pts',(1.83739739357112,11.5320543368675,-48.3484273824224));
#31291=CARTESIAN_POINT('Ctrl Pts',(2.88857791672651,11.5986492866067,-48.3459483822799));
#31292=CARTESIAN_POINT('Ctrl Pts',(3.59085027388967,11.6392592214936,-48.3412545192878));
#31293=CARTESIAN_POINT('Ctrl Pts',(4.29256572521535,11.6756605207398,-48.3310538583792));
#31294=CARTESIAN_POINT('Ctrl Pts',(0.43457187364779,11.467516130595,-48.3550823667143));
#31295=CARTESIAN_POINT('Ctrl Pts',(0.707588293928371,11.4749860898031,-48.3541407510376));
#31296=CARTESIAN_POINT('Ctrl Pts',(0.998330962585111,11.4844803122479,-48.3524253715956));
#31297=CARTESIAN_POINT('Ctrl Pts',(1.61221600331842,11.5105174196337,-48.3485410607123));
#31298=CARTESIAN_POINT('Ctrl Pts',(1.93535675582816,11.5270830007415,-48.3463749782919));
#31299=CARTESIAN_POINT('Ctrl Pts',(2.94880362400346,11.5919036248635,-48.3427355509074));
#31300=CARTESIAN_POINT('Ctrl Pts',(3.62682139903089,11.6298708101947,-48.3372561068183));
#31301=CARTESIAN_POINT('Ctrl Pts',(4.29322407507397,11.6636703105734,-48.3260557751567));
#31302=CARTESIAN_POINT('Ctrl Pts',(0.785669116593031,11.4659265087692,-48.353624938571));
#31303=CARTESIAN_POINT('Ctrl Pts',(0.998676156491118,11.4745419834779,-48.352053093827));
#31304=CARTESIAN_POINT('Ctrl Pts',(1.24336152271037,11.4840908039497,-48.3500372977499));
#31305=CARTESIAN_POINT('Ctrl Pts',(1.78640027440588,11.5090816899177,-48.3454511925554));
#31306=CARTESIAN_POINT('Ctrl Pts',(2.08475123053189,11.5245577996643,-48.3428851569693));
#31307=CARTESIAN_POINT('Ctrl Pts',(3.04577954599007,11.5859418512174,-48.3377026419571));
#31308=CARTESIAN_POINT('Ctrl Pts',(3.68879009429774,11.6209827896584,-48.3313642361181));
#31309=CARTESIAN_POINT('Ctrl Pts',(4.29389281449159,11.6514649415801,-48.3199255790041));
#31310=CARTESIAN_POINT('Ctrl Pts',(1.48799468014872,11.4643966328772,-48.3438941182188));
#31311=CARTESIAN_POINT('Ctrl Pts',(1.61377824696731,11.4744825705815,-48.3421773991261));
#31312=CARTESIAN_POINT('Ctrl Pts',(1.78770682158171,11.4843329006934,-48.340137776651));
#31313=CARTESIAN_POINT('Ctrl Pts',(2.21034412030734,11.5079260458425,-48.3350871090452));
#31314=CARTESIAN_POINT('Ctrl Pts',(2.45904980773078,11.5217114161925,-48.3320814058289));
#31315=CARTESIAN_POINT('Ctrl Pts',(3.2850802554449,11.5755468354576,-48.3246778344458));
#31316=CARTESIAN_POINT('Ctrl Pts',(3.83438595516491,11.6050189470212,-48.3171415021045));
#31317=CARTESIAN_POINT('Ctrl Pts',(4.29532858873579,11.6282480883245,-48.3065253445687));
#31318=CARTESIAN_POINT('Ctrl Pts',(1.83922300075916,11.4644563788109,-48.3356207260099));
#31319=CARTESIAN_POINT('Ctrl Pts',(1.93779750981832,11.4748353413218,-48.3343702273184));
#31320=CARTESIAN_POINT('Ctrl Pts',(2.08702911273414,11.4849166217024,-48.3325976279216));
#31321=CARTESIAN_POINT('Ctrl Pts',(2.4601131356293,11.508146276442,-48.3277770168468));
#31322=CARTESIAN_POINT('Ctrl Pts',(2.68396272136668,11.5213343690929,-48.3247339909556));
#31323=CARTESIAN_POINT('Ctrl Pts',(3.4274100778507,11.5710816706554,-48.3166668015675));
#31324=CARTESIAN_POINT('Ctrl Pts',(3.91801312076524,11.5979431249203,-48.308810638791));
#31325=CARTESIAN_POINT('Ctrl Pts',(4.29609562356237,11.6172366040622,-48.299255306286));
#31326=CARTESIAN_POINT('Ctrl Pts',(2.8931453826154,11.4583384590298,-48.2947245924959));
#31327=CARTESIAN_POINT('Ctrl Pts',(2.95442665337013,11.4700074930205,-48.2942918711471));
#31328=CARTESIAN_POINT('Ctrl Pts',(3.05143599905993,11.4818828006791,-48.2936814855085));
#31329=CARTESIAN_POINT('Ctrl Pts',(3.2896917488815,11.5065304546877,-48.2916809761507));
#31330=CARTESIAN_POINT('Ctrl Pts',(3.43093653344645,11.5193254972046,-48.2902937014525));
#31331=CARTESIAN_POINT('Ctrl Pts',(3.88020208317704,11.5598336028455,-48.2862238405637));
#31332=CARTESIAN_POINT('Ctrl Pts',(4.15587731818982,11.5806510816358,-48.2821814457028));
#31333=CARTESIAN_POINT('Ctrl Pts',(4.29866044559197,11.5884292819489,-48.2774220038378));
#31334=CARTESIAN_POINT('Ctrl Pts',(3.59439815510631,11.4609474762041,-48.2515240163507));
#31335=CARTESIAN_POINT('Ctrl Pts',(3.63137389790745,11.4731609516943,-48.2527720831628));
#31336=CARTESIAN_POINT('Ctrl Pts',(3.69355131246284,11.4863352799677,-48.2541165047803));
#31337=CARTESIAN_POINT('Ctrl Pts',(3.83871344717961,11.5121367174564,-48.256744523456));
#31338=CARTESIAN_POINT('Ctrl Pts',(3.921698167341,11.5247638266717,-48.2580281205142));
#31339=CARTESIAN_POINT('Ctrl Pts',(4.15746922938038,11.5581209387927,-48.2614073735947));
#31340=CARTESIAN_POINT('Ctrl Pts',(4.2970724728136,11.5743267261738,-48.2630314915227));
#31341=CARTESIAN_POINT('Ctrl Pts',(4.30071410004375,11.5746245276893,-48.2630127553113));
#31342=CARTESIAN_POINT('Ctrl Pts',(4.29550794738005,11.4732422824942,-48.1954680629781));
#31343=CARTESIAN_POINT('Ctrl Pts',(4.29556063460006,11.4851966459098,-48.200433936555));
#31344=CARTESIAN_POINT('Ctrl Pts',(4.29569371583995,11.4974720069511,-48.2071191491468));
#31345=CARTESIAN_POINT('Ctrl Pts',(4.29625434599591,11.5208685373805,-48.221588093388));
#31346=CARTESIAN_POINT('Ctrl Pts',(4.29668189491196,11.5319897067687,-48.2293718250376));
#31347=CARTESIAN_POINT('Ctrl Pts',(4.29860676262893,11.5609276470972,-48.2508605601154));
#31348=CARTESIAN_POINT('Ctrl Pts',(4.30074630239865,11.5743188502015,-48.2627031036729));
#31349=CARTESIAN_POINT('Ctrl Pts',(4.30427685533896,11.5746245485739,-48.2627017315157));
#31350=CARTESIAN_POINT('Ctrl Pts',(4.30427685447981,11.5746245484995,-48.2627017315161));
#31351=CARTESIAN_POINT('Ctrl Pts',(4.30406730074831,11.5746064038392,-48.2627018128455));
#31352=CARTESIAN_POINT('Ctrl Pts',(4.30391112003706,11.574549785394,-48.2626633000481));
#31353=CARTESIAN_POINT('Ctrl Pts',(4.30379489777073,11.5744984448496,-48.2626265378358));
#31354=CARTESIAN_POINT('Ctrl Pts',(4.30367838955579,11.5744469779889,-48.2625896851753));
#31355=CARTESIAN_POINT('Ctrl Pts',(4.30360215028203,11.5743997047815,-48.2625535320247));
#31356=CARTESIAN_POINT('Ctrl Pts',(4.30355585183876,11.5743705526458,-48.262531196277));
#31357=CARTESIAN_POINT('Ctrl Pts',(4.30346336852036,11.5743123198834,-48.2624865795701));
#31358=CARTESIAN_POINT('Ctrl Pts',(4.30341313104675,11.5742733795723,-48.2624559072521));
#31359=CARTESIAN_POINT('Ctrl Pts',(4.30336529688495,11.5742358022889,-48.26242627286));
#31360=CARTESIAN_POINT('Ctrl Pts',(4.30326962856134,11.5741606477221,-48.2623670040757));
#31361=CARTESIAN_POINT('Ctrl Pts',(4.30319991820999,11.5740963865912,-48.2623154901695));
#31362=CARTESIAN_POINT('Ctrl Pts',(4.30313175144365,11.574029268754,-48.2622613949826));
#31363=CARTESIAN_POINT('Ctrl Pts',(4.30289813112297,11.5737992433104,-48.2620760006094));
#31364=CARTESIAN_POINT('Ctrl Pts',(4.3027074795769,11.573544153445,-48.2618660736616));
#31365=CARTESIAN_POINT('Ctrl Pts',(4.30254169594019,11.5732903201701,-48.261656181311));
#31366=CARTESIAN_POINT('Ctrl Pts',(4.3023183694699,11.5729483823864,-48.2613734361696));
#31367=CARTESIAN_POINT('Ctrl Pts',(4.30213864866023,11.5726061687533,-48.2610884915831));
#31368=CARTESIAN_POINT('Ctrl Pts',(4.30197216232291,11.5722518188883,-48.2607931815174));
#31369=CARTESIAN_POINT('Ctrl Pts',(4.30174482657617,11.5717679570144,-48.2603899380116));
#31370=CARTESIAN_POINT('Ctrl Pts',(4.30155414381932,11.5712800182779,-48.2599826422918));
#31371=CARTESIAN_POINT('Ctrl Pts',(4.30138186491148,11.5707911792801,-48.2595751390173));
#31372=CARTESIAN_POINT('Ctrl Pts',(4.30108725143153,11.5699552176404,-48.2588782692768));
#31373=CARTESIAN_POINT('Ctrl Pts',(4.30084610919985,11.5691127678859,-48.2581774873085));
#31374=CARTESIAN_POINT('Ctrl Pts',(4.30063043411004,11.5682688436763,-48.2574784824322));
#31375=CARTESIAN_POINT('Ctrl Pts',(4.30026642622229,11.566844501768,-48.256298729644));
#31376=CARTESIAN_POINT('Ctrl Pts',(4.29997599910921,11.5654127733926,-48.2551211964302));
#31377=CARTESIAN_POINT('Ctrl Pts',(4.29971880605547,11.5639752439749,-48.2539487703289));
#31378=CARTESIAN_POINT('Ctrl Pts',(4.29931853639503,11.5617380163222,-48.2521241230817));
#31379=CARTESIAN_POINT('Ctrl Pts',(4.29900214095316,11.5594864489408,-48.2503113515096));
#31380=CARTESIAN_POINT('Ctrl Pts',(4.29872534939056,11.5572216878539,-48.2485130362479));
#31381=CARTESIAN_POINT('Ctrl Pts',(4.29830910660352,11.5538159103875,-48.2458087061396));
#31382=CARTESIAN_POINT('Ctrl Pts',(4.29798570586486,11.5503795187906,-48.2431361939227));
#31383=CARTESIAN_POINT('Ctrl Pts',(4.29770861623514,11.5469146456565,-48.2405017858792));
#31384=CARTESIAN_POINT('Ctrl Pts',(4.29756852994005,11.5451629336172,-48.2391699263543));
#31385=CARTESIAN_POINT('Ctrl Pts',(4.29744108789414,11.5434032086018,-48.2378472629719));
#31386=CARTESIAN_POINT('Ctrl Pts',(4.29732351748428,11.5416356868782,-48.2365347367302));
#31387=CARTESIAN_POINT('Ctrl Pts',(4.29694599926989,11.5359601802111,-48.2323202191171));
#31388=CARTESIAN_POINT('Ctrl Pts',(4.29666691876312,11.5302068971307,-48.228210625839));
#31389=CARTESIAN_POINT('Ctrl Pts',(4.29644147322476,11.5243619443827,-48.2242324297731));
#31390=CARTESIAN_POINT('Ctrl Pts',(4.29624888339644,11.519368816311,-48.2208340032489));
#31391=CARTESIAN_POINT('Ctrl Pts',(4.29609717557184,11.5143094135622,-48.2175317826848));
#31392=CARTESIAN_POINT('Ctrl Pts',(4.29597403091793,11.5091702721658,-48.2143536212674));
#31393=CARTESIAN_POINT('Ctrl Pts',(4.29584159356509,11.5036433226738,-48.2109356305416));
#31394=CARTESIAN_POINT('Ctrl Pts',(4.29574246556238,11.4980242335258,-48.2076595865044));
#31395=CARTESIAN_POINT('Ctrl Pts',(4.29566813462061,11.4922875984294,-48.2045854548351));
#31396=CARTESIAN_POINT('Ctrl Pts',(4.29560429163279,11.4873603915918,-48.2019450772747));
#31397=CARTESIAN_POINT('Ctrl Pts',(4.29555890131979,11.4823456579696,-48.1994525269835));
#31398=CARTESIAN_POINT('Ctrl Pts',(4.29552851076737,11.4772262324437,-48.1971803260925));
#31399=CARTESIAN_POINT('Ctrl Pts',(4.29552351828933,11.4763852270169,-48.1968070550545));
#31400=CARTESIAN_POINT('Ctrl Pts',(4.29551893289638,11.4755414144694,-48.1964398420676));
#31401=CARTESIAN_POINT('Ctrl Pts',(4.2955147414803,11.4746947555587,-48.196079159465));
#31402=CARTESIAN_POINT('Ctrl Pts',(4.29551234923451,11.4742115259827,-48.1958733002944));
#31403=CARTESIAN_POINT('Ctrl Pts',(4.29551008533479,11.4737273695405,-48.1956695693956));
#31404=CARTESIAN_POINT('Ctrl Pts',(4.29550794738005,11.4732422824942,-48.1954680629781));
#31405=CARTESIAN_POINT('Ctrl Pts',(48.8335265683621,16.4830954176946,-21.353262804034));
#31406=CARTESIAN_POINT('Ctrl Pts',(48.5210265683622,16.4830954176946,-21.353262804034));
#31407=CARTESIAN_POINT('Ctrl Pts',(48.5210265683621,16.1705954176947,-21.353262804034));
#31408=CARTESIAN_POINT('Ctrl Pts',(48.8335265706117,16.4830954176946,-21.5676091116417));
#31409=CARTESIAN_POINT('Ctrl Pts',(48.5563370700187,16.4830954176946,-21.54119704969));
#31410=CARTESIAN_POINT('Ctrl Pts',(48.5210265683621,16.2080086375453,-21.5523883700179));
#31411=CARTESIAN_POINT('Ctrl Pts',(48.8183477161632,16.4830954176946,-21.7820280540439));
#31412=CARTESIAN_POINT('Ctrl Pts',(48.5755877658885,16.4830954176946,-21.7471528982396));
#31413=CARTESIAN_POINT('Ctrl Pts',(48.5134371390849,16.2456676717398,-21.7511508011048));
#31414=CARTESIAN_POINT('Ctrl Pts',(48.7505672098116,16.4830954176946,-22.2011670980052));
#31415=CARTESIAN_POINT('Ctrl Pts',(48.5696939191561,16.4830954176946,-22.1499363086026));
#31416=CARTESIAN_POINT('Ctrl Pts',(48.4795468922649,16.319697904787,-22.1389084821703));
#31417=CARTESIAN_POINT('Ctrl Pts',(48.7009182366022,16.4830954176946,-22.407870378551));
#31418=CARTESIAN_POINT('Ctrl Pts',(48.5510364183067,16.4830954176946,-22.3516070845003));
#31419=CARTESIAN_POINT('Ctrl Pts',(48.4548516611731,16.3563211717407,-22.3292253454905));
#31420=CARTESIAN_POINT('Ctrl Pts',(48.6088737900635,16.4830954176946,-22.6047435324922));
#31421=CARTESIAN_POINT('Ctrl Pts',(48.4916148036563,16.4830954176946,-22.5499211492369));
#31422=CARTESIAN_POINT('Ctrl Pts',(48.4087001792128,16.3915662868154,-22.5111558702763));
#31423=CARTESIAN_POINT('Ctrl Pts',(48.5210265682481,16.1706033612914,-21.3533050824651));
#31424=CARTESIAN_POINT('Ctrl Pts',(48.5210260905822,16.1872388804039,-21.4418447279119));
#31425=CARTESIAN_POINT('Ctrl Pts',(48.5195289950699,16.2039304589262,-21.5303529580501));
#31426=CARTESIAN_POINT('Ctrl Pts',(48.5163532494991,16.2206573802635,-21.6187323309531));
#31427=CARTESIAN_POINT('Ctrl Pts',(48.5134900262187,16.2357382201841,-21.6984143685593));
#31428=CARTESIAN_POINT('Ctrl Pts',(48.509262165005,16.2508479929972,-21.7779925874712));
#31429=CARTESIAN_POINT('Ctrl Pts',(48.5034990985229,16.2659683787707,-21.8573738795946));
#31430=CARTESIAN_POINT('Ctrl Pts',(48.5015994066349,16.270952543761,-21.8835405041115));
#31431=CARTESIAN_POINT('Ctrl Pts',(48.499532585912,16.275937822519,-21.9096854870959));
#31432=CARTESIAN_POINT('Ctrl Pts',(48.4972915416398,16.2809234207259,-21.9358046625462));
#31433=CARTESIAN_POINT('Ctrl Pts',(48.4970276525395,16.2815104885682,-21.9388802669846));
#31434=CARTESIAN_POINT('Ctrl Pts',(48.4967613650824,16.2820975177296,-21.9419552962478));
#31435=CARTESIAN_POINT('Ctrl Pts',(48.4964926678709,16.2826845076336,-21.9450297471065));
#31436=CARTESIAN_POINT('Ctrl Pts',(48.4911785363218,16.2942936402729,-22.0058343837204));
#31437=CARTESIAN_POINT('Ctrl Pts',(48.4850832026772,16.3059124438886,-22.066544098701));
#31438=CARTESIAN_POINT('Ctrl Pts',(48.4777339713189,16.3175327023971,-22.1271197666865));
#31439=CARTESIAN_POINT('Ctrl Pts',(48.4708550229911,16.3284093715259,-22.1838191505642));
#31440=CARTESIAN_POINT('Ctrl Pts',(48.4628780808606,16.339287358577,-22.2404012791344));
#31441=CARTESIAN_POINT('Ctrl Pts',(48.453373849129,16.3501570443392,-22.2968182791175));
#31442=CARTESIAN_POINT('Ctrl Pts',(48.4445365333712,16.3602639996386,-22.34927647427));
#31443=CARTESIAN_POINT('Ctrl Pts',(48.4343790058226,16.3703637977871,-22.4015919817819));
#31444=CARTESIAN_POINT('Ctrl Pts',(48.4225135354583,16.3804457145562,-22.4537104745914));
#31445=CARTESIAN_POINT('Ctrl Pts',(48.4181477680927,16.3841552432864,-22.4728868922186));
#31446=CARTESIAN_POINT('Ctrl Pts',(48.4135503242605,16.3878623190466,-22.4920364694703));
#31447=CARTESIAN_POINT('Ctrl Pts',(48.4087001792128,16.3915662868154,-22.5111558702763));
#31448=CARTESIAN_POINT('Ctrl Pts',(48.521026568362,16.1705954176947,21.5181263879131));
#31449=CARTESIAN_POINT('Ctrl Pts',(48.521026568362,16.4830954176946,21.5181263879131));
#31450=CARTESIAN_POINT('Ctrl Pts',(48.833526568362,16.4830954176946,21.5181263879131));
#31451=CARTESIAN_POINT('Ctrl Pts',(48.521026568362,16.2080322538905,21.7173776481921));
#31452=CARTESIAN_POINT('Ctrl Pts',(48.5563586162256,16.4830954176918,21.7061753278482));
#31453=CARTESIAN_POINT('Ctrl Pts',(48.833526568103,16.4830954176946,21.7326096831721));
#31454=CARTESIAN_POINT('Ctrl Pts',(48.5135293069769,16.2453207379311,21.9141872379789));
#31455=CARTESIAN_POINT('Ctrl Pts',(48.5754705520278,16.4830954176946,21.9101416977376));
#31456=CARTESIAN_POINT('Ctrl Pts',(48.8185320523741,16.4830954176946,21.9449194637153));
#31457=CARTESIAN_POINT('Ctrl Pts',(48.4797929446078,16.3193045764618,22.3017217477063));
#31458=CARTESIAN_POINT('Ctrl Pts',(48.5698564439212,16.4830954176946,22.3126619379227));
#31459=CARTESIAN_POINT('Ctrl Pts',(48.7510593140707,16.4830954176946,22.3638116144414));
#31460=CARTESIAN_POINT('Ctrl Pts',(48.4548701098381,16.3563070925481,22.4940162271868));
#31461=CARTESIAN_POINT('Ctrl Pts',(48.5510669794482,16.483095417693,22.5163687361117));
#31462=CARTESIAN_POINT('Ctrl Pts',(48.700968878949,16.4830954176946,22.5726256902424));
#31463=CARTESIAN_POINT('Ctrl Pts',(48.4087001792127,16.3915662868154,22.6760194541556));
#31464=CARTESIAN_POINT('Ctrl Pts',(48.4916148036562,16.4830954176946,22.7147847331162));
#31465=CARTESIAN_POINT('Ctrl Pts',(48.6088737900633,16.4830954176946,22.7696071163714));
#31466=CARTESIAN_POINT('Ctrl Pts',(48.4087001792127,16.3915662868154,22.6760194541555));
#31467=CARTESIAN_POINT('Ctrl Pts',(48.4215041465258,16.3817881293016,22.6255458743838));
#31468=CARTESIAN_POINT('Ctrl Pts',(48.4325629456394,16.3719647253873,22.5747387277194));
#31469=CARTESIAN_POINT('Ctrl Pts',(48.442243951573,16.3621195256861,22.5237189880492));
#31470=CARTESIAN_POINT('Ctrl Pts',(48.4524806610765,16.351709197458,22.4697706424398));
#31471=CARTESIAN_POINT('Ctrl Pts',(48.4611763864365,16.3412744261774,22.4155842444699));
#31472=CARTESIAN_POINT('Ctrl Pts',(48.4687118641718,16.3308372397184,22.3612726664185));
#31473=CARTESIAN_POINT('Ctrl Pts',(48.4771655296529,16.3191282962395,22.3003432962141));
#31474=CARTESIAN_POINT('Ctrl Pts',(48.4841586198759,16.3074162297974,22.239256014571));
#31475=CARTESIAN_POINT('Ctrl Pts',(48.4901689987576,16.2957263502233,22.1781386555071));
#31476=CARTESIAN_POINT('Ctrl Pts',(48.4924694182924,16.2912521518638,22.1547465250811));
#31477=CARTESIAN_POINT('Ctrl Pts',(48.4946253459155,16.2867811561769,22.1313497223861));
#31478=CARTESIAN_POINT('Ctrl Pts',(48.4966618765561,16.2823146437397,22.1079546137713));
#31479=CARTESIAN_POINT('Ctrl Pts',(48.49689257277,16.2818086815469,22.1053044385793));
#31480=CARTESIAN_POINT('Ctrl Pts',(48.4971214898655,16.2813027193741,22.1026539911944));
#31481=CARTESIAN_POINT('Ctrl Pts',(48.4973486349728,16.2807967549782,22.1000032598185));
#31482=CARTESIAN_POINT('Ctrl Pts',(48.5070811654924,16.2591176002569,21.9864268578278));
#31483=CARTESIAN_POINT('Ctrl Pts',(48.5135451570134,16.2374836515957,21.872573572219));
#31484=CARTESIAN_POINT('Ctrl Pts',(48.5172287291613,16.2159059273928,21.7584858701599));
#31485=CARTESIAN_POINT('Ctrl Pts',(48.5198114921994,16.2007765512654,21.6784924593757));
#31486=CARTESIAN_POINT('Ctrl Pts',(48.5210261401518,16.1856747351528,21.5983834228076));
#31487=CARTESIAN_POINT('Ctrl Pts',(48.5210265682489,16.1706033824536,21.518168778977));
#31488=CARTESIAN_POINT('Origin',(48.6088737900632,16.1705954176946,22.7696071163714));
#31489=CARTESIAN_POINT('Ctrl Pts',(-48.3539734316379,16.1705954176947,-21.3532628040341));
#31490=CARTESIAN_POINT('Ctrl Pts',(-48.353973431638,16.4830954176946,-21.3532628040341));
#31491=CARTESIAN_POINT('Ctrl Pts',(-48.6664734316379,16.4830954176946,-21.3532628040341));
#31492=CARTESIAN_POINT('Ctrl Pts',(-48.3539734316379,16.2080105885521,-21.5523987534991));
#31493=CARTESIAN_POINT('Ctrl Pts',(-48.3892858729637,16.4830954176974,-21.5412073890877));
#31494=CARTESIAN_POINT('Ctrl Pts',(-48.6664734316171,16.4830954176946,-21.5676219963864));
#31495=CARTESIAN_POINT('Ctrl Pts',(-48.3464913697085,16.2453321156391,-21.7493863021592));
#31496=CARTESIAN_POINT('Ctrl Pts',(-48.4084615410216,16.483095417695,-21.7452887921056));
#31497=CARTESIAN_POINT('Ctrl Pts',(-48.6515093147605,16.4830954176946,-21.7801227265566));
#31498=CARTESIAN_POINT('Ctrl Pts',(-48.3126208434,16.3195206182106,-22.137986751486));
#31499=CARTESIAN_POINT('Ctrl Pts',(-48.4027468354045,16.4830954176942,-22.1489298171496));
#31500=CARTESIAN_POINT('Ctrl Pts',(-48.5837682481807,16.4830954176946,-22.2001688119519));
#31501=CARTESIAN_POINT('Ctrl Pts',(-48.2869930772645,16.3569362864368,-22.3324004616851));
#31502=CARTESIAN_POINT('Ctrl Pts',(-48.3829333544402,16.4830954176958,-22.355111170887));
#31503=CARTESIAN_POINT('Ctrl Pts',(-48.5323224387334,16.4830954176946,-22.4111700033582));
#31504=CARTESIAN_POINT('Ctrl Pts',(-48.241647042494,16.391566286814,-22.5111558702805));
#31505=CARTESIAN_POINT('Ctrl Pts',(-48.324561666938,16.4830954176946,-22.5499211492407));
#31506=CARTESIAN_POINT('Ctrl Pts',(-48.4418206533465,16.4830954176946,-22.6047435324958));
#31507=CARTESIAN_POINT('Origin',(-48.6664734316379,16.1705954176946,-21.3532628040342));
#31508=CARTESIAN_POINT('Ctrl Pts',(-48.2416470424944,16.3915662868137,-22.511155870279));
#31509=CARTESIAN_POINT('Ctrl Pts',(-48.2516296638352,16.3839427400264,-22.4718041113854));
#31510=CARTESIAN_POINT('Ctrl Pts',(-48.260532619053,16.3762820912579,-22.4321984891174));
#31511=CARTESIAN_POINT('Ctrl Pts',(-48.2685549114895,16.3686030213912,-22.3924368065077));
#31512=CARTESIAN_POINT('Ctrl Pts',(-48.2774078505434,16.3601288429616,-22.3485581077925));
#31513=CARTESIAN_POINT('Ctrl Pts',(-48.285188292822,16.3516321729391,-22.3044890886349));
#31514=CARTESIAN_POINT('Ctrl Pts',(-48.2921179089163,16.343129468787,-22.2603152652558));
#31515=CARTESIAN_POINT('Ctrl Pts',(-48.2995987350645,16.3339504247122,-22.2126276749908));
#31516=CARTESIAN_POINT('Ctrl Pts',(-48.3060875995565,16.3247641828062,-22.1648171335444));
#31517=CARTESIAN_POINT('Ctrl Pts',(-48.3118160984604,16.315583691338,-22.1169491583698));
#31518=CARTESIAN_POINT('Ctrl Pts',(-48.3187204578189,16.3045187660849,-22.0592555622088));
#31519=CARTESIAN_POINT('Ctrl Pts',(-48.3245201692789,16.2934618759648,-22.0014770742633));
#31520=CARTESIAN_POINT('Ctrl Pts',(-48.3295569233971,16.2824285258603,-21.9436866585553));
#31521=CARTESIAN_POINT('Ctrl Pts',(-48.329804419995,16.2818863678454,-21.9408469465223));
#31522=CARTESIAN_POINT('Ctrl Pts',(-48.3300499019331,16.2813441490099,-21.9380066039067));
#31523=CARTESIAN_POINT('Ctrl Pts',(-48.3302933786148,16.2808018618168,-21.9351655909642));
#31524=CARTESIAN_POINT('Ctrl Pts',(-48.3403316897726,16.2584438785268,-21.8180333394403));
#31525=CARTESIAN_POINT('Ctrl Pts',(-48.3468913580189,16.2361414811697,-21.7006457858735));
#31526=CARTESIAN_POINT('Ctrl Pts',(-48.3505104144184,16.2139052642594,-21.5830426396001));
#31527=CARTESIAN_POINT('Ctrl Pts',(-48.3528642839503,16.1994426122,-21.5065524078089));
#31528=CARTESIAN_POINT('Ctrl Pts',(-48.353973022726,16.1850078872687,-21.4299706573745));
#31529=CARTESIAN_POINT('Ctrl Pts',(-48.3539734315249,16.1706033824528,-21.353305195093));
#31530=CARTESIAN_POINT('Ctrl Pts',(-48.2412034662232,16.4951170400788,-22.7555193836954));
#31531=CARTESIAN_POINT('Ctrl Pts',(-48.353973431638,16.5812943361539,-22.718696491988));
#31532=CARTESIAN_POINT('Ctrl Pts',(-48.353973431638,16.716129330846,-22.6610856347191));
#31533=CARTESIAN_POINT('Ctrl Pts',(-48.245981940911,15.222424873626,-19.7666451786995));
#31534=CARTESIAN_POINT('Ctrl Pts',(-48.353973431638,15.3157731517017,-19.7471174013183));
#31535=CARTESIAN_POINT('Ctrl Pts',(-48.353973431638,15.4434377916669,-19.6823200414401));
#31536=CARTESIAN_POINT('Ctrl Pts',(-48.2504725327236,14.1211388850897,-16.7051598239745));
#31537=CARTESIAN_POINT('Ctrl Pts',(-48.3539734316379,14.2126904025447,-16.6868950101451));
#31538=CARTESIAN_POINT('Ctrl Pts',(-48.3539734316379,14.3421540079377,-16.6323059622874));
#31539=CARTESIAN_POINT('Ctrl Pts',(-48.2559025241611,12.8451845281714,-11.9819322414057));
#31540=CARTESIAN_POINT('Ctrl Pts',(-48.3539734316379,12.9358419174516,-11.9627573972046));
#31541=CARTESIAN_POINT('Ctrl Pts',(-48.3539734316379,13.0661994464396,-11.9283372932442));
#31542=CARTESIAN_POINT('Ctrl Pts',(-48.2574842477434,12.4841939488209,-10.3943253952016));
#31543=CARTESIAN_POINT('Ctrl Pts',(-48.353973431638,12.5748700381568,-10.377060491345));
#31544=CARTESIAN_POINT('Ctrl Pts',(-48.3539734316379,12.7052089420493,-10.3474501811343));
#31545=CARTESIAN_POINT('Ctrl Pts',(-48.2600649268728,11.9034070980987,-7.16859371359221));
#31546=CARTESIAN_POINT('Ctrl Pts',(-48.3539734316379,11.9947391307946,-7.15708402075537));
#31547=CARTESIAN_POINT('Ctrl Pts',(-48.3539734316379,12.1244225188063,-7.13575072146176));
#31548=CARTESIAN_POINT('Ctrl Pts',(-48.2610519234887,11.6863323985655,-5.5241818920662));
#31549=CARTESIAN_POINT('Ctrl Pts',(-48.353973431638,11.7776141645414,-5.51460558027628));
#31550=CARTESIAN_POINT('Ctrl Pts',(-48.3539734316379,11.9073477677922,-5.49868534862248));
#31551=CARTESIAN_POINT('Ctrl Pts',(-48.261663511885,11.5522837206279,-3.87248433002591));
#31552=CARTESIAN_POINT('Ctrl Pts',(-48.353973431638,11.6436417569439,-3.86503544728664));
#31553=CARTESIAN_POINT('Ctrl Pts',(-48.3539734316379,11.7732992272621,-3.85446429447611));
#31554=CARTESIAN_POINT('Origin',(0.0835265683620477,11.3536536794531,0.0824317919394229));
#31555=CARTESIAN_POINT('Origin',(0.0835265683620477,11.3536536794531,0.0824317919394229));
#31556=CARTESIAN_POINT('Ctrl Pts',(48.5210265683622,16.8990456170575,-23.0860157986068));
#31557=CARTESIAN_POINT('Ctrl Pts',(48.5210265683622,16.7639535854308,-23.14458938147));
#31558=CARTESIAN_POINT('Ctrl Pts',(48.4074773267406,16.6779610391845,-23.1819141669453));
#31559=CARTESIAN_POINT('Ctrl Pts',(48.5210265683621,15.5488264423803,-19.9724299127091));
#31560=CARTESIAN_POINT('Ctrl Pts',(48.5210265683621,15.421754102374,-20.0395475263466));
#31561=CARTESIAN_POINT('Ctrl Pts',(48.4125145055694,15.3277344823348,-20.0578585833071));
#31562=CARTESIAN_POINT('Ctrl Pts',(48.5210265683621,14.3828771896198,-16.7823795949988));
#31563=CARTESIAN_POINT('Ctrl Pts',(48.5210265683621,14.2535943246426,-16.8384455883479));
#31564=CARTESIAN_POINT('Ctrl Pts',(48.4172647900869,14.1617844287939,-16.8558621541832));
#31565=CARTESIAN_POINT('Ctrl Pts',(48.5210265683621,13.0662924545663,-11.9287072175551));
#31566=CARTESIAN_POINT('Ctrl Pts',(48.5210265683621,12.9358690854413,-11.9631452471962));
#31567=CARTESIAN_POINT('Ctrl Pts',(48.4228719618904,12.845200563322,-11.9823199869963));
#31568=CARTESIAN_POINT('Ctrl Pts',(48.5210265683621,12.7052707111109,-10.3477586668265));
#31569=CARTESIAN_POINT('Ctrl Pts',(48.5210265683621,12.5748662546476,-10.377384989854));
#31570=CARTESIAN_POINT('Ctrl Pts',(48.4244550341077,12.4841786131515,-10.3946498939195));
#31571=CARTESIAN_POINT('Ctrl Pts',(48.5210265683621,12.0967706305342,-6.98287544832615));
#31572=CARTESIAN_POINT('Ctrl Pts',(48.5210265683621,11.9671239054848,-7.00421648724047));
#31573=CARTESIAN_POINT('Ctrl Pts',(48.4271609489138,11.8756772066794,-7.01505958302208));
#31574=CARTESIAN_POINT('Ctrl Pts',(48.5210265683621,11.867306293034,-5.19149268823613));
#31575=CARTESIAN_POINT('Ctrl Pts',(48.5210265683621,11.7375302448688,-5.20668019500151));
#31576=CARTESIAN_POINT('Ctrl Pts',(48.4282082222567,11.6462130037594,-5.21561646581236));
#31577=CARTESIAN_POINT('Ctrl Pts',(48.5210265683621,11.7377723215061,-3.39157010211078));
#31578=CARTESIAN_POINT('Ctrl Pts',(48.521026568362,11.6080928971653,-3.40090234579438));
#31579=CARTESIAN_POINT('Ctrl Pts',(48.4288000980576,11.5166787215354,-3.4074882922648));
#31580=CARTESIAN_POINT('Ctrl Pts',(48.4082566029293,16.4951170442608,22.9203829774002));
#31581=CARTESIAN_POINT('Ctrl Pts',(48.521026568362,16.5812943403342,22.8835600856804));
#31582=CARTESIAN_POINT('Ctrl Pts',(48.521026568362,16.716129335031,22.8259492283893));
#31583=CARTESIAN_POINT('Ctrl Pts',(48.4130350776236,15.2224248760375,19.9315087692866));
#31584=CARTESIAN_POINT('Ctrl Pts',(48.521026568362,15.3157731540769,19.9119809919554));
#31585=CARTESIAN_POINT('Ctrl Pts',(48.521026568362,15.4434377940522,19.8471836320167));
#31586=CARTESIAN_POINT('Ctrl Pts',(48.4175256694355,14.12113888602,16.870023411326));
#31587=CARTESIAN_POINT('Ctrl Pts',(48.521026568362,14.2126904034778,16.8517585975199));
#31588=CARTESIAN_POINT('Ctrl Pts',(48.521026568362,14.3421540088633,16.7971695496233));
#31589=CARTESIAN_POINT('Ctrl Pts',(48.4229556608863,12.8451845281721,12.1467958252831));
#31590=CARTESIAN_POINT('Ctrl Pts',(48.521026568362,12.9358419174544,12.1276209810818));
#31591=CARTESIAN_POINT('Ctrl Pts',(48.521026568362,13.0661994464451,12.0932008771218));
#31592=CARTESIAN_POINT('Ctrl Pts',(48.4245373844683,12.4841939488219,10.5591889790814));
#31593=CARTESIAN_POINT('Ctrl Pts',(48.521026568362,12.5748700381609,10.541924075223));
#31594=CARTESIAN_POINT('Ctrl Pts',(48.521026568362,12.7052089420549,10.5123137650119));
#31595=CARTESIAN_POINT('Ctrl Pts',(48.427118063595,11.9034070974575,7.33345729393522));
#31596=CARTESIAN_POINT('Ctrl Pts',(48.521026568362,11.9947391301531,7.32194760111541));
#31597=CARTESIAN_POINT('Ctrl Pts',(48.521026568362,12.124422518164,7.30061430182188));
#31598=CARTESIAN_POINT('Ctrl Pts',(48.4281050602037,11.686332397615,5.68904546884577));
#31599=CARTESIAN_POINT('Ctrl Pts',(48.5210265683621,11.7776141635803,5.67946915707043));
#31600=CARTESIAN_POINT('Ctrl Pts',(48.521026568362,11.9073477668319,5.66354892543314));
#31601=CARTESIAN_POINT('Ctrl Pts',(48.4287166486124,11.5522837197589,4.03734790320594));
#31602=CARTESIAN_POINT('Ctrl Pts',(48.5210265683621,11.6436417560773,4.02989902048659));
#31603=CARTESIAN_POINT('Ctrl Pts',(48.521026568362,11.7732992263959,4.01932786770446));
#31604=CARTESIAN_POINT('Ctrl Pts',(48.4286600918172,11.5746245485738,4.30318207891633));
#31605=CARTESIAN_POINT('Ctrl Pts',(48.4289711156128,11.5746245276893,4.29961932362112));
#31606=CARTESIAN_POINT('Ctrl Pts',(48.4433803641393,11.5884292819488,4.29756566916935));
#31607=CARTESIAN_POINT('Ctrl Pts',(48.4724914340702,11.6268390447666,4.29414590646321));
#31608=CARTESIAN_POINT('Ctrl Pts',(48.4870160522355,11.6516801004069,4.29278764850995));
#31609=CARTESIAN_POINT('Ctrl Pts',(48.4970122186807,11.6756605207397,4.29147094879272));
#31610=CARTESIAN_POINT('Origin',(0.0835265683620477,16.1705954176946,0.0824317919394229));
#31611=CARTESIAN_POINT('Origin',(22.7707018927938,16.1705954176946,48.6077790136406));
#31612=CARTESIAN_POINT('Origin',(-48.6664734316379,16.1705954176946,-44.2925682080606));
#31613=CARTESIAN_POINT('Origin',(-48.6664734316379,16.1705954176946,21.5181263879129));
#31614=CARTESIAN_POINT('Ctrl Pts',(-48.3539734316379,16.8990456227292,23.2508793955723));
#31615=CARTESIAN_POINT('Ctrl Pts',(-48.3539734316379,16.7639535910939,23.3094529784638));
#31616=CARTESIAN_POINT('Ctrl Pts',(-48.2404241899901,16.6779610448551,23.3467777639552));
#31617=CARTESIAN_POINT('Ctrl Pts',(-48.3539734316379,15.5488264456615,20.1372935055198));
#31618=CARTESIAN_POINT('Ctrl Pts',(-48.3539734316379,15.4217541056756,20.204411119231));
#31619=CARTESIAN_POINT('Ctrl Pts',(-48.2454613688405,15.3277344856077,20.2227221761541));
#31620=CARTESIAN_POINT('Ctrl Pts',(-48.3539734316379,14.3828771908746,16.9472431835038));
#31621=CARTESIAN_POINT('Ctrl Pts',(-48.353973431638,14.2535943258927,17.0033091768937));
#31622=CARTESIAN_POINT('Ctrl Pts',(-48.2502116533547,14.1617844300463,17.0207257427074));
#31623=CARTESIAN_POINT('Ctrl Pts',(-48.3539734316379,13.0662924545663,12.0935708014341));
#31624=CARTESIAN_POINT('Ctrl Pts',(-48.3539734316379,12.9358690854431,12.1280088310745));
#31625=CARTESIAN_POINT('Ctrl Pts',(-48.2558188251637,12.8452005633196,12.1471835708758));
#31626=CARTESIAN_POINT('Ctrl Pts',(-48.3539734316379,12.7052707111123,10.5126222507054));
#31627=CARTESIAN_POINT('Ctrl Pts',(-48.3539734316379,12.5748662546484,10.5422485737337));
#31628=CARTESIAN_POINT('Ctrl Pts',(-48.2574018973817,12.4841786131498,10.5595134777991));
#31629=CARTESIAN_POINT('Ctrl Pts',(-48.3539734316379,12.09677062968,7.14773902748995));
#31630=CARTESIAN_POINT('Ctrl Pts',(-48.353973431638,11.9671239046302,7.16908006640543));
#31631=CARTESIAN_POINT('Ctrl Pts',(-48.2601078121902,11.8756772058235,7.17992316216539));
#31632=CARTESIAN_POINT('Ctrl Pts',(-48.353973431638,11.8673062918515,5.35635626264026));
#31633=CARTESIAN_POINT('Ctrl Pts',(-48.3539734316379,11.7375302436853,5.37154376938283));
#31634=CARTESIAN_POINT('Ctrl Pts',(-48.261155085551,11.6462130025588,5.38048004017552));
#31635=CARTESIAN_POINT('Ctrl Pts',(-48.353973431638,11.7377723204669,3.55643367171442));
#31636=CARTESIAN_POINT('Ctrl Pts',(-48.353973431638,11.6080928961254,3.5657659153597));
#31637=CARTESIAN_POINT('Ctrl Pts',(-48.2617469613299,11.5166787204998,3.57235186180297));
#31638=CARTESIAN_POINT('Ctrl Pts',(-48.2416470424886,16.3915662868154,22.6760194541553));
#31639=CARTESIAN_POINT('Ctrl Pts',(-48.2550583113966,16.3813243440928,22.6231518753406));
#31640=CARTESIAN_POINT('Ctrl Pts',(-48.2665413365694,16.371060182303,22.5700615306077));
#31641=CARTESIAN_POINT('Ctrl Pts',(-48.2765223146654,16.3607859543218,22.5168101838168));
#31642=CARTESIAN_POINT('Ctrl Pts',(-48.2870013352819,16.3499990508944,22.4609016390319));
#31643=CARTESIAN_POINT('Ctrl Pts',(-48.2958241781355,16.3392010160241,22.404815463508));
#31644=CARTESIAN_POINT('Ctrl Pts',(-48.3034279033223,16.3284020448452,22.3486028384447));
#31645=CARTESIAN_POINT('Ctrl Pts',(-48.3117577974371,16.3165717532105,22.2870218103047));
#31646=CARTESIAN_POINT('Ctrl Pts',(-48.318624191821,16.304740305612,22.225288907512));
#31647=CARTESIAN_POINT('Ctrl Pts',(-48.3245425371134,16.2929170788295,22.1634496834489));
#31648=CARTESIAN_POINT('Ctrl Pts',(-48.3262538527391,16.289498340696,22.1455685992625));
#31649=CARTESIAN_POINT('Ctrl Pts',(-48.3278855787644,16.2860802681944,22.12767850517));
#31650=CARTESIAN_POINT('Ctrl Pts',(-48.3294494632194,16.2826630404187,22.1097802343589));
#31651=CARTESIAN_POINT('Ctrl Pts',(-48.3297163898139,16.282079781873,22.1067253255002));
#31652=CARTESIAN_POINT('Ctrl Pts',(-48.3299809399224,16.2814964941327,22.1036698975148));
#31653=CARTESIAN_POINT('Ctrl Pts',(-48.3302431245746,16.2809131770539,22.1006139497897));
#31654=CARTESIAN_POINT('Ctrl Pts',(-48.3374362318239,16.2649097143329,22.0167731927283));
#31655=CARTESIAN_POINT('Ctrl Pts',(-48.3428413032002,16.2489117074373,21.9326789574656));
#31656=CARTESIAN_POINT('Ctrl Pts',(-48.346668755976,16.2329404500536,21.8484396681528));
#31657=CARTESIAN_POINT('Ctrl Pts',(-48.3508266167155,16.2155904609288,21.7569283538995));
#31658=CARTESIAN_POINT('Ctrl Pts',(-48.3531227295817,16.1982718719703,21.6652451220175));
#31659=CARTESIAN_POINT('Ctrl Pts',(-48.353776871749,16.1810063870583,21.573494203965));
#31660=CARTESIAN_POINT('Ctrl Pts',(-48.3539083353861,16.177536524456,21.5550549257804));
#31661=CARTESIAN_POINT('Ctrl Pts',(-48.3539733323427,16.1740687951328,21.5366128328767));
#31662=CARTESIAN_POINT('Ctrl Pts',(-48.3539734315243,16.1706033612909,21.5181686663419));
#31663=CARTESIAN_POINT('Ctrl Pts',(-48.353987706665,11.4728541727075,0.0824317919420715));
#31664=CARTESIAN_POINT('Ctrl Pts',(-48.3539872411712,11.4515020042572,0.0824317919420012));
#31665=CARTESIAN_POINT('Ctrl Pts',(-48.3536289324683,11.4284235901226,0.0824317919405622));
#31666=CARTESIAN_POINT('Ctrl Pts',(-48.3495242803204,11.3941472536996,0.0824317919402862));
#31667=CARTESIAN_POINT('Ctrl Pts',(-48.3539734316379,11.3720285904897,0.08243179194024));
#31668=CARTESIAN_POINT('Ctrl Pts',(-48.3539734316379,11.3536536794531,0.0824317919394318));
#31669=CARTESIAN_POINT('Ctrl Pts',(-48.3539875902917,11.4675161305949,0.433477097230381));
#31670=CARTESIAN_POINT('Ctrl Pts',(-48.3539275501285,11.4488974993902,0.355621276400125));
#31671=CARTESIAN_POINT('Ctrl Pts',(-48.353663231583,11.4285976962987,0.338435236571238));
#31672=CARTESIAN_POINT('Ctrl Pts',(-48.3495016478723,11.3940705712691,0.360237634010735));
#31673=CARTESIAN_POINT('Ctrl Pts',(-48.3539734316379,11.3720285904897,0.399226071278088));
#31674=CARTESIAN_POINT('Ctrl Pts',(-48.3539734316379,11.3536536794531,0.433719204637307));
#31675=CARTESIAN_POINT('Ctrl Pts',(-48.3525301621484,11.4659265087691,0.784574340176142));
#31676=CARTESIAN_POINT('Ctrl Pts',(-48.3527335277693,11.447718516688,0.651206502089013));
#31677=CARTESIAN_POINT('Ctrl Pts',(-48.3522992264021,11.428587933622,0.625439688759691));
#31678=CARTESIAN_POINT('Ctrl Pts',(-48.3473885439727,11.3934281614349,0.66646486508276));
#31679=CARTESIAN_POINT('Ctrl Pts',(-48.3508557705029,11.3718199008203,0.733256854734286));
#31680=CARTESIAN_POINT('Ctrl Pts',(-48.3501520759131,11.3536536794531,0.785006622606324));
#31681=CARTESIAN_POINT('Ctrl Pts',(-48.3427993417961,11.4643966328771,1.48689990373394));
#31682=CARTESIAN_POINT('Ctrl Pts',(-48.3443675175871,11.4452664260877,1.29386039425038));
#31683=CARTESIAN_POINT('Ctrl Pts',(-48.3432090309081,11.4271829834973,1.26166887657828));
#31684=CARTESIAN_POINT('Ctrl Pts',(-48.3361366891649,11.39130385313,1.32614678064444));
#31685=CARTESIAN_POINT('Ctrl Pts',(-48.3366948692382,11.3711415135622,1.42281620238213));
#31686=CARTESIAN_POINT('Ctrl Pts',(-48.3348648315386,11.3536536794531,1.48749857171648));
#31687=CARTESIAN_POINT('Ctrl Pts',(-48.334525949587,11.4644563788108,1.83812822434599));
#31688=CARTESIAN_POINT('Ctrl Pts',(-48.3370692580422,11.4439380177891,1.64093757517121));
#31689=CARTESIAN_POINT('Ctrl Pts',(-48.3353565172244,11.425732495649,1.61090009066833));
#31690=CARTESIAN_POINT('Ctrl Pts',(-48.326934699005,11.389794304459,1.67960165301714));
#31691=CARTESIAN_POINT('Ctrl Pts',(-48.3256515256245,11.3706718159735,1.77834069986839));
#31692=CARTESIAN_POINT('Ctrl Pts',(-48.3233989425165,11.3536536794531,1.83870311340059));
#31693=CARTESIAN_POINT('Ctrl Pts',(-48.3072618605772,11.4603777656236,2.54074314558774));
#31694=CARTESIAN_POINT('Ctrl Pts',(-48.3087333779098,11.4381382649983,2.39327412400269));
#31695=CARTESIAN_POINT('Ctrl Pts',(-48.3062335055346,11.4203247666438,2.37176704511889));
#31696=CARTESIAN_POINT('Ctrl Pts',(-48.2977571518657,11.3861758639155,2.42404521997606));
#31697=CARTESIAN_POINT('Ctrl Pts',(-48.2950709238183,11.3696277842964,2.49783047371681));
#31698=CARTESIAN_POINT('Ctrl Pts',(-48.2928171719614,11.3536536794531,2.54094611738018));
#31699=CARTESIAN_POINT('Ctrl Pts',(-48.2896456942886,11.4600103666203,2.8917100690178));
#31700=CARTESIAN_POINT('Ctrl Pts',(-48.2899913249917,11.4370088609558,2.76883563487708));
#31701=CARTESIAN_POINT('Ctrl Pts',(-48.2869150458799,11.4187667259072,2.75380781417152));
#31702=CARTESIAN_POINT('Ctrl Pts',(-48.2785859525266,11.3847952022384,2.80028584083724));
#31703=CARTESIAN_POINT('Ctrl Pts',(-48.2755338718729,11.369053450208,2.86179168820836));
#31704=CARTESIAN_POINT('Ctrl Pts',(-48.2737012896825,11.3536536794531,2.89198459022056));
#31705=CARTESIAN_POINT('Ctrl Pts',(-48.2472153956208,11.4633689234831,3.59326763363504));
#31706=CARTESIAN_POINT('Ctrl Pts',(-48.2437182974631,11.4394032486783,3.52561349527619));
#31707=CARTESIAN_POINT('Ctrl Pts',(-48.2392225168533,11.4193327724023,3.52141678779854));
#31708=CARTESIAN_POINT('Ctrl Pts',(-48.2313449268363,11.3835624194323,3.55118314893263));
#31709=CARTESIAN_POINT('Ctrl Pts',(-48.2285187243939,11.3679565169509,3.58514621754432));
#31710=CARTESIAN_POINT('Ctrl Pts',(-48.2278104516838,11.3536536794531,3.59381163136407));
#31711=CARTESIAN_POINT('Ctrl Pts',(-48.2224012632416,11.4670948793492,3.94385827482222));
#31712=CARTESIAN_POINT('Ctrl Pts',(-48.2161873228526,11.4429270404433,3.90682984480091));
#31713=CARTESIAN_POINT('Ctrl Pts',(-48.2108487059855,11.4214568596339,3.9069829679927));
#31714=CARTESIAN_POINT('Ctrl Pts',(-48.203275617213,11.3837102983034,3.92583579004338));
#31715=CARTESIAN_POINT('Ctrl Pts',(-48.2010411453076,11.3674339177823,3.94453548890227));
#31716=CARTESIAN_POINT('Ctrl Pts',(-48.2010354948423,11.3536536794531,3.94460021021516));
#31717=CARTESIAN_POINT('Ctrl Pts',(-48.1943732865555,11.4732422824942,4.29441317095732));
#31718=CARTESIAN_POINT('Ctrl Pts',(-48.1844415394016,11.4493335556629,4.29430779651731));
#31719=CARTESIAN_POINT('Ctrl Pts',(-48.178454383799,11.4261172510678,4.29450986621179));
#31720=CARTESIAN_POINT('Ctrl Pts',(-48.1714459461707,11.384958159128,4.29496669282076));
#31721=CARTESIAN_POINT('Ctrl Pts',(-48.170424664145,11.3670153717833,4.29522144973525));
#31722=CARTESIAN_POINT('Ctrl Pts',(-48.170424664145,11.3536536794531,4.29522144973525));
#31723=CARTESIAN_POINT('Origin',(-48.483024238303,11.3534224546476,4.32103607293009));
#31724=CARTESIAN_POINT('Ctrl Pts',(48.5210408433891,11.4728541727075,0.0824317919368853));
#31725=CARTESIAN_POINT('Ctrl Pts',(48.5210409597623,11.4781922148201,0.4334770972252));
#31726=CARTESIAN_POINT('Ctrl Pts',(48.5195837679409,11.4874426767152,0.784346426598513));
#31727=CARTESIAN_POINT('Ctrl Pts',(48.5162561594212,11.5143737377389,1.48575918656021));
#31728=CARTESIAN_POINT('Ctrl Pts',(48.5143857427228,11.5320543368676,1.83630261714859));
#31729=CARTESIAN_POINT('Ctrl Pts',(48.5119067425813,11.5986492866067,2.88748314030395));
#31730=CARTESIAN_POINT('Ctrl Pts',(48.5072128795892,11.6392592214936,3.58975549746708));
#31731=CARTESIAN_POINT('Ctrl Pts',(48.4970122186807,11.6756605207398,4.29147094879272));
#31732=CARTESIAN_POINT('Ctrl Pts',(48.5210407270154,11.467516130595,0.433477097225236));
#31733=CARTESIAN_POINT('Ctrl Pts',(48.5200991113385,11.4749860898032,0.706493517505826));
#31734=CARTESIAN_POINT('Ctrl Pts',(48.5183837318963,11.484480312248,0.997236186162579));
#31735=CARTESIAN_POINT('Ctrl Pts',(48.5144994210127,11.5105174196337,1.61112122689591));
#31736=CARTESIAN_POINT('Ctrl Pts',(48.5123333385923,11.5270830007415,1.93426197940565));
#31737=CARTESIAN_POINT('Ctrl Pts',(48.5086939112088,11.5919036248635,2.94770884758093));
#31738=CARTESIAN_POINT('Ctrl Pts',(48.5032144671198,11.6298708101947,3.62572662260832));
#31739=CARTESIAN_POINT('Ctrl Pts',(48.4920141354581,11.6636703105733,4.29212929865133));
#31740=CARTESIAN_POINT('Ctrl Pts',(48.5195832988718,11.4659265087693,0.784574340170486));
#31741=CARTESIAN_POINT('Ctrl Pts',(48.5180114541276,11.4745419834779,0.997581380068577));
#31742=CARTESIAN_POINT('Ctrl Pts',(48.5159956580504,11.4840908039497,1.24226674628784));
#31743=CARTESIAN_POINT('Ctrl Pts',(48.5114095528557,11.5090816899177,1.78530549798337));
#31744=CARTESIAN_POINT('Ctrl Pts',(48.5088435172697,11.5245577996643,2.08365645410939));
#31745=CARTESIAN_POINT('Ctrl Pts',(48.5036610022584,11.5859418512174,3.04468476956754));
#31746=CARTESIAN_POINT('Ctrl Pts',(48.4973225964196,11.6209827896584,3.68769531787518));
#31747=CARTESIAN_POINT('Ctrl Pts',(48.4858839393055,11.6514649415801,4.29279803806896));
#31748=CARTESIAN_POINT('Ctrl Pts',(48.5098524785193,11.4643966328772,1.48689990372619));
#31749=CARTESIAN_POINT('Ctrl Pts',(48.5081357594265,11.4744825705816,1.61268347054477));
#31750=CARTESIAN_POINT('Ctrl Pts',(48.5060961369513,11.4843329006934,1.78661204515917));
#31751=CARTESIAN_POINT('Ctrl Pts',(48.5010454693456,11.5079260458425,2.20924934388482));
#31752=CARTESIAN_POINT('Ctrl Pts',(48.4980397661294,11.5217114161925,2.45795503130826));
#31753=CARTESIAN_POINT('Ctrl Pts',(48.4906361947471,11.5755468354576,3.28398547902237));
#31754=CARTESIAN_POINT('Ctrl Pts',(48.4830998624059,11.6050189470212,3.83329117874236));
#31755=CARTESIAN_POINT('Ctrl Pts',(48.4724837048702,11.6282480883245,4.29423381231316));
#31756=CARTESIAN_POINT('Ctrl Pts',(48.5015790863104,11.4644563788109,1.83812822433663));
#31757=CARTESIAN_POINT('Ctrl Pts',(48.5003285876188,11.4748353413218,1.93670273339578));
#31758=CARTESIAN_POINT('Ctrl Pts',(48.498555988222,11.4849166217024,2.08593433631161));
#31759=CARTESIAN_POINT('Ctrl Pts',(48.4937353771472,11.508146276442,2.45901835920677));
#31760=CARTESIAN_POINT('Ctrl Pts',(48.4906923512561,11.5213343690929,2.68286794494415));
#31761=CARTESIAN_POINT('Ctrl Pts',(48.4826251618687,11.5710816706553,3.42631530142816));
#31762=CARTESIAN_POINT('Ctrl Pts',(48.4747689990924,11.5979431249203,3.91691834434268));
#31763=CARTESIAN_POINT('Ctrl Pts',(48.4652136665875,11.6172366040621,4.29500084713974));
#31764=CARTESIAN_POINT('Ctrl Pts',(48.4606829527973,11.4583384590298,2.89205060619288));
#31765=CARTESIAN_POINT('Ctrl Pts',(48.4602502314484,11.4700074930205,2.95333187694758));
#31766=CARTESIAN_POINT('Ctrl Pts',(48.4596398458099,11.481882800679,3.05034122263737));
#31767=CARTESIAN_POINT('Ctrl Pts',(48.457639336452,11.5065304546877,3.28859697245894));
#31768=CARTESIAN_POINT('Ctrl Pts',(48.4562520617537,11.5193254972046,3.42984175702388));
#31769=CARTESIAN_POINT('Ctrl Pts',(48.4521822008652,11.5598336028455,3.87910730675446));
#31770=CARTESIAN_POINT('Ctrl Pts',(48.4481398060042,11.5806510816358,4.15478254176723));
#31771=CARTESIAN_POINT('Ctrl Pts',(48.4433803641393,11.5884292819488,4.29756566916935));
#31772=CARTESIAN_POINT('Ctrl Pts',(48.4174823766521,11.4609474762041,3.59330337868378));
#31773=CARTESIAN_POINT('Ctrl Pts',(48.4187304434642,11.4731609516943,3.63027912148489));
#31774=CARTESIAN_POINT('Ctrl Pts',(48.4200748650817,11.4863352799677,3.69245653604027));
#31775=CARTESIAN_POINT('Ctrl Pts',(48.4227028837574,11.5121367174564,3.83761867075702));
#31776=CARTESIAN_POINT('Ctrl Pts',(48.4239864808157,11.5247638266716,3.92060339091839));
#31777=CARTESIAN_POINT('Ctrl Pts',(48.4273657338961,11.5581209387927,4.15637445295775));
#31778=CARTESIAN_POINT('Ctrl Pts',(48.4289898518242,11.5743267261738,4.29597769639097));
#31779=CARTESIAN_POINT('Ctrl Pts',(48.4289711156128,11.5746245276893,4.29961932362112));
#31780=CARTESIAN_POINT('Ctrl Pts',(48.3614264232796,11.4732422824942,4.29441317095744));
#31781=CARTESIAN_POINT('Ctrl Pts',(48.3663922968565,11.4851966459098,4.29446585817745));
#31782=CARTESIAN_POINT('Ctrl Pts',(48.3730775094482,11.497472006951,4.29459893941734));
#31783=CARTESIAN_POINT('Ctrl Pts',(48.3875464536895,11.5208685373805,4.29515956957329));
#31784=CARTESIAN_POINT('Ctrl Pts',(48.395330185339,11.5319897067687,4.29558711848934));
#31785=CARTESIAN_POINT('Ctrl Pts',(48.4168189204169,11.5609276470972,4.2975119862063));
#31786=CARTESIAN_POINT('Ctrl Pts',(48.4286614639743,11.5743188502015,4.29965152597602));
#31787=CARTESIAN_POINT('Ctrl Pts',(48.4286600918172,11.5746245485738,4.30318207891633));
#31788=CARTESIAN_POINT('Ctrl Pts',(48.4286600918175,11.5746245484995,4.30318207805718));
#31789=CARTESIAN_POINT('Ctrl Pts',(48.428660173147,11.5746064038391,4.30297252432489));
#31790=CARTESIAN_POINT('Ctrl Pts',(48.4286216603492,11.5745497853935,4.302816343613));
#31791=CARTESIAN_POINT('Ctrl Pts',(48.4285848981368,11.5744984448488,4.30270012134642));
#31792=CARTESIAN_POINT('Ctrl Pts',(48.4285480454769,11.574446977989,4.30258361313381));
#31793=CARTESIAN_POINT('Ctrl Pts',(48.4285118923269,11.5743997047824,4.30250737386098));
#31794=CARTESIAN_POINT('Ctrl Pts',(48.4284895565794,11.574370552647,4.30246107541817));
#31795=CARTESIAN_POINT('Ctrl Pts',(48.4284449398726,11.5743123198847,4.30236859209968));
#31796=CARTESIAN_POINT('Ctrl Pts',(48.4284142675547,11.5742733795738,4.30231835462613));
#31797=CARTESIAN_POINT('Ctrl Pts',(48.4283846331628,11.5742358022906,4.30227052046444));
#31798=CARTESIAN_POINT('Ctrl Pts',(48.4283253643788,11.5741606477241,4.30217485214104));
#31799=CARTESIAN_POINT('Ctrl Pts',(48.428273850473,11.5740963865937,4.30210514179006));
#31800=CARTESIAN_POINT('Ctrl Pts',(48.4282197552865,11.5740292687569,4.30203697502406));
#31801=CARTESIAN_POINT('Ctrl Pts',(48.4280343609139,11.5737992433141,4.3018033547035));
#31802=CARTESIAN_POINT('Ctrl Pts',(48.4278244339668,11.5735441534495,4.3016127031576));
#31803=CARTESIAN_POINT('Ctrl Pts',(48.4276145416169,11.5732903201755,4.30144691952107));
#31804=CARTESIAN_POINT('Ctrl Pts',(48.4273317964772,11.5729483823938,4.3012235930516));
#31805=CARTESIAN_POINT('Ctrl Pts',(48.4270468518926,11.5726061687629,4.30104387224263));
#31806=CARTESIAN_POINT('Ctrl Pts',(48.4267515418286,11.5722518189,4.3008773859058));
#31807=CARTESIAN_POINT('Ctrl Pts',(48.4263482983298,11.5717679570344,4.30065005016229));
#31808=CARTESIAN_POINT('Ctrl Pts',(48.4259410026168,11.571280018306,4.30045936740763));
#31809=CARTESIAN_POINT('Ctrl Pts',(48.4255334993493,11.5707911793166,4.30028708850175));
#31810=CARTESIAN_POINT('Ctrl Pts',(48.4248366295841,11.5699552176474,4.29999247500965));
#31811=CARTESIAN_POINT('Ctrl Pts',(48.4241358475905,11.5691127678625,4.29975133277005));
#31812=CARTESIAN_POINT('Ctrl Pts',(48.4234368426892,11.5682688436226,4.2995356576737));
#31813=CARTESIAN_POINT('Ctrl Pts',(48.4222570898919,11.5668445017031,4.29917164978511));
#31814=CARTESIAN_POINT('Ctrl Pts',(48.4210795566691,11.5654127733163,4.2988812226714));
#31815=CARTESIAN_POINT('Ctrl Pts',(48.4199071305588,11.5639752438872,4.29862402961716));
#31816=CARTESIAN_POINT('Ctrl Pts',(48.4180824832977,11.5617380162167,4.29822375995592));
#31817=CARTESIAN_POINT('Ctrl Pts',(48.4162697117118,11.5594864488171,4.29790736451354));
#31818=CARTESIAN_POINT('Ctrl Pts',(48.4144713964367,11.5572216877119,4.29763057295059));
#31819=CARTESIAN_POINT('Ctrl Pts',(48.4117670663131,11.5538159102244,4.2972143301638));
#31820=CARTESIAN_POINT('Ctrl Pts',(48.4090945540814,11.550379518606,4.29689092942539));
#31821=CARTESIAN_POINT('Ctrl Pts',(48.4064601460237,11.5469146454501,4.29661383979601));
#31822=CARTESIAN_POINT('Ctrl Pts',(48.4051282865519,11.545162933479,4.29647375350743));
#31823=CARTESIAN_POINT('Ctrl Pts',(48.4038056232218,11.5434032085324,4.2963463114669));
#31824=CARTESIAN_POINT('Ctrl Pts',(48.4024930970316,11.5416356868782,4.29622874106166));
#31825=CARTESIAN_POINT('Ctrl Pts',(48.3982785721702,11.5359601704501,4.295851222198));
#31826=CARTESIAN_POINT('Ctrl Pts',(48.3941689719985,11.5302068773408,4.295572141369));
#31827=CARTESIAN_POINT('Ctrl Pts',(48.390190769549,11.5243619142254,4.29534669563895));
#31828=CARTESIAN_POINT('Ctrl Pts',(48.3867923502581,11.5193687959371,4.29515410636583));
#31829=CARTESIAN_POINT('Ctrl Pts',(48.3834901365878,11.5143094032157,4.29500239890131));
#31830=CARTESIAN_POINT('Ctrl Pts',(48.3803119815688,11.5091702721658,4.29487925449532));
#31831=CARTESIAN_POINT('Ctrl Pts',(48.3767563627651,11.5034207757166,4.29474148444857));
#31832=CARTESIAN_POINT('Ctrl Pts',(48.3733540435004,11.4975716267243,4.29463972870061));
#31833=CARTESIAN_POINT('Ctrl Pts',(48.3701734723775,11.49159405132,4.29456450114538));
#31834=CARTESIAN_POINT('Ctrl Pts',(48.3675896123393,11.4867379366112,4.29450338712962));
#31835=CARTESIAN_POINT('Ctrl Pts',(48.3651512727409,11.4817961991037,4.29445995841077));
#31836=CARTESIAN_POINT('Ctrl Pts',(48.3629292995066,11.4767527247579,4.29443096808727));
#31837=CARTESIAN_POINT('Ctrl Pts',(48.3624161617827,11.4755879956304,4.29442427312426));
#31838=CARTESIAN_POINT('Ctrl Pts',(48.3619147674745,11.4744178750436,4.29441835222065));
#31839=CARTESIAN_POINT('Ctrl Pts',(48.3614264232796,11.4732422824942,4.29441317095744));
#31840=CARTESIAN_POINT('Ctrl Pts',(21.3906463937529,16.4830953098781,48.8309185363369));
#31841=CARTESIAN_POINT('Ctrl Pts',(21.4003401995189,16.4833744495148,48.4949669229311));
#31842=CARTESIAN_POINT('Ctrl Pts',(21.3997327223527,16.1481826330634,48.5190454048188));
#31843=CARTESIAN_POINT('Ctrl Pts',(21.6479745476933,16.483095324294,48.8379328597607));
#31844=CARTESIAN_POINT('Ctrl Pts',(21.6200830023851,16.483319828549,48.5460524616203));
#31845=CARTESIAN_POINT('Ctrl Pts',(21.6389642094873,16.1929802521112,48.5225608943597));
#31846=CARTESIAN_POINT('Ctrl Pts',(21.9045410908616,16.4830953387802,48.8243898617382));
#31847=CARTESIAN_POINT('Ctrl Pts',(21.8672452314961,16.483273583025,48.5750825049463));
#31848=CARTESIAN_POINT('Ctrl Pts',(21.8768838415007,16.2379895254129,48.5158004457527));
#31849=CARTESIAN_POINT('Ctrl Pts',(22.4076757669193,16.4830953673845,48.743210136482));
#31850=CARTESIAN_POINT('Ctrl Pts',(22.3511228078461,16.4831976839893,48.5682561154872));
#31851=CARTESIAN_POINT('Ctrl Pts',(22.3423318951884,16.3268490737816,48.4752349408482));
#31852=CARTESIAN_POINT('Ctrl Pts',(22.6581433216875,16.4830953816853,48.6788328743123));
#31853=CARTESIAN_POINT('Ctrl Pts',(22.5967474570195,16.4831654080667,48.5419054522021));
#31854=CARTESIAN_POINT('Ctrl Pts',(22.5727876009851,16.3712675955695,48.4432313777772));
#31855=CARTESIAN_POINT('Ctrl Pts',(22.8868233850503,16.4830953949244,48.5476959795698));
#31856=CARTESIAN_POINT('Ctrl Pts',(22.8291967273507,16.4831380278819,48.4517667232661));
#31857=CARTESIAN_POINT('Ctrl Pts',(22.7844241394783,16.4123847430248,48.3774109749067));
#31858=CARTESIAN_POINT('Ctrl Pts',(21.5192634427593,16.17060336129,48.5199317918263));
#31859=CARTESIAN_POINT('Ctrl Pts',(21.6170999500073,16.1889856471435,48.5199312682443));
#31860=CARTESIAN_POINT('Ctrl Pts',(21.7148708403879,16.2074307865443,48.518116604729));
#31861=CARTESIAN_POINT('Ctrl Pts',(21.8124883377731,16.2259200040867,48.5142156384362));
#31862=CARTESIAN_POINT('Ctrl Pts',(21.908956873748,16.2441916028821,48.5103605866552));
#31863=CARTESIAN_POINT('Ctrl Pts',(22.0052762797485,16.2625063923372,48.5044686188699));
#31864=CARTESIAN_POINT('Ctrl Pts',(22.1013380589794,16.2808424439029,48.4962332420434));
#31865=CARTESIAN_POINT('Ctrl Pts',(22.1040951139171,16.2813687042107,48.4959968797094));
#31866=CARTESIAN_POINT('Ctrl Pts',(22.1068517512828,16.2818949414479,48.4957586005132));
#31867=CARTESIAN_POINT('Ctrl Pts',(22.109607981701,16.2824211576432,48.4955183962497));
#31868=CARTESIAN_POINT('Ctrl Pts',(22.1685278155313,16.2936700614283,48.4903835587579));
#31869=CARTESIAN_POINT('Ctrl Pts',(22.2274507987805,16.3049460203239,48.4844875476039));
#31870=CARTESIAN_POINT('Ctrl Pts',(22.2862696411608,16.3162274856622,48.4774282375931));
#31871=CARTESIAN_POINT('Ctrl Pts',(22.340258020577,16.3265824672703,48.4709486692804));
#31872=CARTESIAN_POINT('Ctrl Pts',(22.3941591829442,16.3369421989583,48.4634895977143));
#31873=CARTESIAN_POINT('Ctrl Pts',(22.4478699699773,16.3472864072044,48.4547032934322));
#31874=CARTESIAN_POINT('Ctrl Pts',(22.4969660605998,16.3567418669644,48.4466718864263));
#31875=CARTESIAN_POINT('Ctrl Pts',(22.5459033047808,16.3661844046848,48.4375317183341));
#31876=CARTESIAN_POINT('Ctrl Pts',(22.5945805754926,16.3755943695783,48.4269802673523));
#31877=CARTESIAN_POINT('Ctrl Pts',(22.6221833139186,16.380930346632,48.4209970037632));
#31878=CARTESIAN_POINT('Ctrl Pts',(22.6497020262212,16.3862557688531,48.4145592382452));
#31879=CARTESIAN_POINT('Ctrl Pts',(22.677114230578,16.3915662868154,48.4076054027901));
#31880=CARTESIAN_POINT('Origin',(21.5192211643356,16.1705954176946,48.8324317919394));
#31881=CARTESIAN_POINT('Ctrl Pts',(-48.6664734316379,16.4830954176946,21.5181263879129));
#31882=CARTESIAN_POINT('Ctrl Pts',(-48.353973431638,16.4830954176946,21.5181263879129));
#31883=CARTESIAN_POINT('Ctrl Pts',(-48.3539734316379,16.1705954176947,21.5181263879129));
#31884=CARTESIAN_POINT('Ctrl Pts',(-48.6664734339897,16.4830954176946,21.7328421481057));
#31885=CARTESIAN_POINT('Ctrl Pts',(-48.3893416276193,16.4830954176967,21.7063677013623));
#31886=CARTESIAN_POINT('Ctrl Pts',(-48.3539734316379,16.208073041206,21.7175947316477));
#31887=CARTESIAN_POINT('Ctrl Pts',(-48.6512918054456,16.4830954176946,21.9468604135708));
#31888=CARTESIAN_POINT('Ctrl Pts',(-48.4085265371208,16.4830954176942,21.9119950055367));
#31889=CARTESIAN_POINT('Ctrl Pts',(-48.3463826153449,16.2456622380852,21.9159853456124));
#31890=CARTESIAN_POINT('Ctrl Pts',(-48.583556384038,16.4830954176946,22.3658173905146));
#31891=CARTESIAN_POINT('Ctrl Pts',(-48.4026513877734,16.483095417695,22.3146013303459));
#31892=CARTESIAN_POINT('Ctrl Pts',(-48.312514911035,16.3196601510152,22.3035748967492));
#31893=CARTESIAN_POINT('Ctrl Pts',(-48.5339575321232,16.4830954176946,22.5725362595963));
#31894=CARTESIAN_POINT('Ctrl Pts',(-48.3840456652921,16.483095417695,22.5162624682257));
#31895=CARTESIAN_POINT('Ctrl Pts',(-48.2878455968984,16.3562852232532,22.4939033682569));
#31896=CARTESIAN_POINT('Ctrl Pts',(-48.4418206533393,16.4830954176946,22.7696071163712));
#31897=CARTESIAN_POINT('Ctrl Pts',(-48.3245616669322,16.4830954176946,22.7147847331159));
#31898=CARTESIAN_POINT('Ctrl Pts',(-48.2416470424886,16.3915662868154,22.6760194541553));
#31899=CARTESIAN_POINT('Origin',(-48.4418206533391,16.1705954176946,22.7696071163712));
#31900=CARTESIAN_POINT('Origin',(0.0835265683620477,11.3536536794531,0.0824317919394229));
#31901=CARTESIAN_POINT('Origin',(0.0835265683620477,11.353653679453,0.0824317919394229));
#31902=CARTESIAN_POINT('Ctrl Pts',(23.2519741921975,16.8990456314821,48.5199317919394));
#31903=CARTESIAN_POINT('Ctrl Pts',(23.3105477751332,16.763953599836,48.5199317919394));
#31904=CARTESIAN_POINT('Ctrl Pts',(23.3478725606479,16.6779610536085,48.4063825502508));
#31905=CARTESIAN_POINT('Ctrl Pts',(20.1383882957297,15.5488264507417,48.5199317919394));
#31906=CARTESIAN_POINT('Ctrl Pts',(20.2055059095578,15.4217541107764,48.5199317919394));
#31907=CARTESIAN_POINT('Ctrl Pts',(20.2238169664254,15.3277344906633,48.411419729136));
#31908=CARTESIAN_POINT('Ctrl Pts',(16.9483379670617,14.3828771928117,48.5199317919394));
#31909=CARTESIAN_POINT('Ctrl Pts',(17.0044039605232,14.2535943278388,48.5199317919394));
#31910=CARTESIAN_POINT('Ctrl Pts',(17.0218205262955,14.1617844319789,48.4161700136446));
#31911=CARTESIAN_POINT('Ctrl Pts',(12.0946655778594,13.0662924545662,48.5199317919394));
#31912=CARTESIAN_POINT('Ctrl Pts',(12.1291036075007,12.9358690854399,48.5199317919394));
#31913=CARTESIAN_POINT('Ctrl Pts',(12.1482783473018,12.8452005633163,48.4217771854608));
#31914=CARTESIAN_POINT('Ctrl Pts',(10.5137170271294,12.7052707111067,48.5199317919394));
#31915=CARTESIAN_POINT('Ctrl Pts',(10.5433433501585,12.5748662546398,48.5199317919394));
#31916=CARTESIAN_POINT('Ctrl Pts',(10.5606082542232,12.4841786131435,48.4233602576764));
#31917=CARTESIAN_POINT('Ctrl Pts',(7.14883379663184,12.0967706283699,48.5199317919394));
#31918=CARTESIAN_POINT('Ctrl Pts',(7.1701748355487,11.9671239033221,48.5199317919394));
#31919=CARTESIAN_POINT('Ctrl Pts',(7.18101793127648,11.8756772045064,48.426066172497));
#31920=CARTESIAN_POINT('Ctrl Pts',(5.35745102444326,11.8673062899501,48.5199317919395));
#31921=CARTESIAN_POINT('Ctrl Pts',(5.3726385311504,11.7375302417815,48.5199317919394));
#31922=CARTESIAN_POINT('Ctrl Pts',(5.38157480191148,11.6462130006682,48.4271134458431));
#31923=CARTESIAN_POINT('Ctrl Pts',(3.55752842609651,11.7377723188913,48.5199317919395));
#31924=CARTESIAN_POINT('Ctrl Pts',(3.56686066968263,11.6080928945489,48.5199317919394));
#31925=CARTESIAN_POINT('Ctrl Pts',(3.57344661608542,11.5166787189151,48.4277053216402));
#31926=CARTESIAN_POINT('Origin',(-44.291473431638,16.1705954176946,48.8324317919394));
#31927=CARTESIAN_POINT('Origin',(-21.3521680276115,16.1705954176946,48.8324317919394));
#31928=CARTESIAN_POINT('Origin',(0.0835265683620477,16.1705954176946,0.0824317919394229));
#31929=CARTESIAN_POINT('Origin',(-22.6036487560697,16.1705954176946,48.6077790136406));
#31930=CARTESIAN_POINT('Ctrl Pts',(0.0835265683646154,11.4728541727075,
48.5199460669665));
#31931=CARTESIAN_POINT('Ctrl Pts',(0.0835265683646867,11.4942063411577,
48.5199465324602));
#31932=CARTESIAN_POINT('Ctrl Pts',(0.0835265683659855,11.5200575082527,
48.5195892904601));
#31933=CARTESIAN_POINT('Ctrl Pts',(0.0835265683637358,11.5731362269332,
48.5213546907495));
#31934=CARTESIAN_POINT('Ctrl Pts',(0.0835265683629213,11.5876793312944,
48.5199317919394));
#31935=CARTESIAN_POINT('Ctrl Pts',(0.0835265683619702,11.6131136241746,
48.5199317919394));
#31936=CARTESIAN_POINT('Ctrl Pts',(-0.267518736923682,11.47819221482,48.5199461833397));
#31937=CARTESIAN_POINT('Ctrl Pts',(-0.189316787738642,11.4971000233706,
48.519886961282));
#31938=CARTESIAN_POINT('Ctrl Pts',(-0.189103448006821,11.5200113925673,
48.519586959612));
#31939=CARTESIAN_POINT('Ctrl Pts',(-0.227816669701683,11.5731490589916,
48.5213559145826));
#31940=CARTESIAN_POINT('Ctrl Pts',(-0.266743231125736,11.5876793312944,
48.5199317919394));
#31941=CARTESIAN_POINT('Ctrl Pts',(-0.266821084249534,11.6131136241746,
48.5199317919394));
#31942=CARTESIAN_POINT('Ctrl Pts',(-0.618388066296979,11.4874426767151,
48.5184889915183));
#31943=CARTESIAN_POINT('Ctrl Pts',(-0.484920402710071,11.5031786713302,
48.5195752074935));
#31944=CARTESIAN_POINT('Ctrl Pts',(-0.484557203618662,11.524500508176,48.5196902430683));
#31945=CARTESIAN_POINT('Ctrl Pts',(-0.550623003964169,11.5776504745526,
48.5214911613193));
#31946=CARTESIAN_POINT('Ctrl Pts',(-0.617052003398677,11.5930695682598,
48.5199317919388));
#31947=CARTESIAN_POINT('Ctrl Pts',(-0.617168736861038,11.6169153282063,
48.5199317919388));
#31948=CARTESIAN_POINT('Ctrl Pts',(-1.31980082625865,11.5143737377389,48.5151613829986));
#31949=CARTESIAN_POINT('Ctrl Pts',(-1.12748086026437,11.5255419633077,48.5183112784636));
#31950=CARTESIAN_POINT('Ctrl Pts',(-1.1269213087647,11.5448479357173,48.5193460059348));
#31951=CARTESIAN_POINT('Ctrl Pts',(-1.22201691763213,11.5959692446121,48.5214366576314));
#31952=CARTESIAN_POINT('Ctrl Pts',(-1.31767207799737,11.6126245374907,48.5199317919371));
#31953=CARTESIAN_POINT('Ctrl Pts',(-1.31778153573108,11.6321221443329,48.5199317919372));
#31954=CARTESIAN_POINT('Ctrl Pts',(-1.67034425684702,11.5320543368675,48.5132909663004));
#31955=CARTESIAN_POINT('Ctrl Pts',(-1.47443454802356,11.5418711528743,48.517374142432));
#31956=CARTESIAN_POINT('Ctrl Pts',(-1.47382850347521,11.5607507931985,48.5189135245549));
#31957=CARTESIAN_POINT('Ctrl Pts',(-1.57060291962576,11.609808871885,48.5212544268116));
#31958=CARTESIAN_POINT('Ctrl Pts',(-1.66798338032313,11.6267892697563,48.5199317919361));
#31959=CARTESIAN_POINT('Ctrl Pts',(-1.66804668198961,11.6435272564279,48.5199317919363));
#31960=CARTESIAN_POINT('Ctrl Pts',(-2.72152478000237,11.5986492866067,48.5108119661587));
#31961=CARTESIAN_POINT('Ctrl Pts',(-2.60108318318851,11.612020620858,48.5172046544326));
#31962=CARTESIAN_POINT('Ctrl Pts',(-2.60045731731407,11.6290600690797,48.5194534619891));
#31963=CARTESIAN_POINT('Ctrl Pts',(-2.6593197052731,11.6658592241824,48.5212339924693));
#31964=CARTESIAN_POINT('Ctrl Pts',(-2.71880795910599,11.6794362415569,48.5199317919341));
#31965=CARTESIAN_POINT('Ctrl Pts',(-2.7185946017063,11.689147704808,48.5199317919344));
#31966=CARTESIAN_POINT('Ctrl Pts',(-3.42379713716555,11.6392592214936,48.5061181031666));
#31967=CARTESIAN_POINT('Ctrl Pts',(-3.35185488688305,11.6580360440914,48.5141149281055));
#31968=CARTESIAN_POINT('Ctrl Pts',(-3.35085409224963,11.678564828469,48.5175683502973));
#31969=CARTESIAN_POINT('Ctrl Pts',(-3.38453260249245,11.7135824344713,48.5204767822116));
#31970=CARTESIAN_POINT('Ctrl Pts',(-3.4192119073687,11.728071256096,48.5199317919341));
#31971=CARTESIAN_POINT('Ctrl Pts',(-3.41862985610554,11.734768153188,48.5199317919344));
#31972=CARTESIAN_POINT('Ctrl Pts',(-4.12551258849121,11.6756605207398,48.4959174422581));
#31973=CARTESIAN_POINT('Ctrl Pts',(-4.12419588877397,11.6996409410726,48.5059136087032));
#31974=CARTESIAN_POINT('Ctrl Pts',(-4.12290068805218,11.7229366511894,48.5119171961235));
#31975=CARTESIAN_POINT('Ctrl Pts',(-4.12038695498645,11.7642258753786,48.5189262877417));
#31976=CARTESIAN_POINT('Ctrl Pts',(-4.11916842264252,11.7822193894509,48.5199317919394));
#31977=CARTESIAN_POINT('Ctrl Pts',(-4.11800505968102,11.7955954176946,48.5199317919394));
#31978=CARTESIAN_POINT('Origin',(-4.11644600935663,11.7956965877495,48.2062629115074));
#31979=CARTESIAN_POINT('Ctrl Pts',(-21.3521680276115,16.1705954176947,48.5199317919394));
#31980=CARTESIAN_POINT('Ctrl Pts',(-21.3521680276115,16.4830954176946,48.5199317919395));
#31981=CARTESIAN_POINT('Ctrl Pts',(-21.3521680276115,16.4830954176946,48.8324317919394));
#31982=CARTESIAN_POINT('Ctrl Pts',(-21.5512737421848,16.208004907791,48.5199317919394));
#31983=CARTESIAN_POINT('Ctrl Pts',(-21.5400855159438,16.4830954176967,48.5552391421598));
#31984=CARTESIAN_POINT('Ctrl Pts',(-21.566494676323,16.4830954176946,48.8324317919409));
#31985=CARTESIAN_POINT('Ctrl Pts',(-21.7482599692405,16.2453260884686,48.5124525747896));
#31986=CARTESIAN_POINT('Ctrl Pts',(-21.7441579658526,16.4830954176946,48.5744206138524));
#31987=CARTESIAN_POINT('Ctrl Pts',(-21.7789938361076,16.4830954176946,48.8174733646386));
#31988=CARTESIAN_POINT('Ctrl Pts',(-22.1369289600096,16.3195276817375,48.4785758857753));
#31989=CARTESIAN_POINT('Ctrl Pts',(-22.1478705006132,16.4830954176946,48.5687045084598));
#31990=CARTESIAN_POINT('Ctrl Pts',(-22.1991140172779,16.4830954176946,48.7497199726123));
#31991=CARTESIAN_POINT('Ctrl Pts',(-22.3313759293136,16.3569498947407,48.4529336183403));
#31992=CARTESIAN_POINT('Ctrl Pts',(-22.3540938889857,16.4830954176935,48.5488684947966));
#31993=CARTESIAN_POINT('Ctrl Pts',(-22.4101480350136,16.4830954176946,48.6982467590681));
#31994=CARTESIAN_POINT('Ctrl Pts',(-22.5100610938555,16.3915662868148,48.4076054027924));
#31995=CARTESIAN_POINT('Ctrl Pts',(-22.548826372816,16.4830954176946,48.4905200272361));
#31996=CARTESIAN_POINT('Ctrl Pts',(-22.6036487560711,16.4830954176946,48.6077790136438));
#31997=CARTESIAN_POINT('Ctrl Pts',(-22.510061093855,16.3915662868147,48.4076054027925));
#31998=CARTESIAN_POINT('Ctrl Pts',(-22.470838026846,16.3839676712791,48.4175553780106));
#31999=CARTESIAN_POINT('Ctrl Pts',(-22.4313616813393,16.3763319926636,48.4264324211722));
#32000=CARTESIAN_POINT('Ctrl Pts',(-22.3917296389681,16.3686778876786,48.4344340496838));
#32001=CARTESIAN_POINT('Ctrl Pts',(-22.3479890308505,16.3602302986418,48.4432651892387));
#32002=CARTESIAN_POINT('Ctrl Pts',(-22.3040585025035,16.3517602066229,48.451029983322));
#32003=CARTESIAN_POINT('Ctrl Pts',(-22.2600230793043,16.3432839722933,48.4579483574562));
#32004=CARTESIAN_POINT('Ctrl Pts',(-22.2124872920991,16.3341339643652,48.4654166712991));
#32005=CARTESIAN_POINT('Ctrl Pts',(-22.1648284589081,16.3249766329791,48.4718982624129));
#32006=CARTESIAN_POINT('Ctrl Pts',(-22.1171112171318,16.3158247537685,48.4776226213431));
#32007=CARTESIAN_POINT('Ctrl Pts',(-22.0590026864533,16.3046798880117,48.4845935625403));
#32008=CARTESIAN_POINT('Ctrl Pts',(-22.0008060837811,16.2935427876858,48.4904415667607));
#32009=CARTESIAN_POINT('Ctrl Pts',(-21.942594596444,16.2824290454294,48.4955150476558));
#32010=CARTESIAN_POINT('Ctrl Pts',(-21.9397573875572,16.2818873652605,48.4957623274581));
#32011=CARTESIAN_POINT('Ctrl Pts',(-21.9369195504994,16.2813456246244,48.4960075961641));
#32012=CARTESIAN_POINT('Ctrl Pts',(-21.9340810451365,16.28080381591,48.496250863188));
#32013=CARTESIAN_POINT('Ctrl Pts',(-21.8165634625776,16.2583722745907,48.5063224145554));
#32014=CARTESIAN_POINT('Ctrl Pts',(-21.6987927520804,16.2359974208102,48.5128922231434));
#32015=CARTESIAN_POINT('Ctrl Pts',(-21.5808083365145,16.21368980715,48.5165038490348));
#32016=CARTESIAN_POINT('Ctrl Pts',(-21.5046957442586,16.199299005665,48.5188337347873));
#32017=CARTESIAN_POINT('Ctrl Pts',(-21.4284939067714,16.1849361189809,48.5199313850954));
#32018=CARTESIAN_POINT('Ctrl Pts',(-21.3522104186698,16.1706033824526,48.5199317918264));
#32019=CARTESIAN_POINT('Ctrl Pts',(-22.754424611923,16.495117042058,48.4071618265161));
#32020=CARTESIAN_POINT('Ctrl Pts',(-22.7176017202102,16.581294338131,48.5199317919394));
#32021=CARTESIAN_POINT('Ctrl Pts',(-22.6599908629307,16.7161293328258,48.5199317919394));
#32022=CARTESIAN_POINT('Ctrl Pts',(-19.765550405457,15.2224248747711,48.4119403012087));
#32023=CARTESIAN_POINT('Ctrl Pts',(-19.7460226280874,15.3157731528558,48.5199317919394));
#32024=CARTESIAN_POINT('Ctrl Pts',(-19.6812252681849,15.4434377928151,48.5199317919394));
#32025=CARTESIAN_POINT('Ctrl Pts',(-16.7040650491873,14.1211388855287,48.4164308930203));
#32026=CARTESIAN_POINT('Ctrl Pts',(-16.6858002353668,14.2126904029842,48.5199317919394));
#32027=CARTESIAN_POINT('Ctrl Pts',(-16.6312111874939,14.3421540083754,48.5199317919394));
#32028=CARTESIAN_POINT('Ctrl Pts',(-11.9808374649863,12.8451845281724,48.4218608844626));
#32029=CARTESIAN_POINT('Ctrl Pts',(-11.9616626207849,12.9358419174536,48.5199317919394));
#32030=CARTESIAN_POINT('Ctrl Pts',(-11.9272425168244,13.0661994464424,48.5199317919394));
#32031=CARTESIAN_POINT('Ctrl Pts',(-10.3932306187778,12.4841939488199,48.4234426080441));
#32032=CARTESIAN_POINT('Ctrl Pts',(-10.3759657149212,12.5748700381561,48.5199317919394));
#32033=CARTESIAN_POINT('Ctrl Pts',(-10.3463554047103,12.7052089420493,48.5199317919394));
#32034=CARTESIAN_POINT('Ctrl Pts',(-7.1674989354977,11.9034070977967,48.4260232871746));
#32035=CARTESIAN_POINT('Ctrl Pts',(-7.15598924266794,11.9947391304937,48.5199317919394));
#32036=CARTESIAN_POINT('Ctrl Pts',(-7.13465594337445,12.1244225185051,48.5199317919394));
#32037=CARTESIAN_POINT('Ctrl Pts',(-5.52308711228244,11.6863323981099,48.4270102837803));
#32038=CARTESIAN_POINT('Ctrl Pts',(-5.51351080050052,11.7776141640752,48.5199317919394));
#32039=CARTESIAN_POINT('Ctrl Pts',(-5.49759056885458,11.9073477673264,48.5199317919394));
#32040=CARTESIAN_POINT('Ctrl Pts',(-3.87138954853958,11.5522837202171,48.4276218721885));
#32041=CARTESIAN_POINT('Ctrl Pts',(-3.86394066580964,11.6436417565348,48.5199317919394));
#32042=CARTESIAN_POINT('Ctrl Pts',(-3.85336951301254,11.7732992268532,48.5199317919394));
#32043=CARTESIAN_POINT('Origin',(44.4585265683622,-14.4544045823054,-44.2925682080604));
#32044=CARTESIAN_POINT('Origin',(49.7710265683622,-14.4544045823054,-44.2925682080604));
#32045=CARTESIAN_POINT('Origin',(44.4585265683622,-14.4544045823054,-49.6050682080604));
#32046=CARTESIAN_POINT('Origin',(0.0835265683620477,-14.4544045823054,-49.6050682080606));
#32047=CARTESIAN_POINT('Origin',(-44.2914734316379,-14.4544045823054,-49.6050682080606));
#32048=CARTESIAN_POINT('Origin',(49.7710265683621,-14.4544045823054,0.0824317919395964));
#32049=CARTESIAN_POINT('Origin',(49.7710265683619,-14.4544045823054,36.6697170232579));
#32050=CARTESIAN_POINT('Origin',(-44.291473431638,-14.4544045823054,-44.2925682080606));
#32051=CARTESIAN_POINT('Origin',(-49.603973431638,-14.4544045823054,-44.2925682080605));
#32052=CARTESIAN_POINT('Origin',(44.4585265683621,-14.4544045823054,44.4574317919394));
#32053=CARTESIAN_POINT('Origin',(44.458526568362,-14.4544045823054,49.7699317919394));
#32054=CARTESIAN_POINT('Origin',(-49.603973431638,-14.4544045823054,0.0824317919394229));
#32055=CARTESIAN_POINT('Origin',(-49.603973431638,-14.4544045823054,44.4574317919389));
#32056=CARTESIAN_POINT('Origin',(0.0835265683620476,-14.4544045823054,49.7699317919394));
#32057=CARTESIAN_POINT('Origin',(-44.2914734316384,-14.4544045823054,49.7699317919394));
#32058=CARTESIAN_POINT('Origin',(-44.2914734316384,-14.4544045823054,44.457431791939));
#32059=CARTESIAN_POINT('Origin',(44.4585265683622,16.1705954176946,-44.2925682080604));
#32060=CARTESIAN_POINT('Origin',(49.7710265683622,16.1705954176946,-44.2925682080604));
#32061=CARTESIAN_POINT('Origin',(44.4585265683622,16.1705954176946,-49.6050682080604));
#32062=CARTESIAN_POINT('Origin',(-44.291473431638,16.1705954176946,-49.6050682080606));
#32063=CARTESIAN_POINT('Origin',(-44.2914734316379,16.1705954176946,-49.6050682080606));
#32064=CARTESIAN_POINT('Origin',(49.7710265683622,16.1705954176946,-44.2925682080603));
#32065=CARTESIAN_POINT('Origin',(49.7710265683619,16.1705954176946,36.6697170232579));
#32066=CARTESIAN_POINT('Origin',(-44.291473431638,16.1705954176946,-44.2925682080606));
#32067=CARTESIAN_POINT('Origin',(-49.603973431638,16.1705954176946,-44.2925682080605));
#32068=CARTESIAN_POINT('Origin',(44.4585265683621,16.1705954176946,44.4574317919394));
#32069=CARTESIAN_POINT('Origin',(44.458526568362,16.1705954176946,49.7699317919394));
#32070=CARTESIAN_POINT('Origin',(-49.603973431638,16.1705954176946,-44.2925682080606));
#32071=CARTESIAN_POINT('Origin',(-49.603973431638,16.1705954176946,44.4574317919389));
#32072=CARTESIAN_POINT('Origin',(-44.2914734316379,16.1705954176946,49.7699317919394));
#32073=CARTESIAN_POINT('Origin',(-44.2914734316384,16.1705954176946,49.7699317919394));
#32074=CARTESIAN_POINT('Origin',(-44.2914734316384,16.1705954176946,44.457431791939));
#32075=CARTESIAN_POINT('Origin',(44.4585265683621,16.1705954176946,44.4574317919394));
#32076=CARTESIAN_POINT('Origin',(41.173224139993,16.1705954176946,46.8471376742924));
#32077=CARTESIAN_POINT('Origin',(40.162361854341,16.1705954176946,47.5824317919394));
#32078=CARTESIAN_POINT('Origin',(40.162361854341,16.1705954176946,48.8324317919394));
#32079=CARTESIAN_POINT('Origin',(48.8335265683621,16.1705954176946,42.8336341598436));
#32080=CARTESIAN_POINT('Origin',(48.8335265683621,16.1705954176946,35.8884670232579));
#32081=CARTESIAN_POINT('Origin',(48.8335265683621,16.1705954176946,29.6248403980433));
#32082=CARTESIAN_POINT('Origin',(26.1374820022305,16.1705954176946,48.8324317919394));
#32083=CARTESIAN_POINT('Origin',(29.625935174466,16.1705954176946,48.8324317919394));
#32084=CARTESIAN_POINT('Origin',(47.583526568362,16.1705954176946,29.6248403980433));
#32085=CARTESIAN_POINT('Origin',(46.5220740543956,16.1705954176946,28.9646748425997));
#32086=CARTESIAN_POINT('Origin',(29.625935174466,16.1705954176946,47.5824317919394));
#32087=CARTESIAN_POINT('Origin',(28.9657696190223,16.1705954176946,46.5209792779729));
#32088=CARTESIAN_POINT('Origin',(0.0835265683620477,16.1705954176946,0.0824317919394229));
#32089=CARTESIAN_POINT('Origin',(44.4585265683621,15.8580954176946,44.4574317919394));
#32090=CARTESIAN_POINT('Origin',(40.667792997167,15.8580954176946,47.2147847331159));
#32091=CARTESIAN_POINT('Origin',(40.162361854341,15.8580954176946,47.5824317919394));
#32092=CARTESIAN_POINT('Origin',(40.162361854341,15.8580954176946,48.2074317919394));
#32093=CARTESIAN_POINT('Origin',(48.2085265683621,15.8580954176946,0.0824317919394229));
#32094=CARTESIAN_POINT('Origin',(48.2085265683621,15.8580954176946,35.8884670232579));
#32095=CARTESIAN_POINT('Origin',(48.2085265683621,15.8580954176946,29.6248403980433));
#32096=CARTESIAN_POINT('Origin',(0.0835265683619977,15.8580954176946,48.2074317919394));
#32097=CARTESIAN_POINT('Origin',(29.625935174466,15.8580954176946,48.2074317919394));
#32098=CARTESIAN_POINT('Origin',(47.583526568362,15.8580954176946,29.6248403980433));
#32099=CARTESIAN_POINT('Origin',(47.0528003113788,15.8580954176946,29.2947576203215));
#32100=CARTESIAN_POINT('Origin',(29.625935174466,15.8580954176946,47.5824317919394));
#32101=CARTESIAN_POINT('Origin',(29.2958523967441,15.8580954176946,47.0517055349562));
#32102=CARTESIAN_POINT('Origin',(0.0835265683620477,15.8580954176946,0.0824317919394229));
#32103=CARTESIAN_POINT('Origin',(40.1623618543411,16.1705954176946,-47.4175682080604));
#32104=CARTESIAN_POINT('Origin',(40.1623618543411,16.1705954176946,-48.6675682080604));
#32105=CARTESIAN_POINT('Origin',(47.5835265683622,16.1705954176946,-39.9964034940393));
#32106=CARTESIAN_POINT('Origin',(48.8335265683622,16.1705954176946,-39.9964034940393));
#32107=CARTESIAN_POINT('Origin',(42.8347289362664,16.1705954176946,-48.6675682080604));
#32108=CARTESIAN_POINT('Origin',(29.6259351744661,16.1705954176946,-48.6675682080605));
#32109=CARTESIAN_POINT('Origin',(48.8335265683621,16.1705954176946,-25.9715236419289));
#32110=CARTESIAN_POINT('Origin',(29.6259351744661,16.1705954176946,-47.4175682080605));
#32111=CARTESIAN_POINT('Origin',(28.9657696190224,16.1705954176946,-46.356115694094));
#32112=CARTESIAN_POINT('Origin',(0.0835265683620477,16.1705954176946,0.0824317919394229));
#32113=CARTESIAN_POINT('Origin',(40.1623618543411,15.8580954176946,-47.4175682080604));
#32114=CARTESIAN_POINT('Origin',(40.1623618543411,15.8580954176946,-48.0425682080604));
#32115=CARTESIAN_POINT('Origin',(47.5835265683622,15.8580954176946,-39.9964034940393));
#32116=CARTESIAN_POINT('Origin',(48.2085265683622,15.8580954176946,-39.9964034940393));
#32117=CARTESIAN_POINT('Origin',(0.0835265683622157,15.8580954176946,-48.0425682080606));
#32118=CARTESIAN_POINT('Origin',(29.6259351744661,15.8580954176946,-48.0425682080605));
#32119=CARTESIAN_POINT('Origin',(48.208526568362,15.8580954176946,0.0824317919396409));
#32120=CARTESIAN_POINT('Origin',(29.6259351744661,15.8580954176946,-47.4175682080605));
#32121=CARTESIAN_POINT('Origin',(29.2958523967443,15.8580954176946,-46.8868419510772));
#32122=CARTESIAN_POINT('Origin',(0.0835265683620477,15.8580954176946,0.0824317919394229));
#32123=CARTESIAN_POINT('Origin',(-47.4164734316379,16.1705954176946,-39.9964034940395));
#32124=CARTESIAN_POINT('Origin',(-48.6664734316379,16.1705954176946,-39.9964034940395));
#32125=CARTESIAN_POINT('Origin',(-39.9953087176169,16.1705954176946,-47.4175682080606));
#32126=CARTESIAN_POINT('Origin',(-39.9953087176169,16.1705954176946,-48.6675682080606));
#32127=CARTESIAN_POINT('Origin',(-48.6664734316379,16.1705954176946,-42.6687705759647));
#32128=CARTESIAN_POINT('Origin',(-25.9704288655064,16.1705954176946,-48.6675682080606));
#32129=CARTESIAN_POINT('Origin',(-29.4588820377419,16.1705954176946,-48.6675682080606));
#32130=CARTESIAN_POINT('Origin',(-29.4588820377419,16.1705954176946,-47.4175682080606));
#32131=CARTESIAN_POINT('Origin',(-28.7987164822982,16.1705954176946,-46.3561156940941));
#32132=CARTESIAN_POINT('Origin',(0.0835265683620477,16.1705954176946,0.0824317919394229));
#32133=CARTESIAN_POINT('Origin',(-47.4164734316379,15.8580954176946,-39.9964034940395));
#32134=CARTESIAN_POINT('Origin',(-48.0414734316379,15.8580954176946,-39.9964034940395));
#32135=CARTESIAN_POINT('Origin',(-39.9953087176169,15.8580954176946,-47.4175682080606));
#32136=CARTESIAN_POINT('Origin',(-39.9953087176169,15.8580954176946,-48.0425682080606));
#32137=CARTESIAN_POINT('Origin',(-48.0414734316379,15.8580954176946,0.0824317919394229));
#32138=CARTESIAN_POINT('Origin',(0.0835265683620977,15.8580954176946,-48.0425682080605));
#32139=CARTESIAN_POINT('Origin',(-29.4588820377419,15.8580954176946,-48.0425682080606));
#32140=CARTESIAN_POINT('Origin',(-29.4588820377419,15.8580954176946,-47.4175682080606));
#32141=CARTESIAN_POINT('Origin',(-29.1287992600201,15.8580954176946,-46.8868419510773));
#32142=CARTESIAN_POINT('Origin',(0.0835265683620477,15.8580954176946,0.0824317919394229));
#32143=CARTESIAN_POINT('Origin',(0.0835265683620477,-12.5794045823054,0.0824317919394229));
#32144=CARTESIAN_POINT('',(7.59696574233659,-12.5794045823054,18.6174859267129));
#32145=CARTESIAN_POINT('',(-6.17974956131282,-12.5794045823054,19.076414315977));
#32146=CARTESIAN_POINT('Origin',(-5.38208978662056,-12.5794045823054,16.6574349341085));
#32147=CARTESIAN_POINT('',(7.67510093260532,-12.5794045823054,20.9630507178886));
#32148=CARTESIAN_POINT('',(15.3925785990455,-12.5794045823054,23.5078932009404));
#32149=CARTESIAN_POINT('Origin',(-6.17974956131282,-12.5794045823054,19.076414315977));
#32150=CARTESIAN_POINT('',(46.9585265683621,-12.5794045823054,36.5987899438301));
#32151=CARTESIAN_POINT('',(14.5949188243533,-17.1192738307565,25.9268725828089));
#32152=CARTESIAN_POINT('',(44.4818701996542,-11.3294045823054,35.7821111511702));
#32153=CARTESIAN_POINT('',(16.3756046859818,-11.3294045823054,26.5140547199659));
#32154=CARTESIAN_POINT('',(44.4818701996542,17.4534666579714,35.7821111511702));
#32155=CARTESIAN_POINT('Origin',(8.06655569071,-12.5794045823054,19.7759268101363));
#32156=CARTESIAN_POINT('Origin',(0.0835265683620477,-11.3294045823054,0.0824317919394229));
#32157=CARTESIAN_POINT('Origin',(0.0835265683620477,-10.0794045823054,0.0824317919394229));
#32158=CARTESIAN_POINT('Origin',(0.0835265683620477,-14.4544045823054,0.0824317919394229));
#32159=CARTESIAN_POINT('Origin',(17.9541833518389,-17.1192738307565,25.7183855703182));
#32160=CARTESIAN_POINT('',(18.353013239185,-11.3294045823054,24.508895879384));
#32161=CARTESIAN_POINT('',(18.353013239185,-11.3294045823054,24.508895879384));
#32162=CARTESIAN_POINT('',(18.353013239185,-11.3294045823054,24.508895879384));
#32163=CARTESIAN_POINT('Origin',(14.5949188243533,-17.1192738307565,25.9268725828089));
#32164=CARTESIAN_POINT('Origin',(48.8335265683621,-11.3294045823054,37.2170722197182));
#32165=CARTESIAN_POINT('',(48.8335265683621,21.5220065103812,36.6697170232579));
#32166=CARTESIAN_POINT('',(48.8335265683621,-11.3294045823054,34.5598618267976));
#32167=CARTESIAN_POINT('Origin',(48.8335265683621,-11.3294045823054,34.5598618267976));
#32168=CARTESIAN_POINT('',(45.272154845105,-11.3294045823054,33.3854975524836));
#32169=CARTESIAN_POINT('',(45.272154845105,17.4534666579714,33.3854975524836));
#32170=CARTESIAN_POINT('',(48.8335265683621,-11.3294045823054,34.5598618267976));
#32171=CARTESIAN_POINT('Origin',(16.7670594440865,-11.3294045823054,25.3269308122136));
#32172=CARTESIAN_POINT('',(44.4818701996542,-11.3294045823054,35.7821111511702));
#32173=CARTESIAN_POINT('Origin',(0.0835265683620477,21.5220065103812,37.6072170232579));
#32174=CARTESIAN_POINT('',(48.8335265683621,21.5220065103812,37.6072170232579));
#32175=CARTESIAN_POINT('Origin',(48.8335265683619,21.5220065103812,0.0824317919392537));
#32176=CARTESIAN_POINT('',(48.8335265683621,21.5220065103812,38.3884670232579));
#32177=CARTESIAN_POINT('Origin',(46.9585265683619,21.5220065103812,0.0824317919392602));
#32178=CARTESIAN_POINT('',(46.9585265683621,21.5220065103812,38.3884670232579));
#32179=CARTESIAN_POINT('Origin',(0.0835265683620477,21.5220065103812,36.6697170232579));
#32180=CARTESIAN_POINT('Origin',(0.0835265683620477,21.5220065103812,38.3884670232579));
#32181=CARTESIAN_POINT('Origin',(0.0835265683620477,21.5220065103812,37.6072170232579));
#32182=CARTESIAN_POINT('',(48.8335265683621,21.5220065103812,37.6072170232579));
#32183=CARTESIAN_POINT('Origin',(48.8335265683619,21.5220065103812,0.0824317919392537));
#32184=CARTESIAN_POINT('',(48.8335265683621,21.5220065103812,38.3884670232579));
#32185=CARTESIAN_POINT('Origin',(0.0835265683620477,21.5220065103812,38.3884670232579));
#32186=CARTESIAN_POINT('',(46.9585265683621,21.5220065103812,38.3884670232579));
#32187=CARTESIAN_POINT('Origin',(0.0835265683620477,21.5220065103812,36.6697170232579));
#32188=CARTESIAN_POINT('',(48.8335265683621,21.5220065103812,36.6697170232579));
#32189=CARTESIAN_POINT('Origin',(48.8335265683619,21.5220065103812,0.0824317919392537));
#32190=CARTESIAN_POINT('',(48.8335265683621,21.5220065103812,35.8884670232579));
#32191=CARTESIAN_POINT('Origin',(0.0835265683620477,21.5220065103812,35.8884670232579));
#32192=CARTESIAN_POINT('',(46.958526568362,21.5220065103812,35.8884670232579));
#32193=CARTESIAN_POINT('Origin',(46.9585265683619,21.5220065103812,0.0824317919392602));
#32194=CARTESIAN_POINT('Origin',(44.4818701996542,17.4534666579714,35.7821111511702));
#37619=UNCERTAINTY_MEASURE_WITH_UNIT(LENGTH_MEASURE(0.01),#37626,
'DISTANCE_ACCURACY_VALUE',
'Maximum model space distance between geometric entities at asserted c
onnectivities');
#37621=UNCERTAINTY_MEASURE_WITH_UNIT(LENGTH_MEASURE(0.01),#37626,
'DISTANCE_ACCURACY_VALUE',
'Maximum model space distance between geometric entities at asserted c
onnectivities');
#37623=(
GEOMETRIC_REPRESENTATION_CONTEXT(3)
GLOBAL_UNCERTAINTY_ASSIGNED_CONTEXT((#37619))
GLOBAL_UNIT_ASSIGNED_CONTEXT((#37626,#37628,#37629))
REPRESENTATION_CONTEXT('','3D')
);
#37625=(
GEOMETRIC_REPRESENTATION_CONTEXT(3)
GLOBAL_UNCERTAINTY_ASSIGNED_CONTEXT((#37621))
GLOBAL_UNIT_ASSIGNED_CONTEXT((#37626,#37628,#37629))
REPRESENTATION_CONTEXT('','3D')
);
#37626=(
LENGTH_UNIT()
NAMED_UNIT(*)
SI_UNIT(.MILLI.,.METRE.)
);
#37628=(
NAMED_UNIT(*)
PLANE_ANGLE_UNIT()
SI_UNIT($,.RADIAN.)
);
#37629=(
NAMED_UNIT(*)
SI_UNIT($,.STERADIAN.)
SOLID_ANGLE_UNIT()
);
#37631=SHAPE_DEFINITION_REPRESENTATION(#37634,#37639);
#37634=PRODUCT_DEFINITION_SHAPE('',$,#37643);
#37639=SHAPE_REPRESENTATION('',(#11523),#37623);
#37641=PRODUCT_DEFINITION_CONTEXT('part definition',#37652,'design');
#37643=PRODUCT_DEFINITION('Part 1 - Rim','Part 1 - Rim',#37646,#37641);
#37646=PRODUCT_DEFINITION_FORMATION('',$,#37655);
#37652=APPLICATION_CONTEXT(
'Core Data for Automotive Mechanical Design Process');
#37653=PRODUCT_CONTEXT('part definition',#37652,'mechanical');
#37655=PRODUCT('Part 1 - Rim','Part 1 - Rim',$,(#37653));
#37658=PRESENTATION_STYLE_ASSIGNMENT((#37661));
#37661=SURFACE_STYLE_USAGE(.BOTH.,#37664);
#37664=SURFACE_SIDE_STYLE('',(#37667));
#37667=SURFACE_STYLE_FILL_AREA(#37670);
#37670=FILL_AREA_STYLE('Opaque(97,158,199)',(#37673));
#37673=FILL_AREA_STYLE_COLOUR('Opaque(97,158,199)',#37676);
#37676=COLOUR_RGB('Opaque(97,158,199)',0.380392156862745,0.619607843137255,
0.780392156862745);
ENDSEC;
END-ISO-10303-21;
